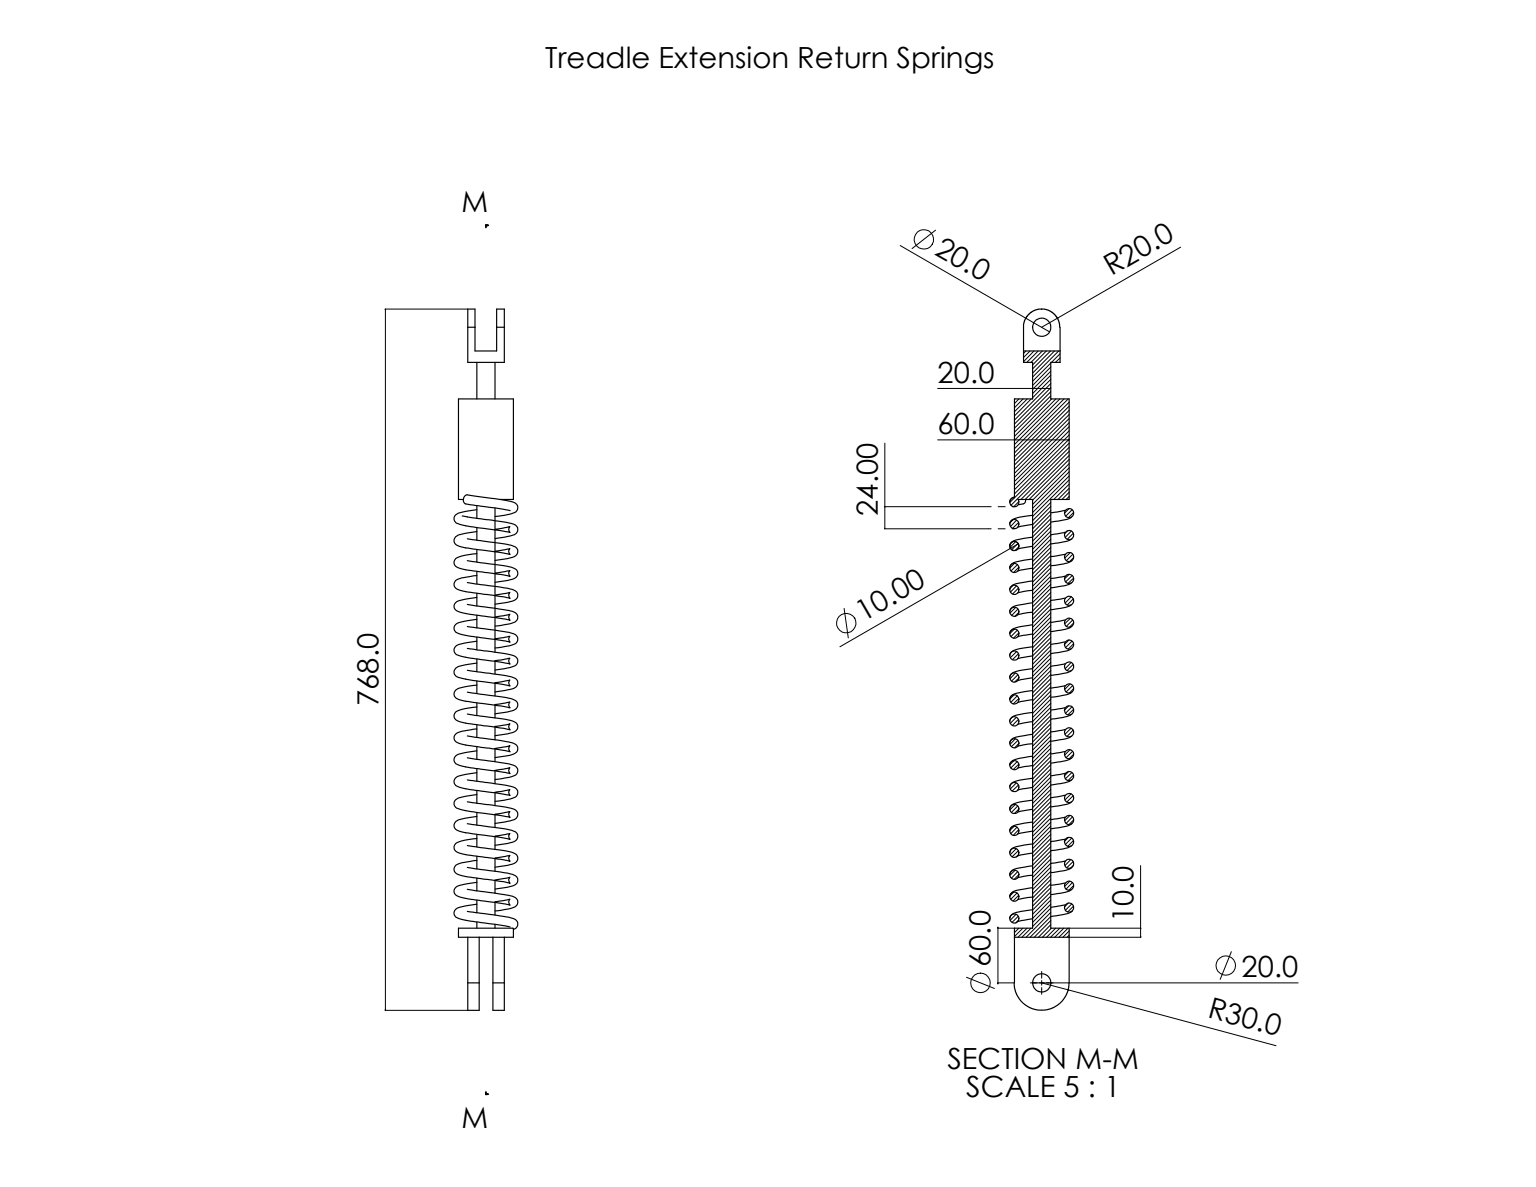
ISO-10303-21;
HEADER;
FILE_DESCRIPTION (('STEP AP214'),
    '1' );
FILE_NAME ('Treadle Extension Return Springs.step',
    '2026-10-21T17:07:05',
    ( '' ),
    ( '' ),
    'SwSTEP 2.0',
    'SolidWorks 2025',
    '' );
FILE_SCHEMA (( 'AUTOMOTIVE_DESIGN' ));
ENDSEC;

DATA;
#1=CARTESIAN_POINT ( 'NONE',  ( 745.1769319972822814, -41.80559628986934229, -346.2694204179732083 ) ) ;
#2=CARTESIAN_POINT ( 'NONE',  ( 764.0069404352550464, -207.0783235625960685, -359.2566176426627180 ) ) ;
#5=( BOUNDED_CURVE ( )  B_SPLINE_CURVE ( 2, ( #42977, #27813, #34735, #31272, #11342, #6564, #43210, #24332, #11582, #18730, #45142, #13500, #10036, #41910, #10254, #1170, #25872, #11803, #43435, #23072, #9239, #22634, #8789, #2069, #32818, #29794, #39983, #36732, #8332, #5090, #40437, #18964, #26092, #37170, #33058, #30023, #43655, #1395, #5529, #15499, #33484, #44108, #12472, #23310, #5303, #15279, #37412, #22395, #5769, #44335, #36499, #29579, #1830, #4863, #29365, #26551, #22857, #19625, #33720, #12025, #40649, #40206, #8568, #36950, #19181, #16161, #33266, #30243, #12690, #26770, #1612, #19399, #15711, #15939, #43874, #12253, #26333, #9002, #40875, #10150, #30713, #2768, #31156, #19857, #37866, #12929, #13166, #27016, #27245, #16861, #37632, #16626, #2991, #23530, #9913, #34150, #5983, #34634, #20075, #27462, #30941, #23985, #24225, #41115, #45034, #20540, #41337, #2520, #17078, #6462, #13390, #45254, #13613, #9467, #44568, #44809, #9687, #23751, #6212, #20305, #34397, #38106, #41560, #41801, #2288, #16387, #38333, #27697, #6679, #33937, #30466, #15422, #12398, #1747, #26925, #19779, #41028, #9388, #44026, #23223, #23455, #33195, #36878, #12841, #8717, #20002, #22552, #9151, #5912, #29712, #34079, #37554, #2216, #29500, #43572, #5445, #30169, #11940, #22783, #8482, #26008, #43789, #19319, #16085, #5228, #40579, #33403, #33863, #12618, #26252, #15629, #5690, #12171, #44260, #19540, #40117, #26477, #26696, #33635, #15854, #29942, #1532, #16310, #37328, #1988, #30392, #44485, #19108, #36657, #40365, #8925, #5017, #22995, #37090, #40793, #41950, #41259, #37788, #45414, #7068, #13775, #27854, #23906, #13537, #9837, #2443, #45176, #34552, #13999, #6822, #28067, #42163, #31078, #10291, #10514, #21149, #17466, #24367, #41720, #10074, #9615, #38471, #38706, #16781, #16545, #24589, #34998, #30630, #44725, #38254, #17221, #13088, #41483, #23677, #27171, #38027, #6137, #20227, #6382, #27611, #34315, #20901, #2684, #20678, #30861, #44955, #13312, #27388, #20463, #2911, #17001, #3131, #24145, #6600, #3375, #34768, #31548, #45650, #31306, #14912, #129, #7303, #25284, #14218, #22057, #14460, #39636, #15137, #18602, #39862, #7748, #17698, #21827, #3611, #28288, #42386, #10757, #25523, #11673, #10994, #31759, #24833, #4055, #29230, #32687, #35920, #38953, #25750, #43305, #11439, #28993, #21380, #32231, #8203, #35454, #4291, #35231, #3826, #25062, #1034, #28537, #17915, #39175, #7525, #810, #31985, #356, #42632, #21599, #35679, #18156, #591, #18382, #14693, #42848, #28769, #11215, #39397, #32462, #43074, #7991, #36147, #4509, #5627, #30330, #11887, #1692, #26638, #29661, #33579, #33143, #44424, #37267, #30115, #12115, #40065, #43737, #15796, #12561, #1930, #8664, #32923, #15579, #43521, #26859, #26196, #40311, #12778, #5175, #33808, #29886, #25959, #18831, #43973, #19052, #19721, #15367, #37036, #8426, #16253, #26424, #4729, #40734, #1268, #36823, #2162, #40968, #40524, #29448, #22271, #36367, #44203, #16033, #22495, #19261, #36606, #4960, #12348, #1479, #22726, #33350, #8875, #22939, #9090, #5388, #19482, #23158, #37501, #27335, #5861, #31026, #30804, #17168, #10234, #2854, #17407, #16481, #41428, #34247, #9779, #27554, #3076, #2380, #44662, #6543, #13939, #20623, #16947, #41658, #16720, #19950, #45124, #44897, #3310, #24083, #24313, #13482, #10013, #38197, #34717, #30561, #31253, #45591, #23620, #28014, #34943, #41890, #23399, #34025, #45354, #13715, #31489, #2620, #13023, #9330, #13257, #27113, #41203, #23846, #34494, #9560, #27793, #37729, #38418, #6081, #20168, #37958, #6317, #20845, #20399, #6769, #42797, #3555, #38648, #35867, #32175, #763, #32414, #42108, #21772, #7006, #14163, #538, #21093, #28940, #21320, #14864, #22007, #25464, #976, #14642, #24535, #28716, #10458, #35179, #17640, #31704, #43017, #18551, #17859, #71, #11382, #28234, #39119, #42329, #298, #10695, #31926, #3994, #24778, #35396, #39583, #38896, #39339, #7250, #3769, #7940, #14398, #11157, #25227, #28478, #32633, #42579, #18092, #18334, #10937, #25009, #36097, #4244, #7692, #4462, #15079, #7468, #21540, #35622, #32859, #18773, #4675, #11839, #29399, #22894, #25910, #9040, #11621, #25699, #5575, #40474, #4903, #40253, #36545, #29166, #26138, #15533, #40685, #33527, #23109, #37211, #12064, #36986, #19667, #2112, #19002, #39810, #40020, #29836, #36314, #8157, #5340, #19215, #1875, #19434, #43250, #8826, #22220, #22440, #1209, #33760, #33094, #1431, #15317, #8610, #12511, #43471, #15748, #8371, #43917, #29614, #43692, #22675, #36772, #15983, #5127, #33302, #12297, #30066, #26372, #44147, #26587, #45296, #34441, #12730, #41840, #38146, #9957, #23352, #13210, #13655, #31199, #41380, #9282, #23573, #30281, #41600, #13431, #38369, #37454, #23794, #6497, #6027, #33978, #20575, #37905, #37678, #24027, #17117, #9729, #24261, #5813, #2564, #41158, #16669, #2806, #16429, #34671, #12973, #10185, #44374, #26809, #6716, #27736, #20119, #40915, #6259, #34194, #20792, #30978, #34888, #20346, #16897, #16201, #2329, #45076, #19901, #30509, #30755, #44612, #9509, #27063, #44848, #27287, #39526, #31651, #27962, #45535, #21263, #38836, #42277, #17805, #32114, #25404, #10880, #31872, #24948, #19, #7189, #3939, #35342, #28417, #10637, #21712, #7881, #38590, #42515, #7635, #24718, #14584, #14111, #3251, #21957, #42058, #17343, #14805, #13888, #28184, #18033, #10406, #24483, #42736, #39063, #35809, #39280, #3718, #3493, #6945, #21028, #7411, #35116, #4185, #243, #18280, #28879, #32354, #31429, #21486, #17581, #35563, #14339, #479, #28658, #11100, #708, #25170, #42959, #11327, #5288, #36043, #33043, #43193, #39969, #11562, #25859, #43639, #22167, #29348, #40421, #36257, #33249, #1154, #4614, #26315, #18711, #4406, #1595, #15693, #12456, #29109, #12008, #12236, #8314, #8106, #8773, #29777, #22614, #22841, #36934, #39758, #15021, #32800, #15259, #25644, #43421, #8550, #11788, #43853, #22379, #15920, #18496, #32575, #26535, #19381, #36483, #1381, #4848, #918, #15484, #18947, #30004, #33466, #44091, #40633, #29564, #36714, #8986, #26072, #40185, #5074, #19165, #27679, #30228, #16845, #13596, #37396, #41784, #2973, #9895, #37153, #5512, #13149, #37848, #45236, #16371, #5968, #30698, #5750, #26999, #23738, #12911, #2504, #30448, #41543, #23054, #41322, #17062, #23968, #19608, #33701, #27230, #6197, #2051, #44551, #16145, #44794, #19839, #41095, #20288, #9450, #16610, #23514, #38090, #44319, #9672, #12674, #26754, #40858, #9220, #34618, #23295, #33921, #34381, #2272, #37615, #20058, #2750, #13373, #30924, #34135, #45020, #27446, #6445, #20524, #31139, #42687, #35062, #14529, #35753, #39233, #14755, #28354, #38317, #42458, #24207, #3194, #24897, #31372, #4132, #14285, #45710, #31822, #25119, #10134, #7134, #17283, #14062, #45480, #28134, #17758, #42010, #3436, #28605, #10354, #7362, #7586, #35293 ),
 .UNSPECIFIED., .F., .T. ) 
 B_SPLINE_CURVE_WITH_KNOTS ( ( 3, 2, 2, 2, 2, 2, 2, 2, 2, 2, 2, 2, 2, 2, 2, 2, 2, 2, 2, 2, 2, 2, 2, 2, 2, 2, 2, 2, 2, 2, 2, 2, 2, 2, 2, 2, 2, 2, 2, 2, 2, 2, 2, 2, 2, 2, 2, 2, 2, 2, 2, 2, 2, 2, 2, 2, 2, 2, 2, 2, 2, 2, 2, 2, 2, 2, 2, 2, 2, 2, 2, 2, 2, 2, 2, 2, 2, 2, 2, 2, 2, 2, 2, 2, 2, 2, 2, 2, 2, 2, 2, 2, 2, 2, 2, 2, 2, 2, 2, 2, 2, 2, 2, 2, 2, 2, 2, 2, 2, 2, 2, 2, 2, 2, 2, 2, 2, 2, 2, 2, 2, 2, 2, 2, 2, 2, 2, 2, 2, 2, 2, 2, 2, 2, 2, 2, 2, 2, 2, 2, 2, 2, 2, 2, 2, 2, 2, 2, 2, 2, 2, 2, 2, 2, 2, 2, 2, 2, 2, 2, 2, 2, 2, 2, 2, 2, 2, 2, 2, 2, 2, 2, 2, 2, 2, 2, 2, 2, 2, 2, 2, 2, 2, 2, 2, 2, 2, 2, 2, 2, 2, 2, 2, 2, 2, 2, 2, 2, 2, 2, 2, 2, 2, 2, 2, 2, 2, 2, 2, 2, 2, 2, 2, 2, 2, 2, 2, 2, 2, 2, 2, 2, 2, 2, 2, 2, 2, 2, 2, 2, 2, 2, 2, 2, 2, 2, 2, 2, 2, 2, 2, 2, 2, 2, 2, 2, 2, 2, 2, 2, 2, 2, 2, 2, 2, 2, 2, 2, 2, 2, 2, 2, 2, 2, 2, 2, 2, 2, 2, 2, 2, 2, 2, 2, 2, 2, 2, 2, 2, 2, 2, 2, 2, 2, 2, 2, 2, 2, 2, 2, 2, 2, 2, 2, 2, 2, 2, 2, 2, 2, 2, 2, 2, 2, 2, 2, 2, 2, 2, 2, 2, 2, 2, 2, 2, 2, 2, 2, 2, 2, 2, 2, 2, 2, 2, 2, 2, 2, 2, 2, 2, 2, 2, 2, 2, 2, 2, 2, 2, 2, 2, 2, 2, 2, 2, 2, 2, 2, 2, 2, 2, 2, 2, 2, 2, 2, 2, 2, 2, 2, 2, 2, 2, 2, 2, 2, 2, 2, 2, 2, 2, 2, 2, 2, 2, 2, 2, 2, 2, 2, 2, 2, 2, 2, 2, 2, 2, 2, 2, 2, 2, 2, 2, 2, 2, 2, 2, 2, 2, 2, 2, 2, 2, 2, 2, 2, 2, 2, 2, 2, 2, 2, 2, 2, 2, 2, 2, 2, 2, 2, 2, 2, 2, 2, 2, 2, 2, 2, 2, 2, 2, 3 ),
 ( 0.000000000000000000, 0.002272727272727272617, 0.004545454545454545234, 0.006818181818181817851, 0.009090909090909090468, 0.01136363636363636395, 0.01363636363636363570, 0.01590909090909090745, 0.01818181818181818094, 0.02045454545454545442, 0.02272727272727272790, 0.02500000000000000139, 0.02727272727272727140, 0.02954545454545454489, 0.03181818181818181490, 0.03409090909090908839, 0.03636363636363636187, 0.03863636363636363535, 0.04090909090909090884, 0.04318181818181818232, 0.04545454545454545581, 0.04772727272727272929, 0.05000000000000000278, 0.05227272727272727626, 0.05454545454545454281, 0.05681818181818181629, 0.05909090909090908977, 0.06136363636363636326, 0.06363636363636362980, 0.06590909090909090329, 0.06818181818181817677, 0.07045454545454545026, 0.07272727272727272374, 0.07499999999999999722, 0.07727272727272727071, 0.07954545454545454419, 0.08181818181818181768, 0.08409090909090909116, 0.08636363636363636465, 0.08863636363636363813, 0.09090909090909091161, 0.09318181818181818510, 0.09545454545454545858, 0.09772727272727273207, 0.1000000000000000056, 0.1022727272727272790, 0.1045454545454545525, 0.1068181818181818121, 0.1090909090909090856, 0.1113636363636363591, 0.1136363636363636326, 0.1159090909090909061, 0.1181818181818181795, 0.1204545454545454530, 0.1227272727272727265, 0.1250000000000000000, 0.1272727272727272596, 0.1295454545454545470, 0.1318181818181818066, 0.1340909090909090939, 0.1363636363636363535, 0.1386363636363636409, 0.1409090909090909005, 0.1431818181818181879, 0.1454545454545454475, 0.1477272727272727348, 0.1499999999999999944, 0.1522727272727272818, 0.1545454545454545414, 0.1568181818181818288, 0.1590909090909090884, 0.1613636363636363757, 0.1636363636363636354, 0.1659090909090909227, 0.1681818181818181823, 0.1704545454545454419, 0.1727272727272727293, 0.1749999999999999889, 0.1772727272727272763, 0.1795454545454545359, 0.1818181818181818232, 0.1840909090909090828, 0.1863636363636363702, 0.1886363636363636298, 0.1909090909090909172, 0.1931818181818181768, 0.1954545454545454641, 0.1977272727272727237, 0.2000000000000000111, 0.2022727272727272707, 0.2045454545454545581, 0.2068181818181818177, 0.2090909090909091050, 0.2113636363636363646, 0.2136363636363636243, 0.2159090909090909116, 0.2181818181818181712, 0.2204545454545454586, 0.2227272727272727182, 0.2250000000000000056, 0.2272727272727272652, 0.2295454545454545525, 0.2318181818181818121, 0.2340909090909090995, 0.2363636363636363591, 0.2386363636363636465, 0.2409090909090909061, 0.2431818181818181934, 0.2454545454545454530, 0.2477272727272727404, 0.2500000000000000000, 0.2522727272727272596, 0.2545454545454545192, 0.2568181818181818343, 0.2590909090909090939, 0.2613636363636363535, 0.2636363636363636131, 0.2659090909090909283, 0.2681818181818181879, 0.2704545454545454475, 0.2727272727272727071, 0.2750000000000000222, 0.2772727272727272818, 0.2795454545454545414, 0.2818181818181818010, 0.2840909090909091161, 0.2863636363636363757, 0.2886363636363636354, 0.2909090909090908950, 0.2931818181818181546, 0.2954545454545454697, 0.2977272727272727293, 0.2999999999999999889, 0.3022727272727272485, 0.3045454545454545636, 0.3068181818181818232, 0.3090909090909090828, 0.3113636363636363424, 0.3136363636363636576, 0.3159090909090909172, 0.3181818181818181768, 0.3204545454545454364, 0.3227272727272727515, 0.3250000000000000111, 0.3272727272727272707, 0.3295454545454545303, 0.3318181818181818454, 0.3340909090909090495, 0.3363636363636363646, 0.3386363636363636243, 0.3409090909090908839, 0.3431818181818181990, 0.3454545454545454586, 0.3477272727272727182, 0.3499999999999999778, 0.3522727272727272929, 0.3545454545454545525, 0.3568181818181818121, 0.3590909090909090717, 0.3613636363636363869, 0.3636363636363636465, 0.3659090909090909061, 0.3681818181818181657, 0.3704545454545454808, 0.3727272727272727404, 0.3750000000000000000, 0.3772727272727272596, 0.3795454545454545192, 0.3818181818181818343, 0.3840909090909090939, 0.3863636363636363535, 0.3886363636363636131, 0.3909090909090909283, 0.3931818181818181879, 0.3954545454545454475, 0.3977272727272727071, 0.4000000000000000222, 0.4022727272727272818, 0.4045454545454545414, 0.4068181818181818010, 0.4090909090909091161, 0.4113636363636363757, 0.4136363636363636354, 0.4159090909090908950, 0.4181818181818182101, 0.4204545454545454697, 0.4227272727272727293, 0.4249999999999999889, 0.4272727272727272485, 0.4295454545454545636, 0.4318181818181818232, 0.4340909090909090828, 0.4363636363636363424, 0.4386363636363636576, 0.4409090909090909172, 0.4431818181818181768, 0.4454545454545454364, 0.4477272727272727515, 0.4500000000000000111, 0.4522727272727272707, 0.4545454545454545303, 0.4568181818181818454, 0.4590909090909091050, 0.4613636363636363646, 0.4636363636363636243, 0.4659090909090908839, 0.4681818181818181990, 0.4704545454545454586, 0.4727272727272727182, 0.4749999999999999778, 0.4772727272727272929, 0.4795454545454545525, 0.4818181818181818121, 0.4840909090909090717, 0.4863636363636363869, 0.4886363636363636465, 0.4909090909090909061, 0.4931818181818181657, 0.4954545454545454808, 0.4977272727272727959, 0.5000000000000000000, 0.5022727272727273151, 0.5045454545454545192, 0.5068181818181818343, 0.5090909090909090384, 0.5113636363636363535, 0.5136363636363636687, 0.5159090909090908728, 0.5181818181818181879, 0.5204545454545455030, 0.5227272727272727071, 0.5250000000000000222, 0.5272727272727272263, 0.5295454545454545414, 0.5318181818181818565, 0.5340909090909090606, 0.5363636363636363757, 0.5386363636363636909, 0.5409090909090908950, 0.5431818181818182101, 0.5454545454545454142, 0.5477272727272727293, 0.5500000000000000444, 0.5522727272727272485, 0.5545454545454545636, 0.5568181818181817677, 0.5590909090909090828, 0.5613636363636363980, 0.5636363636363636020, 0.5659090909090909172, 0.5681818181818182323, 0.5704545454545454364, 0.5727272727272727515, 0.5749999999999999556, 0.5772727272727272707, 0.5795454545454545858, 0.5818181818181817899, 0.5840909090909089940, 0.5863636363636363091, 0.5886363636363636243, 0.5909090909090909394, 0.5931818181818181435, 0.5954545454545454586, 0.5977272727272727737, 0.5999999999999999778, 0.6022727272727272929, 0.6045454545454544970, 0.6068181818181818121, 0.6090909090909091272, 0.6113636363636363313, 0.6136363636363636465, 0.6159090909090909616, 0.6181818181818181657, 0.6204545454545454808, 0.6227272727272726849, 0.6250000000000000000, 0.6272727272727273151, 0.6295454545454545192, 0.6318181818181818343, 0.6340909090909090384, 0.6363636363636363535, 0.6386363636363636687, 0.6409090909090908728, 0.6431818181818181879, 0.6454545454545455030, 0.6477272727272727071, 0.6500000000000000222, 0.6522727272727272263, 0.6545454545454545414, 0.6568181818181818565, 0.6590909090909090606, 0.6613636363636363757, 0.6636363636363636909, 0.6659090909090908950, 0.6681818181818180991, 0.6704545454545454142, 0.6727272727272727293, 0.6750000000000000444, 0.6772727272727272485, 0.6795454545454545636, 0.6818181818181817677, 0.6840909090909090828, 0.6863636363636363980, 0.6886363636363636020, 0.6909090909090909172, 0.6931818181818182323, 0.6954545454545454364, 0.6977272727272727515, 0.6999999999999999556, 0.7022727272727272707, 0.7045454545454545858, 0.7068181818181817899, 0.7090909090909091050, 0.7113636363636363091, 0.7136363636363636243, 0.7159090909090909394, 0.7181818181818181435, 0.7204545454545454586, 0.7227272727272727737, 0.7249999999999999778, 0.7272727272727272929, 0.7295454545454544970, 0.7318181818181818121, 0.7340909090909091272, 0.7363636363636363313, 0.7386363636363636465, 0.7409090909090909616, 0.7431818181818181657, 0.7454545454545454808, 0.7477272727272726849, 0.7500000000000000000, 0.7522727272727273151, 0.7545454545454545192, 0.7568181818181818343, 0.7590909090909090384, 0.7613636363636363535, 0.7636363636363636687, 0.7659090909090908728, 0.7681818181818181879, 0.7704545454545455030, 0.7727272727272727071, 0.7750000000000000222, 0.7772727272727272263, 0.7795454545454545414, 0.7818181818181818565, 0.7840909090909090606, 0.7863636363636363757, 0.7886363636363636909, 0.7909090909090908950, 0.7931818181818182101, 0.7954545454545454142, 0.7977272727272727293, 0.8000000000000000444, 0.8022727272727272485, 0.8045454545454545636, 0.8068181818181817677, 0.8090909090909090828, 0.8113636363636363980, 0.8136363636363636020, 0.8159090909090909172, 0.8181818181818182323, 0.8204545454545454364, 0.8227272727272727515, 0.8249999999999999556, 0.8272727272727272707, 0.8295454545454545858, 0.8318181818181817899, 0.8340909090909091050, 0.8363636363636364202, 0.8386363636363636243, 0.8409090909090909394, 0.8431818181818181435, 0.8454545454545454586, 0.8477272727272727737, 0.8499999999999999778, 0.8522727272727272929, 0.8545454545454544970, 0.8568181818181818121, 0.8590909090909091272, 0.8613636363636363313, 0.8636363636363636465, 0.8659090909090909616, 0.8681818181818181657, 0.8704545454545454808, 0.8727272727272726849, 0.8750000000000000000, 0.8772727272727273151, 0.8795454545454545192, 0.8818181818181818343, 0.8840909090909090384, 0.8863636363636363535, 0.8886363636363636687, 0.8909090909090908728, 0.8931818181818181879, 0.8954545454545455030, 0.8977272727272727071, 0.9000000000000000222, 0.9022727272727272263, 0.9045454545454545414, 0.9068181818181818565, 0.9090909090909090606, 0.9113636363636363757, 0.9136363636363636909, 0.9159090909090908950, 0.9181818181818182101, 0.9204545454545453032, 0.9227272727272727293, 0.9250000000000000444, 0.9272727272727272485, 0.9295454545454545636, 0.9318181818181817677, 0.9340909090909090828, 0.9363636363636363980, 0.9386363636363636020, 0.9409090909090909172, 0.9431818181818182323, 0.9454545454545454364, 0.9477272727272727515, 0.9499999999999999556, 0.9522727272727272707, 0.9545454545454545858, 0.9568181818181817899, 0.9590909090909091050, 0.9613636363636363091, 0.9636363636363636243, 0.9659090909090909394, 0.9681818181818181435, 0.9704545454545454586, 0.9727272727272727737, 0.9749999999999999778, 0.9772727272727272929, 0.9779695260516495514 ),
 .UNSPECIFIED. ) 
 CURVE ( )  GEOMETRIC_REPRESENTATION_ITEM ( )  RATIONAL_B_SPLINE_CURVE ( ( 1.000000000000000000, 0.9898214418809326842, 1.000000000000000000, 0.9898214418809326842, 1.000000000000000000, 0.9898214418809326842, 1.000000000000000000, 0.9898214418809326842, 1.000000000000000000, 0.9898214418809326842, 1.000000000000000000, 0.9898214418809326842, 1.000000000000000000, 0.9898214418809326842, 1.000000000000000000, 0.9898214418809326842, 1.000000000000000000, 0.9898214418809326842, 1.000000000000000000, 0.9898214418809326842, 1.000000000000000000, 0.9898214418809326842, 1.000000000000000000, 0.9898214418809326842, 1.000000000000000000, 0.9898214418809326842, 1.000000000000000000, 0.9898214418809326842, 1.000000000000000000, 0.9898214418809326842, 1.000000000000000000, 0.9898214418809326842, 1.000000000000000000, 0.9898214418809326842, 1.000000000000000000, 0.9898214418809326842, 1.000000000000000000, 0.9898214418809326842, 1.000000000000000000, 0.9898214418809326842, 1.000000000000000000, 0.9898214418809326842, 1.000000000000000000, 0.9898214418809326842, 1.000000000000000000, 0.9898214418809326842, 1.000000000000000000, 0.9898214418809326842, 1.000000000000000000, 0.9898214418809326842, 1.000000000000000000, 0.9898214418809326842, 1.000000000000000000, 0.9898214418809326842, 1.000000000000000000, 0.9898214418809326842, 1.000000000000000000, 0.9898214418809326842, 1.000000000000000000, 0.9898214418809326842, 1.000000000000000000, 0.9898214418809326842, 1.000000000000000000, 0.9898214418809326842, 1.000000000000000000, 0.9898214418809326842, 1.000000000000000000, 0.9898214418809326842, 1.000000000000000000, 0.9898214418809326842, 1.000000000000000000, 0.9898214418809326842, 1.000000000000000000, 0.9898214418809326842, 1.000000000000000000, 0.9898214418809326842, 1.000000000000000000, 0.9898214418809326842, 1.000000000000000000, 0.9898214418809326842, 1.000000000000000000, 0.9898214418809326842, 1.000000000000000000, 0.9898214418809326842, 1.000000000000000000, 0.9898214418809326842, 1.000000000000000000, 0.9898214418809326842, 1.000000000000000000, 0.9898214418809326842, 1.000000000000000000, 0.9898214418809326842, 1.000000000000000000, 0.9898214418809326842, 1.000000000000000000, 0.9898214418809326842, 1.000000000000000000, 0.9898214418809326842, 1.000000000000000000, 0.9898214418809326842, 1.000000000000000000, 0.9898214418809326842, 1.000000000000000000, 0.9898214418809326842, 1.000000000000000000, 0.9898214418809326842, 1.000000000000000000, 0.9898214418809326842, 1.000000000000000000, 0.9898214418809326842, 1.000000000000000000, 0.9898214418809326842, 1.000000000000000000, 0.9898214418809326842, 1.000000000000000000, 0.9898214418809326842, 1.000000000000000000, 0.9898214418809326842, 1.000000000000000000, 0.9898214418809326842, 1.000000000000000000, 0.9898214418809326842, 1.000000000000000000, 0.9898214418809326842, 1.000000000000000000, 0.9898214418809326842, 1.000000000000000000, 0.9898214418809326842, 1.000000000000000000, 0.9898214418809326842, 1.000000000000000000, 0.9898214418809326842, 1.000000000000000000, 0.9898214418809326842, 1.000000000000000000, 0.9898214418809326842, 1.000000000000000000, 0.9898214418809326842, 1.000000000000000000, 0.9898214418809326842, 1.000000000000000000, 0.9898214418809326842, 1.000000000000000000, 0.9898214418809326842, 1.000000000000000000, 0.9898214418809326842, 1.000000000000000000, 0.9898214418809326842, 1.000000000000000000, 0.9898214418809326842, 1.000000000000000000, 0.9898214418809326842, 1.000000000000000000, 0.9898214418809326842, 1.000000000000000000, 0.9898214418809326842, 1.000000000000000000, 0.9898214418809326842, 1.000000000000000000, 0.9898214418809326842, 1.000000000000000000, 0.9898214418809326842, 1.000000000000000000, 0.9898214418809326842, 1.000000000000000000, 0.9898214418809326842, 1.000000000000000000, 0.9898214418809326842, 1.000000000000000000, 0.9898214418809326842, 1.000000000000000000, 0.9898214418809326842, 1.000000000000000000, 0.9898214418809326842, 1.000000000000000000, 0.9898214418809326842, 1.000000000000000000, 0.9898214418809326842, 1.000000000000000000, 0.9898214418809326842, 1.000000000000000000, 0.9898214418809326842, 1.000000000000000000, 0.9898214418809326842, 1.000000000000000000, 0.9898214418809326842, 1.000000000000000000, 0.9898214418809326842, 1.000000000000000000, 0.9898214418809326842, 1.000000000000000000, 0.9898214418809326842, 1.000000000000000000, 0.9898214418809326842, 1.000000000000000000, 0.9898214418809326842, 1.000000000000000000, 0.9898214418809326842, 1.000000000000000000, 0.9898214418809326842, 1.000000000000000000, 0.9898214418809326842, 1.000000000000000000, 0.9898214418809326842, 1.000000000000000000, 0.9898214418809326842, 1.000000000000000000, 0.9898214418809326842, 1.000000000000000000, 0.9898214418809326842, 1.000000000000000000, 0.9898214418809326842, 1.000000000000000000, 0.9898214418809326842, 1.000000000000000000, 0.9898214418809326842, 1.000000000000000000, 0.9898214418809326842, 1.000000000000000000, 0.9898214418809326842, 1.000000000000000000, 0.9898214418809326842, 1.000000000000000000, 0.9898214418809326842, 1.000000000000000000, 0.9898214418809326842, 1.000000000000000000, 0.9898214418809326842, 1.000000000000000000, 0.9898214418809326842, 1.000000000000000000, 0.9898214418809326842, 1.000000000000000000, 0.9898214418809326842, 1.000000000000000000, 0.9898214418809326842, 1.000000000000000000, 0.9898214418809326842, 1.000000000000000000, 0.9898214418809326842, 1.000000000000000000, 0.9898214418809326842, 1.000000000000000000, 0.9898214418809326842, 1.000000000000000000, 0.9898214418809326842, 1.000000000000000000, 0.9898214418809326842, 1.000000000000000000, 0.9898214418809326842, 1.000000000000000000, 0.9898214418809326842, 1.000000000000000000, 0.9898214418809326842, 1.000000000000000000, 0.9898214418809326842, 1.000000000000000000, 0.9898214418809326842, 1.000000000000000000, 0.9898214418809326842, 1.000000000000000000, 0.9898214418809326842, 1.000000000000000000, 0.9898214418809326842, 1.000000000000000000, 0.9898214418809326842, 1.000000000000000000, 0.9898214418809326842, 1.000000000000000000, 0.9898214418809326842, 1.000000000000000000, 0.9898214418809326842, 1.000000000000000000, 0.9898214418809326842, 1.000000000000000000, 0.9898214418809326842, 1.000000000000000000, 0.9898214418809326842, 1.000000000000000000, 0.9898214418809326842, 1.000000000000000000, 0.9898214418809326842, 1.000000000000000000, 0.9898214418809326842, 1.000000000000000000, 0.9898214418809326842, 1.000000000000000000, 0.9898214418809326842, 1.000000000000000000, 0.9898214418809326842, 1.000000000000000000, 0.9898214418809326842, 1.000000000000000000, 0.9898214418809326842, 1.000000000000000000, 0.9898214418809326842, 1.000000000000000000, 0.9898214418809326842, 1.000000000000000000, 0.9898214418809326842, 1.000000000000000000, 0.9898214418809326842, 1.000000000000000000, 0.9898214418809326842, 1.000000000000000000, 0.9898214418809326842, 1.000000000000000000, 0.9898214418809326842, 1.000000000000000000, 0.9898214418809326842, 1.000000000000000000, 0.9898214418809326842, 1.000000000000000000, 0.9898214418809326842, 1.000000000000000000, 0.9898214418809326842, 1.000000000000000000, 0.9898214418809326842, 1.000000000000000000, 0.9898214418809326842, 1.000000000000000000, 0.9898214418809326842, 1.000000000000000000, 0.9898214418809326842, 1.000000000000000000, 0.9898214418809326842, 1.000000000000000000, 0.9898214418809326842, 1.000000000000000000, 0.9898214418809326842, 1.000000000000000000, 0.9898214418809326842, 1.000000000000000000, 0.9898214418809326842, 1.000000000000000000, 0.9898214418809326842, 1.000000000000000000, 0.9898214418809326842, 1.000000000000000000, 0.9898214418809326842, 1.000000000000000000, 0.9898214418809326842, 1.000000000000000000, 0.9898214418809326842, 1.000000000000000000, 0.9898214418809326842, 1.000000000000000000, 0.9898214418809326842, 1.000000000000000000, 0.9898214418809326842, 1.000000000000000000, 0.9898214418809326842, 1.000000000000000000, 0.9898214418809326842, 1.000000000000000000, 0.9898214418809326842, 1.000000000000000000, 0.9898214418809326842, 1.000000000000000000, 0.9898214418809326842, 1.000000000000000000, 0.9898214418809326842, 1.000000000000000000, 0.9898214418809326842, 1.000000000000000000, 0.9898214418809326842, 1.000000000000000000, 0.9898214418809326842, 1.000000000000000000, 0.9898214418809326842, 1.000000000000000000, 0.9898214418809326842, 1.000000000000000000, 0.9898214418809326842, 1.000000000000000000, 0.9898214418809326842, 1.000000000000000000, 0.9898214418809326842, 1.000000000000000000, 0.9898214418809326842, 1.000000000000000000, 0.9898214418809326842, 1.000000000000000000, 0.9898214418809326842, 1.000000000000000000, 0.9898214418809326842, 1.000000000000000000, 0.9898214418809326842, 1.000000000000000000, 0.9898214418809326842, 1.000000000000000000, 0.9898214418809326842, 1.000000000000000000, 0.9898214418809326842, 1.000000000000000000, 0.9898214418809326842, 1.000000000000000000, 0.9898214418809326842, 1.000000000000000000, 0.9898214418809326842, 1.000000000000000000, 0.9898214418809326842, 1.000000000000000000, 0.9898214418809326842, 1.000000000000000000, 0.9898214418809326842, 1.000000000000000000, 0.9898214418809326842, 1.000000000000000000, 0.9898214418809326842, 1.000000000000000000, 0.9898214418809326842, 1.000000000000000000, 0.9898214418809326842, 1.000000000000000000, 0.9898214418809326842, 1.000000000000000000, 0.9898214418809326842, 1.000000000000000000, 0.9898214418809326842, 1.000000000000000000, 0.9898214418809326842, 1.000000000000000000, 0.9898214418809326842, 1.000000000000000000, 0.9898214418809326842, 1.000000000000000000, 0.9898214418809326842, 1.000000000000000000, 0.9898214418809326842, 1.000000000000000000, 0.9898214418809326842, 1.000000000000000000, 0.9898214418809326842, 1.000000000000000000, 0.9898214418809326842, 1.000000000000000000, 0.9898214418809326842, 1.000000000000000000, 0.9898214418809326842, 1.000000000000000000, 0.9898214418809326842, 1.000000000000000000, 0.9898214418809326842, 1.000000000000000000, 0.9898214418809326842, 1.000000000000000000, 0.9898214418809326842, 1.000000000000000000, 0.9898214418809326842, 1.000000000000000000, 0.9898214418809326842, 1.000000000000000000, 0.9898214418809326842, 1.000000000000000000, 0.9898214418809326842, 1.000000000000000000, 0.9898214418809326842, 1.000000000000000000, 0.9898214418809326842, 1.000000000000000000, 0.9898214418809326842, 1.000000000000000000, 0.9898214418809326842, 1.000000000000000000, 0.9898214418809326842, 1.000000000000000000, 0.9898214418809326842, 1.000000000000000000, 0.9898214418809326842, 1.000000000000000000, 0.9898214418809326842, 1.000000000000000000, 0.9898214418809326842, 1.000000000000000000, 0.9898214418809326842, 1.000000000000000000, 0.9898214418809326842, 1.000000000000000000, 0.9898214418809326842, 1.000000000000000000, 0.9898214418809326842, 1.000000000000000000, 0.9898214418809326842, 1.000000000000000000, 0.9898214418809326842, 1.000000000000000000, 0.9898214418809326842, 1.000000000000000000, 0.9898214418809326842, 1.000000000000000000, 0.9898214418809326842, 1.000000000000000000, 0.9898214418809326842, 1.000000000000000000, 0.9898214418809326842, 1.000000000000000000, 0.9898214418809326842, 1.000000000000000000, 0.9898214418809326842, 1.000000000000000000, 0.9898214418809326842, 1.000000000000000000, 0.9898214418809326842, 1.000000000000000000, 0.9898214418809326842, 1.000000000000000000, 0.9898214418809326842, 1.000000000000000000, 0.9898214418809326842, 1.000000000000000000, 0.9898214418809326842, 1.000000000000000000, 0.9898214418809326842, 1.000000000000000000, 0.9898214418809326842, 1.000000000000000000, 0.9898214418809326842, 1.000000000000000000, 0.9898214418809326842, 1.000000000000000000, 0.9898214418809326842, 1.000000000000000000, 0.9898214418809326842, 1.000000000000000000, 0.9898214418809326842, 1.000000000000000000, 0.9898214418809326842, 1.000000000000000000, 0.9898214418809326842, 1.000000000000000000, 0.9898214418809326842, 1.000000000000000000, 0.9898214418809326842, 1.000000000000000000, 0.9898214418809326842, 1.000000000000000000, 0.9898214418809326842, 1.000000000000000000, 0.9898214418809326842, 1.000000000000000000, 0.9898214418809326842, 1.000000000000000000, 0.9898214418809326842, 1.000000000000000000, 0.9898214418809326842, 1.000000000000000000, 0.9898214418809326842, 1.000000000000000000, 0.9898214418809326842, 1.000000000000000000, 0.9898214418809326842, 1.000000000000000000, 0.9898214418809326842, 1.000000000000000000, 0.9898214418809326842, 1.000000000000000000, 0.9898214418809326842, 1.000000000000000000, 0.9898214418809326842, 1.000000000000000000, 0.9898214418809326842, 1.000000000000000000, 0.9898214418809326842, 1.000000000000000000, 0.9898214418809326842, 1.000000000000000000, 0.9898214418809326842, 1.000000000000000000, 0.9898214418809326842, 1.000000000000000000, 0.9898214418809326842, 1.000000000000000000, 0.9898214418809326842, 1.000000000000000000, 0.9898214418809326842, 1.000000000000000000, 0.9898214418809326842, 1.000000000000000000, 0.9898214418809326842, 1.000000000000000000, 0.9898214418809326842, 1.000000000000000000, 0.9898214418809326842, 1.000000000000000000, 0.9898214418809326842, 1.000000000000000000, 0.9898214418809326842, 1.000000000000000000, 0.9898214418809326842, 1.000000000000000000, 0.9898214418809326842, 1.000000000000000000, 0.9898214418809326842, 1.000000000000000000, 0.9898214418809326842, 1.000000000000000000, 0.9898214418809326842, 1.000000000000000000, 0.9898214418809326842, 1.000000000000000000, 0.9898214418809326842, 1.000000000000000000, 0.9898214418809326842, 1.000000000000000000, 0.9898214418809326842, 1.000000000000000000, 0.9898214418809326842, 1.000000000000000000, 0.9898214418809326842, 1.000000000000000000, 0.9898214418809326842, 1.000000000000000000, 0.9898214418809326842, 1.000000000000000000, 0.9898214418809326842, 1.000000000000000000, 0.9898214418809326842, 1.000000000000000000, 0.9898214418809326842, 1.000000000000000000, 0.9898214418809326842, 1.000000000000000000, 0.9898214418809326842, 1.000000000000000000, 0.9898214418809326842, 1.000000000000000000, 0.9898214418809326842, 1.000000000000000000, 0.9898214418809326842, 1.000000000000000000, 0.9898214418809326842, 1.000000000000000000, 0.9898214418809326842, 1.000000000000000000, 0.9898214418809326842, 1.000000000000000000, 0.9898214418809326842, 1.000000000000000000, 0.9898214418809326842, 1.000000000000000000, 0.9898214418809326842, 1.000000000000000000, 0.9898214418809326842, 1.000000000000000000, 0.9898214418809326842, 1.000000000000000000, 0.9898214418809326842, 1.000000000000000000, 0.9898214418809326842, 1.000000000000000000, 0.9898214418809326842, 1.000000000000000000, 0.9898214418809326842, 1.000000000000000000, 0.9898214418809326842, 1.000000000000000000, 0.9898214418809326842, 1.000000000000000000, 0.9898214418809326842, 1.000000000000000000, 0.9898214418809326842, 1.000000000000000000, 0.9898214418809326842, 1.000000000000000000, 0.9898214418809326842, 1.000000000000000000, 0.9898214418809326842, 1.000000000000000000, 0.9898214418809326842, 1.000000000000000000, 0.9898214418809326842, 1.000000000000000000, 0.9898214418809326842, 1.000000000000000000, 0.9898214418809326842, 1.000000000000000000, 0.9898214418809326842, 1.000000000000000000, 0.9898214418809326842, 1.000000000000000000, 0.9898214418809326842, 1.000000000000000000, 0.9898214418809326842, 1.000000000000000000, 0.9898214418809326842, 1.000000000000000000, 0.9898214418809326842, 1.000000000000000000, 0.9898214418809326842, 1.000000000000000000, 0.9898214418809326842, 1.000000000000000000, 0.9898214418809326842, 1.000000000000000000, 0.9898214418809326842, 1.000000000000000000, 0.9898214418809326842, 1.000000000000000000, 0.9898214418809326842, 1.000000000000000000, 0.9898214418809326842, 1.000000000000000000, 0.9898214418809326842, 1.000000000000000000, 0.9898214418809326842, 1.000000000000000000, 0.9898214418809326842, 1.000000000000000000, 0.9898214418809326842, 1.000000000000000000, 0.9898214418809326842, 1.000000000000000000, 0.9898214418809326842, 1.000000000000000000, 0.9898214418809326842, 1.000000000000000000, 0.9898214418809326842, 1.000000000000000000, 0.9898214418809326842, 1.000000000000000000, 0.9898214418809326842, 1.000000000000000000, 0.9898214418809326842, 1.000000000000000000, 0.9898214418809326842, 1.000000000000000000, 0.9898214418809326842, 1.000000000000000000, 0.9898214418809326842, 1.000000000000000000, 0.9898214418809326842, 1.000000000000000000, 0.9898214418809326842, 1.000000000000000000, 0.9898214418809326842, 1.000000000000000000, 0.9898214418809326842, 1.000000000000000000, 0.9898214418809326842, 1.000000000000000000, 0.9898214418809326842, 1.000000000000000000, 0.9898214418809326842, 1.000000000000000000, 0.9898214418809326842, 1.000000000000000000, 0.9898214418809326842, 1.000000000000000000, 0.9898214418809326842, 1.000000000000000000, 0.9898214418809326842, 1.000000000000000000, 0.9898214418809326842, 1.000000000000000000, 0.9898214418809326842, 1.000000000000000000, 0.9898214418809326842, 1.000000000000000000, 0.9898214418809326842, 1.000000000000000000, 0.9898214418809326842, 1.000000000000000000, 0.9898214418809326842, 1.000000000000000000, 0.9898214418809326842, 1.000000000000000000, 0.9898214418809326842, 1.000000000000000000, 0.9898214418809326842, 1.000000000000000000, 0.9898214418809326842, 1.000000000000000000, 0.9898214418809326842, 1.000000000000000000, 0.9898214418809326842, 1.000000000000000000, 0.9898214418809326842, 1.000000000000000000, 0.9898214418809326842, 1.000000000000000000, 0.9898214418809326842, 1.000000000000000000, 0.9898214418809326842, 1.000000000000000000, 0.9898214418809326842, 1.000000000000000000, 0.9898214418809326842, 1.000000000000000000, 0.9898214418809326842, 1.000000000000000000, 0.9898214418809326842, 1.000000000000000000, 0.9898214418809326842, 1.000000000000000000, 0.9898214418809326842, 1.000000000000000000, 0.9898214418809326842, 1.000000000000000000, 0.9898214418809326842, 1.000000000000000000, 0.9898214418809326842, 1.000000000000000000, 0.9898214418809326842, 1.000000000000000000, 0.9898214418809326842, 1.000000000000000000, 0.9898214418809326842, 1.000000000000000000, 0.9898214418809326842, 1.000000000000000000, 0.9898214418809326842, 1.000000000000000000, 0.9898214418809326842, 1.000000000000000000, 0.9898214418809326842, 1.000000000000000000, 0.9898214418809326842, 1.000000000000000000, 0.9898214418809326842, 1.000000000000000000, 0.9898214418809326842, 1.000000000000000000, 0.9898214418809326842, 1.000000000000000000, 0.9898214418809326842, 1.000000000000000000, 0.9898214418809326842, 1.000000000000000000, 0.9898214418809326842, 1.000000000000000000, 0.9898214418809326842, 1.000000000000000000, 0.9898214418809326842, 1.000000000000000000, 0.9898214418809326842, 1.000000000000000000, 0.9898214418809326842, 1.000000000000000000, 0.9898214418809326842, 1.000000000000000000, 0.9898214418809326842, 1.000000000000000000, 0.9898214418809326842, 1.000000000000000000, 0.9898214418809326842, 1.000000000000000000, 0.9898214418809326842, 1.000000000000000000, 0.9898214418809326842, 1.000000000000000000, 0.9898214418809326842, 1.000000000000000000, 0.9898214418809326842, 1.000000000000000000, 0.9898214418809326842, 1.000000000000000000, 0.9898214418809326842, 1.000000000000000000, 0.9898214418809326842, 1.000000000000000000, 0.9968793409778355930, 0.9956722167842187998 ) ) 
 REPRESENTATION_ITEM ( '' )  );
#7=CARTESIAN_POINT ( 'NONE',  ( 770.0799878456142551, -205.9874144716870035, -362.9823548866085616 ) ) ;
#9=CARTESIAN_POINT ( 'NONE',  ( 768.8385539511368734, -47.26014174441477422, -306.4236121716840557 ) ) ;
#14=CARTESIAN_POINT ( 'NONE',  ( 786.2694204179717872, -309.2817908451525568, -305.1769319972829067 ) ) ;
#17=CARTESIAN_POINT ( 'NONE',  ( 758.4439275373578084, -156.5545181178802636, -353.2243759319684386 ) ) ;
#18=CARTESIAN_POINT ( 'NONE',  ( 804.9363028652555840, -160.2709662947836762, -338.2165204200192079 ) ) ;
#19=CARTESIAN_POINT ( 'NONE',  ( 755.3201227861273992, -339.7255117493285184, -345.3687786644892981 ) ) ;
#24=CARTESIAN_POINT ( 'NONE',  ( 787.4999999999992042, -462.9681489794447202, -270.0000000000000568 ) ) ;
#28=CARTESIAN_POINT ( 'NONE',  ( 799.9636004259356241, -382.9181544815159555, -311.2241431872006956 ) ) ;
#32=CARTESIAN_POINT ( 'NONE',  ( 804.4286716492782716, -377.3618753856920875, -345.3141322388244703 ) ) ;
#34=CARTESIAN_POINT ( 'NONE',  ( 755.5913626894240451, -229.6454272087890729, -346.6156483768012890 ) ) ;
#37=CARTESIAN_POINT ( 'NONE',  ( 796.7737145352015204, -404.6346026584193396, -370.7187646348536987 ) ) ;
#43=CARTESIAN_POINT ( 'NONE',  ( 812.7932403749906598, -39.18005720387496638, -327.7687537140311633 ) ) ;
#44=CARTESIAN_POINT ( 'NONE',  ( 803.6646147819161570, -281.9073299311468759, -348.8264449731210561 ) ) ;
#48=CARTESIAN_POINT ( 'NONE',  ( 773.7305795820266212, -33.28179084515333130, -374.8230680027170365 ) ) ;
#49=CARTESIAN_POINT ( 'NONE',  ( 760.5453621957607311, -93.07832356259645223, -323.8424801807151425 ) ) ;
#55=CARTESIAN_POINT ( 'NONE',  ( 793.2243759319678702, -98.53286901714187707, -318.4439275373583200 ) ) ;
#57=CARTESIAN_POINT ( 'NONE',  ( 794.9819416627830151, -84.99823902205663728, -319.9864689768909898 ) ) ;
#58=CARTESIAN_POINT ( 'NONE',  ( 805.1016975059191054, -390.8965053807772279, -343.0745993439771837 ) ) ;
#62=CARTESIAN_POINT ( 'NONE',  ( 791.1614460488616487, -395.2601417444136587, -373.5763878283158874 ) ) ;
#67=CARTESIAN_POINT ( 'NONE',  ( 814.5518280994195948, -255.7255117493287742, -332.4837098697145734 ) ) ;
#71=CARTESIAN_POINT ( 'NONE',  ( 755.5713283507202505, -245.3618753856925139, -334.6858677611754729 ) ) ;
#72=ORIENTED_EDGE ( 'NONE', *, *, #44085, .T. ) ;
#73=CARTESIAN_POINT ( 'NONE',  ( 767.8955696845333705, -360.4527844766010958, -362.1676090361162323 ) ) ;
#74=CARTESIAN_POINT ( 'NONE',  ( 778.2165204200184689, -22.81642084023865280, -364.9363028652563230 ) ) ;
#81=CARTESIAN_POINT ( 'NONE',  ( 768.0187753319979720, -32.63460265842044095, -318.0580252608186242 ) ) ;
#83=CARTESIAN_POINT ( 'NONE',  ( 745.7194118038753459, -277.6454272087889308, -348.7631598425976449 ) ) ;
#86=CARTESIAN_POINT ( 'NONE',  ( 795.1360043628807261, -212.0891481129652902, -360.2193346964456282 ) ) ;
#87=CARTESIAN_POINT ( 'NONE',  ( 787.6308680596127942, -395.2601417444136587, -364.1105419155492768 ) ) ;
#89=CARTESIAN_POINT ( 'NONE',  ( 779.4763451958990572, -104.7363362996985785, -365.0264073115438919 ) ) ;
#93=CARTESIAN_POINT ( 'NONE',  ( 745.1769319972822814, 6.194403710130517382, -346.2694204179732083 ) ) ;
#94=CARTESIAN_POINT ( 'NONE',  ( 792.2312462859673587, -323.9073299311468190, -307.2067596250082602 ) ) ;
#97=CARTESIAN_POINT ( 'NONE',  ( 771.2633955100217236, -71.90732993114760063, -363.4237431249939618 ) ) ;
#99=CARTESIAN_POINT ( 'NONE',  ( 793.4146539503750546, -193.9874144716870319, -307.6481478633938877 ) ) ;
#101=CARTESIAN_POINT ( 'NONE',  ( 792.2312462859673587, -443.9073299311464780, -307.2067596250082602 ) ) ;
#105=ADVANCED_FACE ( 'NONE', ( #37931 ), #16695, .F. ) ;
#106=CARTESIAN_POINT ( 'NONE',  ( 803.6646147819161570, -449.9073299311463643, -348.8264449731210561 ) ) ;
#107=CARTESIAN_POINT ( 'NONE',  ( 779.9999999999992042, -462.9681489794448339, -370.0000000000000568 ) ) ;
#113=CARTESIAN_POINT ( 'NONE',  ( 756.1348686366196716, -305.2601417444139429, -347.5531968255698416 ) ) ;
#117=CARTESIAN_POINT ( 'NONE',  ( 749.8865473780648472, -284.5328690171412518, -322.1177392798429082 ) ) ;
#122=CARTESIAN_POINT ( 'NONE',  ( 803.8651313633788504, -53.26014174441475291, -332.4468031744301015 ) ) ;
#123=CARTESIAN_POINT ( 'NONE',  ( 756.5762568750052424, -147.1800572038746395, -348.7366044899774238 ) ) ;
#124=CARTESIAN_POINT ( 'NONE',  ( 797.8594530101008786, -205.5436935675108430, -322.1405469898980982 ) ) ;
#126=CARTESIAN_POINT ( 'NONE',  ( 745.7998596910086917, -149.3618753856928265, -332.5602148656461168 ) ) ;
#129=CARTESIAN_POINT ( 'NONE',  ( 755.5713283507202505, -125.3618753856928834, -334.6858677611754729 ) ) ;
#131=CARTESIAN_POINT ( 'NONE',  ( 800.9840315886518738, -388.9181544815158986, -354.1144889064786412 ) ) ;
#140=CARTESIAN_POINT ( 'NONE',  ( 772.4468031744293057, -393.8272453906067199, -363.8651313633793620 ) ) ;
#141=CARTESIAN_POINT ( 'NONE',  ( 756.3353852180819104, -365.9073299311465917, -331.1735550268788302 ) ) ;
#142=CARTESIAN_POINT ( 'NONE',  ( 781.2370466360911223, -164.7363362996983938, -304.9990715423533629 ) ) ;
#146=CARTESIAN_POINT ( 'NONE',  ( 805.0264073115434940, -294.3510508353230648, -339.4763451958999099 ) ) ;
#147=CARTESIAN_POINT ( 'NONE',  ( 803.6646147819161570, -449.9073299311463643, -348.8264449731210561 ) ) ;
#148=CARTESIAN_POINT ( 'NONE',  ( 802.2119215644370342, -150.0090635724257027, -367.5423716828165084 ) ) ;
#151=EDGE_CURVE ( 'NONE', #10014, #17032, #19697, .T. ) ;
#154=CARTESIAN_POINT ( 'NONE',  ( 749.2812353651451076, -198.4527844766017495, -323.2262854647983090 ) ) ;
#158=CARTESIAN_POINT ( 'NONE',  ( 746.7653713866222915, -113.2601417444145682, -351.0478386215610271 ) ) ;
#160=CARTESIAN_POINT ( 'NONE',  ( 754.9967657858570647, -337.5436935675102177, -365.0032342141425374 ) ) ;
#166=CARTESIAN_POINT ( 'NONE',  ( 791.1614460488616487, -395.2601417444136587, -373.5763878283158874 ) ) ;
#167=CARTESIAN_POINT ( 'NONE',  ( 745.7998596910086917, -413.3618753856920307, -332.5602148656461168 ) ) ;
#172=CARTESIAN_POINT ( 'NONE',  ( 776.2433038121456548, -180.8965053807779952, -374.8207195650711014 ) ) ;
#177=CARTESIAN_POINT ( 'NONE',  ( 747.2067596250078623, -27.18005720387500901, -352.2312462859687230 ) ) ;
#181=CARTESIAN_POINT ( 'NONE',  ( 810.4231160770870019, -456.5545181178792404, -321.9338519418446936 ) ) ;
#182=ORIENTED_EDGE ( 'NONE', *, *, #32039, .F. ) ;
#186=CARTESIAN_POINT ( 'NONE',  ( 785.3141322388236176, -285.7255117493286889, -364.4286716492789537 ) ) ;
#191=CARTESIAN_POINT ( 'NONE',  ( 799.2566176426618085, -264.0090635724253616, -324.0069404352559559 ) ) ;
#192=CARTESIAN_POINT ( 'NONE',  ( 778.2165204200184689, -238.8164208402379813, -364.9363028652563230 ) ) ;
#194=CARTESIAN_POINT ( 'NONE',  ( 800.0135310231082713, -110.0891481129656597, -325.0180583372163028 ) ) ;
#198=CARTESIAN_POINT ( 'NONE',  ( 791.7608162188021197, 205.0000000000000568, -339.9999999999999432 ) ) ;
#199=CARTESIAN_POINT ( 'NONE',  ( 755.8990559732751535, -35.46360902697151829, -365.9055244015606831 ) ) ;
#200=CARTESIAN_POINT ( 'NONE',  ( 779.9999999999992042, 16.45630643248849267, -339.9999999999999432 ) ) ;
#206=CARTESIAN_POINT ( 'NONE',  ( 780.5236548040995785, 3.263663700301089765, -314.9735926884559944 ) ) ;
#207=CARTESIAN_POINT ( 'NONE',  ( 808.3070685750232087, -114.9982390220565378, -361.1904061080339829 ) ) ;
#211=CARTESIAN_POINT ( 'NONE',  ( 796.9462024416508257, -228.4527844766015789, -308.9653473494370246 ) ) ;
#216=CARTESIAN_POINT ( 'NONE',  ( 773.7943932421234194, -287.8055962898685038, -305.5313806188329409 ) ) ;
#218=CARTESIAN_POINT ( 'NONE',  ( 749.2812353651451076, -318.4527844766014368, -323.2262854647983090 ) ) ;
#219=LINE ( 'NONE', #30953, #25011 ) ;
#222=CARTESIAN_POINT ( 'NONE',  ( 756.5762568750052424, -387.1800572038738437, -348.7366044899774238 ) ) ;
#224=CARTESIAN_POINT ( 'NONE',  ( 755.0636971347428243, -196.2709662947835909, -341.7834795799807353 ) ) ;
#225=CARTESIAN_POINT ( 'NONE',  ( 776.2433038121456548, -84.89650538077830788, -374.8207195650711014 ) ) ;
#229=CARTESIAN_POINT ( 'NONE',  ( 779.4709603349208464, -216.3510508353233490, -314.7162404726379918 ) ) ;
#231=CARTESIAN_POINT ( 'NONE',  ( 798.0661480581538854, -50.53286901714203339, -309.5768839229118043 ) ) ;
#233=CARTESIAN_POINT ( 'NONE',  ( 808.9106007788763009, -452.9681489794446065, -335.7521713694408731 ) ) ;
#237=CARTESIAN_POINT ( 'NONE',  ( 814.8207195650702488, -338.1908817542433212, -336.2433038121456548 ) ) ;
#240=CARTESIAN_POINT ( 'NONE',  ( 754.7162404726377645, -134.7363362996984790, -339.4709603349214717 ) ) ;
#241=CARTESIAN_POINT ( 'NONE',  ( 801.9419747391806368, -162.4527844766018632, -351.9812246680014027 ) ) ;
#243=CARTESIAN_POINT ( 'NONE',  ( 778.2165204200184689, -358.8164208402375834, -364.9363028652563230 ) ) ;
#244=ORIENTED_EDGE ( 'NONE', *, *, #43927, .T. ) ;
#253=CARTESIAN_POINT ( 'NONE',  ( 810.4231160770870019, -384.5545181178795247, -321.9338519418446936 ) ) ;
#254=CARTESIAN_POINT ( 'NONE',  ( 782.4968714119720516, 13.18357915976123174, -305.0891759886411023 ) ) ;
#257=CARTESIAN_POINT ( 'NONE',  ( 771.2633955100217236, -359.9073299311467053, -363.4237431249939618 ) ) ;
#261=CARTESIAN_POINT ( 'NONE',  ( 784.1219089521767955, -237.2817908451526421, -315.0488828828318333 ) ) ;
#264=CARTESIAN_POINT ( 'NONE',  ( 779.9999999999992042, 126.4563064324884465, -329.9999999999999432 ) ) ;
#265=CARTESIAN_POINT ( 'NONE',  ( 808.3070685750232087, -426.9982390220555430, -361.1904061080339829 ) ) ;
#269=CARTESIAN_POINT ( 'NONE',  ( 809.4421496042219815, -454.3218287316016699, -345.7584569706272077 ) ) ;
#271=CARTESIAN_POINT ( 'NONE',  ( 796.9462024416508257, -60.45278447660215448, -308.9653473494370246 ) ) ;
#272=CARTESIAN_POINT ( 'NONE',  ( 758.0580252608178853, -270.4527844766014937, -328.0187753319985404 ) ) ;
#276=CARTESIAN_POINT ( 'NONE',  ( 764.1737431748507561, -58.37269993606236085, -371.6461892240376415 ) ) ;
#277=CARTESIAN_POINT ( 'NONE',  ( 803.8651313633788504, -77.26014174441466764, -332.4468031744301015 ) ) ;
#280=VECTOR ( 'NONE', #1161, 1000.000000000000000 ) ;
#283=CARTESIAN_POINT ( 'NONE',  ( 771.2633955100217236, -95.90732993114751537, -363.4237431249939618 ) ) ;
#284=CARTESIAN_POINT ( 'NONE',  ( 803.8651313633788504, -389.2601417444136018, -332.4468031744301015 ) ) ;
#287=CARTESIAN_POINT ( 'NONE',  ( 793.4146539503750546, -409.9874144716863498, -307.6481478633938877 ) ) ;
#293=CARTESIAN_POINT ( 'NONE',  ( 796.7737145352015204, -260.6346026584197375, -370.7187646348536987 ) ) ;
#298=CARTESIAN_POINT ( 'NONE',  ( 764.8639956371174549, -248.0891481129651766, -319.7806653035542581 ) ) ;
#300=CARTESIAN_POINT ( 'NONE',  ( 788.7366044899766848, -371.9073299311465917, -316.5762568750059813 ) ) ;
#301=CARTESIAN_POINT ( 'NONE',  ( 759.7806653035534055, -30.99823902205680071, -324.8639956371180801 ) ) ;
#304=FACE_OUTER_BOUND ( 'NONE', #10068, .T. ) ;
#306=CARTESIAN_POINT ( 'NONE',  ( 794.9819416627830151, -12.99823902205686821, -319.9864689768909898 ) ) ;
#310=CARTESIAN_POINT ( 'NONE',  ( 799.9636004259356241, -262.9181544815162965, -311.2241431872006956 ) ) ;
#313=CARTESIAN_POINT ( 'NONE',  ( 800.0135310231082713, -254.0891481129652334, -325.0180583372163028 ) ) ;
#314=CARTESIAN_POINT ( 'NONE',  ( 789.9200121543843807, -385.9874144716864066, -317.0176451133914384 ) ) ;
#316=CARTESIAN_POINT ( 'NONE',  ( 763.0428371773158460, -131.4636090269711985, -358.7617431975195359 ) ) ;
#319=CARTESIAN_POINT ( 'NONE',  ( 808.7758568127978833, -4.169232653505813069, -320.0363995740631822 ) ) ;
#320=CARTESIAN_POINT ( 'NONE',  ( 777.4774526936600978, -322.2709662947830793, -304.7301800767028226 ) ) ;
#321=CARTESIAN_POINT ( 'NONE',  ( 759.9999999999992042, 205.0000000000000568, -360.0000000000000000 ) ) ;
#325=CARTESIAN_POINT ( 'NONE',  ( 813.2346286133761168, -197.2601417444143124, -328.9521613784389160 ) ) ;
#327=CARTESIAN_POINT ( 'NONE',  ( 755.2512626584698410, -439.5436935675101040, -315.2512626584710915 ) ) ;
#333=CARTESIAN_POINT ( 'NONE',  ( 790.8050863131179540, -452.8379544210779954, -362.5841948692291226 ) ) ;
#339=VECTOR ( 'NONE', #33787, 1000.000000000000000 ) ;
#340=CARTESIAN_POINT ( 'NONE',  ( 757.2208543904082489, -304.7146871989594388, -350.9844846989624330 ) ) ;
#342=AXIS2_PLACEMENT_3D ( 'NONE', #45315, #17601, #13908 ) ;
#343=CARTESIAN_POINT ( 'NONE',  ( 766.5853460496234675, -301.9874144716867477, -372.3518521366060554 ) ) ;
#349=CARTESIAN_POINT ( 'NONE',  ( 755.5713283507202505, -149.3618753856928265, -334.6858677611754729 ) ) ;
#350=CARTESIAN_POINT ( 'NONE',  ( 759.7806653035534055, -222.9982390220561399, -324.8639956371180801 ) ) ;
#353=CARTESIAN_POINT ( 'NONE',  ( 745.4481719005789273, -147.7255117493291152, -347.5162901302853129 ) ) ;
#356=CARTESIAN_POINT ( 'NONE',  ( 758.0580252608178853, -150.4527844766018916, -328.0187753319985404 ) ) ;
#358=CARTESIAN_POINT ( 'NONE',  ( 790.9844846989617508, -406.3726999360612808, -317.2208543904092721 ) ) ;
#368=CARTESIAN_POINT ( 'NONE',  ( 761.4292242960306112, -377.4636090269704596, -323.2154366446414429 ) ) ;
#370=CARTESIAN_POINT ( 'NONE',  ( 755.8990559732751535, -179.4636090269710849, -365.9055244015606831 ) ) ;
#374=CARTESIAN_POINT ( 'NONE',  ( 761.2382568024794409, -303.6237781080503169, -356.9571628226838129 ) ) ;
#375=CARTESIAN_POINT ( 'NONE',  ( 800.2193346964447755, -450.9982390220554294, -355.1360043628815788 ) ) ;
#376=CARTESIAN_POINT ( 'NONE',  ( 791.0478386215596629, -189.8272453906073736, -306.7653713866226326 ) ) ;
#383=CARTESIAN_POINT ( 'NONE',  ( 767.7687537140311633, -215.9073299311471317, -372.7932403749916830 ) ) ;
#388=CARTESIAN_POINT ( 'NONE',  ( 807.5423716828161105, -105.0783235625964096, -362.2119215644372048 ) ) ;
#390=CARTESIAN_POINT ( 'NONE',  ( 814.5518280994195948, -351.7255117493284047, -332.4837098697145734 ) ) ;
#392=CARTESIAN_POINT ( 'NONE',  ( 758.7867965644027208, 16.45630643248849267, -318.7867965644036872 ) ) ;
#395=CARTESIAN_POINT ( 'NONE',  ( 752.4576283171824116, -405.0783235625954148, -317.7880784355627952 ) ) ;
#397=CARTESIAN_POINT ( 'NONE',  ( 747.2067596250078623, -411.1800572038738437, -352.2312462859687230 ) ) ;
#401=AXIS2_PLACEMENT_3D ( 'NONE', #14674, #35902, #42831 ) ;
#403=CARTESIAN_POINT ( 'NONE',  ( 764.3348316497523456, -190.7146871989597798, -308.6759233522265617 ) ) ;
#410=CARTESIAN_POINT ( 'NONE',  ( 748.9653473494363425, -26.63460265842045871, -356.9462024416521331 ) ) ;
#414=CARTESIAN_POINT ( 'NONE',  ( 797.8822607201568644, -438.5545181178793541, -370.1134526219340160 ) ) ;
#418=CARTESIAN_POINT ( 'NONE',  ( 781.8018195045266339, -286.2709662947833635, -365.1927285166406705 ) ) ;
#422=CARTESIAN_POINT ( 'NONE',  ( 763.0428371773158460, -275.4636090269708575, -358.7617431975195359 ) ) ;
#423=CARTESIAN_POINT ( 'NONE',  ( 804.9363028652555840, -256.2709662947834204, -338.2165204200192079 ) ) ;
#425=CARTESIAN_POINT ( 'NONE',  ( 781.7834795799800531, -130.8164208402383224, -315.0636971347436202 ) ) ;
#432=CARTESIAN_POINT ( 'NONE',  ( 745.1792804349281596, -86.19088175424408860, -343.7566961878542884 ) ) ;
#439=CARTESIAN_POINT ( 'NONE',  ( 804.1105419155481968, -51.82724539060782121, -347.6308680596136469 ) ) ;
#440=CARTESIAN_POINT ( 'NONE',  ( 763.2262854647970016, -104.6346026584202207, -309.2812353651462445 ) ) ;
#447=CARTESIAN_POINT ( 'NONE',  ( 748.3538107759620743, -304.7146871989594388, -355.8262568251490165 ) ) ;
#451=CARTESIAN_POINT ( 'NONE',  ( 801.1904061080336987, -308.0891481129650629, -368.3070685750235498 ) ) ;
#456=CARTESIAN_POINT ( 'NONE',  ( 774.6858677611749044, -393.7255117493283478, -315.5713283507209894 ) ) ;
#459=CARTESIAN_POINT ( 'NONE',  ( 791.1614460488616487, -83.26014174441466764, -373.5763878283158874 ) ) ;
#462=VECTOR ( 'NONE', #12893, 1000.000000000000000 ) ;
#464=CARTESIAN_POINT ( 'NONE',  ( 779.4709603349208464, -192.3510508353233774, -314.7162404726379918 ) ) ;
#468=CARTESIAN_POINT ( 'NONE',  ( 813.9316612368132837, -31.44195992623299674, -348.6739635108323228 ) ) ;
#474=CARTESIAN_POINT ( 'NONE',  ( 754.3581564841646241, -353.4636090269705733, -316.1443688327762516 ) ) ;
#477=CARTESIAN_POINT ( 'NONE',  ( 786.5483106153019435, -175.6454272087892718, -364.1601925771022366 ) ) ;
#478=CARTESIAN_POINT ( 'NONE',  ( 759.9864689768902508, -146.0891481129655176, -354.9819416627836404 ) ) ;
#479=CARTESIAN_POINT ( 'NONE',  ( 755.3201227861273992, -363.7255117493284615, -345.3687786644892981 ) ) ;
#481=CARTESIAN_POINT ( 'NONE',  ( 770.0799878456142551, 10.01258552831232329, -362.9823548866085616 ) ) ;
#484=CIRCLE ( 'NONE', #5652, 30.00000000000002842 ) ;
#489=CARTESIAN_POINT ( 'NONE',  ( 747.6481478633932056, -373.0999726633340856, -353.4146539503763620 ) ) ;
#491=CARTESIAN_POINT ( 'NONE',  ( 796.9462024416508257, 11.54721552339759860, -308.9653473494370246 ) ) ;
#495=CARTESIAN_POINT ( 'NONE',  ( 800.0135310231082713, -350.0891481129648923, -325.0180583372163028 ) ) ;
#498=CARTESIAN_POINT ( 'NONE',  ( 755.8894580844503253, -231.8272453906072315, -332.3691319403863531 ) ) ;
#502=CARTESIAN_POINT ( 'NONE',  ( 759.0252816721024374, -432.9982390220555999, -368.0189434323527280 ) ) ;
#507=CARTESIAN_POINT ( 'NONE',  ( 777.5031285880264704, -70.81642084023850714, -374.9108240113588408 ) ) ;
#508=CARTESIAN_POINT ( 'NONE',  ( 758.0580252608178853, -294.4527844766013800, -328.0187753319985404 ) ) ;
#512=CARTESIAN_POINT ( 'NONE',  ( 797.8822607201568644, -78.55451811788046257, -370.1134526219340160 ) ) ;
#513=CARTESIAN_POINT ( 'NONE',  ( 770.0799878456142551, -85.98741447168738716, -362.9823548866085616 ) ) ;
#517=CARTESIAN_POINT ( 'NONE',  ( 754.8072714833581358, -4.816420840238714085, -338.1981804954720587 ) ) ;
#519=CARTESIAN_POINT ( 'NONE',  ( 768.0187753319979720, -80.63460265842029173, -318.0580252608186242 ) ) ;
#522=CARTESIAN_POINT ( 'NONE',  ( 775.9200461376533440, -407.8055962898681628, -315.3028492785443291 ) ) ;
#525=CARTESIAN_POINT ( 'NONE',  ( 812.6845335610512393, -415.9874144716862361, -353.5525998758768651 ) ) ;
#532=CARTESIAN_POINT ( 'NONE',  ( 812.7932403749906598, -255.1800572038742700, -327.7687537140311633 ) ) ;
#536=CARTESIAN_POINT ( 'NONE',  ( 760.7433823573367135, -60.00906357242598688, -355.9930595647440441 ) ) ;
#538=CARTESIAN_POINT ( 'NONE',  ( 797.6776695296629214, -235.5436935675107293, -357.6776695296636603 ) ) ;
#540=CARTESIAN_POINT ( 'NONE',  ( 800.2193346964447755, -354.9982390220557704, -355.1360043628815788 ) ) ;
#541=CARTESIAN_POINT ( 'NONE',  ( 765.0180583372156207, -48.99823902205675807, -360.0135310231089534 ) ) ;
#546=CARTESIAN_POINT ( 'NONE',  ( 785.3687786644884454, -35.36187538569316047, -315.3201227861279676 ) ) ;
#550=CARTESIAN_POINT ( 'NONE',  ( 786.2694204179717872, -285.2817908451526137, -305.1769319972829067 ) ) ;
#554=CARTESIAN_POINT ( 'NONE',  ( 804.4286716492782716, -257.3618753856924286, -345.3141322388244703 ) ) ;
#556=CARTESIAN_POINT ( 'NONE',  ( 796.9571628226829034, -119.4636090269712554, -321.2382568024804641 ) ) ;
#558=FACE_BOUND ( 'NONE', #9290, .T. ) ;
#559=CARTESIAN_POINT ( 'NONE',  ( 796.7737145352015204, -308.6346026584195670, -370.7187646348536987 ) ) ;
#564=CARTESIAN_POINT ( 'NONE',  ( 808.7758568127978833, -196.1692326535052473, -320.0363995740631822 ) ) ;
#566=CARTESIAN_POINT ( 'NONE',  ( 808.3070685750230950, -450.9982390220554294, -361.1904061080339261 ) ) ;
#572=CARTESIAN_POINT ( 'NONE',  ( 763.2154366446407039, 2.376221891948710585, -321.4292242960311228 ) ) ;
#574=CARTESIAN_POINT ( 'NONE',  ( 799.9999999999993179, -512.9681489794448908, -370.0000000000000000 ) ) ;
#578=CARTESIAN_POINT ( 'NONE',  ( 779.4709603349208464, -288.3510508353231216, -314.7162404726379918 ) ) ;
#580=CARTESIAN_POINT ( 'NONE',  ( 815.0009284576459549, -294.3510508353230648, -338.7629533639073429 ) ) ;
#583=ORIENTED_EDGE ( 'NONE', *, *, #12485, .T. ) ;
#585=CARTESIAN_POINT ( 'NONE',  ( 758.6633372737375112, -68.53286901714197654, -326.9102291470432533 ) ) ;
#586=CARTESIAN_POINT ( 'NONE',  ( 803.4237431249931660, -159.1800572038746111, -331.2633955100225194 ) ) ;
#587=CARTESIAN_POINT ( 'NONE',  ( 781.7834795799800531, -202.8164208402380950, -315.0636971347436202 ) ) ;
#589=CARTESIAN_POINT ( 'NONE',  ( 815.2698199232961542, -136.8164208402382371, -342.5225473063383106 ) ) ;
#591=CARTESIAN_POINT ( 'NONE',  ( 771.1735550268780344, -153.1800572038746111, -316.3353852180828198 ) ) ;
#594=CARTESIAN_POINT ( 'NONE',  ( 804.6971507214547046, -387.2817908451522726, -344.0799538623459739 ) ) ;
#602=CARTESIAN_POINT ( 'NONE',  ( 805.2837595273609850, -386.7363362996977116, -340.5290396650784714 ) ) ;
#604=CARTESIAN_POINT ( 'NONE',  ( 749.5768839229115201, -180.5545181178801499, -358.0661480581553064 ) ) ;
#608=CARTESIAN_POINT ( 'NONE',  ( 802.7791456095903868, -340.7146871989592114, -329.0155153010375102 ) ) ;
#609=CARTESIAN_POINT ( 'NONE',  ( 754.8072714833581358, -436.8164208402372992, -338.1981804954720587 ) ) ;
#610=CARTESIAN_POINT ( 'NONE',  ( 802.2119215644370342, -174.0090635724256742, -367.5423716828165084 ) ) ;
#615=CARTESIAN_POINT ( 'NONE',  ( 813.1304606946831655, -209.9073299311471317, -352.3570229623691716 ) ) ;
#617=CARTESIAN_POINT ( 'NONE',  ( 804.9363028652555840, -16.27096629478413092, -338.2165204200192079 ) ) ;
#619=CARTESIAN_POINT ( 'NONE',  ( 744.8212110874229666, -90.89650538077827946, -336.2046728542121627 ) ) ;
#621=CARTESIAN_POINT ( 'NONE',  ( 792.2312462859673587, -323.9073299311468190, -307.2067596250082602 ) ) ;
#627=CARTESIAN_POINT ( 'NONE',  ( 815.1787889125755555, -414.8965053807771710, -343.7953271457877804 ) ) ;
#629=CARTESIAN_POINT ( 'NONE',  ( 800.9747183278959710, -420.9982390220555999, -311.9810565676471583 ) ) ;
#632=ORIENTED_EDGE ( 'NONE', *, *, #43023, .F. ) ;
#634=CARTESIAN_POINT ( 'NONE',  ( 746.0683387631852383, -187.4419599262325278, -331.3260364891676204 ) ) ;
#639=CARTESIAN_POINT ( 'NONE',  ( 815.2698199232961542, -40.81642084023859951, -342.5225473063383106 ) ) ;
#643=CARTESIAN_POINT ( 'NONE',  ( 745.7194118038753459, -445.6454272087883055, -348.7631598425976449 ) ) ;
#648=CARTESIAN_POINT ( 'NONE',  ( 791.9812246680005501, -284.6346026584196807, -361.9419747391813189 ) ) ;
#652=CARTESIAN_POINT ( 'NONE',  ( 796.9571628226829034, -287.4636090269708575, -321.2382568024804641 ) ) ;
#653=CARTESIAN_POINT ( 'NONE',  ( 788.7366044899766848, -299.9073299311468759, -316.5762568750059813 ) ) ;
#655=CARTESIAN_POINT ( 'NONE',  ( 803.6646147819161570, -113.9073299311474301, -348.8264449731210561 ) ) ;
#657=EDGE_LOOP ( 'NONE', ( #6082, #28881, #4838, #12896, #5628, #10326, #36542, #16472, #9881, #21547, #42805 ) ) ;
#662=CARTESIAN_POINT ( 'NONE',  ( 754.3581564841646241, -89.46360902697134065, -316.1443688327762516 ) ) ;
#669=CARTESIAN_POINT ( 'NONE',  ( 769.0155153010367712, -58.37269993606236085, -362.7791456095907279 ) ) ;
#670=CARTESIAN_POINT ( 'NONE',  ( 782.5225473063383106, -94.27096629478387513, -375.2698199232970637 ) ) ;
#672=CARTESIAN_POINT ( 'NONE',  ( 797.6776695296629214, -451.5436935675099903, -357.6776695296636603 ) ) ;
#674=CARTESIAN_POINT ( 'NONE',  ( 808.3070685750230950, -234.9982390220561683, -361.1904061080339261 ) ) ;
#679=CARTESIAN_POINT ( 'NONE',  ( 811.6461892240364477, -316.7146871989593819, -324.1737431748509835 ) ) ;
#681=CARTESIAN_POINT ( 'NONE',  ( 763.2262854647970016, -320.6346026584195670, -309.2812353651462445 ) ) ;
#685=CARTESIAN_POINT ( 'NONE',  ( 759.9864689768902508, -434.0891481129646081, -354.9819416627836404 ) ) ;
#687=CARTESIAN_POINT ( 'NONE',  ( 754.8072714833581358, -196.8164208402380950, -338.1981804954720587 ) ) ;
#688=CARTESIAN_POINT ( 'NONE',  ( 813.9316612368132837, -79.44195992623286884, -348.6739635108323228 ) ) ;
#692=CIRCLE ( 'NONE', #18407, 30.00000000000008171 ) ;
#695=CARTESIAN_POINT ( 'NONE',  ( 758.6633372737375112, -236.5328690171414792, -326.9102291470432533 ) ) ;
#697=CARTESIAN_POINT ( 'NONE',  ( 813.2346286133761168, -29.26014174441482751, -328.9521613784389160 ) ) ;
#699=CARTESIAN_POINT ( 'NONE',  ( 806.8957046614239061, -452.9681489794451181, -342.6393539086462852 ) ) ;
#703=CARTESIAN_POINT ( 'NONE',  ( 755.8990559732751535, -347.4636090269705733, -365.9055244015606831 ) ) ;
#706=CARTESIAN_POINT ( 'NONE',  ( 790.0220218866281812, -175.0999726633346825, -363.2186876482849129 ) ) ;
#707=CARTESIAN_POINT ( 'NONE',  ( 781.7834795799800531, -178.8164208402381519, -315.0636971347436202 ) ) ;
#708=CARTESIAN_POINT ( 'NONE',  ( 755.5713283507202505, -365.3618753856920875, -334.6858677611754729 ) ) ;
#719=CARTESIAN_POINT ( 'NONE',  ( 812.3518521366052028, -409.0999726633340288, -326.5853460496235243 ) ) ;
#720=CARTESIAN_POINT ( 'NONE',  ( 751.9810565676468741, -2.089148112965993231, -360.9747183278973921 ) ) ;
#723=CARTESIAN_POINT ( 'NONE',  ( 803.4237431249931660, -351.1800572038740142, -331.2633955100225194 ) ) ;
#727=CARTESIAN_POINT ( 'NONE',  ( 783.0745993439762742, -272.1908817542434917, -365.1016975059196739 ) ) ;
#732=CARTESIAN_POINT ( 'NONE',  ( 814.2001403089898304, -449.3618753856918602, -347.4397851343538264 ) ) ;
#737=CARTESIAN_POINT ( 'NONE',  ( 763.0537975583475827, -96.45278447660203369, -371.0346526505627480 ) ) ;
#738=CARTESIAN_POINT ( 'NONE',  ( 797.8594530101008786, -301.5436935675105588, -322.1405469898980982 ) ) ;
#742=CARTESIAN_POINT ( 'NONE',  ( 788.6739635108323228, -79.64542720878957027, -373.9316612368139090 ) ) ;
#743=CARTESIAN_POINT ( 'NONE',  ( 786.6156483768007774, -97.44195992623281199, -315.5913626894246136 ) ) ;
#747=CARTESIAN_POINT ( 'NONE',  ( 797.6776695296629214, 4.456306432488530866, -357.6776695296636603 ) ) ;
#748=CARTESIAN_POINT ( 'NONE',  ( 756.1348686366196716, -113.2601417444145682, -347.5531968255698416 ) ) ;
#750=CARTESIAN_POINT ( 'NONE',  ( 762.3223304703356007, -103.5436935675111272, -322.3223304703362828 ) ) ;
#751=CARTESIAN_POINT ( 'NONE',  ( 805.1016975059191054, -414.8965053807771710, -343.0745993439771837 ) ) ;
#754=DIRECTION ( 'NONE',  ( -1.000000000000000000, -0.000000000000000000, -0.000000000000000000 ) ) ;
#760=ORIENTED_EDGE ( 'NONE', *, *, #25320, .T. ) ;
#761=CARTESIAN_POINT ( 'NONE',  ( 793.0897708529556667, -78.55451811788046257, -361.3366627262616362 ) ) ;
#763=CARTESIAN_POINT ( 'NONE',  ( 804.9363028652555840, -232.2709662947834488, -338.2165204200192079 ) ) ;
#765=CARTESIAN_POINT ( 'NONE',  ( 797.8594530101008786, -397.5436935675100472, -322.1405469898980982 ) ) ;
#766=CARTESIAN_POINT ( 'NONE',  ( 774.6858677611749044, -33.72551174932952733, -315.5713283507209894 ) ) ;
#771=EDGE_CURVE ( 'NONE', #13016, #19801, #19550, .T. ) ;
#772=CARTESIAN_POINT ( 'NONE',  ( 755.0636971347428243, -4.270966294784170003, -341.7834795799807353 ) ) ;
#775=CARTESIAN_POINT ( 'NONE',  ( 809.0717654672305343, -292.9181544815162397, -360.1688906516309885 ) ) ;
#778=CARTESIAN_POINT ( 'NONE',  ( 754.8072714833581358, -268.8164208402378108, -338.1981804954720587 ) ) ;
#780=CARTESIAN_POINT ( 'NONE',  ( 793.0897708529556667, -126.5545181178803205, -361.3366627262616362 ) ) ;
#783=CARTESIAN_POINT ( 'NONE',  ( 745.7998596910086917, -341.3618753856922012, -332.5602148656461168 ) ) ;
#787=CARTESIAN_POINT ( 'NONE',  ( 795.6651683502461765, -202.7146871989597514, -371.3240766477733814 ) ) ;
#789=CARTESIAN_POINT ( 'NONE',  ( 815.1787889125755555, -438.8965053807771710, -343.7953271457877804 ) ) ;
#794=CARTESIAN_POINT ( 'NONE',  ( 780.5290396650775619, 11.64894916467595642, -365.2837595273619513 ) ) ;
#800=CARTESIAN_POINT ( 'NONE',  ( 786.6156483768007774, -289.4419599262321299, -315.5913626894246136 ) ) ;
#801=CARTESIAN_POINT ( 'NONE',  ( 751.2241431872005251, -280.1692326535049347, -359.9636004259367610 ) ) ;
#806=CARTESIAN_POINT ( 'NONE',  ( 805.0264073115434940, -78.35105083532376113, -339.4763451958999099 ) ) ;
#808=CARTESIAN_POINT ( 'NONE',  ( 804.7487373415286811, -163.5436935675109567, -364.7487373415288516 ) ) ;
#809=EDGE_LOOP ( 'NONE', ( #44423, #29622, #244, #36475, #38067, #15995 ) ) ;
#810=CARTESIAN_POINT ( 'NONE',  ( 755.5713283507202505, -149.3618753856928265, -334.6858677611754729 ) ) ;
#811=VERTEX_POINT ( 'NONE', #11356 ) ;
#812=CARTESIAN_POINT ( 'NONE',  ( 769.0155153010367712, -442.3726999360611103, -362.7791456095907279 ) ) ;
#813=( BOUNDED_CURVE ( )  B_SPLINE_CURVE ( 2, ( #30233, #2278, #8779, #33709, #16615, #44325, #30702 ),
 .UNSPECIFIED., .F., .T. ) 
 B_SPLINE_CURVE_WITH_KNOTS ( ( 3, 2, 2, 3 ),
 ( 0.006081874955971018626, 0.006818181818181817851, 0.009090909090909090468, 0.01033270150184909669 ),
 .UNSPECIFIED. ) 
 CURVE ( )  GEOMETRIC_REPRESENTATION_ITEM ( )  RATIONAL_B_SPLINE_CURVE ( ( 0.4977709609702910543, 0.4983514209501199721, 0.5000002209606653203, 0.4949109396520706694, 0.5000002209606653203, 0.4972194953619585855, 0.4974774836351868457 ) ) 
 REPRESENTATION_ITEM ( '' )  );
#818=DIRECTION ( 'NONE',  ( 0.000000000000000000, -1.000000000000000000, 0.000000000000000000 ) ) ;
#820=VERTEX_POINT ( 'NONE', #11128 ) ;
#821=CARTESIAN_POINT ( 'NONE',  ( 769.9779781133707957, -379.0999726633341993, -316.7813123517150871 ) ) ;
#823=CARTESIAN_POINT ( 'NONE',  ( 786.2694204179717872, -213.2817908451527842, -305.1769319972829067 ) ) ;
#828=CARTESIAN_POINT ( 'NONE',  ( 789.9200121543843807, -313.9874144716866908, -317.0176451133914384 ) ) ;
#830=CARTESIAN_POINT ( 'NONE',  ( 768.9521613784389729, -177.8272453906074304, -373.2346286133773106 ) ) ;
#834=CARTESIAN_POINT ( 'NONE',  ( 772.4837098697145166, -215.3618753856925707, -374.5518280994205611 ) ) ;
#836=CARTESIAN_POINT ( 'NONE',  ( 758.0580252608178853, -6.452784476602343666, -328.0187753319985404 ) ) ;
#838=CARTESIAN_POINT ( 'NONE',  ( 778.7502325331095108, -96.35105083532370429, -304.6391490659818828 ) ) ;
#840=CARTESIAN_POINT ( 'NONE',  ( 751.6929314249748586, -342.9982390220557136, -318.8095938919659034 ) ) ;
#845=CARTESIAN_POINT ( 'NONE',  ( 791.1614460488616487, -419.2601417444136587, -373.5763878283158874 ) ) ;
#846=CARTESIAN_POINT ( 'NONE',  ( 749.2812353651451076, -414.4527844766010389, -323.2262854647983090 ) ) ;
#850=CARTESIAN_POINT ( 'NONE',  ( 754.8983024940795303, -186.8965053807779668, -336.9254006560228163 ) ) ;
#852=CARTESIAN_POINT ( 'NONE',  ( 758.0141637701419768, -207.0783235625960685, -367.2620300519063790 ) ) ;
#859=CARTESIAN_POINT ( 'NONE',  ( 744.7301800767019131, -52.81642084023856398, -337.4774526936615757 ) ) ;
#860=CARTESIAN_POINT ( 'NONE',  ( 757.7880784355613741, -450.0090635724248500, -312.4576283171834916 ) ) ;
#862=CARTESIAN_POINT ( 'NONE',  ( 804.8461984189677878, -314.1908817542433781, -336.9566956441385628 ) ) ;
#869=CARTESIAN_POINT ( 'NONE',  ( 763.8424801807145741, -306.0090635724252479, -320.5453621957614700 ) ) ;
#870=CARTESIAN_POINT ( 'NONE',  ( 781.7834795799800531, -274.8164208402378108, -315.0636971347436202 ) ) ;
#872=CARTESIAN_POINT ( 'NONE',  ( 803.4237431249931660, -135.1800572038746679, -331.2633955100225194 ) ) ;
#878=CARTESIAN_POINT ( 'NONE',  ( 795.8262568251477660, -70.37269993606230400, -308.3538107759623585 ) ) ;
#885=CARTESIAN_POINT ( 'NONE',  ( 814.2001403089898304, -89.36187538569299704, -347.4397851343538264 ) ) ;
#889=CARTESIAN_POINT ( 'NONE',  ( 754.9967657858570647, -241.5436935675106156, -365.0032342141425374 ) ) ;
#892=CARTESIAN_POINT ( 'NONE',  ( 810.1134526219336749, -320.5328690171411949, -357.8822607201570349 ) ) ;
#894=CARTESIAN_POINT ( 'NONE',  ( 758.8095938919642549, -320.0891481129648355, -311.6929314249763365 ) ) ;
#898=CARTESIAN_POINT ( 'NONE',  ( 785.3141322388236176, -405.7255117493283478, -364.4286716492789537 ) ) ;
#899=CARTESIAN_POINT ( 'NONE',  ( 778.1981804954714335, -226.2709662947834204, -314.8072714833589885 ) ) ;
#900=CARTESIAN_POINT ( 'NONE',  ( 778.7502325331095108, -72.35105083532378956, -304.6391490659818828 ) ) ;
#905=CARTESIAN_POINT ( 'NONE',  ( 763.2154366446407039, -237.6237781080505442, -321.4292242960311228 ) ) ;
#907=CARTESIAN_POINT ( 'NONE',  ( 810.1134526219336749, -56.53286901714201917, -357.8822607201570349 ) ) ;
#911=VERTEX_POINT ( 'NONE', #25198 ) ;
#912=CARTESIAN_POINT ( 'NONE',  ( 750.9282345327678740, -328.9181544815160692, -319.8311093483690115 ) ) ;
#916=CARTESIAN_POINT ( 'NONE',  ( 804.4086373105744769, -193.6454272087891582, -333.3843516231986541 ) ) ;
#917=CARTESIAN_POINT ( 'NONE',  ( 762.1405469898971887, -169.5436935675108430, -357.8594530101015607 ) ) ;
#918=CARTESIAN_POINT ( 'NONE',  ( 778.1981804954715471, -394.2709662947829088, -314.8072714833591021 ) ) ;
#929=CARTESIAN_POINT ( 'NONE',  ( 749.5768839229115201, -396.5545181178794678, -358.0661480581553064 ) ) ;
#931=CARTESIAN_POINT ( 'NONE',  ( 787.5162901302840055, -11.36187538569323863, -305.4481719005793252 ) ) ;
#934=CARTESIAN_POINT ( 'NONE',  ( 800.0135310231082713, -374.0891481129647786, -325.0180583372163028 ) ) ;
#938=CARTESIAN_POINT ( 'NONE',  ( 793.0897708529556667, -246.5545181178799510, -361.3366627262616362 ) ) ;
#943=CARTESIAN_POINT ( 'NONE',  ( 772.4999999999993179, -512.9681489794448908, -339.9999999999999432 ) ) ;
#947=CARTESIAN_POINT ( 'NONE',  ( 800.2193346964447755, -306.9982390220558273, -355.1360043628815788 ) ) ;
#951=CARTESIAN_POINT ( 'NONE',  ( 768.9521613784389729, -57.82724539060780700, -373.2346286133773106 ) ) ;
#952=CARTESIAN_POINT ( 'NONE',  ( 780.5290396650775619, -108.3510508353236759, -365.2837595273619513 ) ) ;
#956=CARTESIAN_POINT ( 'NONE',  ( 768.0187753319979720, -8.634602658420517329, -318.0580252608186242 ) ) ;
#957=CARTESIAN_POINT ( 'NONE',  ( 798.7617431975189675, -147.6237781080508285, -323.0428371773161871 ) ) ;
#959=CARTESIAN_POINT ( 'NONE',  ( 804.9363028652555840, -112.2709662947838325, -338.2165204200192079 ) ) ;
#961=CARTESIAN_POINT ( 'NONE',  ( 765.8855110935204493, -406.1692326535045368, -319.0159684113471599 ) ) ;
#974=CARTESIAN_POINT ( 'NONE',  ( 759.0159684113467620, -88.91815448151682233, -325.8855110935213020 ) ) ;
#976=CARTESIAN_POINT ( 'NONE',  ( 774.6312213355098493, -239.3618753856924855, -364.6798772138717482 ) ) ;
#978=CARTESIAN_POINT ( 'NONE',  ( 756.3353852180819104, -389.9073299311465348, -331.1735550268788302 ) ) ;
#979=CARTESIAN_POINT ( 'NONE',  ( 759.9864689768902508, -50.08914811296584446, -354.9819416627836404 ) ) ;
#984=CARTESIAN_POINT ( 'NONE',  ( 754.8072714833581358, -28.81642084023863148, -338.1981804954720587 ) ) ;
#986=ORIENTED_EDGE ( 'NONE', *, *, #23842, .F. ) ;
#987=CARTESIAN_POINT ( 'NONE',  ( 764.1737431748507561, -298.3726999360616787, -371.6461892240376415 ) ) ;
#991=CARTESIAN_POINT ( 'NONE',  ( 774.6312213355099630, -263.3618753856924855, -364.6798772138717482 ) ) ;
#994=CARTESIAN_POINT ( 'NONE',  ( 802.5472867521000353, -148.3726999360620198, -350.8726784830461156 ) ) ;
#997=CARTESIAN_POINT ( 'NONE',  ( 759.8311093483677041, -22.16923265350575889, -310.9282345327691814 ) ) ;
#998=CARTESIAN_POINT ( 'NONE',  ( 754.9967657858570647, -361.5436935675103882, -365.0032342141425943 ) ) ;
#1003=CARTESIAN_POINT ( 'NONE',  ( 810.1134526219336749, -248.5328690171414223, -357.8822607201570349 ) ) ;
#1005=CARTESIAN_POINT ( 'NONE',  ( 804.7487373415286811, 4.456306432488530866, -364.7487373415288516 ) ) ;
#1011=CARTESIAN_POINT ( 'NONE',  ( 803.8651313633788504, 18.73985825558501972, -332.4468031744301015 ) ) ;
#1020=CARTESIAN_POINT ( 'NONE',  ( 783.0433043558608688, -288.8965053807775121, -315.1538015810313027 ) ) ;
#1023=CARTESIAN_POINT ( 'NONE',  ( 807.5423716828161105, -321.0783235625956991, -362.2119215644372048 ) ) ;
#1030=DIRECTION ( 'NONE',  ( 0.000000000000000000, 0.000000000000000000, 1.000000000000000000 ) ) ;
#1031=CARTESIAN_POINT ( 'NONE',  ( 749.2812353651451076, -198.4527844766017495, -323.2262854647983090 ) ) ;
#1034=CARTESIAN_POINT ( 'NONE',  ( 757.8323909638828582, -146.6346026584200786, -352.1044303154654358 ) ) ;
#1037=CARTESIAN_POINT ( 'NONE',  ( 757.4527132478984868, -424.3726999360612808, -329.1273215169538844 ) ) ;
#1043=CARTESIAN_POINT ( 'NONE',  ( 755.5913626894240451, -397.6454272087885329, -346.6156483768012890 ) ) ;
#1045=CARTESIAN_POINT ( 'NONE',  ( 815.3608509340175488, -218.7363362996982232, -341.2497674668889545 ) ) ;
#1050=CARTESIAN_POINT ( 'NONE',  ( 763.2154366446407039, -333.6237781080502600, -321.4292242960311228 ) ) ;
#1052=CARTESIAN_POINT ( 'NONE',  ( 771.3260364891663130, -187.6454272087892434, -306.0683387631859773 ) ) ;
#1056=VECTOR ( 'NONE', #20439, 1000.000000000000000 ) ;
#1057=CARTESIAN_POINT ( 'NONE',  ( 744.7301800767020268, -244.8164208402379245, -337.4774526936615189 ) ) ;
#1059=CARTESIAN_POINT ( 'NONE',  ( 778.2165204200184689, -22.81642084023865280, -364.9363028652563230 ) ) ;
#1061=CARTESIAN_POINT ( 'NONE',  ( 778.7502325331095108, -120.3510508353236048, -304.6391490659818828 ) ) ;
#1063=CARTESIAN_POINT ( 'NONE',  ( 777.5031285880264704, -358.8164208402375834, -374.9108240113588408 ) ) ;
#1070=CARTESIAN_POINT ( 'NONE',  ( 747.3154664389472828, -403.9874144716863498, -326.4474001241230781 ) ) ;
#1071=CARTESIAN_POINT ( 'NONE',  ( 810.7187646348534145, -450.4527844766009821, -356.7737145352016341 ) ) ;
#1075=CARTESIAN_POINT ( 'NONE',  ( 766.7756240680305382, -182.5328690171416497, -361.5560724626415663 ) ) ;
#1077=CARTESIAN_POINT ( 'NONE',  ( 759.8311093483677041, -238.1692326535050768, -310.9282345327691814 ) ) ;
#1082=CARTESIAN_POINT ( 'NONE',  ( 785.3687786644884454, -155.3618753856927128, -315.3201227861279676 ) ) ;
#1085=CARTESIAN_POINT ( 'NONE',  ( 772.5602148656447525, -57.72551174932945628, -305.7998596910095443 ) ) ;
#1087=CARTESIAN_POINT ( 'NONE',  ( 807.2620300519052989, -432.0090635724247932, -318.0141637701419768 ) ) ;
#1089=CARTESIAN_POINT ( 'NONE',  ( 805.2837595273609850, -314.7363362996979959, -340.5290396650784714 ) ) ;
#1093=CARTESIAN_POINT ( 'NONE',  ( 802.1676090361156639, -278.6346026584196807, -327.8955696845344505 ) ) ;
#1097=CARTESIAN_POINT ( 'NONE',  ( 769.0155153010367712, -274.3726999360617356, -362.7791456095907279 ) ) ;
#1098=CARTESIAN_POINT ( 'NONE',  ( 759.9864689768902508, -290.0891481129650629, -354.9819416627836404 ) ) ;
#1100=CARTESIAN_POINT ( 'NONE',  ( 797.8594530101008786, -157.5436935675108998, -322.1405469898980982 ) ) ;
#1106=CARTESIAN_POINT ( 'NONE',  ( 815.3608509340175488, -98.73633629969859271, -341.2497674668889545 ) ) ;
#1112=CARTESIAN_POINT ( 'NONE',  ( 763.2262854647970016, -128.6346026584201354, -309.2812353651462445 ) ) ;
#1117=CARTESIAN_POINT ( 'NONE',  ( 800.9747183278959710, -252.9982390220560831, -311.9810565676471583 ) ) ;
#1122=CARTESIAN_POINT ( 'NONE',  ( 815.0009284576459549, -318.3510508353230080, -338.7629533639073429 ) ) ;
#1124=CARTESIAN_POINT ( 'NONE',  ( 777.5031285880264704, -358.8164208402375834, -374.9108240113588408 ) ) ;
#1128=CARTESIAN_POINT ( 'NONE',  ( 758.0580252608178853, -414.4527844766010389, -328.0187753319985404 ) ) ;
#1130=CARTESIAN_POINT ( 'NONE',  ( 803.6646147819161570, -209.9073299311470748, -348.8264449731210561 ) ) ;
#1133=CARTESIAN_POINT ( 'NONE',  ( 808.7758568127978833, -100.1692326535055315, -320.0363995740631822 ) ) ;
#1139=CARTESIAN_POINT ( 'NONE',  ( 803.8651313633788504, -221.2601417444142271, -332.4468031744301015 ) ) ;
#1142=CARTESIAN_POINT ( 'NONE',  ( 749.8865473780648472, -68.53286901714197654, -322.1177392798429082 ) ) ;
#1144=CARTESIAN_POINT ( 'NONE',  ( 805.7454966640377734, -452.9681489794450044, -346.1170114844039745 ) ) ;
#1147=CARTESIAN_POINT ( 'NONE',  ( 804.1009440267234822, -359.4636090269705164, -314.0944755984392600 ) ) ;
#1152=CARTESIAN_POINT ( 'NONE',  ( 763.8424801807145741, -186.0090635724255890, -320.5453621957614700 ) ) ;
#1153=CARTESIAN_POINT ( 'NONE',  ( 759.7806653035534055, -174.9982390220563673, -324.8639956371180801 ) ) ;
#1154=CARTESIAN_POINT ( 'NONE',  ( 802.1676090361155502, -374.6346026584193396, -327.8955696845344505 ) ) ;
#1156=CARTESIAN_POINT ( 'NONE',  ( 765.8855110935204493, 25.83076734649409545, -319.0159684113471599 ) ) ;
#1161=DIRECTION ( 'NONE',  ( -0.000000000000000000, -1.110223024625155554E-15, -1.000000000000000000 ) ) ;
#1165=CARTESIAN_POINT ( 'NONE',  ( 749.5768839229115201, -420.5545181178793541, -358.0661480581553064 ) ) ;
#1166=CARTESIAN_POINT ( 'NONE',  ( 767.6429770376291799, -9.180057203875058747, -306.8695393053162093 ) ) ;
#1169=CARTESIAN_POINT ( 'NONE',  ( 771.1735550268778070, -393.1800572038737300, -316.3353852180827630 ) ) ;
#1170=CARTESIAN_POINT ( 'NONE',  ( 804.6798772138710092, 8.274488250670337663, -334.6312213355106451 ) ) ;
#1173=CARTESIAN_POINT ( 'NONE',  ( 787.5531968255692163, -261.8272453906071746, -316.1348686366205811 ) ) ;
#1183=CARTESIAN_POINT ( 'NONE',  ( 802.1676090361156639, -302.6346026584196238, -327.8955696845344505 ) ) ;
#1187=CARTESIAN_POINT ( 'NONE',  ( 814.4686193811664907, -51.28179084515328867, -346.2056067578752732 ) ) ;
#1188=CARTESIAN_POINT ( 'NONE',  ( 796.7845633553578182, -105.6237781080509421, -358.5707757039688204 ) ) ;
#1192=CARTESIAN_POINT ( 'NONE',  ( 801.9419747391806368, -18.45278447660230725, -351.9812246680014027 ) ) ;
#1193=CARTESIAN_POINT ( 'NONE',  ( 772.3691319403857278, -119.2601417444145397, -315.8894580844506663 ) ) ;
#1194=CARTESIAN_POINT ( 'NONE',  ( 788.7366044899766848, -131.9073299311473875, -316.5762568750059813 ) ) ;
#1195=CARTESIAN_POINT ( 'NONE',  ( 786.6156483768007774, -433.4419599262316183, -315.5913626894246136 ) ) ;
#1207=CARTESIAN_POINT ( 'NONE',  ( 784.1219089521767955, -93.28179084515315367, -315.0488828828318333 ) ) ;
#1209=CARTESIAN_POINT ( 'NONE',  ( 781.8018195045267476, -286.2709662947833067, -365.1927285166407273 ) ) ;
#1211=CARTESIAN_POINT ( 'NONE',  ( 765.0180583372156207, -384.9982390220556567, -360.0135310231089534 ) ) ;
#1212=CARTESIAN_POINT ( 'NONE',  ( 803.6646147819161570, -65.90732993114758642, -348.8264449731210561 ) ) ;
#1214=FACE_BOUND ( 'NONE', #39130, .T. ) ;
#1217=CARTESIAN_POINT ( 'NONE',  ( 813.5763878283155464, -27.82724539060790292, -351.1614460488615350 ) ) ;
#1220=CARTESIAN_POINT ( 'NONE',  ( 788.6739635108323228, -319.6454272087888739, -373.9316612368139090 ) ) ;
#1223=CARTESIAN_POINT ( 'NONE',  ( 788.8264449731200330, -261.1800572038741848, -363.6646147819171233 ) ) ;
#1225=CARTESIAN_POINT ( 'NONE',  ( 787.5531968255692163, -141.8272453906075157, -316.1348686366205811 ) ) ;
#1229=CARTESIAN_POINT ( 'NONE',  ( 815.0009284576459549, -6.351050835323991173, -338.7629533639073429 ) ) ;
#1230=CARTESIAN_POINT ( 'NONE',  ( 758.8095938919644823, -344.0891481129648355, -311.6929314249762797 ) ) ;
#1234=CARTESIAN_POINT ( 'NONE',  ( 754.0944755984390895, -231.6237781080504874, -364.1009440267246760 ) ) ;
#1237=CARTESIAN_POINT ( 'NONE',  ( 812.7932403749906598, 8.819942796124882634, -327.7687537140311633 ) ) ;
#1245=CARTESIAN_POINT ( 'NONE',  ( 763.2154366446407039, -21.62377810805121570, -321.4292242960311228 ) ) ;
#1253=CARTESIAN_POINT ( 'NONE',  ( 764.0069404352550464, -327.0783235625956991, -359.2566176426627180 ) ) ;
#1255=CARTESIAN_POINT ( 'NONE',  ( 803.8556311672234642, -321.6237781080502600, -365.6418435158340117 ) ) ;
#1262=CARTESIAN_POINT ( 'NONE',  ( 789.9200121543843807, -73.98741447168741558, -317.0176451133914384 ) ) ;
#1265=CARTESIAN_POINT ( 'NONE',  ( 787.4397851343537695, -189.7255117493290300, -374.2001403089903988 ) ) ;
#1268=CARTESIAN_POINT ( 'NONE',  ( 797.8594530101009923, -181.5436935675108430, -322.1405469898982119 ) ) ;
#1271=CARTESIAN_POINT ( 'NONE',  ( 805.2837595273609850, -434.7363362996975980, -340.5290396650784714 ) ) ;
#1276=DIRECTION ( 'NONE',  ( 1.000000000000000000, 0.000000000000000000, 0.000000000000000000 ) ) ;
#1278=CARTESIAN_POINT ( 'NONE',  ( 755.1538015810308480, -446.1908817542429802, -343.0433043558613804 ) ) ;
#1280=CARTESIAN_POINT ( 'NONE',  ( 813.5763878283155464, -219.8272453906073167, -351.1614460488615350 ) ) ;
#1285=CARTESIAN_POINT ( 'NONE',  ( 770.0799878456142551, -325.9874144716865771, -362.9823548866085616 ) ) ;
#1286=PLANE ( 'NONE',  #12170 ) ;
#1287=CARTESIAN_POINT ( 'NONE',  ( 764.1737431748507561, -202.3726999360618777, -371.6461892240376415 ) ) ;
#1292=CARTESIAN_POINT ( 'NONE',  ( 813.1304606946831655, -257.9073299311469327, -352.3570229623691716 ) ) ;
#1295=CARTESIAN_POINT ( 'NONE',  ( 767.8955696845333705, -24.45278447660229304, -362.1676090361162323 ) ) ;
#1297=CARTESIAN_POINT ( 'NONE',  ( 805.9055244015594326, -123.6237781080508569, -315.8990559732753240 ) ) ;
#1299=CARTESIAN_POINT ( 'NONE',  ( 772.4837098697144029, -383.3618753856921444, -374.5518280994205611 ) ) ;
#1300=EDGE_CURVE ( 'NONE', #38426, #11372, #5435, .T. ) ;
#1306=CARTESIAN_POINT ( 'NONE',  ( 801.9419747391806368, -378.4527844766011526, -351.9812246680014027 ) ) ;
#1307=CARTESIAN_POINT ( 'NONE',  ( 764.1737431748507561, -10.37269993606250473, -371.6461892240376415 ) ) ;
#1311=CARTESIAN_POINT ( 'NONE',  ( 803.2186876482843445, -175.9874144716871172, -350.0220218866286928 ) ) ;
#1313=CARTESIAN_POINT ( 'NONE',  ( 764.3348316497523456, -214.7146871989597230, -308.6759233522265617 ) ) ;
#1317=CARTESIAN_POINT ( 'NONE',  ( 778.2165204200184689, -142.8164208402382656, -364.9363028652563230 ) ) ;
#1319=CARTESIAN_POINT ( 'NONE',  ( 772.4837098697144029, -95.36187538569294020, -374.5518280994205611 ) ) ;
#1321=CARTESIAN_POINT ( 'NONE',  ( 773.4516893846965786, -19.64542720878974791, -315.8398074228977066 ) ) ;
#1323=CARTESIAN_POINT ( 'NONE',  ( 802.9823548866075953, -313.0999726633342561, -330.0799878456151077 ) ) ;
#1326=CARTESIAN_POINT ( 'NONE',  ( 774.6312213355099630, -311.3618753856922581, -364.6798772138717482 ) ) ;
#1330=CARTESIAN_POINT ( 'NONE',  ( 790.9844846989617508, -286.3726999360617356, -317.2208543904092721 ) ) ;
#1331=CARTESIAN_POINT ( 'NONE',  ( 794.9819416627830151, -300.9982390220559409, -319.9864689768909898 ) ) ;
#1333=CARTESIAN_POINT ( 'NONE',  ( 791.9812246680005501, -140.6346026584201070, -361.9419747391813189 ) ) ;
#1334=CARTESIAN_POINT ( 'NONE',  ( 779.9999999999992042, -462.9681489794448339, -339.9999999999999432 ) ) ;
#1336=CARTESIAN_POINT ( 'NONE',  ( 779.9999999999992042, -452.9681489794448339, -350.0000000000000000 ) ) ;
#1339=CARTESIAN_POINT ( 'NONE',  ( 781.2370466360911223, -68.73633629969867798, -304.9990715423533629 ) ) ;
#1346=CARTESIAN_POINT ( 'NONE',  ( 749.2812353651451076, -150.4527844766018916, -323.2262854647983090 ) ) ;
#1350=CARTESIAN_POINT ( 'NONE',  ( 798.7617431975189675, -435.6237781080499190, -323.0428371773161871 ) ) ;
#1352=CARTESIAN_POINT ( 'NONE',  ( 787.5162901302840055, -275.3618753856923149, -305.4481719005792684 ) ) ;
#1355=CARTESIAN_POINT ( 'NONE',  ( 805.9055244015594326, -339.6237781080502600, -315.8990559732753240 ) ) ;
#1357=CARTESIAN_POINT ( 'NONE',  ( 812.7932403749906598, -351.1800572038740142, -327.7687537140311633 ) ) ;
#1362=CARTESIAN_POINT ( 'NONE',  ( 759.7806653035534055, -414.9982390220555430, -324.8639956371180801 ) ) ;
#1363=CARTESIAN_POINT ( 'NONE',  ( 813.2346286133761168, -125.2601417444145255, -328.9521613784389160 ) ) ;
#1368=CARTESIAN_POINT ( 'NONE',  ( 793.2243759319678702, -242.5328690171414507, -318.4439275373583200 ) ) ;
#1370=CARTESIAN_POINT ( 'NONE',  ( 792.2269492836462632, -443.1233509495419298, -372.8191558162650949 ) ) ;
#1371=CARTESIAN_POINT ( 'NONE',  ( 748.3538107759620743, -64.71468719896019195, -355.8262568251490165 ) ) ;
#1375=CARTESIAN_POINT ( 'NONE',  ( 814.8207195650702488, -386.1908817542432075, -336.2433038121456548 ) ) ;
#1379=CARTESIAN_POINT ( 'NONE',  ( 800.9840315886518738, -172.9181544815165239, -354.1144889064786412 ) ) ;
#1380=CARTESIAN_POINT ( 'NONE',  ( 768.0187753319979720, -200.6346026584199365, -318.0580252608186242 ) ) ;
#1381=CARTESIAN_POINT ( 'NONE',  ( 771.1735550268780344, -393.1800572038737869, -316.3353852180828198 ) ) ;
#1391=CARTESIAN_POINT ( 'NONE',  ( 750.9282345327678740, -424.9181544815158986, -319.8311093483690115 ) ) ;
#1392=CARTESIAN_POINT ( 'NONE',  ( 745.4481719005789273, -27.72551174932954510, -347.5162901302853697 ) ) ;
#1394=CARTESIAN_POINT ( 'NONE',  ( 803.6646147819161570, -401.9073299311463643, -348.8264449731210561 ) ) ;
#1395=CARTESIAN_POINT ( 'NONE',  ( 755.3201227861273992, -3.725511749329622813, -345.3687786644892981 ) ) ;
#1398=CARTESIAN_POINT ( 'NONE',  ( 758.4439275373578084, -252.5545181178799226, -353.2243759319684386 ) ) ;
#1399=CARTESIAN_POINT ( 'NONE',  ( 777.4774526936600978, -154.2709662947836478, -304.7301800767027657 ) ) ;
#1402=CARTESIAN_POINT ( 'NONE',  ( 762.3223304703356007, 16.45630643248849267, -322.3223304703362828 ) ) ;
#1408=CARTESIAN_POINT ( 'NONE',  ( 754.8072714833581358, -316.8164208402377540, -338.1981804954720587 ) ) ;
#1410=CARTESIAN_POINT ( 'NONE',  ( 809.0717654672305343, -100.9181544815167513, -360.1688906516309885 ) ) ;
#1411=CARTESIAN_POINT ( 'NONE',  ( 789.9200121543843807, -121.9874144716872593, -317.0176451133914384 ) ) ;
#1414=CARTESIAN_POINT ( 'NONE',  ( 802.1676090361156639, -14.63460265842049424, -327.8955696845344505 ) ) ;
#1415=CARTESIAN_POINT ( 'NONE',  ( 784.0799538623451781, -131.8055962898690439, -364.6971507214555572 ) ) ;
#1416=CARTESIAN_POINT ( 'NONE',  ( 794.9819416627830151, -132.9982390220564810, -319.9864689768909898 ) ) ;
#1419=CARTESIAN_POINT ( 'NONE',  ( 768.8385539511368734, 24.73985825558500551, -306.4236121716840557 ) ) ;
#1430=CARTESIAN_POINT ( 'NONE',  ( 766.9102291470427417, -90.55451811788041994, -318.6633372737382501 ) ) ;
#1431=CARTESIAN_POINT ( 'NONE',  ( 771.2633955100217236, -287.9073299311468759, -363.4237431249939618 ) ) ;
#1434=CARTESIAN_POINT ( 'NONE',  ( 803.6646147819161570, -377.9073299311466485, -348.8264449731210561 ) ) ;
#1435=CARTESIAN_POINT ( 'NONE',  ( 764.8639956371174549, -32.08914811296588709, -319.7806653035542013 ) ) ;
#1439=CARTESIAN_POINT ( 'NONE',  ( 744.6391490659812007, -14.73633629969885384, -338.7502325331110455 ) ) ;
#1442=CARTESIAN_POINT ( 'NONE',  ( 745.7194118038753459, -301.6454272087889308, -348.7631598425976449 ) ) ;
#1445=CARTESIAN_POINT ( 'NONE',  ( 774.6312213355099630, -287.3618753856923718, -364.6798772138717482 ) ) ;
#1446=CARTESIAN_POINT ( 'NONE',  ( 755.8894580844503253, -135.8272453906076009, -332.3691319403863531 ) ) ;
#1449=CARTESIAN_POINT ( 'NONE',  ( 800.1688906516307043, -10.16923265350579442, -369.0717654672308186 ) ) ;
#1450=CARTESIAN_POINT ( 'NONE',  ( 796.9462024416508257, -348.4527844766012095, -308.9653473494370246 ) ) ;
#1454=CARTESIAN_POINT ( 'NONE',  ( 766.5853460496234675, -253.9874144716868329, -372.3518521366060554 ) ) ;
#1456=CARTESIAN_POINT ( 'NONE',  ( 813.9316612368132837, -439.4419599262316751, -348.6739635108323228 ) ) ;
#1461=CARTESIAN_POINT ( 'NONE',  ( 801.3366627262608972, -32.53286901714208312, -353.0897708529566899 ) ) ;
#1465=ORIENTED_EDGE ( 'NONE', *, *, #22138, .T. ) ;
#1466=CARTESIAN_POINT ( 'NONE',  ( 803.2186876482843445, -319.9874144716866340, -350.0220218866286928 ) ) ;
#1469=CARTESIAN_POINT ( 'NONE',  ( 754.0944755984390895, -327.6237781080502600, -364.1009440267246760 ) ) ;
#1476=CARTESIAN_POINT ( 'NONE',  ( 754.9967657858570647, -169.5436935675108430, -365.0032342141425374 ) ) ;
#1479=CARTESIAN_POINT ( 'NONE',  ( 785.3141322388236176, -189.7255117493290300, -364.4286716492789537 ) ) ;
#1481=CARTESIAN_POINT ( 'NONE',  ( 784.1219089521767955, -429.2817908451521021, -315.0488828828318333 ) ) ;
#1485=DIRECTION ( 'NONE',  ( 0.000000000000000000, -1.000000000000000000, 0.000000000000000000 ) ) ;
#1489=CARTESIAN_POINT ( 'NONE',  ( 775.8780910478218402, -441.2817908451521021, -364.9511171171680530 ) ) ;
#1491=CARTESIAN_POINT ( 'NONE',  ( 755.8990559732751535, -203.4636090269709996, -365.9055244015606831 ) ) ;
#1493=DIRECTION ( 'NONE',  ( 0.000000000000000000, 0.000000000000000000, -1.000000000000000000 ) ) ;
#1494=CARTESIAN_POINT ( 'NONE',  ( 759.7806653035534055, -174.9982390220563673, -324.8639956371180801 ) ) ;
#1495=CARTESIAN_POINT ( 'NONE',  ( 765.8855110935204493, -310.1692326535048778, -319.0159684113471599 ) ) ;
#1497=CARTESIAN_POINT ( 'NONE',  ( 812.3518521366052028, -217.0999726633345972, -326.5853460496235243 ) ) ;
#1500=CARTESIAN_POINT ( 'NONE',  ( 759.0159684113467620, -40.91815448151695023, -325.8855110935213020 ) ) ;
#1502=CARTESIAN_POINT ( 'NONE',  ( 808.3070685750232087, -234.9982390220561683, -361.1904061080339829 ) ) ;
#1505=CARTESIAN_POINT ( 'NONE',  ( 755.3201227861273992, -27.72551174932954510, -345.3687786644892981 ) ) ;
#1508=ADVANCED_FACE ( 'NONE', ( #20430, #38223 ), #24111, .T. ) ;
#1509=CARTESIAN_POINT ( 'NONE',  ( 808.7758568127978833, -148.1692326535053610, -320.0363995740631822 ) ) ;
#1511=CARTESIAN_POINT ( 'NONE',  ( 747.2067596250078623, -363.1800572038739006, -352.2312462859687230 ) ) ;
#1516=CARTESIAN_POINT ( 'NONE',  ( 803.6646147819161570, -377.9073299311466485, -348.8264449731210561 ) ) ;
#1518=CARTESIAN_POINT ( 'NONE',  ( 776.2046728542105711, 3.809118245755632959, -304.8212110874238761 ) ) ;
#1522=CARTESIAN_POINT ( 'NONE',  ( 786.6156483768007774, -217.4419599262324141, -315.5913626894246136 ) ) ;
#1524=CARTESIAN_POINT ( 'NONE',  ( 756.1443688327750579, -213.6237781080506011, -314.3581564841659315 ) ) ;
#1528=EDGE_CURVE ( 'NONE', #39743, #11556, #13743, .T. ) ;
#1531=CARTESIAN_POINT ( 'NONE',  ( 810.7187646348534145, -66.45278447660216159, -356.7737145352016341 ) ) ;
#1532=CARTESIAN_POINT ( 'NONE',  ( 778.1981804954715471, -82.27096629478390355, -314.8072714833591021 ) ) ;
#1534=CARTESIAN_POINT ( 'NONE',  ( 805.2837595273609850, -2.736336299698892027, -340.5290396650784714 ) ) ;
#1536=CARTESIAN_POINT ( 'NONE',  ( 772.4468031744293057, -321.8272453906070609, -363.8651313633793620 ) ) ;
#1545=CARTESIAN_POINT ( 'NONE',  ( 755.5913626894240451, -325.6454272087888739, -346.6156483768012890 ) ) ;
#1546=CARTESIAN_POINT ( 'NONE',  ( 762.1405469898971887, -313.5436935675102745, -357.8594530101015607 ) ) ;
#1547=CARTESIAN_POINT ( 'NONE',  ( 768.0187753319979720, -152.6346026584200786, -318.0580252608186242 ) ) ;
#1551=CARTESIAN_POINT ( 'NONE',  ( 793.5525998758768083, -103.0999726633349525, -372.6845335610516941 ) ) ;
#1557=CARTESIAN_POINT ( 'NONE',  ( 745.0891759886404770, -124.2709662947837899, -342.4968714119734159 ) ) ;
#1562=CARTESIAN_POINT ( 'NONE',  ( 814.9108240113580450, -256.2709662947834204, -337.5031285880265273 ) ) ;
#1563=CARTESIAN_POINT ( 'NONE',  ( 812.7932403749906598, -447.1800572038736732, -327.7687537140311633 ) ) ;
#1565=VECTOR ( 'NONE', #44163, 1000.000000000000000 ) ;
#1566=CARTESIAN_POINT ( 'NONE',  ( 761.9338519418445230, -326.5328690171411381, -370.4231160770881957 ) ) ;
#1567=CARTESIAN_POINT ( 'NONE',  ( 745.7998596910086917, -77.36187538569302546, -332.5602148656461168 ) ) ;
#1569=CARTESIAN_POINT ( 'NONE',  ( 804.7487373415286811, -355.5436935675103882, -364.7487373415288516 ) ) ;
#1574=CARTESIAN_POINT ( 'NONE',  ( 805.9055244015594326, -123.6237781080508569, -315.8990559732753240 ) ) ;
#1579=CARTESIAN_POINT ( 'NONE',  ( 790.8726784830453198, -250.7146871989595809, -362.5472867521010585 ) ) ;
#1582=CARTESIAN_POINT ( 'NONE',  ( 752.4576283171824116, -429.0783235625953580, -317.7880784355627952 ) ) ;
#1583=CARTESIAN_POINT ( 'NONE',  ( 801.9858362298568863, -75.07832356259649487, -312.7379699480935642 ) ) ;
#1585=VERTEX_POINT ( 'NONE', #4019 ) ;
#1587=CARTESIAN_POINT ( 'NONE',  ( 802.2119215644370342, -366.0090635724250774, -367.5423716828165084 ) ) ;
#1588=CARTESIAN_POINT ( 'NONE',  ( 774.6858677611749044, -225.7255117493289163, -315.5713283507209894 ) ) ;
#1592=CARTESIAN_POINT ( 'NONE',  ( 800.9840315886518738, -220.9181544815164102, -354.1144889064786412 ) ) ;
#1593=CARTESIAN_POINT ( 'NONE',  ( 791.9812246680005501, -188.6346026584199365, -361.9419747391813189 ) ) ;
#1595=CARTESIAN_POINT ( 'NONE',  ( 804.4286716492782716, -377.3618753856920875, -345.3141322388244703 ) ) ;
#1598=CARTESIAN_POINT ( 'NONE',  ( 788.8264449731200330, -117.1800572038746964, -363.6646147819171233 ) ) ;
#1604=LINE ( 'NONE', #25652, #280 ) ;
#1608=CARTESIAN_POINT ( 'NONE',  ( 802.2119215644370342, -462.0090635724247932, -367.5423716828165084 ) ) ;
#1609=CARTESIAN_POINT ( 'NONE',  ( 751.9810565676468741, -26.08914811296592262, -360.9747183278973921 ) ) ;
#1611=CARTESIAN_POINT ( 'NONE',  ( 758.0580252608178853, -414.4527844766010389, -328.0187753319985404 ) ) ;
#1612=CARTESIAN_POINT ( 'NONE',  ( 785.3141322388236176, -21.72551174932956641, -364.4286716492789537 ) ) ;
#1615=CARTESIAN_POINT ( 'NONE',  ( 804.1105419155481968, -267.8272453906071746, -347.6308680596136469 ) ) ;
#1616=CARTESIAN_POINT ( 'NONE',  ( 792.2312462859673587, -155.9073299311473306, -307.2067596250082602 ) ) ;
#1619=CARTESIAN_POINT ( 'NONE',  ( 768.1267186599862953, 16.45630643248851044, -317.8138973628999224 ) ) ;
#1621=DIRECTION ( 'NONE',  ( 0.9164815115825496461, 0.1263042864341401839, 0.3796167358741286413 ) ) ;
#1623=CARTESIAN_POINT ( 'NONE',  ( 764.8639956371174549, -320.0891481129648355, -319.7806653035542013 ) ) ;
#1625=CARTESIAN_POINT ( 'NONE',  ( 748.6759233522253680, -112.3726999360621761, -324.3348316497537098 ) ) ;
#1626=CARTESIAN_POINT ( 'NONE',  ( 799.4546378042377910, -129.0783235625963243, -356.1575198192848006 ) ) ;
#1629=CARTESIAN_POINT ( 'NONE',  ( 803.4237431249931660, -39.18005720387496638, -331.2633955100225194 ) ) ;
#1630=CARTESIAN_POINT ( 'NONE',  ( 793.2243759319678702, -146.5328690171417350, -318.4439275373583200 ) ) ;
#1631=CARTESIAN_POINT ( 'NONE',  ( 774.6858677611749044, -129.7255117493292289, -315.5713283507209894 ) ) ;
#1633=CARTESIAN_POINT ( 'NONE',  ( 790.8726784830453198, -442.7146871989589840, -362.5472867521010585 ) ) ;
#1639=CARTESIAN_POINT ( 'NONE',  ( 746.4236121716829757, -279.8272453906071746, -328.8385539511384650 ) ) ;
#1645=ORIENTED_EDGE ( 'NONE', *, *, #20048, .T. ) ;
#1646=CARTESIAN_POINT ( 'NONE',  ( 758.4439275373578084, -132.5545181178802920, -353.2243759319684386 ) ) ;
#1648=VERTEX_POINT ( 'NONE', #28962 ) ;
#1649=CARTESIAN_POINT ( 'NONE',  ( 803.6646147819161570, -401.9073299311463643, -348.8264449731210561 ) ) ;
#1650=CARTESIAN_POINT ( 'NONE',  ( 800.2193346964447755, -90.99823902205663728, -355.1360043628815788 ) ) ;
#1654=CARTESIAN_POINT ( 'NONE',  ( 814.2805881961230625, -1.645427208789804308, -331.2368401574024119 ) ) ;
#1657=CARTESIAN_POINT ( 'NONE',  ( 745.7194118038753459, -325.6454272087888739, -348.7631598425976449 ) ) ;
#1659=CARTESIAN_POINT ( 'NONE',  ( 779.9999999999992042, -462.9681489794448339, -339.9999999999999432 ) ) ;
#1660=CARTESIAN_POINT ( 'NONE',  ( 803.4237431249931660, -279.1800572038741848, -331.2633955100225194 ) ) ;
#1662=CARTESIAN_POINT ( 'NONE',  ( 769.0155153010367712, -154.3726999360620198, -362.7791456095907279 ) ) ;
#1665=CARTESIAN_POINT ( 'NONE',  ( 763.2262854647970016, -344.6346026584195101, -309.2812353651462445 ) ) ;
#1669=CARTESIAN_POINT ( 'NONE',  ( 783.7566961878529810, -432.8965053807771142, -305.1792804349288417 ) ) ;
#1675=CARTESIAN_POINT ( 'NONE',  ( 800.7704444035546203, -28.16923265350574468, -326.0291762391768771 ) ) ;
#1681=CARTESIAN_POINT ( 'NONE',  ( 756.7813123517142913, -331.9874144716865203, -329.9779781133712504 ) ) ;
#1684=CARTESIAN_POINT ( 'NONE',  ( 793.4146539503750546, -313.9874144716866908, -307.6481478633938877 ) ) ;
#1689=CARTESIAN_POINT ( 'NONE',  ( 777.5031285880264704, -166.8164208402382087, -374.9108240113588408 ) ) ;
#1692=CARTESIAN_POINT ( 'NONE',  ( 804.4286716492782716, -161.3618753856927697, -345.3141322388244703 ) ) ;
#1694=CARTESIAN_POINT ( 'NONE',  ( 760.7433823573367135, -420.0090635724249069, -355.9930595647440441 ) ) ;
#1701=CARTESIAN_POINT ( 'NONE',  ( 790.0220218866281812, -439.0999726633339719, -363.2186876482849129 ) ) ;
#1704=CARTESIAN_POINT ( 'NONE',  ( 802.2119215644370342, -198.0090635724255606, -367.5423716828165084 ) ) ;
#1708=CARTESIAN_POINT ( 'NONE',  ( 792.1044303154645831, -180.4527844766017211, -317.8323909638837677 ) ) ;
#1709=CARTESIAN_POINT ( 'NONE',  ( 754.9735926884551418, -378.3510508353227806, -340.5236548041000333 ) ) ;
#1711=CARTESIAN_POINT ( 'NONE',  ( 745.1792804349281596, -230.1908817542436338, -343.7566961878542884 ) ) ;
#1712=CARTESIAN_POINT ( 'NONE',  ( 799.9999999999993179, -462.9681489794448339, -362.3606797749978909 ) ) ;
#1714=CARTESIAN_POINT ( 'NONE',  ( 772.4468031744293057, -57.82724539060780700, -363.8651313633793620 ) ) ;
#1716=CARTESIAN_POINT ( 'NONE',  ( 796.9462024416508257, -252.4527844766015789, -308.9653473494370246 ) ) ;
#1720=CARTESIAN_POINT ( 'NONE',  ( 785.3687786644884454, -35.36187538569316047, -315.3201227861279676 ) ) ;
#1722=CARTESIAN_POINT ( 'NONE',  ( 754.0944755984390895, -135.6237781080508853, -364.1009440267246760 ) ) ;
#1724=CARTESIAN_POINT ( 'NONE',  ( 777.4774526936600978, -370.2709662947831362, -304.7301800767027657 ) ) ;
#1728=CARTESIAN_POINT ( 'NONE',  ( 805.1927285166397041, -376.8164208402375834, -341.8018195045277707 ) ) ;
#1731=CARTESIAN_POINT ( 'NONE',  ( 772.5602148656447525, -441.7255117493282910, -305.7998596910095443 ) ) ;
#1732=CARTESIAN_POINT ( 'NONE',  ( 772.4999999999993179, -512.9681489794448908, -339.9999999999999432 ) ) ;
#1736=CARTESIAN_POINT ( 'NONE',  ( 758.6633372737375112, -212.5328690171415076, -326.9102291470432533 ) ) ;
#1740=CARTESIAN_POINT ( 'NONE',  ( 754.0944755984390895, -231.6237781080504874, -364.1009440267246760 ) ) ;
#1741=CARTESIAN_POINT ( 'NONE',  ( 779.9999999999992042, 126.4563064324884465, -329.9999999999999432 ) ) ;
#1744=CARTESIAN_POINT ( 'NONE',  ( 757.8323909638827445, -146.6346026584200217, -352.1044303154654358 ) ) ;
#1746=CARTESIAN_POINT ( 'NONE',  ( 745.0891759886404770, -76.27096629478394618, -342.4968714119734159 ) ) ;
#1747=CARTESIAN_POINT ( 'NONE',  ( 764.8639956371174549, -56.08914811296581604, -319.7806653035542581 ) ) ;
#1749=CARTESIAN_POINT ( 'NONE',  ( 801.5560724626406000, -0.5545181178807169209, -326.7756240680316182 ) ) ;
#1750=CARTESIAN_POINT ( 'NONE',  ( 769.9779781133707957, -307.0999726633343130, -316.7813123517150871 ) ) ;
#1758=CARTESIAN_POINT ( 'NONE',  ( 801.5560724626406000, -336.5545181178796952, -326.7756240680316182 ) ) ;
#1759=CARTESIAN_POINT ( 'NONE',  ( 767.8955696845333705, -336.4527844766012095, -362.1676090361162323 ) ) ;
#1760=CARTESIAN_POINT ( 'NONE',  ( 759.9864689768902508, -146.0891481129655176, -354.9819416627836404 ) ) ;
#1764=CARTESIAN_POINT ( 'NONE',  ( 768.9521613784389729, -129.8272453906075725, -373.2346286133773106 ) ) ;
#1772=CARTESIAN_POINT ( 'NONE',  ( 759.0252816721024374, -144.9982390220564525, -368.0189434323527280 ) ) ;
#1775=CARTESIAN_POINT ( 'NONE',  ( 796.7737145352015204, -260.6346026584197375, -370.7187646348536987 ) ) ;
#1777=CARTESIAN_POINT ( 'NONE',  ( 793.3938497862117174, -453.0432664090020580, -372.3358127763067955 ) ) ;
#1780=CARTESIAN_POINT ( 'NONE',  ( 776.2433038121456548, -348.8965053807774552, -374.8207195650711014 ) ) ;
#1781=CARTESIAN_POINT ( 'NONE',  ( 787.5162901302840055, -83.36187538569296862, -305.4481719005792684 ) ) ;
#1784=CARTESIAN_POINT ( 'NONE',  ( 811.0346526505616112, -350.6346026584192828, -323.0537975583477532 ) ) ;
#1787=ORIENTED_EDGE ( 'NONE', *, *, #3181, .F. ) ;
#1791=CARTESIAN_POINT ( 'NONE',  ( 791.1614460488616487, -131.2601417444144829, -373.5763878283158874 ) ) ;
#1796=CARTESIAN_POINT ( 'NONE',  ( 779.4709603349208464, -0.3510508353240099355, -314.7162404726379918 ) ) ;
#1799=CARTESIAN_POINT ( 'NONE',  ( 781.2497674668890113, -420.3510508353225532, -375.3608509340180603 ) ) ;
#1805=CARTESIAN_POINT ( 'NONE',  ( 802.2119215644370342, -390.0090635724249069, -367.5423716828165084 ) ) ;
#1808=CARTESIAN_POINT ( 'NONE',  ( 804.4286716492782716, -233.3618753856925423, -345.3141322388244703 ) ) ;
#1811=CARTESIAN_POINT ( 'NONE',  ( 760.7433823573367135, -228.0090635724254753, -355.9930595647440441 ) ) ;
#1812=CARTESIAN_POINT ( 'NONE',  ( 767.8955696845333705, -216.4527844766016926, -362.1676090361162323 ) ) ;
#1815=CARTESIAN_POINT ( 'NONE',  ( 767.8955696845333705, -96.45278447660203369, -362.1676090361162323 ) ) ;
#1826=CARTESIAN_POINT ( 'NONE',  ( 807.2620300519052989, -456.0090635724247932, -318.0141637701419768 ) ) ;
#1827=CARTESIAN_POINT ( 'NONE',  ( 792.3570229623691148, -45.18005720387493795, -373.1304606946836770 ) ) ;
#1829=CARTESIAN_POINT ( 'NONE',  ( 778.1981804954714335, -394.2709662947827951, -314.8072714833589885 ) ) ;
#1830=CARTESIAN_POINT ( 'NONE',  ( 788.7366044899766848, -11.90732993114778182, -316.5762568750059813 ) ) ;
#1831=ADVANCED_FACE ( 'NONE', ( #32886 ), #35889, .F. ) ;
#1834=CARTESIAN_POINT ( 'NONE',  ( 755.5913626894240451, -277.6454272087889308, -346.6156483768012890 ) ) ;
#1835=CARTESIAN_POINT ( 'NONE',  ( 767.6429770376289525, -177.1800572038744690, -306.8695393053162093 ) ) ;
#1836=EDGE_CURVE ( 'NONE', #1585, #820, #32766, .T. ) ;
#1840=DIRECTION ( 'NONE',  ( 0.000000000000000000, -1.000000000000000000, 0.000000000000000000 ) ) ;
#1847=CARTESIAN_POINT ( 'NONE',  ( 804.6798772138708955, -351.7255117493284047, -334.6312213355107019 ) ) ;
#1850=CARTESIAN_POINT ( 'NONE',  ( 749.5768839229115201, -84.55451811788046257, -358.0661480581553064 ) ) ;
#1851=CARTESIAN_POINT ( 'NONE',  ( 760.5453621957607311, -117.0783235625963528, -323.8424801807151425 ) ) ;
#1855=CARTESIAN_POINT ( 'NONE',  ( 774.6858677611749044, -33.72551174932952733, -315.5713283507209894 ) ) ;
#1856=CARTESIAN_POINT ( 'NONE',  ( 802.7791456095903868, -124.7146871989599930, -329.0155153010375102 ) ) ;
#1857=CARTESIAN_POINT ( 'NONE',  ( 781.7834795799800531, -130.8164208402383224, -315.0636971347436202 ) ) ;
#1860=CARTESIAN_POINT ( 'NONE',  ( 760.5453621957607311, -429.0783235625953580, -323.8424801807151425 ) ) ;
#1866=CARTESIAN_POINT ( 'NONE',  ( 783.7953271457878373, -272.1908817542434917, -375.1787889125761239 ) ) ;
#1873=CARTESIAN_POINT ( 'NONE',  ( 761.4292242960306112, -113.4636090269712554, -323.2154366446414429 ) ) ;
#1874=CARTESIAN_POINT ( 'NONE',  ( 764.8639956371174549, -104.0891481129656881, -319.7806653035542013 ) ) ;
#1875=CARTESIAN_POINT ( 'NONE',  ( 800.2193346964446619, -282.9982390220559409, -355.1360043628816925 ) ) ;
#1877=CARTESIAN_POINT ( 'NONE',  ( 804.6798772138708955, -423.7255117493281205, -334.6312213355107019 ) ) ;
#1878=CARTESIAN_POINT ( 'NONE',  ( 788.8264449731200330, -69.18005720387488111, -363.6646147819171233 ) ) ;
#1880=DIRECTION ( 'NONE',  ( 0.000000000000000000, -1.000000000000000000, 0.000000000000000000 ) ) ;
#1881=AXIS2_PLACEMENT_3D ( 'NONE', #11229, #39189, #39876 ) ;
#1885=CARTESIAN_POINT ( 'NONE',  ( 809.0717654672305343, -340.9181544815160123, -360.1688906516309885 ) ) ;
#1889=CARTESIAN_POINT ( 'NONE',  ( 778.1981804954714335, -298.2709662947830793, -314.8072714833589885 ) ) ;
#1892=CARTESIAN_POINT ( 'NONE',  ( 776.9254006560222479, -140.1908817542438896, -314.8983024940802125 ) ) ;
#1896=CARTESIAN_POINT ( 'NONE',  ( 808.0189434323515343, -398.0891481129647218, -319.0252816721025511 ) ) ;
#1900=CARTESIAN_POINT ( 'NONE',  ( 814.5518280994195948, -15.72551174932958951, -332.4837098697145734 ) ) ;
#1906=CARTESIAN_POINT ( 'NONE',  ( 804.9511171171677688, -5.805596289869448867, -335.8780910478229202 ) ) ;
#1913=CARTESIAN_POINT ( 'NONE',  ( 805.1927285166397041, -40.81642084023859951, -341.8018195045277707 ) ) ;
#1915=CARTESIAN_POINT ( 'NONE',  ( 802.7791456095903868, -316.7146871989593819, -329.0155153010375102 ) ) ;
#1919=CARTESIAN_POINT ( 'NONE',  ( 771.2368401574024119, -325.4419599262320162, -374.2805881961240857 ) ) ;
#1927=CARTESIAN_POINT ( 'NONE',  ( 763.0537975583475827, -192.4527844766016926, -371.0346526505627480 ) ) ;
#1930=CARTESIAN_POINT ( 'NONE',  ( 767.8955696845334842, -168.4527844766018347, -362.1676090361161755 ) ) ;
#1932=CARTESIAN_POINT ( 'NONE',  ( 785.3687786644884454, 12.63812461430668321, -315.3201227861279676 ) ) ;
#1939=CARTESIAN_POINT ( 'NONE',  ( 787.5531968255692163, -429.8272453906067199, -316.1348686366205811 ) ) ;
#1942=CARTESIAN_POINT ( 'NONE',  ( 764.1737431748507561, -226.3726999360617924, -371.6461892240376415 ) ) ;
#1944=CIRCLE ( 'NONE', #7884, 10.00000000000000888 ) ;
#1946=CARTESIAN_POINT ( 'NONE',  ( 756.5762568750052424, -195.1800572038744974, -348.7366044899774238 ) ) ;
#1947=CARTESIAN_POINT ( 'NONE',  ( 802.7791456095903868, -364.7146871989592114, -329.0155153010375102 ) ) ;
#1949=CARTESIAN_POINT ( 'NONE',  ( 754.3581564841646241, -233.4636090269708575, -316.1443688327762516 ) ) ;
#1952=CARTESIAN_POINT ( 'NONE',  ( 786.5483106153019435, -55.64542720878963422, -364.1601925771022366 ) ) ;
#1956=CARTESIAN_POINT ( 'NONE',  ( 792.2312462859673587, -251.9073299311470748, -307.2067596250082602 ) ) ;
#1958=DIRECTION ( 'NONE',  ( 0.000000000000000000, -1.000000000000000000, 0.000000000000000000 ) ) ;
#1960=CARTESIAN_POINT ( 'NONE',  ( 778.1981804954714335, -58.27096629478398171, -314.8072714833589885 ) ) ;
#1963=CARTESIAN_POINT ( 'NONE',  ( 744.9990715423526808, -138.3510508353236048, -341.2370466360926002 ) ) ;
#1965=CARTESIAN_POINT ( 'NONE',  ( 754.9967657858570647, -385.5436935675102745, -365.0032342141425374 ) ) ;
#1970=CARTESIAN_POINT ( 'NONE',  ( 781.8018195045266339, -406.2709662947829088, -365.1927285166406705 ) ) ;
#1972=CARTESIAN_POINT ( 'NONE',  ( 793.3938497862117174, -453.0432664090020012, -372.3358127763067955 ) ) ;
#1976=CARTESIAN_POINT ( 'NONE',  ( 765.8855110935204493, -214.1692326535052189, -319.0159684113471599 ) ) ;
#1977=CARTESIAN_POINT ( 'NONE',  ( 759.7806653035534055, -126.9982390220565094, -324.8639956371180801 ) ) ;
#1979=CARTESIAN_POINT ( 'NONE',  ( 746.7653713866222915, -209.2601417444142839, -351.0478386215610271 ) ) ;
#1982=AXIS2_PLACEMENT_3D ( 'NONE', #35770, #7151, #28373 ) ;
#1984=CARTESIAN_POINT ( 'NONE',  ( 803.4237431249931660, -159.1800572038746111, -331.2633955100225194 ) ) ;
#1987=CARTESIAN_POINT ( 'NONE',  ( 808.0189434323515343, -86.08914811296573077, -319.0252816721025511 ) ) ;
#1988=CARTESIAN_POINT ( 'NONE',  ( 788.7366044899766848, -83.90732993114754379, -316.5762568750059813 ) ) ;
#1990=CARTESIAN_POINT ( 'NONE',  ( 793.9708237608222134, -22.91815448151701062, -319.2295555964448681 ) ) ;
#1993=CARTESIAN_POINT ( 'NONE',  ( 786.5483106153019435, -343.6454272087887603, -364.1601925771022366 ) ) ;
#2000=CARTESIAN_POINT ( 'NONE',  ( 796.9571628226829034, -335.4636090269705733, -321.2382568024804641 ) ) ;
#2001=CARTESIAN_POINT ( 'NONE',  ( 764.8639956371174549, -320.0891481129648355, -319.7806653035542013 ) ) ;
#2002=CARTESIAN_POINT ( 'NONE',  ( 774.6312213355099630, -143.3618753856927697, -364.6798772138717482 ) ) ;
#2005=LINE ( 'NONE', #36893, #4197 ) ;
#2006=CARTESIAN_POINT ( 'NONE',  ( 784.0799538623451781, -275.8055962898685038, -364.6971507214555572 ) ) ;
#2007=CARTESIAN_POINT ( 'NONE',  ( 752.7379699480933368, -108.0090635724258448, -361.9858362298580232 ) ) ;
#2014=CARTESIAN_POINT ( 'NONE',  ( 810.7187646348534145, -138.4527844766019200, -356.7737145352016341 ) ) ;
#2017=CARTESIAN_POINT ( 'NONE',  ( 815.2698199232961542, -256.8164208402379245, -342.5225473063383106 ) ) ;
#2022=CARTESIAN_POINT ( 'NONE',  ( 749.8865473780648472, -332.5328690171411381, -322.1177392798429082 ) ) ;
#2024=CARTESIAN_POINT ( 'NONE',  ( 744.7301800767019131, -100.8164208402383792, -337.4774526936615757 ) ) ;
#2026=CARTESIAN_POINT ( 'NONE',  ( 763.2262854647970016, -368.6346026584193964, -309.2812353651462445 ) ) ;
#2031=CARTESIAN_POINT ( 'NONE',  ( 766.5853460496234675, -109.9874144716873019, -372.3518521366060554 ) ) ;
#2036=VERTEX_POINT ( 'NONE', #19918 ) ;
#2037=CARTESIAN_POINT ( 'NONE',  ( 761.2382568024794409, -15.62377810805123524, -356.9571628226838129 ) ) ;
#2039=CARTESIAN_POINT ( 'NONE',  ( 744.9990715423526808, -426.3510508353226669, -341.2370466360926002 ) ) ;
#2043=CARTESIAN_POINT ( 'NONE',  ( 757.7880784355613741, -378.0090635724250774, -312.4576283171834916 ) ) ;
#2044=CARTESIAN_POINT ( 'NONE',  ( 805.1927285166397041, -232.8164208402379245, -341.8018195045277707 ) ) ;
#2049=CARTESIAN_POINT ( 'NONE',  ( 786.5483106153019435, -223.6454272087891013, -364.1601925771022366 ) ) ;
#2050=CARTESIAN_POINT ( 'NONE',  ( 781.7834795799800531, -226.8164208402380098, -315.0636971347436202 ) ) ;
#2051=CARTESIAN_POINT ( 'NONE',  ( 781.7834795799800531, -418.8164208402374129, -315.0636971347436202 ) ) ;
#2054=CARTESIAN_POINT ( 'NONE',  ( 788.8264449731200330, -93.18005720387481006, -363.6646147819171233 ) ) ;
#2065=CARTESIAN_POINT ( 'NONE',  ( 809.0717654672305343, -460.9181544815156713, -360.1688906516309885 ) ) ;
#2066=CARTESIAN_POINT ( 'NONE',  ( 763.0537975583476964, -24.45278447660228949, -371.0346526505628617 ) ) ;
#2068=CARTESIAN_POINT ( 'NONE',  ( 804.6798772138708955, -399.7255117493283478, -334.6312213355107019 ) ) ;
#2069=CARTESIAN_POINT ( 'NONE',  ( 795.1360043628808398, 3.910851887033986785, -360.2193346964456282 ) ) ;
#2072=CARTESIAN_POINT ( 'NONE',  ( 802.5472867521000353, -292.3726999360616219, -350.8726784830461156 ) ) ;
#2073=CARTESIAN_POINT ( 'NONE',  ( 746.8695393053150156, -149.9073299311473875, -327.6429770376306010 ) ) ;
#2076=CARTESIAN_POINT ( 'NONE',  ( 772.1467562141141343, 16.45630643248850689, -315.9110025235851253 ) ) ;
#2083=CARTESIAN_POINT ( 'NONE',  ( 756.3353852180819104, -365.9073299311465917, -331.1735550268788302 ) ) ;
#2086=CARTESIAN_POINT ( 'NONE',  ( 755.8990559732751535, -107.4636090269713122, -365.9055244015606831 ) ) ;
#2087=CARTESIAN_POINT ( 'NONE',  ( 763.2154366446407039, -165.6237781080507716, -321.4292242960311228 ) ) ;
#2092=CARTESIAN_POINT ( 'NONE',  ( 795.1360043628807261, -44.08914811296584446, -360.2193346964456282 ) ) ;
#2093=CARTESIAN_POINT ( 'NONE',  ( 801.3366627262608972, -176.5328690171416213, -353.0897708529566899 ) ) ;
#2094=CARTESIAN_POINT ( 'NONE',  ( 788.8264449731200330, -141.1800572038746395, -363.6646147819171233 ) ) ;
#2096=CARTESIAN_POINT ( 'NONE',  ( 804.1601925771018387, -439.4419599262316751, -346.5483106153029098 ) ) ;
#2101=CARTESIAN_POINT ( 'NONE',  ( 781.2370466360911223, -260.7363362996981095, -304.9990715423533629 ) ) ;
#2110=CARTESIAN_POINT ( 'NONE',  ( 804.8461984189677878, -122.1908817542439749, -336.9566956441385628 ) ) ;
#2111=CARTESIAN_POINT ( 'NONE',  ( 757.8323909638827445, -98.63460265842024910, -352.1044303154654358 ) ) ;
#2112=CARTESIAN_POINT ( 'NONE',  ( 800.0135310231082713, -278.0891481129651197, -325.0180583372163028 ) ) ;
#2114=CARTESIAN_POINT ( 'NONE',  ( 800.0135310231082713, -422.0891481129647218, -325.0180583372163028 ) ) ;
#2115=CARTESIAN_POINT ( 'NONE',  ( 759.7806653035534055, -78.99823902205662307, -324.8639956371180801 ) ) ;
#2123=CARTESIAN_POINT ( 'NONE',  ( 752.7379699480933368, -348.0090635724251342, -361.9858362298580232 ) ) ;
#2126=CARTESIAN_POINT ( 'NONE',  ( 785.3687786644884454, -299.3618753856922581, -315.3201227861279676 ) ) ;
#2128=CARTESIAN_POINT ( 'NONE',  ( 780.5236548040995785, -188.7363362996983085, -314.9735926884559944 ) ) ;
#2131=CARTESIAN_POINT ( 'NONE',  ( 751.6929314249750860, -366.9982390220557136, -318.8095938919659034 ) ) ;
#2136=CARTESIAN_POINT ( 'NONE',  ( 772.5602148656447525, -33.72551174932952733, -305.7998596910095443 ) ) ;
#2137=CARTESIAN_POINT ( 'NONE',  ( 768.0187753319979720, -248.6346026584197659, -318.0580252608186242 ) ) ;
#2138=DIRECTION ( 'NONE',  ( -1.000000000000000000, 0.000000000000000000, -0.000000000000000000 ) ) ;
#2141=CARTESIAN_POINT ( 'NONE',  ( 754.8983024940795303, -42.89650538077842157, -336.9254006560228163 ) ) ;
#2148=CARTESIAN_POINT ( 'NONE',  ( 793.2243759319678702, -338.5328690171411381, -318.4439275373583200 ) ) ;
#2151=CARTESIAN_POINT ( 'NONE',  ( 791.1614460488616487, -347.2601417444138860, -373.5763878283158874 ) ) ;
#2153=ORIENTED_EDGE ( 'NONE', *, *, #42791, .T. ) ;
#2158=CARTESIAN_POINT ( 'NONE',  ( 792.3570229623688874, -213.1800572038743553, -373.1304606946836202 ) ) ;
#2162=CARTESIAN_POINT ( 'NONE',  ( 802.1676090361155502, -182.6346026584199649, -327.8955696845344505 ) ) ;
#2164=CARTESIAN_POINT ( 'NONE',  ( 755.0636971347428243, -340.2709662947831362, -341.7834795799807353 ) ) ;
#2165=CARTESIAN_POINT ( 'NONE',  ( 774.6858677611749044, 14.27448825067031812, -315.5713283507209894 ) ) ;
#2170=CARTESIAN_POINT ( 'NONE',  ( 791.7608162188021197, 178.9475563372491251, -360.0000000000000000 ) ) ;
#2172=CARTESIAN_POINT ( 'NONE',  ( 804.4086373105744769, -433.6454272087884760, -333.3843516231986541 ) ) ;
#2176=CARTESIAN_POINT ( 'NONE',  ( 793.5525998758768083, -223.0999726633346256, -372.6845335610516941 ) ) ;
#2179=CARTESIAN_POINT ( 'NONE',  ( 768.0187753319979720, -200.6346026584199365, -318.0580252608186242 ) ) ;
#2180=CARTESIAN_POINT ( 'NONE',  ( 801.3366627262608972, -368.5328690171409676, -353.0897708529566899 ) ) ;
#2182=CARTESIAN_POINT ( 'NONE',  ( 746.4236121716829757, -207.8272453906073451, -328.8385539511384650 ) ) ;
#2185=CARTESIAN_POINT ( 'NONE',  ( 787.5531968255692163, -93.82724539060770041, -316.1348686366205811 ) ) ;
#2188=CARTESIAN_POINT ( 'NONE',  ( 764.0069404352550464, -423.0783235625953580, -359.2566176426627180 ) ) ;
#2189=CARTESIAN_POINT ( 'NONE',  ( 745.4481719005789273, -267.7255117493287457, -347.5162901302853697 ) ) ;
#2192=CARTESIAN_POINT ( 'NONE',  ( 804.6798772138708955, -39.72551174932951312, -334.6312213355107019 ) ) ;
#2194=CARTESIAN_POINT ( 'NONE',  ( 748.3538107759620743, -160.7146871989598651, -355.8262568251490165 ) ) ;
#2196=CARTESIAN_POINT ( 'NONE',  ( 767.6429770376289525, -393.1800572038737300, -306.8695393053162093 ) ) ;
#2200=CARTESIAN_POINT ( 'NONE',  ( 768.0187753319979720, -392.6346026584193396, -318.0580252608186242 ) ) ;
#2206=CARTESIAN_POINT ( 'NONE',  ( 801.3366627262608972, -224.5328690171415076, -353.0897708529566899 ) ) ;
#2207=CARTESIAN_POINT ( 'NONE',  ( 778.1981804954714335, -130.2709662947837899, -314.8072714833589885 ) ) ;
#2209=CARTESIAN_POINT ( 'NONE',  ( 798.0661480581538854, -242.5328690171414507, -309.5768839229118043 ) ) ;
#2213=CARTESIAN_POINT ( 'NONE',  ( 778.1981804954714335, -178.2709662947835625, -314.8072714833589885 ) ) ;
#2215=CARTESIAN_POINT ( 'NONE',  ( 792.3570229623688874, -93.18005720387481006, -373.1304606946836202 ) ) ;
#2216=CARTESIAN_POINT ( 'NONE',  ( 801.9419747391806368, -66.45278447660216159, -351.9812246680014027 ) ) ;
#2218=CARTESIAN_POINT ( 'NONE',  ( 798.5707757039680246, -5.463609026971610660, -356.7845633553585003 ) ) ;
#2220=CARTESIAN_POINT ( 'NONE',  ( 802.5472867521000353, -340.3726999360615082, -350.8726784830461156 ) ) ;
#2226=CARTESIAN_POINT ( 'NONE',  ( 793.9708237608222134, -310.9181544815160123, -319.2295555964448681 ) ) ;
#2227=CARTESIAN_POINT ( 'NONE',  ( 791.9812246680005501, -308.6346026584195670, -361.9419747391813189 ) ) ;
#2228=CARTESIAN_POINT ( 'NONE',  ( 811.3240766477731540, -148.3726999360620198, -355.6651683502462902 ) ) ;
#2232=CARTESIAN_POINT ( 'NONE',  ( 756.7813123517142913, -259.9874144716869182, -329.9779781133712504 ) ) ;
#2233=CARTESIAN_POINT ( 'NONE',  ( 745.1792804349281596, -110.1908817542440033, -343.7566961878542884 ) ) ;
#2240=CARTESIAN_POINT ( 'NONE',  ( 787.5162901302840055, -179.3618753856927128, -305.4481719005793252 ) ) ;
#2243=CARTESIAN_POINT ( 'NONE',  ( 744.7301800767019131, -316.8164208402377540, -337.4774526936615757 ) ) ;
#2249=CARTESIAN_POINT ( 'NONE',  ( 759.8311093483677041, -358.1692326535047641, -310.9282345327691814 ) ) ;
#2250=CARTESIAN_POINT ( 'NONE',  ( 814.5518280994195948, -87.72551174932937101, -332.4837098697145734 ) ) ;
#2252=CARTESIAN_POINT ( 'NONE',  ( 751.6929314249748586, -390.9982390220557136, -318.8095938919659034 ) ) ;
#2256=CARTESIAN_POINT ( 'NONE',  ( 768.8385539511368734, -119.2601417444145397, -306.4236121716840557 ) ) ;
#2262=CARTESIAN_POINT ( 'NONE',  ( 746.0683387631852383, -427.4419599262317888, -331.3260364891676204 ) ) ;
#2265=ORIENTED_EDGE ( 'NONE', *, *, #28091, .F. ) ;
#2266=CARTESIAN_POINT ( 'NONE',  ( 781.2370466360911223, -380.7363362996977116, -304.9990715423533629 ) ) ;
#2267=CARTESIAN_POINT ( 'NONE',  ( 755.0636971347428243, -244.2709662947834204, -341.7834795799807353 ) ) ;
#2270=CARTESIAN_POINT ( 'NONE',  ( 798.5707757039680246, -221.4636090269709428, -356.7845633553585003 ) ) ;
#2271=CARTESIAN_POINT ( 'NONE',  ( 759.7806653035534055, -222.9982390220561399, -324.8639956371180801 ) ) ;
#2272=CARTESIAN_POINT ( 'NONE',  ( 781.8018195045267476, -430.2709662947827383, -365.1927285166407273 ) ) ;
#2275=CARTESIAN_POINT ( 'NONE',  ( 765.0180583372156207, -96.99823902205660886, -360.0135310231089534 ) ) ;
#2276=ORIENTED_EDGE ( 'NONE', *, *, #36789, .T. ) ;
#2278=CARTESIAN_POINT ( 'NONE',  ( 781.3877698825695006, 18.31902617013176027, -309.9999999999999432 ) ) ;
#2284=CARTESIAN_POINT ( 'NONE',  ( 757.7880784355613741, -450.0090635724248500, -312.4576283171834916 ) ) ;
#2285=CARTESIAN_POINT ( 'NONE',  ( 814.2001403089898304, -41.36187538569314626, -347.4397851343538264 ) ) ;
#2287=CARTESIAN_POINT ( 'NONE',  ( 764.8639956371174549, -440.0891481129644944, -319.7806653035542013 ) ) ;
#2288=CARTESIAN_POINT ( 'NONE',  ( 756.5762568750052424, -51.18005720387493085, -348.7366044899774238 ) ) ;
#2292=CARTESIAN_POINT ( 'NONE',  ( 804.6971507214547046, -291.2817908451525000, -344.0799538623459739 ) ) ;
#2293=CARTESIAN_POINT ( 'NONE',  ( 772.5602148656447525, -177.7255117493290868, -305.7998596910095443 ) ) ;
#2296=DIRECTION ( 'NONE',  ( 0.000000000000000000, 0.000000000000000000, -1.000000000000000000 ) ) ;
#2297=CARTESIAN_POINT ( 'NONE',  ( 779.9999999999992042, -462.9681489794448339, -309.9999999999998863 ) ) ;
#2298=CARTESIAN_POINT ( 'NONE',  ( 808.7758568127978833, -244.1692326535050768, -320.0363995740631822 ) ) ;
#2303=CARTESIAN_POINT ( 'NONE',  ( 768.0187753319979720, -368.6346026584193964, -318.0580252608186242 ) ) ;
#2305=CARTESIAN_POINT ( 'NONE',  ( 757.7880784355613741, -90.00906357242590161, -312.4576283171834916 ) ) ;
#2306=CARTESIAN_POINT ( 'NONE',  ( 764.0069404352550464, -159.0783235625962391, -359.2566176426627180 ) ) ;
#2310=CARTESIAN_POINT ( 'NONE',  ( 755.3201227861273992, -51.72551174932946338, -345.3687786644892981 ) ) ;
#2311=CARTESIAN_POINT ( 'NONE',  ( 783.0433043558608688, -168.8965053807780237, -315.1538015810313027 ) ) ;
#2314=CARTESIAN_POINT ( 'NONE',  ( 786.2056067578752163, -11.80559628986942577, -374.4686193811670023 ) ) ;
#2320=CARTESIAN_POINT ( 'NONE',  ( 745.1792804349281596, -278.1908817542434917, -343.7566961878542884 ) ) ;
#2327=CARTESIAN_POINT ( 'NONE',  ( 757.4527132478984868, -112.3726999360621761, -329.1273215169538844 ) ) ;
#2328=CARTESIAN_POINT ( 'NONE',  ( 774.6858677611749044, -129.7255117493292289, -315.5713283507209894 ) ) ;
#2329=CARTESIAN_POINT ( 'NONE',  ( 803.4237431249931660, -327.1800572038741279, -331.2633955100225194 ) ) ;
#2331=CARTESIAN_POINT ( 'NONE',  ( 759.7806653035534055, -438.9982390220553157, -324.8639956371180801 ) ) ;
#2338=CARTESIAN_POINT ( 'NONE',  ( 764.1737431748507561, -346.3726999360614514, -371.6461892240376415 ) ) ;
#2340=CARTESIAN_POINT ( 'NONE',  ( 762.3223304703356007, -319.5436935675104451, -322.3223304703362828 ) ) ;
#2342=CARTESIAN_POINT ( 'NONE',  ( 802.9823548866075953, -193.0999726633346256, -330.0799878456151077 ) ) ;
#2346=CARTESIAN_POINT ( 'NONE',  ( 808.3070685750232087, -378.9982390220557136, -361.1904061080339829 ) ) ;
#2352=CARTESIAN_POINT ( 'NONE',  ( 796.9462024416508257, -36.45278447660223975, -308.9653473494370246 ) ) ;
#2353=CARTESIAN_POINT ( 'NONE',  ( 757.8323909638827445, -242.6346026584197659, -352.1044303154654358 ) ) ;
#2358=CARTESIAN_POINT ( 'NONE',  ( 773.3843516231979720, -61.44195992623291147, -364.4086373105754433 ) ) ;
#2368=CARTESIAN_POINT ( 'NONE',  ( 763.2154366446407039, -381.6237781080500326, -321.4292242960311228 ) ) ;
#2372=CARTESIAN_POINT ( 'NONE',  ( 800.1688906516307043, -370.1692326535045936, -369.0717654672308186 ) ) ;
#2377=CARTESIAN_POINT ( 'NONE',  ( 801.1904061080336987, -212.0891481129652902, -368.3070685750235498 ) ) ;
#2379=EDGE_LOOP ( 'NONE', ( #8972, #28124, #19949, #21029, #42065, #14516 ) ) ;
#2380=CARTESIAN_POINT ( 'NONE',  ( 781.7834795799800531, -202.8164208402380950, -315.0636971347436202 ) ) ;
#2382=ADVANCED_FACE ( 'NONE', ( #23813 ), #13228, .F. ) ;
#2383=CARTESIAN_POINT ( 'NONE',  ( 755.5713283507202505, -341.3618753856922012, -334.6858677611754729 ) ) ;
#2384=CARTESIAN_POINT ( 'NONE',  ( 762.3223304703356007, 16.45630643248849267, -322.3223304703362828 ) ) ;
#2392=CARTESIAN_POINT ( 'NONE',  ( 757.4527132478984868, -448.3726999360611103, -329.1273215169538844 ) ) ;
#2397=CARTESIAN_POINT ( 'NONE',  ( 810.4231160770870019, -240.5545181178798941, -321.9338519418446936 ) ) ;
#2400=CARTESIAN_POINT ( 'NONE',  ( 764.8639956371174549, -200.0891481129653187, -319.7806653035542013 ) ) ;
#2401=CARTESIAN_POINT ( 'NONE',  ( 759.2295555964440155, -376.1692326535046504, -353.9708237608231229 ) ) ;
#2402=CARTESIAN_POINT ( 'NONE',  ( 776.2046728542105711, -212.1908817542436623, -304.8212110874238761 ) ) ;
#2405=CARTESIAN_POINT ( 'NONE',  ( 761.4292242960306112, -65.46360902697142592, -323.2154366446414429 ) ) ;
#2409=CARTESIAN_POINT ( 'NONE',  ( 758.6633372737375112, -428.5328690171409107, -326.9102291470432533 ) ) ;
#2410=CARTESIAN_POINT ( 'NONE',  ( 801.1904061080338124, -260.0891481129650629, -368.3070685750236066 ) ) ;
#2414=CARTESIAN_POINT ( 'NONE',  ( 764.8639956371174549, -32.08914811296588709, -319.7806653035542013 ) ) ;
#2417=CARTESIAN_POINT ( 'NONE',  ( 791.1614460488616487, -179.2601417444143692, -373.5763878283158874 ) ) ;
#2419=CARTESIAN_POINT ( 'NONE',  ( 749.2812353651451076, -414.4527844766010389, -323.2262854647983090 ) ) ;
#2424=CARTESIAN_POINT ( 'NONE',  ( 756.5762568750052424, -411.1800572038738437, -348.7366044899774238 ) ) ;
#2425=FACE_OUTER_BOUND ( 'NONE', #15070, .T. ) ;
#2431=CARTESIAN_POINT ( 'NONE',  ( 775.9200461376533440, -239.8055962898687028, -315.3028492785443291 ) ) ;
#2433=CARTESIAN_POINT ( 'NONE',  ( 791.1614460488616487, -251.2601417444141134, -373.5763878283158874 ) ) ;
#2434=CARTESIAN_POINT ( 'NONE',  ( 799.9999999999993179, 205.0000000000000568, -319.9999999999999432 ) ) ;
#2439=CARTESIAN_POINT ( 'NONE',  ( 785.3141322388236176, -189.7255117493290300, -364.4286716492789537 ) ) ;
#2441=CARTESIAN_POINT ( 'NONE',  ( 763.2262854647970016, -128.6346026584201354, -309.2812353651462445 ) ) ;
#2443=CARTESIAN_POINT ( 'NONE',  ( 774.6312213355098493, -95.36187538569296862, -364.6798772138717482 ) ) ;
#2445=CARTESIAN_POINT ( 'NONE',  ( 772.4468031744293057, -33.82724539060788516, -363.8651313633793620 ) ) ;
#2447=CARTESIAN_POINT ( 'NONE',  ( 758.4439275373578084, -372.5545181178796383, -353.2243759319684386 ) ) ;
#2454=CARTESIAN_POINT ( 'NONE',  ( 775.8780910478218402, -369.2817908451523294, -364.9511171171680530 ) ) ;
#2455=CARTESIAN_POINT ( 'NONE',  ( 791.9812246680005501, -332.6346026584195101, -361.9419747391813189 ) ) ;
#2456=CARTESIAN_POINT ( 'NONE',  ( 797.8822607201568644, -150.5545181178802352, -370.1134526219340160 ) ) ;
#2461=CARTESIAN_POINT ( 'NONE',  ( 763.2154366446407039, -261.6237781080504305, -321.4292242960311228 ) ) ;
#2462=CARTESIAN_POINT ( 'NONE',  ( 791.0478386215596629, -117.8272453906076151, -306.7653713866226326 ) ) ;
#2468=CARTESIAN_POINT ( 'NONE',  ( 745.0891759886404770, -172.2709662947836478, -342.4968714119734159 ) ) ;
#2471=CARTESIAN_POINT ( 'NONE',  ( 745.0891759886404770, -316.2709662947832499, -342.4968714119734159 ) ) ;
#2478=CARTESIAN_POINT ( 'NONE',  ( 745.1769319972822814, -377.8055962898682765, -346.2694204179732083 ) ) ;
#2479=CARTESIAN_POINT ( 'NONE',  ( 814.5518280994195948, -111.7255117493293000, -332.4837098697145734 ) ) ;
#2481=CARTESIAN_POINT ( 'NONE',  ( 751.9810565676468741, -386.0891481129647786, -360.9747183278973921 ) ) ;
#2485=CARTESIAN_POINT ( 'NONE',  ( 778.7502325331095108, -144.3510508353235764, -304.6391490659818828 ) ) ;
#2491=CARTESIAN_POINT ( 'NONE',  ( 800.7704444035546203, -4.169232653505813069, -326.0291762391768771 ) ) ;
#2493=CARTESIAN_POINT ( 'NONE',  ( 814.2001403089898304, 6.638124614306706306, -347.4397851343538264 ) ) ;
#2497=CARTESIAN_POINT ( 'NONE',  ( 797.8594530101008786, -181.5436935675108145, -322.1405469898980982 ) ) ;
#2498=CARTESIAN_POINT ( 'NONE',  ( 745.1792804349281596, -422.1908817542430370, -343.7566961878542884 ) ) ;
#2501=CARTESIAN_POINT ( 'NONE',  ( 766.9102291470427417, -234.5545181178799794, -318.6633372737382501 ) ) ;
#2502=CARTESIAN_POINT ( 'NONE',  ( 755.3201227861273992, -219.7255117493289447, -345.3687786644892981 ) ) ;
#2504=CARTESIAN_POINT ( 'NONE',  ( 754.8072714833583632, -412.8164208402373561, -338.1981804954721156 ) ) ;
#2510=CARTESIAN_POINT ( 'NONE',  ( 802.2119215644370342, -6.009063572426154742, -367.5423716828165084 ) ) ;
#2516=CARTESIAN_POINT ( 'NONE',  ( 810.4231160770870019, -432.5545181178793541, -321.9338519418446936 ) ) ;
#2517=CARTESIAN_POINT ( 'NONE',  ( 767.7687537140311633, -71.90732993114760063, -372.7932403749916830 ) ) ;
#2519=CARTESIAN_POINT ( 'NONE',  ( 803.4237431249931660, -423.1800572038737300, -331.2633955100225194 ) ) ;
#2520=CARTESIAN_POINT ( 'NONE',  ( 803.6646147819162707, -41.90732993114767879, -348.8264449731211130 ) ) ;
#2524=CARTESIAN_POINT ( 'NONE',  ( 758.4439275373578084, -276.5545181178798657, -353.2243759319684386 ) ) ;
#2525=CARTESIAN_POINT ( 'NONE',  ( 810.7187646348534145, -210.4527844766016926, -356.7737145352016341 ) ) ;
#2531=CARTESIAN_POINT ( 'NONE',  ( 744.9990715423526808, -234.3510508353232638, -341.2370466360926002 ) ) ;
#2533=CARTESIAN_POINT ( 'NONE',  ( 814.5518280994195948, -279.7255117493288026, -332.4837098697145734 ) ) ;
#2537=CARTESIAN_POINT ( 'NONE',  ( 788.7366044899766848, -347.9073299311467053, -316.5762568750059813 ) ) ;
#2541=CARTESIAN_POINT ( 'NONE',  ( 788.7631598425961101, -49.44195992623295410, -305.7194118038759143 ) ) ;
#2542=CARTESIAN_POINT ( 'NONE',  ( 755.8398074228967971, -139.4419599262326699, -333.4516893846970333 ) ) ;
#2546=CARTESIAN_POINT ( 'NONE',  ( 795.1360043628807261, -68.08914811296575920, -360.2193346964456282 ) ) ;
#2547=CARTESIAN_POINT ( 'NONE',  ( 756.7813123517142913, -163.9874144716871456, -329.9779781133712504 ) ) ;
#2549=CARTESIAN_POINT ( 'NONE',  ( 791.1614460488616487, -11.26014174441488258, -373.5763878283158874 ) ) ;
#2554=CARTESIAN_POINT ( 'NONE',  ( 773.7305795820266212, -273.2817908451526137, -374.8230680027170365 ) ) ;
#2555=CIRCLE ( 'NONE', #20984, 30.00000000000008171 ) ;
#2562=CARTESIAN_POINT ( 'NONE',  ( 769.0155153010367712, -130.3726999360621619, -362.7791456095907279 ) ) ;
#2563=CARTESIAN_POINT ( 'NONE',  ( 774.6312213355099630, -119.3618753856928691, -364.6798772138717482 ) ) ;
#2564=CARTESIAN_POINT ( 'NONE',  ( 756.5762568750052424, -315.1800572038740711, -348.7366044899774238 ) ) ;
#2566=CARTESIAN_POINT ( 'NONE',  ( 785.3687786644884454, -443.3618753856917465, -315.3201227861279676 ) ) ;
#2574=CARTESIAN_POINT ( 'NONE',  ( 754.3581564841646241, -353.4636090269705733, -316.1443688327762516 ) ) ;
#2579=CARTESIAN_POINT ( 'NONE',  ( 756.3353852180819104, -317.9073299311468190, -331.1735550268788302 ) ) ;
#2581=CARTESIAN_POINT ( 'NONE',  ( 775.8780910478218402, -177.2817908451528695, -364.9511171171680530 ) ) ;
#2585=CARTESIAN_POINT ( 'NONE',  ( 805.0032342141413437, -373.5436935675102177, -314.9967657858572352 ) ) ;
#2592=CARTESIAN_POINT ( 'NONE',  ( 748.9653473494363425, -2.634602658420536869, -356.9462024416521331 ) ) ;
#2593=CARTESIAN_POINT ( 'NONE',  ( 794.9819416627830151, -252.9982390220560831, -319.9864689768909898 ) ) ;
#2598=CARTESIAN_POINT ( 'NONE',  ( 786.6156483768007774, -49.44195992623295410, -315.5913626894246136 ) ) ;
#2605=CARTESIAN_POINT ( 'NONE',  ( 762.3223304703356007, -55.54369356751127640, -322.3223304703362828 ) ) ;
#2606=CARTESIAN_POINT ( 'NONE',  ( 794.1144889064781864, -370.1692326535045936, -360.9840315886528401 ) ) ;
#2610=CARTESIAN_POINT ( 'NONE',  ( 758.0141637701419768, -375.0783235625955285, -367.2620300519063790 ) ) ;
#2617=CARTESIAN_POINT ( 'NONE',  ( 787.5162901302840055, -203.3618753856925991, -305.4481719005792684 ) ) ;
#2620=CARTESIAN_POINT ( 'NONE',  ( 756.5762568750052424, -219.1800572038744122, -348.7366044899774238 ) ) ;
#2622=CARTESIAN_POINT ( 'NONE',  ( 765.0180583372156207, -312.9982390220559409, -360.0135310231089534 ) ) ;
#2623=CARTESIAN_POINT ( 'NONE',  ( 804.4086373105744769, -457.6454272087884760, -333.3843516231986541 ) ) ;
#2633=CARTESIAN_POINT ( 'NONE',  ( 755.8894580844503253, -447.8272453906067199, -332.3691319403863531 ) ) ;
#2637=CARTESIAN_POINT ( 'NONE',  ( 745.7194118038753459, -229.6454272087890729, -348.7631598425976449 ) ) ;
#2640=CARTESIAN_POINT ( 'NONE',  ( 797.8594530101008786, -205.5436935675108430, -322.1405469898980982 ) ) ;
#2641=CARTESIAN_POINT ( 'NONE',  ( 757.2208543904082489, -376.7146871989592682, -350.9844846989624330 ) ) ;
#2642=CARTESIAN_POINT ( 'NONE',  ( 752.7379699480933368, -252.0090635724254184, -361.9858362298580232 ) ) ;
#2645=CARTESIAN_POINT ( 'NONE',  ( 796.9571628226829034, -71.46360902697141171, -321.2382568024804641 ) ) ;
#2649=CARTESIAN_POINT ( 'NONE',  ( 777.4774526936600978, -274.2709662947832499, -304.7301800767028226 ) ) ;
#2652=CARTESIAN_POINT ( 'NONE',  ( 804.9363028652555840, -40.27096629478405987, -338.2165204200192079 ) ) ;
#2655=CARTESIAN_POINT ( 'NONE',  ( 803.8556311672234642, -177.6237781080507148, -365.6418435158340117 ) ) ;
#2658=CARTESIAN_POINT ( 'NONE',  ( 811.0346526505616112, -422.6346026584192259, -323.0537975583477532 ) ) ;
#2663=CARTESIAN_POINT ( 'NONE',  ( 797.6776695296629214, -427.5436935675101040, -357.6776695296636603 ) ) ;
#2671=CARTESIAN_POINT ( 'NONE',  ( 799.4546378042377910, -249.0783235625959549, -356.1575198192848006 ) ) ;
#2672=CARTESIAN_POINT ( 'NONE',  ( 755.0636971347428243, -124.2709662947837899, -341.7834795799807353 ) ) ;
#2674=CARTESIAN_POINT ( 'NONE',  ( 815.1787889125755555, -246.8965053807777679, -343.7953271457877804 ) ) ;
#2680=CARTESIAN_POINT ( 'NONE',  ( 793.2243759319678702, -26.53286901714210799, -318.4439275373583200 ) ) ;
#2681=CARTESIAN_POINT ( 'NONE',  ( 756.5762568750052424, -171.1800572038745543, -348.7366044899774238 ) ) ;
#2683=CARTESIAN_POINT ( 'NONE',  ( 814.5518280994195948, -111.7255117493293000, -332.4837098697145734 ) ) ;
#2684=CARTESIAN_POINT ( 'NONE',  ( 797.6776695296629214, -115.5436935675110988, -357.6776695296636603 ) ) ;
#2686=CARTESIAN_POINT ( 'NONE',  ( 766.9102291470427417, -42.55451811788057626, -318.6633372737382501 ) ) ;
#2687=CARTESIAN_POINT ( 'NONE',  ( 775.8780910478218402, -345.2817908451523863, -364.9511171171680530 ) ) ;
#2696=CARTESIAN_POINT ( 'NONE',  ( 755.5913626894240451, -373.6454272087887034, -346.6156483768012890 ) ) ;
#2697=CARTESIAN_POINT ( 'NONE',  ( 755.3201227861273992, -339.7255117493285184, -345.3687786644892981 ) ) ;
#2698=CARTESIAN_POINT ( 'NONE',  ( 804.1009440267234822, -119.4636090269712554, -314.0944755984392600 ) ) ;
#2702=CARTESIAN_POINT ( 'NONE',  ( 770.0799878456142551, -253.9874144716868329, -362.9823548866085616 ) ) ;
#2703=CARTESIAN_POINT ( 'NONE',  ( 804.1009440267234822, -143.4636090269711701, -314.0944755984392600 ) ) ;
#2706=EDGE_CURVE ( 'NONE', #8202, #16020, #43813, .T. ) ;
#2712=CARTESIAN_POINT ( 'NONE',  ( 800.9747183278959710, -156.9982390220564241, -311.9810565676471583 ) ) ;
#2715=CARTESIAN_POINT ( 'NONE',  ( 811.0346526505616112, -302.6346026584196238, -323.0537975583477532 ) ) ;
#2717=CARTESIAN_POINT ( 'NONE',  ( 787.4999999999992042, -462.9681489794448339, -369.0473750965555837 ) ) ;
#2720=ORIENTED_EDGE ( 'NONE', *, *, #37012, .T. ) ;
#2722=CARTESIAN_POINT ( 'NONE',  ( 813.9316612368132837, -367.4419599262319025, -348.6739635108323228 ) ) ;
#2723=CARTESIAN_POINT ( 'NONE',  ( 808.0189434323515343, -110.0891481129656597, -319.0252816721025511 ) ) ;
#2725=CARTESIAN_POINT ( 'NONE',  ( 814.9108240113580450, -376.2709662947829656, -337.5031285880265273 ) ) ;
#2726=CARTESIAN_POINT ( 'NONE',  ( 787.4999999999992042, -512.9681489794448908, -309.9999999999998863 ) ) ;
#2732=CARTESIAN_POINT ( 'NONE',  ( 776.2433038121456548, -156.8965053807780805, -374.8207195650711014 ) ) ;
#2737=CARTESIAN_POINT ( 'NONE',  ( 794.1144889064781864, -10.16923265350579442, -360.9840315886528401 ) ) ;
#2739=CARTESIAN_POINT ( 'NONE',  ( 782.4968714119720516, -10.81642084023869543, -305.0891759886411023 ) ) ;
#2743=CARTESIAN_POINT ( 'NONE',  ( 815.3608509340175488, -410.7363362996976548, -341.2497674668889545 ) ) ;
#2745=CARTESIAN_POINT ( 'NONE',  ( 794.9819416627830151, -252.9982390220560831, -319.9864689768909898 ) ) ;
#2748=CARTESIAN_POINT ( 'NONE',  ( 790.0220218866281812, -271.0999726633344267, -363.2186876482849129 ) ) ;
#2749=CARTESIAN_POINT ( 'NONE',  ( 778.1981804954714335, -202.2709662947834772, -314.8072714833589885 ) ) ;
#2750=CARTESIAN_POINT ( 'NONE',  ( 771.2633955100217236, -431.9073299311464211, -363.4237431249939618 ) ) ;
#2756=CARTESIAN_POINT ( 'NONE',  ( 755.8990559732751535, -11.46360902697159290, -365.9055244015606831 ) ) ;
#2763=CARTESIAN_POINT ( 'NONE',  ( 790.9844846989617508, 1.627300063937458408, -317.2208543904092721 ) ) ;
#2764=CARTESIAN_POINT ( 'NONE',  ( 772.5602148656447525, -81.72551174932937101, -305.7998596910095443 ) ) ;
#2767=CARTESIAN_POINT ( 'NONE',  ( 771.2633955100217236, -431.9073299311464211, -363.4237431249939618 ) ) ;
#2768=CARTESIAN_POINT ( 'NONE',  ( 755.3201227861273992, -27.72551174932954510, -345.3687786644892981 ) ) ;
#2771=CARTESIAN_POINT ( 'NONE',  ( 801.1904061080336987, -188.0891481129653187, -368.3070685750235498 ) ) ;
#2776=CARTESIAN_POINT ( 'NONE',  ( 764.3348316497523456, -262.7146871989594956, -308.6759233522265617 ) ) ;
#2778=CARTESIAN_POINT ( 'NONE',  ( 749.2812353651451076, -270.4527844766014937, -323.2262854647983090 ) ) ;
#2782=CARTESIAN_POINT ( 'NONE',  ( 774.6858677611749044, -345.7255117493285184, -315.5713283507209894 ) ) ;
#2784=CARTESIAN_POINT ( 'NONE',  ( 786.2056067578752163, -59.80559628986927834, -374.4686193811670023 ) ) ;
#2785=CARTESIAN_POINT ( 'NONE',  ( 763.2154366446407039, -141.6237781080508569, -321.4292242960311228 ) ) ;
#2790=CARTESIAN_POINT ( 'NONE',  ( 755.5713283507202505, -77.36187538569302546, -334.6858677611754729 ) ) ;
#2791=CARTESIAN_POINT ( 'NONE',  ( 776.9566956441375396, -156.8965053807780805, -364.8461984189686405 ) ) ;
#2793=CARTESIAN_POINT ( 'NONE',  ( 800.1688906516307043, 13.83076734649413098, -369.0717654672308186 ) ) ;
#2799=CARTESIAN_POINT ( 'NONE',  ( 783.7953271457878373, -320.1908817542434349, -375.1787889125761239 ) ) ;
#2804=CARTESIAN_POINT ( 'NONE',  ( 784.1219089521767955, -141.2817908451530400, -315.0488828828318333 ) ) ;
#2805=CARTESIAN_POINT ( 'NONE',  ( 759.9864689768902508, -122.0891481129656171, -354.9819416627836404 ) ) ;
#2806=CARTESIAN_POINT ( 'NONE',  ( 754.8072714833583632, -316.8164208402377540, -338.1981804954721156 ) ) ;
#2807=ORIENTED_EDGE ( 'NONE', *, *, #14574, .T. ) ;
#2808=CARTESIAN_POINT ( 'NONE',  ( 774.6858677611749044, -417.7255117493283478, -315.5713283507209894 ) ) ;
#2815=CARTESIAN_POINT ( 'NONE',  ( 747.6481478633932056, -349.0999726633342561, -353.4146539503763620 ) ) ;
#2818=CARTESIAN_POINT ( 'NONE',  ( 755.5713283507202505, -317.3618753856922581, -334.6858677611754729 ) ) ;
#2820=CARTESIAN_POINT ( 'NONE',  ( 758.4439275373578084, -180.5545181178801499, -353.2243759319684386 ) ) ;
#2823=CARTESIAN_POINT ( 'NONE',  ( 744.7301800767020268, -364.8164208402375266, -337.4774526936615189 ) ) ;
#2828=CARTESIAN_POINT ( 'NONE',  ( 751.9810565676468741, -2.089148112965993231, -360.9747183278973921 ) ) ;
#2829=CARTESIAN_POINT ( 'NONE',  ( 755.0636971347428243, -244.2709662947834204, -341.7834795799807353 ) ) ;
#2833=CARTESIAN_POINT ( 'NONE',  ( 799.9636004259356241, -22.91815448151701062, -311.2241431872006956 ) ) ;
#2834=CARTESIAN_POINT ( 'NONE',  ( 770.0799878456142551, -37.98741447168752927, -362.9823548866085616 ) ) ;
#2840=EDGE_LOOP ( 'NONE', ( #30324, #23890, #9441, #26256, #17162 ) ) ;
#2841=CARTESIAN_POINT ( 'NONE',  ( 768.0187753319979720, -56.63460265842036279, -318.0580252608186242 ) ) ;
#2842=CARTESIAN_POINT ( 'NONE',  ( 780.5290396650775619, -372.3510508353228374, -365.2837595273619513 ) ) ;
#2845=CARTESIAN_POINT ( 'NONE',  ( 815.1787889125755555, -366.8965053807773984, -343.7953271457877804 ) ) ;
#2849=ORIENTED_EDGE ( 'NONE', *, *, #4352, .F. ) ;
#2851=CARTESIAN_POINT ( 'NONE',  ( 812.7932403749906598, -231.1800572038743553, -327.7687537140311633 ) ) ;
#2854=CARTESIAN_POINT ( 'NONE',  ( 758.0580252608178853, -198.4527844766017495, -328.0187753319985404 ) ) ;
#2857=CARTESIAN_POINT ( 'NONE',  ( 757.8323909638827445, -314.6346026584194533, -352.1044303154654358 ) ) ;
#2858=CARTESIAN_POINT ( 'NONE',  ( 755.8894580844503253, -447.8272453906067199, -332.3691319403863531 ) ) ;
#2861=CARTESIAN_POINT ( 'NONE',  ( 791.7608162188021197, 205.0000000000000568, -339.9999999999999432 ) ) ;
#2864=CARTESIAN_POINT ( 'NONE',  ( 754.7162404726377645, -446.7363362996975980, -339.4709603349214717 ) ) ;
#2865=LINE ( 'NONE', #23856, #12937 ) ;
#2868=CARTESIAN_POINT ( 'NONE',  ( 746.4236121716829757, -255.8272453906072315, -328.8385539511384650 ) ) ;
#2871=CARTESIAN_POINT ( 'NONE',  ( 791.9812246680005501, -212.6346026584198796, -361.9419747391813189 ) ) ;
#2872=CARTESIAN_POINT ( 'NONE',  ( 803.8651313633788504, -413.2601417444136018, -332.4468031744301015 ) ) ;
#2873=CARTESIAN_POINT ( 'NONE',  ( 813.5763878283155464, -243.8272453906072030, -351.1614460488615350 ) ) ;
#2876=CARTESIAN_POINT ( 'NONE',  ( 804.1105419155481968, -75.82724539060775726, -347.6308680596136469 ) ) ;
#2879=CARTESIAN_POINT ( 'NONE',  ( 786.6156483768007774, -433.4419599262316183, -315.5913626894246136 ) ) ;
#2880=CARTESIAN_POINT ( 'NONE',  ( 748.9653473494365699, -266.6346026584197375, -356.9462024416520762 ) ) ;
#2883=CARTESIAN_POINT ( 'NONE',  ( 804.9363028652555840, -88.27096629478390355, -338.2165204200192079 ) ) ;
#2885=CARTESIAN_POINT ( 'NONE',  ( 815.1787889125755555, -150.8965053807781089, -343.7953271457877804 ) ) ;
#2887=CARTESIAN_POINT ( 'NONE',  ( 777.5031285880264704, -406.8164208402375266, -374.9108240113588408 ) ) ;
#2891=CARTESIAN_POINT ( 'NONE',  ( 774.6858677611749044, -417.7255117493283478, -315.5713283507209894 ) ) ;
#2899=CARTESIAN_POINT ( 'NONE',  ( 761.2382568024794409, -255.6237781080504874, -356.9571628226838129 ) ) ;
#2901=CARTESIAN_POINT ( 'NONE',  ( 808.7758568127978833, -244.1692326535050768, -320.0363995740631822 ) ) ;
#2906=CARTESIAN_POINT ( 'NONE',  ( 794.1144889064781864, -58.16923265350564520, -360.9840315886528401 ) ) ;
#2907=CARTESIAN_POINT ( 'NONE',  ( 767.8955696845333705, -168.4527844766018347, -362.1676090361162323 ) ) ;
#2910=CARTESIAN_POINT ( 'NONE',  ( 801.1904061080336987, -116.0891481129656029, -368.3070685750235498 ) ) ;
#2911=CARTESIAN_POINT ( 'NONE',  ( 774.6312213355098493, -119.3618753856928834, -364.6798772138717482 ) ) ;
#2913=CARTESIAN_POINT ( 'NONE',  ( 757.4527132478984868, -40.37269993606240348, -329.1273215169538844 ) ) ;
#2914=CARTESIAN_POINT ( 'NONE',  ( 766.0291762391763086, -346.9181544815160123, -360.7704444035551319 ) ) ;
#2919=FACE_OUTER_BOUND ( 'NONE', #27553, .T. ) ;
#2922=CARTESIAN_POINT ( 'NONE',  ( 757.4527132478984868, -376.3726999360614514, -329.1273215169538844 ) ) ;
#2923=CARTESIAN_POINT ( 'NONE',  ( 771.1735550268778070, -345.1800572038739006, -316.3353852180827630 ) ) ;
#2924=CARTESIAN_POINT ( 'NONE',  ( 754.3581564841646241, -137.4636090269711985, -316.1443688327762516 ) ) ;
#2925=CIRCLE ( 'NONE', #21356, 20.00000000000001776 ) ;
#2929=CARTESIAN_POINT ( 'NONE',  ( 804.1601925771018387, -271.4419599262321867, -346.5483106153029098 ) ) ;
#2931=CARTESIAN_POINT ( 'NONE',  ( 778.7629533639073998, -152.7363362996983938, -375.0009284576466371 ) ) ;
#2936=CARTESIAN_POINT ( 'NONE',  ( 814.5518280994195948, -183.7255117493290300, -332.4837098697145166 ) ) ;
#2939=CARTESIAN_POINT ( 'NONE',  ( 814.5518280994195948, -303.7255117493287457, -332.4837098697145734 ) ) ;
#2945=CARTESIAN_POINT ( 'NONE',  ( 761.9338519418445230, -374.5328690171410813, -370.4231160770881957 ) ) ;
#2946=CARTESIAN_POINT ( 'NONE',  ( 763.2262854647970016, -128.6346026584201354, -309.2812353651462445 ) ) ;
#2949=CARTESIAN_POINT ( 'NONE',  ( 814.2001403089898304, -401.3618753856920307, -347.4397851343538264 ) ) ;
#2954=CARTESIAN_POINT ( 'NONE',  ( 752.4576283171824116, -141.0783235625962959, -317.7880784355627952 ) ) ;
#2961=CARTESIAN_POINT ( 'NONE',  ( 755.2512626584698410, -7.543693567511430942, -315.2512626584710915 ) ) ;
#2965=CARTESIAN_POINT ( 'NONE',  ( 804.9363028652555840, -184.2709662947835909, -338.2165204200192079 ) ) ;
#2966=CARTESIAN_POINT ( 'NONE',  ( 813.5763878283155464, -411.8272453906067199, -351.1614460488615350 ) ) ;
#2968=CARTESIAN_POINT ( 'NONE',  ( 804.9363028652555840, -256.2709662947834204, -338.2165204200192079 ) ) ;
#2971=CARTESIAN_POINT ( 'NONE',  ( 799.2566176426618085, -240.0090635724253900, -324.0069404352559559 ) ) ;
#2972=CARTESIAN_POINT ( 'NONE',  ( 757.8323909638827445, -242.6346026584197659, -352.1044303154654358 ) ) ;
#2973=CARTESIAN_POINT ( 'NONE',  ( 788.8264449731201466, -405.1800572038737869, -363.6646147819170665 ) ) ;
#2974=CARTESIAN_POINT ( 'NONE',  ( 781.7834795799800531, -82.81642084023846451, -315.0636971347436202 ) ) ;
#2975=EDGE_CURVE ( 'NONE', #24210, #43683, #44116, .T. ) ;
#2979=CARTESIAN_POINT ( 'NONE',  ( 772.4999999999993179, -512.9681489794448908, -339.9999999999999432 ) ) ;
#2981=CARTESIAN_POINT ( 'NONE',  ( 749.5768839229115201, -60.55451811788051941, -358.0661480581553064 ) ) ;
#2987=CARTESIAN_POINT ( 'NONE',  ( 755.3028492785439312, -15.28179084515340058, -335.9200461376539693 ) ) ;
#2988=CARTESIAN_POINT ( 'NONE',  ( 805.0032342141413437, -85.54369356751118403, -314.9967657858572352 ) ) ;
#2990=CARTESIAN_POINT ( 'NONE',  ( 804.6798772138708955, -447.7255117493280636, -334.6312213355107019 ) ) ;
#2991=CARTESIAN_POINT ( 'NONE',  ( 774.6858677611749044, -33.72551174932952733, -315.5713283507209894 ) ) ;
#2993=CARTESIAN_POINT ( 'NONE',  ( 763.0537975583475827, -192.4527844766016926, -371.0346526505627480 ) ) ;
#2998=CARTESIAN_POINT ( 'NONE',  ( 813.9316612368132837, -271.4419599262321867, -348.6739635108323228 ) ) ;
#3001=CARTESIAN_POINT ( 'NONE',  ( 745.0891759886404770, -292.2709662947831930, -342.4968714119734159 ) ) ;
#3002=DIRECTION ( 'NONE',  ( -1.000000000000000000, -0.000000000000000000, -0.000000000000000000 ) ) ;
#3005=CARTESIAN_POINT ( 'NONE',  ( 811.6461892240364477, -28.71468719896028077, -324.1737431748509835 ) ) ;
#3006=CARTESIAN_POINT ( 'NONE',  ( 755.5713283507202505, -389.3618753856919739, -334.6858677611754729 ) ) ;
#3009=CARTESIAN_POINT ( 'NONE',  ( 815.1787889125755555, -54.89650538077837183, -343.7953271457877804 ) ) ;
#3010=CARTESIAN_POINT ( 'NONE',  ( 804.1601925771018387, -151.4419599262326415, -346.5483106153029098 ) ) ;
#3015=CARTESIAN_POINT ( 'NONE',  ( 758.0580252608178853, -54.45278447660219001, -328.0187753319985404 ) ) ;
#3016=CARTESIAN_POINT ( 'NONE',  ( 776.9566956441375396, -180.8965053807779952, -364.8461984189686405 ) ) ;
#3019=CARTESIAN_POINT ( 'NONE',  ( 807.5423716828161105, 14.92167643740321381, -362.2119215644372048 ) ) ;
#3024=CARTESIAN_POINT ( 'NONE',  ( 773.7305795820266212, -297.2817908451526137, -374.8230680027170365 ) ) ;
#3028=CARTESIAN_POINT ( 'NONE',  ( 755.8894580844503253, -135.8272453906076009, -332.3691319403863531 ) ) ;
#3029=CARTESIAN_POINT ( 'NONE',  ( 788.8264449731200330, -165.1800572038745258, -363.6646147819171233 ) ) ;
#3036=CARTESIAN_POINT ( 'NONE',  ( 802.2119215644370342, -390.0090635724249069, -367.5423716828165084 ) ) ;
#3040=CARTESIAN_POINT ( 'NONE',  ( 758.0580252608178853, -342.4527844766013231, -328.0187753319985404 ) ) ;
#3041=DIRECTION ( 'NONE',  ( 0.000000000000000000, -1.000000000000000000, 0.000000000000000000 ) ) ;
#3042=CARTESIAN_POINT ( 'NONE',  ( 800.9840315886518738, -220.9181544815164102, -354.1144889064786412 ) ) ;
#3045=CARTESIAN_POINT ( 'NONE',  ( 808.3070685750232087, -402.9982390220555999, -361.1904061080339829 ) ) ;
#3050=CARTESIAN_POINT ( 'NONE',  ( 749.2812353651451076, -54.45278447660219001, -323.2262854647983090 ) ) ;
#3051=CARTESIAN_POINT ( 'NONE',  ( 797.6776695296629214, -259.5436935675106156, -357.6776695296636603 ) ) ;
#3056=CARTESIAN_POINT ( 'NONE',  ( 746.4236121716829757, -39.82724539060786384, -328.8385539511384650 ) ) ;
#3057=CARTESIAN_POINT ( 'NONE',  ( 770.0799878456142551, -61.98741447168745822, -362.9823548866085616 ) ) ;
#3061=CARTESIAN_POINT ( 'NONE',  ( 799.9999999999993179, -512.9681489794448908, -309.9999999999998863 ) ) ;
#3063=CARTESIAN_POINT ( 'NONE',  ( 792.1044303154645831, -60.45278447660215448, -317.8323909638837677 ) ) ;
#3064=CARTESIAN_POINT ( 'NONE',  ( 758.6633372737375112, -380.5328690171409676, -326.9102291470432533 ) ) ;
#3067=CARTESIAN_POINT ( 'NONE',  ( 813.9316612368132837, -367.4419599262319025, -348.6739635108323228 ) ) ;
#3072=CARTESIAN_POINT ( 'NONE',  ( 814.2001403089898304, -209.3618753856926276, -347.4397851343538264 ) ) ;
#3076=CARTESIAN_POINT ( 'NONE',  ( 778.1981804954715471, -202.2709662947835341, -314.8072714833591021 ) ) ;
#3078=CARTESIAN_POINT ( 'NONE',  ( 803.4237431249931660, -375.1800572038739574, -331.2633955100225194 ) ) ;
#3079=CARTESIAN_POINT ( 'NONE',  ( 778.1981804954714335, -10.27096629478414691, -314.8072714833589885 ) ) ;
#3083=EDGE_LOOP ( 'NONE', ( #15792, #4178, #15921, #13120 ) ) ;
#3084=CARTESIAN_POINT ( 'NONE',  ( 791.9812246680005501, 3.365397341579444479, -361.9419747391813189 ) ) ;
#3088=CARTESIAN_POINT ( 'NONE',  ( 745.5313806188320314, -279.2817908451526137, -333.7943932421247268 ) ) ;
#3092=CARTESIAN_POINT ( 'NONE',  ( 800.2193346964447755, -210.9982390220561967, -355.1360043628815788 ) ) ;
#3093=CARTESIAN_POINT ( 'NONE',  ( 783.0433043558608688, -408.8965053807772847, -315.1538015810313027 ) ) ;
#3096=CARTESIAN_POINT ( 'NONE',  ( 799.2566176426618085, -96.00906357242585898, -324.0069404352559559 ) ) ;
#3098=CARTESIAN_POINT ( 'NONE',  ( 781.2497674668890113, 11.64894916467595642, -375.3608509340180603 ) ) ;
#3099=CARTESIAN_POINT ( 'NONE',  ( 746.8695393053151292, -293.9073299311468759, -327.6429770376306578 ) ) ;
#3102=CARTESIAN_POINT ( 'NONE',  ( 788.8264449731200330, -93.18005720387481006, -363.6646147819171233 ) ) ;
#3104=CARTESIAN_POINT ( 'NONE',  ( 754.0944755984390895, -183.6237781080507148, -364.1009440267246760 ) ) ;
#3106=CARTESIAN_POINT ( 'NONE',  ( 800.9747183278959710, -420.9982390220555999, -311.9810565676471583 ) ) ;
#3109=ADVANCED_FACE ( 'NONE', ( #13398 ), #38115, .F. ) ;
#3111=CARTESIAN_POINT ( 'NONE',  ( 758.0580252608178853, -414.4527844766010389, -328.0187753319985404 ) ) ;
#3112=CARTESIAN_POINT ( 'NONE',  ( 791.7608162188021197, 240.0000000000000853, -360.0000000000000000 ) ) ;
#3117=CARTESIAN_POINT ( 'NONE',  ( 764.0069404352550464, -255.0783235625958980, -359.2566176426627180 ) ) ;
#3120=CARTESIAN_POINT ( 'NONE',  ( 813.9316612368132837, -247.4419599262323004, -348.6739635108323228 ) ) ;
#3125=CARTESIAN_POINT ( 'NONE',  ( 783.0433043558608688, -48.89650538077840025, -315.1538015810313027 ) ) ;
#3126=CARTESIAN_POINT ( 'NONE',  ( 771.1735550268778070, -153.1800572038746395, -316.3353852180827630 ) ) ;
#3127=CARTESIAN_POINT ( 'NONE',  ( 765.0180583372156207, -216.9982390220562252, -360.0135310231089534 ) ) ;
#3129=CARTESIAN_POINT ( 'NONE',  ( 772.5602148656447525, -105.7255117493293000, -305.7998596910095443 ) ) ;
#3131=CARTESIAN_POINT ( 'NONE',  ( 767.8955696845334842, -120.4527844766019768, -362.1676090361161755 ) ) ;
#3133=CARTESIAN_POINT ( 'NONE',  ( 755.8894580844503253, -39.82724539060786384, -332.3691319403863531 ) ) ;
#3134=CARTESIAN_POINT ( 'NONE',  ( 755.3028492785439312, -399.2817908451522726, -335.9200461376539693 ) ) ;
#3141=CARTESIAN_POINT ( 'NONE',  ( 802.9823548866075953, -361.0999726633341425, -330.0799878456151077 ) ) ;
#3142=CARTESIAN_POINT ( 'NONE',  ( 754.8072714833581358, -340.8164208402376971, -338.1981804954720587 ) ) ;
#3144=CARTESIAN_POINT ( 'NONE',  ( 813.5763878283155464, -123.8272453906076009, -351.1614460488615350 ) ) ;
#3148=CARTESIAN_POINT ( 'NONE',  ( 761.2382568024794409, -279.6237781080503737, -356.9571628226838129 ) ) ;
#3149=CARTESIAN_POINT ( 'NONE',  ( 804.9363028652555840, -448.2709662947827951, -338.2165204200192079 ) ) ;
#3150=CARTESIAN_POINT ( 'NONE',  ( 773.7305795820266212, -153.2817908451529831, -374.8230680027170365 ) ) ;
#3151=PLANE ( 'NONE',  #34830 ) ;
#3155=CARTESIAN_POINT ( 'NONE',  ( 792.3570229623691148, -165.1800572038745543, -373.1304606946836770 ) ) ;
#3159=CARTESIAN_POINT ( 'NONE',  ( 754.9967657858570647, -289.5436935675103882, -365.0032342141425374 ) ) ;
#3166=CARTESIAN_POINT ( 'NONE',  ( 754.0944755984390895, -375.6237781080501463, -364.1009440267246760 ) ) ;
#3167=CARTESIAN_POINT ( 'NONE',  ( 814.5518280994195948, -135.7255117493291152, -332.4837098697145734 ) ) ;
#3168=CARTESIAN_POINT ( 'NONE',  ( 744.7301800767019131, -388.8164208402374129, -337.4774526936615757 ) ) ;
#3173=CARTESIAN_POINT ( 'NONE',  ( 746.0683387631852383, -139.4419599262326699, -331.3260364891676204 ) ) ;
#3180=CARTESIAN_POINT ( 'NONE',  ( 796.7737145352015204, -20.63460265842048003, -370.7187646348536987 ) ) ;
#3181=EDGE_CURVE ( 'NONE', #29825, #17451, #35755, .T. ) ;
#3184=CARTESIAN_POINT ( 'NONE',  ( 791.9812246680005501, -188.6346026584199365, -361.9419747391813189 ) ) ;
#3185=CARTESIAN_POINT ( 'NONE',  ( 750.9282345327678740, -424.9181544815158986, -319.8311093483690115 ) ) ;
#3189=CARTESIAN_POINT ( 'NONE',  ( 767.8955696845333705, -264.4527844766016074, -362.1676090361162323 ) ) ;
#3192=CARTESIAN_POINT ( 'NONE',  ( 802.9823548866075953, -241.0999726633345119, -330.0799878456151077 ) ) ;
#3193=CARTESIAN_POINT ( 'NONE',  ( 755.5713283507202505, -269.3618753856924286, -334.6858677611754729 ) ) ;
#3194=CARTESIAN_POINT ( 'NONE',  ( 778.1981804954715471, -442.2709662947827383, -314.8072714833591021 ) ) ;
#3195=CARTESIAN_POINT ( 'NONE',  ( 788.7366044899766848, -83.90732993114754379, -316.5762568750059813 ) ) ;
#3199=CARTESIAN_POINT ( 'NONE',  ( 744.6391490659812007, -38.73633629969877035, -338.7502325331110455 ) ) ;
#3206=CARTESIAN_POINT ( 'NONE',  ( 784.1219089521767955, 2.718209154846545683, -315.0488828828318333 ) ) ;
#3207=CARTESIAN_POINT ( 'NONE',  ( 763.0537975583476964, -72.45278447660213317, -371.0346526505628617 ) ) ;
#3210=CARTESIAN_POINT ( 'NONE',  ( 764.8639956371174549, -416.0891481129645513, -319.7806653035542013 ) ) ;
#3212=CARTESIAN_POINT ( 'NONE',  ( 814.2001403089898304, -209.3618753856926276, -347.4397851343538264 ) ) ;
#3218=CARTESIAN_POINT ( 'NONE',  ( 813.2346286133761168, -269.2601417444139997, -328.9521613784389160 ) ) ;
#3221=CARTESIAN_POINT ( 'NONE',  ( 767.7687537140311633, -287.9073299311468759, -372.7932403749916830 ) ) ;
#3222=LINE ( 'NONE', #31169, #16909 ) ;
#3225=CARTESIAN_POINT ( 'NONE',  ( 800.2193346964447755, -402.9982390220555430, -355.1360043628815788 ) ) ;
#3227=CARTESIAN_POINT ( 'NONE',  ( 781.8018195045266339, -190.2709662947835909, -365.1927285166406705 ) ) ;
#3228=CARTESIAN_POINT ( 'NONE',  ( 812.6845335610512393, -55.98741447168748664, -353.5525998758768651 ) ) ;
#3229=CARTESIAN_POINT ( 'NONE',  ( 775.9200461376533440, -191.8055962898689017, -315.3028492785443291 ) ) ;
#3235=CARTESIAN_POINT ( 'NONE',  ( 804.9363028652555840, -88.27096629478390355, -338.2165204200192079 ) ) ;
#3236=CARTESIAN_POINT ( 'NONE',  ( 790.8726784830453198, -202.7146871989597514, -362.5472867521010585 ) ) ;
#3238=CARTESIAN_POINT ( 'NONE',  ( 815.0009284576459549, -6.351050835323991173, -338.7629533639073429 ) ) ;
#3242=VECTOR ( 'NONE', #3579, 1000.000000000000000 ) ;
#3245=CARTESIAN_POINT ( 'NONE',  ( 747.6481478633932056, -301.0999726633342561, -353.4146539503763620 ) ) ;
#3249=CARTESIAN_POINT ( 'NONE',  ( 790.9844846989617508, -142.3726999360620766, -317.2208543904092721 ) ) ;
#3250=CARTESIAN_POINT ( 'NONE',  ( 755.0636971347428243, -148.2709662947837330, -341.7834795799807353 ) ) ;
#3251=CARTESIAN_POINT ( 'NONE',  ( 785.3687786644885591, -347.3618753856922012, -315.3201227861280813 ) ) ;
#3262=CARTESIAN_POINT ( 'NONE',  ( 815.3608509340175488, -362.7363362996977116, -341.2497674668889545 ) ) ;
#3266=CARTESIAN_POINT ( 'NONE',  ( 802.1676090361156639, -326.6346026584193396, -327.8955696845344505 ) ) ;
#3267=CARTESIAN_POINT ( 'NONE',  ( 804.6971507214547046, -219.2817908451527558, -344.0799538623459739 ) ) ;
#3274=CARTESIAN_POINT ( 'NONE',  ( 810.7187646348534145, -402.4527844766010389, -356.7737145352016341 ) ) ;
#3280=CARTESIAN_POINT ( 'NONE',  ( 777.5031285880264704, -46.81642084023858530, -374.9108240113588408 ) ) ;
#3281=CARTESIAN_POINT ( 'NONE',  ( 756.5762568750052424, -291.1800572038741848, -348.7366044899774238 ) ) ;
#3285=CARTESIAN_POINT ( 'NONE',  ( 805.6418435158337843, -29.46360902697153250, -363.8556311672236916 ) ) ;
#3286=CARTESIAN_POINT ( 'NONE',  ( 760.5453621957607311, -69.07832356259653750, -323.8424801807151425 ) ) ;
#3294=CARTESIAN_POINT ( 'NONE',  ( 802.1676090361156639, -62.63460265842031305, -327.8955696845344505 ) ) ;
#3296=CARTESIAN_POINT ( 'NONE',  ( 759.2295555964440155, -352.1692326535046504, -353.9708237608231229 ) ) ;
#3300=CARTESIAN_POINT ( 'NONE',  ( 756.1443688327750579, -405.6237781080500326, -314.3581564841659315 ) ) ;
#3306=CARTESIAN_POINT ( 'NONE',  ( 792.2312462859673587, -251.9073299311470748, -307.2067596250082602 ) ) ;
#3308=ORIENTED_EDGE ( 'NONE', *, *, #36589, .T. ) ;
#3310=CARTESIAN_POINT ( 'NONE',  ( 805.1927285166399315, -208.8164208402380666, -341.8018195045277707 ) ) ;
#3313=CARTESIAN_POINT ( 'NONE',  ( 778.1981804954714335, -370.2709662947831362, -314.8072714833589885 ) ) ;
#3314=CARTESIAN_POINT ( 'NONE',  ( 795.1360043628807261, -20.08914811296592973, -360.2193346964456282 ) ) ;
#3322=CARTESIAN_POINT ( 'NONE',  ( 793.0897708529556667, -462.5545181178792973, -361.3366627262616362 ) ) ;
#3324=DIRECTION ( 'NONE',  ( -0.000000000000000000, -1.110223024625155554E-15, -1.000000000000000000 ) ) ;
#3326=CARTESIAN_POINT ( 'NONE',  ( 754.3581564841646241, -257.4636090269708575, -316.1443688327762516 ) ) ;
#3331=CARTESIAN_POINT ( 'NONE',  ( 800.2193346964447755, -234.9982390220561683, -355.1360043628815788 ) ) ;
#3332=CARTESIAN_POINT ( 'NONE',  ( 758.6633372737375112, -404.5328690171409107, -326.9102291470432533 ) ) ;
#3335=CARTESIAN_POINT ( 'NONE',  ( 804.4086373105744769, -121.6454272087894282, -333.3843516231986541 ) ) ;
#3340=CARTESIAN_POINT ( 'NONE',  ( 786.2056067578752163, 12.19440371013049784, -374.4686193811670023 ) ) ;
#3341=CARTESIAN_POINT ( 'NONE',  ( 813.1304606946831655, -305.9073299311468190, -352.3570229623691716 ) ) ;
#3344=CARTESIAN_POINT ( 'NONE',  ( 785.3687786644884454, -83.36187538569296862, -315.3201227861279676 ) ) ;
#3346=CARTESIAN_POINT ( 'NONE',  ( 788.7631598425961101, -217.4419599262324141, -305.7194118038759143 ) ) ;
#3348=CARTESIAN_POINT ( 'NONE',  ( 782.5225473063381969, -430.2709662947827383, -375.2698199232970637 ) ) ;
#3349=CARTESIAN_POINT ( 'NONE',  ( 779.9999999999992042, -462.9681489794448339, -339.9999999999999432 ) ) ;
#3354=CARTESIAN_POINT ( 'NONE',  ( 762.1405469898971887, -433.5436935675099903, -357.8594530101015607 ) ) ;
#3355=CIRCLE ( 'NONE', #43885, 30.00000000000008171 ) ;
#3361=CARTESIAN_POINT ( 'NONE',  ( 802.7791456095903868, -268.7146871989595525, -329.0155153010375102 ) ) ;
#3363=CARTESIAN_POINT ( 'NONE',  ( 811.6461892240364477, -292.7146871989594956, -324.1737431748509835 ) ) ;
#3369=CARTESIAN_POINT ( 'NONE',  ( 763.2154366446407039, -45.62377810805114109, -321.4292242960311228 ) ) ;
#3370=CARTESIAN_POINT ( 'NONE',  ( 771.1735550268778070, -177.1800572038744690, -316.3353852180827630 ) ) ;
#3371=CARTESIAN_POINT ( 'NONE',  ( 774.6858677611749044, -201.7255117493290015, -315.5713283507209894 ) ) ;
#3374=CARTESIAN_POINT ( 'NONE',  ( 800.9747183278959710, -108.9982390220565804, -311.9810565676471583 ) ) ;
#3375=CARTESIAN_POINT ( 'NONE',  ( 759.9864689768902508, -122.0891481129656171, -354.9819416627836404 ) ) ;
#3377=CARTESIAN_POINT ( 'NONE',  ( 754.7162404726377645, -398.7363362996976548, -339.4709603349214717 ) ) ;
#3385=CARTESIAN_POINT ( 'NONE',  ( 773.4516893846965786, -355.6454272087887603, -315.8398074228977066 ) ) ;
#3386=CARTESIAN_POINT ( 'NONE',  ( 800.2193346964447755, -354.9982390220557704, -355.1360043628815788 ) ) ;
#3387=CARTESIAN_POINT ( 'NONE',  ( 773.7305795820266212, -153.2817908451529831, -374.8230680027170365 ) ) ;
#3389=CIRCLE ( 'NONE', #44586, 30.00000000000008171 ) ;
#3394=CARTESIAN_POINT ( 'NONE',  ( 804.6798772138708955, -447.7255117493280636, -334.6312213355107019 ) ) ;
#3395=CARTESIAN_POINT ( 'NONE',  ( 810.4231160770870019, -144.5545181178802636, -321.9338519418446936 ) ) ;
#3400=CARTESIAN_POINT ( 'NONE',  ( 808.0189434323515343, -206.0891481129653471, -319.0252816721025511 ) ) ;
#3403=CARTESIAN_POINT ( 'NONE',  ( 804.7487373415286811, -331.5436935675104451, -364.7487373415288516 ) ) ;
#3410=CARTESIAN_POINT ( 'NONE',  ( 813.2346286133761168, -389.2601417444136018, -328.9521613784389160 ) ) ;
#3411=CARTESIAN_POINT ( 'NONE',  ( 751.6929314249748586, -126.9982390220565094, -318.8095938919659034 ) ) ;
#3412=CARTESIAN_POINT ( 'NONE',  ( 745.0891759886404770, -436.2709662947827951, -342.4968714119734159 ) ) ;
#3416=CARTESIAN_POINT ( 'NONE',  ( 752.4576283171824116, -165.0783235625962391, -317.7880784355627952 ) ) ;
#3420=CIRCLE ( 'NONE', #15201, 20.00000000000001776 ) ;
#3421=CARTESIAN_POINT ( 'NONE',  ( 767.8955696845333705, -144.4527844766018632, -362.1676090361162323 ) ) ;
#3423=CARTESIAN_POINT ( 'NONE',  ( 749.2812353651451076, -6.452784476602343666, -323.2262854647983090 ) ) ;
#3425=ORIENTED_EDGE ( 'NONE', *, *, #40263, .F. ) ;
#3426=CARTESIAN_POINT ( 'NONE',  ( 802.2119215644370342, -414.0090635724249637, -367.5423716828165084 ) ) ;
#3429=CARTESIAN_POINT ( 'NONE',  ( 757.8323909638827445, -266.6346026584197375, -352.1044303154654358 ) ) ;
#3434=CARTESIAN_POINT ( 'NONE',  ( 787.5531968255692163, -261.8272453906071746, -316.1348686366205811 ) ) ;
#3435=CARTESIAN_POINT ( 'NONE',  ( 803.4237431249931660, -255.1800572038742700, -331.2633955100225194 ) ) ;
#3436=CARTESIAN_POINT ( 'NONE',  ( 800.2193346964446619, -450.9982390220554294, -355.1360043628816925 ) ) ;
#3437=CARTESIAN_POINT ( 'NONE',  ( 771.2633955100217236, -119.9073299311474443, -363.4237431249939618 ) ) ;
#3442=CARTESIAN_POINT ( 'NONE',  ( 786.2694204179717872, -45.28179084515329578, -305.1769319972829067 ) ) ;
#3448=CARTESIAN_POINT ( 'NONE',  ( 758.4439275373578084, -12.55451811788067751, -353.2243759319684386 ) ) ;
#3449=CARTESIAN_POINT ( 'NONE',  ( 811.0346526505617248, -110.6346026584201923, -323.0537975583478101 ) ) ;
#3454=CARTESIAN_POINT ( 'NONE',  ( 792.3570229623688874, -189.1800572038744122, -373.1304606946836202 ) ) ;
#3459=DIRECTION ( 'NONE',  ( -0.000000000000000000, 0.000000000000000000, 1.000000000000000000 ) ) ;
#3460=CARTESIAN_POINT ( 'NONE',  ( 754.0944755984390895, -255.6237781080504874, -364.1009440267246760 ) ) ;
#3463=CARTESIAN_POINT ( 'NONE',  ( 813.1304606946830518, -329.9073299311467053, -352.3570229623690580 ) ) ;
#3464=FACE_OUTER_BOUND ( 'NONE', #14443, .T. ) ;
#3467=CARTESIAN_POINT ( 'NONE',  ( 814.8230680027162407, -29.80559628986937781, -333.7305795820267917 ) ) ;
#3468=CARTESIAN_POINT ( 'NONE',  ( 804.9363028652555840, -376.2709662947829656, -338.2165204200192079 ) ) ;
#3471=CARTESIAN_POINT ( 'NONE',  ( 746.7653713866222915, -65.26014174441471027, -351.0478386215610271 ) ) ;
#3472=CARTESIAN_POINT ( 'NONE',  ( 794.1144889064781864, -178.1692326535052473, -360.9840315886528401 ) ) ;
#3476=CARTESIAN_POINT ( 'NONE',  ( 771.1735550268778070, -81.18005720387481006, -316.3353852180827630 ) ) ;
#3477=CARTESIAN_POINT ( 'NONE',  ( 799.4546378042377910, -201.0783235625961254, -356.1575198192848006 ) ) ;
#3480=CARTESIAN_POINT ( 'NONE',  ( 788.7631598425961101, -25.44195992623301450, -305.7194118038759143 ) ) ;
#3485=CARTESIAN_POINT ( 'NONE',  ( 799.9636004259356241, -310.9181544815160123, -311.2241431872006956 ) ) ;
#3486=AXIS2_PLACEMENT_3D ( 'NONE', #31839, #14303, #14077 ) ;
#3491=CARTESIAN_POINT ( 'NONE',  ( 769.0155153010367712, -154.3726999360620198, -362.7791456095907279 ) ) ;
#3492=CARTESIAN_POINT ( 'NONE',  ( 781.7834795799800531, -154.8164208402382371, -315.0636971347436202 ) ) ;
#3493=CARTESIAN_POINT ( 'NONE',  ( 797.6776695296629214, -355.5436935675103882, -357.6776695296636603 ) ) ;
#3504=CARTESIAN_POINT ( 'NONE',  ( 814.8207195650702488, -362.1908817542432644, -336.2433038121456548 ) ) ;
#3509=CARTESIAN_POINT ( 'NONE',  ( 804.9363028652555840, -376.2709662947829656, -338.2165204200192079 ) ) ;
#3512=CARTESIAN_POINT ( 'NONE',  ( 805.2837595273609850, -218.7363362996982232, -340.5290396650784714 ) ) ;
#3516=CARTESIAN_POINT ( 'NONE',  ( 810.7187646348534145, -426.4527844766010389, -356.7737145352016341 ) ) ;
#3521=CARTESIAN_POINT ( 'NONE',  ( 800.9747183278959710, -36.99823902205679360, -311.9810565676471583 ) ) ;
#3522=CARTESIAN_POINT ( 'NONE',  ( 774.6858677611749044, -297.7255117493286889, -315.5713283507209894 ) ) ;
#3526=CARTESIAN_POINT ( 'NONE',  ( 811.3240766477731540, -28.37269993606244967, -355.6651683502462902 ) ) ;
#3527=CARTESIAN_POINT ( 'NONE',  ( 793.2243759319678702, -74.53286901714196233, -318.4439275373583200 ) ) ;
#3535=CARTESIAN_POINT ( 'NONE',  ( 781.7834795799800531, 13.18357915976123174, -315.0636971347436202 ) ) ;
#3536=VERTEX_POINT ( 'NONE', #11072 ) ;
#3537=CARTESIAN_POINT ( 'NONE',  ( 801.9419747391806368, -66.45278447660216159, -351.9812246680014027 ) ) ;
#3539=CARTESIAN_POINT ( 'NONE',  ( 769.1273215169530886, -382.7146871989591546, -317.4527132478988847 ) ) ;
#3543=CARTESIAN_POINT ( 'NONE',  ( 752.4576283171824116, -405.0783235625954148, -317.7880784355627952 ) ) ;
#3546=ORIENTED_EDGE ( 'NONE', *, *, #36022, .T. ) ;
#3551=CARTESIAN_POINT ( 'NONE',  ( 745.0891759886404770, -244.2709662947834204, -342.4968714119734159 ) ) ;
#3555=CARTESIAN_POINT ( 'NONE',  ( 800.0135310231082713, -230.0891481129652618, -325.0180583372163028 ) ) ;
#3557=CARTESIAN_POINT ( 'NONE',  ( 797.6776695296629214, -355.5436935675103882, -357.6776695296636603 ) ) ;
#3558=CARTESIAN_POINT ( 'NONE',  ( 804.6798772138708955, -15.72551174932958951, -334.6312213355107019 ) ) ;
#3563=CARTESIAN_POINT ( 'NONE',  ( 797.6776695296629214, -19.54369356751139364, -357.6776695296636603 ) ) ;
#3564=DIRECTION ( 'NONE',  ( -0.7071067811865697772, 0.000000000000000000, 0.7071067811865252573 ) ) ;
#3565=DIRECTION ( 'NONE',  ( -0.000000000000000000, 1.110223024625155554E-15, 1.000000000000000000 ) ) ;
#3566=VERTEX_POINT ( 'NONE', #36012 ) ;
#3567=CARTESIAN_POINT ( 'NONE',  ( 745.1792804349281596, -278.1908817542434917, -343.7566961878542884 ) ) ;
#3571=CARTESIAN_POINT ( 'NONE',  ( 774.6312213355099630, -239.3618753856924570, -364.6798772138717482 ) ) ;
#3572=CARTESIAN_POINT ( 'NONE',  ( 756.7813123517142913, -379.9874144716865203, -329.9779781133712504 ) ) ;
#3575=CARTESIAN_POINT ( 'NONE',  ( 766.9102291470427417, -114.5545181178803631, -318.6633372737382501 ) ) ;
#3577=CARTESIAN_POINT ( 'NONE',  ( 761.9338519418445230, 9.467130982857780097, -370.4231160770881957 ) ) ;
#3578=CARTESIAN_POINT ( 'NONE',  ( 758.8095938919644823, -320.0891481129648923, -311.6929314249762797 ) ) ;
#3579=DIRECTION ( 'NONE',  ( -0.000000000000000000, 1.000000000000000000, -0.000000000000000000 ) ) ;
#3580=FACE_OUTER_BOUND ( 'NONE', #40404, .T. ) ;
#3581=CARTESIAN_POINT ( 'NONE',  ( 785.3141322388236176, -93.72551174932934259, -364.4286716492789537 ) ) ;
#3583=CARTESIAN_POINT ( 'NONE',  ( 748.3538107759620743, -208.7146871989596946, -355.8262568251490165 ) ) ;
#3585=CARTESIAN_POINT ( 'NONE',  ( 751.6929314249748586, -438.9982390220553157, -318.8095938919659034 ) ) ;
#3589=CARTESIAN_POINT ( 'NONE',  ( 796.7845633553578182, 14.37622189194867417, -358.5707757039688204 ) ) ;
#3596=CARTESIAN_POINT ( 'NONE',  ( 797.8594530101008786, -229.5436935675106440, -322.1405469898980982 ) ) ;
#3598=CARTESIAN_POINT ( 'NONE',  ( 754.8983024940795303, -282.8965053807776258, -336.9254006560228163 ) ) ;
#3600=CARTESIAN_POINT ( 'NONE',  ( 814.8230680027162407, -293.8055962898685607, -333.7305795820267917 ) ) ;
#3606=CARTESIAN_POINT ( 'NONE',  ( 766.7756240680305382, -38.53286901714206891, -361.5560724626415663 ) ) ;
#3607=CARTESIAN_POINT ( 'NONE',  ( 756.3353852180819104, -197.9073299311472169, -331.1735550268788302 ) ) ;
#3609=CARTESIAN_POINT ( 'NONE',  ( 808.3070685750230950, -138.9982390220563957, -361.1904061080339261 ) ) ;
#3611=CARTESIAN_POINT ( 'NONE',  ( 792.1044303154646968, -132.4527844766019200, -317.8323909638837677 ) ) ;
#3613=CARTESIAN_POINT ( 'NONE',  ( 804.1105419155481968, -387.8272453906067767, -347.6308680596136469 ) ) ;
#3620=CARTESIAN_POINT ( 'NONE',  ( 804.1105419155481968, -387.8272453906067767, -347.6308680596136469 ) ) ;
#3621=CARTESIAN_POINT ( 'NONE',  ( 781.8018195045266339, -358.2709662947829088, -365.1927285166406705 ) ) ;
#3622=CARTESIAN_POINT ( 'NONE',  ( 793.5525998758768083, -175.0999726633346825, -372.6845335610516941 ) ) ;
#3626=CARTESIAN_POINT ( 'NONE',  ( 798.7617431975189675, -291.6237781080503169, -323.0428371773161871 ) ) ;
#3627=CARTESIAN_POINT ( 'NONE',  ( 781.7834795799800531, -442.8164208402372992, -315.0636971347436202 ) ) ;
#3628=CARTESIAN_POINT ( 'NONE',  ( 776.2046728542105711, -164.1908817542438612, -304.8212110874238761 ) ) ;
#3633=CARTESIAN_POINT ( 'NONE',  ( 787.4397851343537695, -213.7255117493289731, -374.2001403089903988 ) ) ;
#3638=CARTESIAN_POINT ( 'NONE',  ( 761.9338519418445230, -110.5328690171418629, -370.4231160770881957 ) ) ;
#3640=CARTESIAN_POINT ( 'NONE',  ( 763.0537975583475827, -336.4527844766012095, -371.0346526505627480 ) ) ;
#3641=DIRECTION ( 'NONE',  ( 1.000000000000000000, 0.000000000000000000, -0.000000000000000000 ) ) ;
#3645=CARTESIAN_POINT ( 'NONE',  ( 746.7653713866222915, -425.2601417444136018, -351.0478386215610271 ) ) ;
#3646=CARTESIAN_POINT ( 'NONE',  ( 782.5225473063381969, -142.2709662947837330, -375.2698199232970637 ) ) ;
#3647=CARTESIAN_POINT ( 'NONE',  ( 796.7737145352015204, -404.6346026584193396, -370.7187646348536987 ) ) ;
#3651=CARTESIAN_POINT ( 'NONE',  ( 768.8385539511368734, -191.2601417444143976, -306.4236121716840557 ) ) ;
#3657=CARTESIAN_POINT ( 'NONE',  ( 758.8095938919642549, -56.08914811296580893, -311.6929314249763365 ) ) ;
#3660=CARTESIAN_POINT ( 'NONE',  ( 744.6391490659812007, -446.7363362996975980, -338.7502325331110455 ) ) ;
#3665=CARTESIAN_POINT ( 'NONE',  ( 755.3201227861273992, -267.7255117493286320, -345.3687786644892981 ) ) ;
#3669=CARTESIAN_POINT ( 'NONE',  ( 793.9708237608222134, -262.9181544815162965, -319.2295555964448681 ) ) ;
#3670=CARTESIAN_POINT ( 'NONE',  ( 762.3223304703356007, -247.5436935675106724, -322.3223304703362828 ) ) ;
#3672=CARTESIAN_POINT ( 'NONE',  ( 781.7834795799800531, -106.8164208402383935, -315.0636971347436202 ) ) ;
#3677=CARTESIAN_POINT ( 'NONE',  ( 745.1792804349281596, -62.19088175424416676, -343.7566961878542884 ) ) ;
#3683=CARTESIAN_POINT ( 'NONE',  ( 755.5913626894240451, -13.64542720878976390, -346.6156483768012890 ) ) ;
#3684=CARTESIAN_POINT ( 'NONE',  ( 813.1304606946831655, -89.90732993114752958, -352.3570229623691716 ) ) ;
#3688=CARTESIAN_POINT ( 'NONE',  ( 763.0537975583475827, -240.4527844766015221, -371.0346526505627480 ) ) ;
#3692=CARTESIAN_POINT ( 'NONE',  ( 766.5853460496234675, -277.9874144716867477, -372.3518521366060554 ) ) ;
#3694=CARTESIAN_POINT ( 'NONE',  ( 808.0189434323515343, -302.0891481129650629, -319.0252816721025511 ) ) ;
#3698=CARTESIAN_POINT ( 'NONE',  ( 801.9419747391806368, -378.4527844766011526, -351.9812246680014027 ) ) ;
#3700=CARTESIAN_POINT ( 'NONE',  ( 788.7366044899766848, -203.9073299311471885, -316.5762568750059813 ) ) ;
#3701=CARTESIAN_POINT ( 'NONE',  ( 814.8230680027162407, -101.8055962898691718, -333.7305795820267917 ) ) ;
#3706=CARTESIAN_POINT ( 'NONE',  ( 765.8855110935204493, -214.1692326535052189, -319.0159684113471599 ) ) ;
#3708=CARTESIAN_POINT ( 'NONE',  ( 744.8212110874229666, -42.89650538077842157, -336.2046728542121627 ) ) ;
#3713=CARTESIAN_POINT ( 'NONE',  ( 793.5525998758768083, -319.0999726633342561, -372.6845335610516941 ) ) ;
#3716=CARTESIAN_POINT ( 'NONE',  ( 755.8894580844503253, -159.8272453906075157, -332.3691319403863531 ) ) ;
#3717=CARTESIAN_POINT ( 'NONE',  ( 802.1676090361156639, -134.6346026584201070, -327.8955696845344505 ) ) ;
#3718=CARTESIAN_POINT ( 'NONE',  ( 800.2193346964446619, -354.9982390220557136, -355.1360043628816925 ) ) ;
#3727=CARTESIAN_POINT ( 'NONE',  ( 766.4474001241216001, -379.0999726633341993, -307.3154664389482491 ) ) ;
#3728=CARTESIAN_POINT ( 'NONE',  ( 814.9108240113580450, -16.27096629478413092, -337.5031285880265273 ) ) ;
#3731=CARTESIAN_POINT ( 'NONE',  ( 791.9812246680005501, -356.6346026584193964, -361.9419747391813189 ) ) ;
#3734=CARTESIAN_POINT ( 'NONE',  ( 780.5236548040995785, -236.7363362996981380, -314.9735926884559944 ) ) ;
#3738=CARTESIAN_POINT ( 'NONE',  ( 755.2512626584698410, -415.5436935675102177, -315.2512626584710915 ) ) ;
#3743=CARTESIAN_POINT ( 'NONE',  ( 763.0537975583475827, -48.45278447660219712, -371.0346526505627480 ) ) ;
#3745=CARTESIAN_POINT ( 'NONE',  ( 797.8594530101008786, -277.5436935675105019, -322.1405469898980982 ) ) ;
#3749=CARTESIAN_POINT ( 'NONE',  ( 745.1792804349281596, -38.19088175424422360, -343.7566961878542884 ) ) ;
#3750=CARTESIAN_POINT ( 'NONE',  ( 765.8855110935204493, -70.16923265350563099, -319.0159684113471599 ) ) ;
#3753=CARTESIAN_POINT ( 'NONE',  ( 771.1735550268778070, 14.81994279612486309, -316.3353852180827630 ) ) ;
#3755=CARTESIAN_POINT ( 'NONE',  ( 788.7366044899766848, -107.9073299311474727, -316.5762568750059813 ) ) ;
#3756=CARTESIAN_POINT ( 'NONE',  ( 795.9930595647434757, -387.0783235625955285, -320.7433823573372820 ) ) ;
#3759=CARTESIAN_POINT ( 'NONE',  ( 783.7566961878529810, -408.8965053807772847, -305.1792804349288417 ) ) ;
#3760=LINE ( 'NONE', #7240, #27889 ) ;
#3761=ORIENTED_EDGE ( 'NONE', *, *, #25566, .T. ) ;
#3765=CARTESIAN_POINT ( 'NONE',  ( 808.3070685750230950, -258.9982390220561115, -361.1904061080339261 ) ) ;
#3769=CARTESIAN_POINT ( 'NONE',  ( 797.8594530101009923, -253.5436935675105588, -322.1405469898982119 ) ) ;
#3771=CARTESIAN_POINT ( 'NONE',  ( 762.1405469898971887, -361.5436935675103882, -357.8594530101015607 ) ) ;
#3772=CARTESIAN_POINT ( 'NONE',  ( 758.0580252608178853, -6.452784476602343666, -328.0187753319985404 ) ) ;
#3777=CARTESIAN_POINT ( 'NONE',  ( 757.8323909638827445, -2.634602658420536869, -352.1044303154654358 ) ) ;
#3778=FACE_OUTER_BOUND ( 'NONE', #39106, .T. ) ;
#3781=CARTESIAN_POINT ( 'NONE',  ( 750.9282345327678740, -280.9181544815162965, -319.8311093483690115 ) ) ;
#3784=CARTESIAN_POINT ( 'NONE',  ( 781.7834795799800531, -274.8164208402378108, -315.0636971347436202 ) ) ;
#3785=CARTESIAN_POINT ( 'NONE',  ( 784.0799538623451781, -395.8055962898682765, -364.6971507214555572 ) ) ;
#3788=CARTESIAN_POINT ( 'NONE',  ( 790.0220218866281812, -127.0999726633348672, -363.2186876482849129 ) ) ;
#3792=CARTESIAN_POINT ( 'NONE',  ( 810.1134526219336749, 15.46713098285775878, -357.8822607201570349 ) ) ;
#3793=CARTESIAN_POINT ( 'NONE',  ( 767.6429770376291799, -321.1800572038740711, -306.8695393053162093 ) ) ;
#3796=CARTESIAN_POINT ( 'NONE',  ( 746.7653713866222915, -185.2601417444143692, -351.0478386215610271 ) ) ;
#3798=CARTESIAN_POINT ( 'NONE',  ( 799.9636004259356241, 1.081845518482914104, -311.2241431872006956 ) ) ;
#3804=CARTESIAN_POINT ( 'NONE',  ( 754.8983024940795303, 5.103494619221427442, -336.9254006560228163 ) ) ;
#3806=LINE ( 'NONE', #574, #29221 ) ;
#3810=CARTESIAN_POINT ( 'NONE',  ( 755.8398074228967971, -307.4419599262320730, -333.4516893846970333 ) ) ;
#3812=CARTESIAN_POINT ( 'NONE',  ( 803.8556311672234642, -297.6237781080502600, -365.6418435158340117 ) ) ;
#3815=EDGE_CURVE ( 'NONE', #31813, #29825, #6235, .T. ) ;
#3816=VERTEX_POINT ( 'NONE', #6003 ) ;
#3819=CARTESIAN_POINT ( 'NONE',  ( 784.0799538623451781, -59.80559628986927834, -364.6971507214555572 ) ) ;
#3820=CARTESIAN_POINT ( 'NONE',  ( 781.7834795799800531, -154.8164208402382371, -315.0636971347436202 ) ) ;
#3821=CARTESIAN_POINT ( 'NONE',  ( 755.5713283507202505, -221.3618753856925707, -334.6858677611754729 ) ) ;
#3823=CARTESIAN_POINT ( 'NONE',  ( 810.7187646348534145, -138.4527844766019200, -356.7737145352016341 ) ) ;
#3824=VERTEX_POINT ( 'NONE', #23331 ) ;
#3825=VECTOR ( 'NONE', #37918, 1000.000000000000000 ) ;
#3826=CARTESIAN_POINT ( 'NONE',  ( 762.1405469898973024, -145.5436935675109851, -357.8594530101016176 ) ) ;
#3828=CARTESIAN_POINT ( 'NONE',  ( 773.4516893846965786, -403.6454272087884760, -315.8398074228977066 ) ) ;
#3836=CARTESIAN_POINT ( 'NONE',  ( 754.7162404726377645, -398.7363362996976548, -339.4709603349214717 ) ) ;
#3838=CARTESIAN_POINT ( 'NONE',  ( 814.4686193811664907, -171.2817908451529263, -346.2056067578752732 ) ) ;
#3843=CARTESIAN_POINT ( 'NONE',  ( 804.9511171171677688, -293.8055962898685607, -335.8780910478229202 ) ) ;
#3845=CARTESIAN_POINT ( 'NONE',  ( 745.7194118038753459, -205.6454272087891297, -348.7631598425976449 ) ) ;
#3851=CARTESIAN_POINT ( 'NONE',  ( 811.0346526505617248, -206.6346026584198796, -323.0537975583478101 ) ) ;
#3853=CARTESIAN_POINT ( 'NONE',  ( 778.1981804954714335, 13.72903370521577138, -314.8072714833589885 ) ) ;
#3855=CARTESIAN_POINT ( 'NONE',  ( 746.0683387631852383, -91.44195992623282621, -331.3260364891676204 ) ) ;
#3857=CARTESIAN_POINT ( 'NONE',  ( 772.5602148656447525, -345.7255117493285184, -305.7998596910095443 ) ) ;
#3864=CARTESIAN_POINT ( 'NONE',  ( 808.7758568127978833, -412.1692326535045936, -320.0363995740631822 ) ) ;
#3865=CARTESIAN_POINT ( 'NONE',  ( 792.2312462859673587, -419.9073299311465348, -307.2067596250082602 ) ) ;
#3869=CARTESIAN_POINT ( 'NONE',  ( 815.1787889125755555, -174.8965053807779952, -343.7953271457877804 ) ) ;
#3875=CARTESIAN_POINT ( 'NONE',  ( 745.0891759886404770, -52.27096629478401724, -342.4968714119734159 ) ) ;
#3879=CARTESIAN_POINT ( 'NONE',  ( 788.6739635108323228, -439.6454272087884760, -373.9316612368139090 ) ) ;
#3883=CARTESIAN_POINT ( 'NONE',  ( 756.3353852180819104, -293.9073299311468759, -331.1735550268788302 ) ) ;
#3887=CARTESIAN_POINT ( 'NONE',  ( 766.0291762391763086, -298.9181544815161828, -360.7704444035551319 ) ) ;
#3888=CARTESIAN_POINT ( 'NONE',  ( 767.8955696845333705, -264.4527844766016074, -362.1676090361162323 ) ) ;
#3890=CARTESIAN_POINT ( 'NONE',  ( 762.3223304703356007, -127.5436935675110561, -322.3223304703362828 ) ) ;
#3896=CARTESIAN_POINT ( 'NONE',  ( 814.2805881961230625, -73.64542720878957027, -331.2368401574024119 ) ) ;
#3902=CARTESIAN_POINT ( 'NONE',  ( 763.8424801807145741, -42.00906357242603661, -320.5453621957614700 ) ) ;
#3903=CARTESIAN_POINT ( 'NONE',  ( 814.5518280994195948, -111.7255117493292857, -332.4837098697145166 ) ) ;
#3907=CARTESIAN_POINT ( 'NONE',  ( 745.0891759886404770, -220.2709662947834772, -342.4968714119734159 ) ) ;
#3912=CARTESIAN_POINT ( 'NONE',  ( 814.8230680027162407, -317.8055962898684470, -333.7305795820267917 ) ) ;
#3915=CARTESIAN_POINT ( 'NONE',  ( 796.7737145352015204, -308.6346026584195670, -370.7187646348536987 ) ) ;
#3918=CARTESIAN_POINT ( 'NONE',  ( 767.8955696845333705, -384.4527844766011526, -362.1676090361162323 ) ) ;
#3920=CARTESIAN_POINT ( 'NONE',  ( 800.0135310231082713, -206.0891481129653471, -325.0180583372163028 ) ) ;
#3921=CARTESIAN_POINT ( 'NONE',  ( 783.7566961878529810, -96.89650538077825104, -305.1792804349288417 ) ) ;
#3924=ORIENTED_EDGE ( 'NONE', *, *, #9203, .T. ) ;
#3925=CARTESIAN_POINT ( 'NONE',  ( 803.8651313633788504, -197.2601417444143124, -332.4468031744301015 ) ) ;
#3927=CARTESIAN_POINT ( 'NONE',  ( 814.8230680027162407, -29.80559628986937781, -333.7305795820267917 ) ) ;
#3929=CARTESIAN_POINT ( 'NONE',  ( 791.7608162188021197, 205.0000000000000568, -319.9999999999999432 ) ) ;
#3933=CARTESIAN_POINT ( 'NONE',  ( 771.3260364891663130, -331.6454272087888171, -306.0683387631859773 ) ) ;
#3936=CARTESIAN_POINT ( 'NONE',  ( 798.5707757039680246, -173.4636090269710849, -356.7845633553585003 ) ) ;
#3937=CARTESIAN_POINT ( 'NONE',  ( 794.9819416627830151, -156.9982390220564241, -319.9864689768909898 ) ) ;
#3939=CARTESIAN_POINT ( 'NONE',  ( 754.8072714833583632, -340.8164208402376403, -338.1981804954721156 ) ) ;
#3949=CARTESIAN_POINT ( 'NONE',  ( 795.8262568251477660, -382.3726999360613945, -308.3538107759623585 ) ) ;
#3951=CARTESIAN_POINT ( 'NONE',  ( 808.0189434323515343, 9.910851887033969021, -319.0252816721025511 ) ) ;
#3955=CARTESIAN_POINT ( 'NONE',  ( 756.5762568750052424, -363.1800572038739006, -348.7366044899774238 ) ) ;
#3958=CARTESIAN_POINT ( 'NONE',  ( 766.9102291470427417, -234.5545181178799794, -318.6633372737382501 ) ) ;
#3962=CARTESIAN_POINT ( 'NONE',  ( 814.9108240113580450, -400.2709662947828519, -337.5031285880265273 ) ) ;
#3967=CARTESIAN_POINT ( 'NONE',  ( 808.3070685750230950, -66.99823902205672255, -361.1904061080339261 ) ) ;
#3968=CARTESIAN_POINT ( 'NONE',  ( 771.1735550268778070, -273.1800572038742985, -316.3353852180827630 ) ) ;
#3973=CARTESIAN_POINT ( 'NONE',  ( 766.4474001241216001, -67.09997266333506616, -307.3154664389482491 ) ) ;
#3974=CARTESIAN_POINT ( 'NONE',  ( 780.5290396650775619, -84.35105083532374692, -365.2837595273619513 ) ) ;
#3977=CARTESIAN_POINT ( 'NONE',  ( 756.5762568750052424, -3.180057203875080063, -348.7366044899774238 ) ) ;
#3979=CARTESIAN_POINT ( 'NONE',  ( 774.6858677611749044, -81.72551174932937101, -315.5713283507209894 ) ) ;
#3980=CARTESIAN_POINT ( 'NONE',  ( 789.9200121543843807, -385.9874144716864066, -317.0176451133914384 ) ) ;
#3983=CARTESIAN_POINT ( 'NONE',  ( 808.7758568127978833, -388.1692326535045936, -320.0363995740631822 ) ) ;
#3987=AXIS2_PLACEMENT_3D ( 'NONE', #32877, #40697, #44160 ) ;
#3988=ORIENTED_EDGE ( 'NONE', *, *, #22865, .F. ) ;
#3989=CARTESIAN_POINT ( 'NONE',  ( 805.0032342141412300, -253.5436935675104735, -314.9967657858571783 ) ) ;
#3993=CARTESIAN_POINT ( 'NONE',  ( 802.9823548866075953, -49.09997266333511590, -330.0799878456151077 ) ) ;
#3994=CARTESIAN_POINT ( 'NONE',  ( 774.6858677611749044, -249.7255117493288594, -315.5713283507209894 ) ) ;
#3996=CARTESIAN_POINT ( 'NONE',  ( 794.9819416627830151, -348.9982390220558273, -319.9864689768909898 ) ) ;
#3997=CARTESIAN_POINT ( 'NONE',  ( 765.0180583372156207, -0.9982390220569063999, -360.0135310231089534 ) ) ;
#4003=CARTESIAN_POINT ( 'NONE',  ( 759.9864689768902508, -26.08914811296592262, -354.9819416627836404 ) ) ;
#4004=FACE_OUTER_BOUND ( 'NONE', #29408, .T. ) ;
#4008=CARTESIAN_POINT ( 'NONE',  ( 783.7953271457878373, -272.1908817542434917, -375.1787889125761239 ) ) ;
#4012=CARTESIAN_POINT ( 'NONE',  ( 774.6858677611749044, -249.7255117493288594, -315.5713283507209894 ) ) ;
#4014=CARTESIAN_POINT ( 'NONE',  ( 755.5913626894240451, -109.6454272087894566, -346.6156483768012890 ) ) ;
#4017=CARTESIAN_POINT ( 'NONE',  ( 794.1144889064781864, -442.1692326535044231, -360.9840315886528401 ) ) ;
#4018=CARTESIAN_POINT ( 'NONE',  ( 805.0032342141413437, -301.5436935675105588, -314.9967657858572352 ) ) ;
#4019=CARTESIAN_POINT ( 'NONE',  ( 787.4999999999992042, -512.9681489794448908, -350.0000000000000000 ) ) ;
#4022=CARTESIAN_POINT ( 'NONE',  ( 746.0683387631852383, -187.4419599262325278, -331.3260364891676204 ) ) ;
#4024=CARTESIAN_POINT ( 'NONE',  ( 805.0032342141412300, -445.5436935675098766, -314.9967657858571783 ) ) ;
#4032=CARTESIAN_POINT ( 'NONE',  ( 800.7704444035546203, 19.83076734649410966, -326.0291762391768771 ) ) ;
#4039=CARTESIAN_POINT ( 'NONE',  ( 805.1016975059191054, -294.8965053807775689, -343.0745993439771837 ) ) ;
#4042=CARTESIAN_POINT ( 'NONE',  ( 748.3538107759620743, -304.7146871989594388, -355.8262568251490165 ) ) ;
#4043=DIRECTION ( 'NONE',  ( 0.000000000000000000, 0.000000000000000000, -1.000000000000000000 ) ) ;
#4048=CARTESIAN_POINT ( 'NONE',  ( 776.9566956441375396, -84.89650538077830788, -364.8461984189686405 ) ) ;
#4049=CARTESIAN_POINT ( 'NONE',  ( 765.0180583372156207, -168.9982390220563673, -360.0135310231089534 ) ) ;
#4050=CARTESIAN_POINT ( 'NONE',  ( 800.2193346964447755, -210.9982390220561967, -355.1360043628815788 ) ) ;
#4053=CARTESIAN_POINT ( 'NONE',  ( 772.4837098697144029, -143.3618753856927697, -374.5518280994205611 ) ) ;
#4055=CARTESIAN_POINT ( 'NONE',  ( 804.4286716492782716, -137.3618753856928265, -345.3141322388244703 ) ) ;
#4057=CARTESIAN_POINT ( 'NONE',  ( 784.1219089521767955, -381.2817908451523294, -315.0488828828318333 ) ) ;
#4061=CYLINDRICAL_SURFACE ( 'NONE', #24012, 10.00000000000000888 ) ;
#4068=CARTESIAN_POINT ( 'NONE',  ( 796.9571628226829034, -383.4636090269704596, -321.2382568024804641 ) ) ;
#4070=CARTESIAN_POINT ( 'NONE',  ( 750.9282345327678740, -184.9181544815165239, -319.8311093483690115 ) ) ;
#4074=CARTESIAN_POINT ( 'NONE',  ( 800.7704444035546203, -340.1692326535047641, -326.0291762391768771 ) ) ;
#4075=CARTESIAN_POINT ( 'NONE',  ( 755.0636971347428243, -436.2709662947827951, -341.7834795799807353 ) ) ;
#4076=CARTESIAN_POINT ( 'NONE',  ( 752.7379699480933368, -180.0090635724255890, -361.9858362298580232 ) ) ;
#4083=CARTESIAN_POINT ( 'NONE',  ( 763.2262854647970016, -224.6346026584198228, -309.2812353651462445 ) ) ;
#4090=CARTESIAN_POINT ( 'NONE',  ( 751.2241431872005251, -88.16923265350555994, -359.9636004259367610 ) ) ;
#4092=CARTESIAN_POINT ( 'NONE',  ( 801.1904061080336987, -332.0891481129649492, -368.3070685750235498 ) ) ;
#4098=CARTESIAN_POINT ( 'NONE',  ( 766.5853460496234675, -397.9874144716864066, -372.3518521366060554 ) ) ;
#4100=CARTESIAN_POINT ( 'NONE',  ( 777.5031285880264704, -430.8164208402374129, -374.9108240113588408 ) ) ;
#4104=VECTOR ( 'NONE', #21357, 1000.000000000000000 ) ;
#4106=CARTESIAN_POINT ( 'NONE',  ( 795.6651683502461765, -178.7146871989598083, -371.3240766477733814 ) ) ;
#4110=ORIENTED_EDGE ( 'NONE', *, *, #45593, .F. ) ;
#4115=CARTESIAN_POINT ( 'NONE',  ( 792.2312462859673587, -35.90732993114770011, -307.2067596250082602 ) ) ;
#4118=CARTESIAN_POINT ( 'NONE',  ( 804.1009440267234822, -431.4636090269702322, -314.0944755984392600 ) ) ;
#4121=SHAPE_DEFINITION_REPRESENTATION ( #14099, #28408 ) ;
#4124=CARTESIAN_POINT ( 'NONE',  ( 788.8264449731200330, -285.1800572038740711, -363.6646147819171233 ) ) ;
#4130=CARTESIAN_POINT ( 'NONE',  ( 775.8780910478218402, -297.2817908451526137, -364.9511171171680530 ) ) ;
#4131=CARTESIAN_POINT ( 'NONE',  ( 804.6798772138708955, -279.7255117493288026, -334.6312213355107019 ) ) ;
#4132=CARTESIAN_POINT ( 'NONE',  ( 788.7366044899766848, -443.9073299311464780, -316.5762568750059813 ) ) ;
#4133=CARTESIAN_POINT ( 'NONE',  ( 800.0135310231082713, -134.0891481129655745, -325.0180583372163028 ) ) ;
#4139=CARTESIAN_POINT ( 'NONE',  ( 810.4231160770870019, -96.55451811788039151, -321.9338519418446936 ) ) ;
#4140=CARTESIAN_POINT ( 'NONE',  ( 759.9999999999992042, -512.9681489794448908, -339.9999999999999432 ) ) ;
#4145=CARTESIAN_POINT ( 'NONE',  ( 800.9840315886518738, -52.91815448151692891, -354.1144889064786412 ) ) ;
#4146=CARTESIAN_POINT ( 'NONE',  ( 767.7687537140311633, -119.9073299311474443, -372.7932403749916830 ) ) ;
#4151=CARTESIAN_POINT ( 'NONE',  ( 815.2698199232961542, -232.8164208402379245, -342.5225473063383106 ) ) ;
#4155=CARTESIAN_POINT ( 'NONE',  ( 807.5423716828161105, -321.0783235625956991, -362.2119215644372048 ) ) ;
#4158=CARTESIAN_POINT ( 'NONE',  ( 792.2312462859673587, -323.9073299311468190, -307.2067596250082602 ) ) ;
#4159=CARTESIAN_POINT ( 'NONE',  ( 779.9999999999992042, -462.9681489794448339, -339.9999999999999432 ) ) ;
#4163=CARTESIAN_POINT ( 'NONE',  ( 762.1405469898971887, -433.5436935675099903, -357.8594530101015607 ) ) ;
#4165=CARTESIAN_POINT ( 'NONE',  ( 812.6845335610512393, -79.98741447168740137, -353.5525998758768651 ) ) ;
#4171=CARTESIAN_POINT ( 'NONE',  ( 802.7791456095903868, -196.7146871989598083, -329.0155153010375102 ) ) ;
#4174=CARTESIAN_POINT ( 'NONE',  ( 798.0661480581538854, -26.53286901714210799, -309.5768839229118043 ) ) ;
#4178=ORIENTED_EDGE ( 'NONE', *, *, #40459, .T. ) ;
#4180=CARTESIAN_POINT ( 'NONE',  ( 791.0478386215596629, -333.8272453906070041, -306.7653713866226326 ) ) ;
#4183=CARTESIAN_POINT ( 'NONE',  ( 775.8780910478218402, -201.2817908451528126, -364.9511171171680530 ) ) ;
#4184=CARTESIAN_POINT ( 'NONE',  ( 771.2633955100217236, -191.9073299311471885, -363.4237431249939618 ) ) ;
#4185=CARTESIAN_POINT ( 'NONE',  ( 781.8018195045267476, -358.2709662947830225, -365.1927285166407273 ) ) ;
#4196=CARTESIAN_POINT ( 'NONE',  ( 776.2046728542105711, -428.1908817542430938, -304.8212110874238761 ) ) ;
#4197=VECTOR ( 'NONE', #23243, 1000.000000000000000 ) ;
#4198=CARTESIAN_POINT ( 'NONE',  ( 758.8095938919644823, -8.089148112965974136, -311.6929314249762797 ) ) ;
#4201=CARTESIAN_POINT ( 'NONE',  ( 805.1927285166397041, -352.8164208402374129, -341.8018195045277707 ) ) ;
#4205=CARTESIAN_POINT ( 'NONE',  ( 793.0897708529556667, -270.5545181178798657, -361.3366627262616362 ) ) ;
#4209=CARTESIAN_POINT ( 'NONE',  ( 808.0189434323515343, -446.0891481129646081, -319.0252816721025511 ) ) ;
#4214=CARTESIAN_POINT ( 'NONE',  ( 767.6429770376289525, -105.1800572038747248, -306.8695393053162093 ) ) ;
#4215=CARTESIAN_POINT ( 'NONE',  ( 755.0636971347428243, -268.2709662947833067, -341.7834795799807353 ) ) ;
#4219=CARTESIAN_POINT ( 'NONE',  ( 754.3581564841646241, -65.46360902697142592, -316.1443688327762516 ) ) ;
#4220=CARTESIAN_POINT ( 'NONE',  ( 775.9200461376533440, -95.80559628986917176, -315.3028492785443291 ) ) ;
#4224=CARTESIAN_POINT ( 'NONE',  ( 795.1360043628807261, 3.910851887033985896, -360.2193346964456282 ) ) ;
#4225=CARTESIAN_POINT ( 'NONE',  ( 764.0069404352550464, -111.0783235625964096, -359.2566176426627180 ) ) ;
#4227=CARTESIAN_POINT ( 'NONE',  ( 804.4286716492782716, -89.36187538569299704, -345.3141322388244703 ) ) ;
#4229=CARTESIAN_POINT ( 'NONE',  ( 804.1601925771018387, -415.4419599262318457, -346.5483106153029098 ) ) ;
#4232=CARTESIAN_POINT ( 'NONE',  ( 781.2497674668890113, -396.3510508353228374, -375.3608509340180603 ) ) ;
#4236=VECTOR ( 'NONE', #31435, 1000.000000000000000 ) ;
#4242=CARTESIAN_POINT ( 'NONE',  ( 796.9571628226829034, -71.46360902697141171, -321.2382568024804641 ) ) ;
#4244=CARTESIAN_POINT ( 'NONE',  ( 791.9812246680005501, -260.6346026584197375, -361.9419747391813189 ) ) ;
#4246=CARTESIAN_POINT ( 'NONE',  ( 755.3201227861273992, -411.7255117493282910, -345.3687786644892981 ) ) ;
#4247=CARTESIAN_POINT ( 'NONE',  ( 803.6646147819161570, -41.90732993114767169, -348.8264449731210561 ) ) ;
#4251=CARTESIAN_POINT ( 'NONE',  ( 778.2165204200184689, -22.81642084023865280, -364.9363028652563230 ) ) ;
#4255=CARTESIAN_POINT ( 'NONE',  ( 771.3260364891663130, -307.6454272087888171, -306.0683387631859773 ) ) ;
#4258=CARTESIAN_POINT ( 'NONE',  ( 778.2165204200184689, -262.8164208402379245, -364.9363028652563230 ) ) ;
#4260=CARTESIAN_POINT ( 'NONE',  ( 755.1538015810308480, -110.1908817542440033, -343.0433043558613804 ) ) ;
#4261=DIRECTION ( 'NONE',  ( 0.000000000000000000, 0.000000000000000000, -1.000000000000000000 ) ) ;
#4262=CARTESIAN_POINT ( 'NONE',  ( 804.7487373415286811, -331.5436935675104451, -364.7487373415288516 ) ) ;
#4267=CARTESIAN_POINT ( 'NONE',  ( 788.7631598425961101, -193.4419599262325278, -305.7194118038759143 ) ) ;
#4269=CARTESIAN_POINT ( 'NONE',  ( 781.2370466360911223, 3.263663700301089765, -304.9990715423533629 ) ) ;
#4274=CARTESIAN_POINT ( 'NONE',  ( 795.1360043628807261, -452.0891481129646650, -360.2193346964456282 ) ) ;
#4279=EDGE_LOOP ( 'NONE', ( #11514, #37775, #36088, #40359, #36090, #1787 ) ) ;
#4280=CARTESIAN_POINT ( 'NONE',  ( 761.2382568024794409, -279.6237781080503737, -356.9571628226838129 ) ) ;
#4282=CARTESIAN_POINT ( 'NONE',  ( 747.3154664389472828, -307.9874144716866340, -326.4474001241230781 ) ) ;
#4283=DIRECTION ( 'NONE',  ( 1.000000000000000000, 0.000000000000000000, -0.000000000000000000 ) ) ;
#4287=CARTESIAN_POINT ( 'NONE',  ( 780.5290396650775619, -84.35105083532374692, -365.2837595273619513 ) ) ;
#4288=FACE_OUTER_BOUND ( 'NONE', #809, .T. ) ;
#4289=CARTESIAN_POINT ( 'NONE',  ( 745.0891759886404770, -148.2709662947837330, -342.4968714119734159 ) ) ;
#4291=CARTESIAN_POINT ( 'NONE',  ( 767.8955696845334842, -144.4527844766018632, -362.1676090361161755 ) ) ;
#4294=CARTESIAN_POINT ( 'NONE',  ( 802.5472867521000353, -436.3726999360612240, -350.8726784830461156 ) ) ;
#4301=CARTESIAN_POINT ( 'NONE',  ( 783.0745993439762742, -392.1908817542432075, -365.1016975059196739 ) ) ;
#4303=CARTESIAN_POINT ( 'NONE',  ( 810.4231160770870019, -168.5545181178802352, -321.9338519418446936 ) ) ;
#4305=CARTESIAN_POINT ( 'NONE',  ( 799.9999999999993179, 166.4563064324884465, -319.9999999999999432 ) ) ;
#4306=CARTESIAN_POINT ( 'NONE',  ( 799.4546378042377910, -321.0783235625956991, -356.1575198192848006 ) ) ;
#4308=CARTESIAN_POINT ( 'NONE',  ( 762.1177392798416577, -186.5545181178801215, -309.8865473780659272 ) ) ;
#4313=CARTESIAN_POINT ( 'NONE',  ( 801.1904061080338124, -212.0891481129653187, -368.3070685750236066 ) ) ;
#4315=CARTESIAN_POINT ( 'NONE',  ( 803.4237431249931660, -15.18005720387504631, -331.2633955100225194 ) ) ;
#4317=CARTESIAN_POINT ( 'NONE',  ( 814.8230680027162407, -101.8055962898691718, -333.7305795820267917 ) ) ;
#4319=CARTESIAN_POINT ( 'NONE',  ( 796.9462024416508257, -324.4527844766013231, -308.9653473494370246 ) ) ;
#4325=CARTESIAN_POINT ( 'NONE',  ( 803.8556311672234642, -417.6237781080499190, -365.6418435158340117 ) ) ;
#4327=CARTESIAN_POINT ( 'NONE',  ( 815.2698199232961542, -424.8164208402372992, -342.5225473063383106 ) ) ;
#4332=CARTESIAN_POINT ( 'NONE',  ( 801.3366627262608972, -176.5328690171416213, -353.0897708529566899 ) ) ;
#4334=CARTESIAN_POINT ( 'NONE',  ( 754.0944755984390895, -183.6237781080507148, -364.1009440267246760 ) ) ;
#4340=CARTESIAN_POINT ( 'NONE',  ( 814.2001403089898304, -41.36187538569314626, -347.4397851343538264 ) ) ;
#4342=CARTESIAN_POINT ( 'NONE',  ( 755.8990559732751535, -443.4636090269702322, -365.9055244015606831 ) ) ;
#4348=CARTESIAN_POINT ( 'NONE',  ( 792.1044303154645831, -300.4527844766012663, -317.8323909638837677 ) ) ;
#4352=EDGE_CURVE ( 'NONE', #30163, #19609, #2865, .T. ) ;
#4353=CARTESIAN_POINT ( 'NONE',  ( 761.4292242960306112, -305.4636090269706870, -323.2154366446414429 ) ) ;
#4354=CARTESIAN_POINT ( 'NONE',  ( 771.2633955100217236, -287.9073299311468759, -363.4237431249939618 ) ) ;
#4356=CARTESIAN_POINT ( 'NONE',  ( 774.6858677611749044, -129.7255117493292289, -315.5713283507209894 ) ) ;
#4359=CIRCLE ( 'NONE', #27193, 4.999999999999982236 ) ;
#4362=CARTESIAN_POINT ( 'NONE',  ( 799.9636004259356241, -70.91815448151683654, -311.2241431872006956 ) ) ;
#4363=CARTESIAN_POINT ( 'NONE',  ( 799.9999999999993179, -512.9681489794448908, -339.9999999999999432 ) ) ;
#4368=CARTESIAN_POINT ( 'NONE',  ( 759.0252816721024374, -120.9982390220565378, -368.0189434323527280 ) ) ;
#4370=CARTESIAN_POINT ( 'NONE',  ( 789.5670355615794733, -453.0432664090020012, -363.0970091259334822 ) ) ;
#4371=EDGE_CURVE ( 'NONE', #30631, #35503, #14730, .T. ) ;
#4373=CARTESIAN_POINT ( 'NONE',  ( 792.3570229623688874, -237.1800572038742985, -373.1304606946836202 ) ) ;
#4377=CARTESIAN_POINT ( 'NONE',  ( 771.2368401574024119, -301.4419599262320730, -374.2805881961240857 ) ) ;
#4379=CARTESIAN_POINT ( 'NONE',  ( 815.2698199232961542, -328.8164208402375834, -342.5225473063383106 ) ) ;
#4384=CARTESIAN_POINT ( 'NONE',  ( 785.3687786644884454, -419.3618753856918033, -315.3201227861279676 ) ) ;
#4387=CARTESIAN_POINT ( 'NONE',  ( 795.6651683502461765, -82.71468719896012090, -371.3240766477733814 ) ) ;
#4388=LINE ( 'NONE', #28217, #21097 ) ;
#4393=CARTESIAN_POINT ( 'NONE',  ( 761.2382568024794409, -231.6237781080504874, -356.9571628226838129 ) ) ;
#4395=CARTESIAN_POINT ( 'NONE',  ( 815.1787889125755555, -78.89650538077832209, -343.7953271457877804 ) ) ;
#4400=CARTESIAN_POINT ( 'NONE',  ( 786.2694204179717872, -333.2817908451523863, -305.1769319972829067 ) ) ;
#4404=CARTESIAN_POINT ( 'NONE',  ( 790.9844846989617508, -190.3726999360619629, -317.2208543904092721 ) ) ;
#4405=CARTESIAN_POINT ( 'NONE',  ( 781.8018195045266339, -166.2709662947835909, -365.1927285166406705 ) ) ;
#4406=CARTESIAN_POINT ( 'NONE',  ( 805.1927285166399315, -376.8164208402375834, -341.8018195045277707 ) ) ;
#4416=CARTESIAN_POINT ( 'NONE',  ( 788.6739635108323228, -415.6454272087885897, -373.9316612368139090 ) ) ;
#4418=CARTESIAN_POINT ( 'NONE',  ( 772.5602148656447525, -9.725511749329603717, -305.7998596910095443 ) ) ;
#4422=CARTESIAN_POINT ( 'NONE',  ( 797.8594530101008786, -373.5436935675101040, -322.1405469898980982 ) ) ;
#4424=EDGE_CURVE ( 'NONE', #12399, #24210, #3389, .T. ) ;
#4426=CARTESIAN_POINT ( 'NONE',  ( 772.4999999999993179, -462.9681489794447771, -310.9526249034443026 ) ) ;
#4427=CARTESIAN_POINT ( 'NONE',  ( 804.6971507214547046, -243.2817908451526705, -344.0799538623459739 ) ) ;
#4437=CARTESIAN_POINT ( 'NONE',  ( 795.1360043628807261, -308.0891481129650629, -360.2193346964456282 ) ) ;
#4442=CARTESIAN_POINT ( 'NONE',  ( 797.8822607201568644, -54.55451811788054783, -370.1134526219340160 ) ) ;
#4443=CARTESIAN_POINT ( 'NONE',  ( 775.9200461376533440, -119.8055962898690865, -315.3028492785443291 ) ) ;
#4446=CARTESIAN_POINT ( 'NONE',  ( 764.8639956371174549, -8.089148112965974136, -319.7806653035542013 ) ) ;
#4447=CARTESIAN_POINT ( 'NONE',  ( 783.0433043558608688, -144.8965053807781089, -315.1538015810313027 ) ) ;
#4449=CARTESIAN_POINT ( 'NONE',  ( 800.0135310231082713, -110.0891481129656597, -325.0180583372163028 ) ) ;
#4450=CARTESIAN_POINT ( 'NONE',  ( 755.0488828828309806, -401.8055962898681059, -344.1219089521771934 ) ) ;
#4456=ORIENTED_EDGE ( 'NONE', *, *, #28091, .T. ) ;
#4460=CARTESIAN_POINT ( 'NONE',  ( 787.5531968255692163, -69.82724539060775726, -316.1348686366205811 ) ) ;
#4462=CARTESIAN_POINT ( 'NONE',  ( 785.3141322388236176, -261.7255117493288026, -364.4286716492789537 ) ) ;
#4464=CARTESIAN_POINT ( 'NONE',  ( 802.1676090361156639, -398.6346026584193396, -327.8955696845344505 ) ) ;
#4465=CARTESIAN_POINT ( 'NONE',  ( 785.3141322388236176, -45.72551174932949181, -364.4286716492789537 ) ) ;
#4469=CARTESIAN_POINT ( 'NONE',  ( 755.5713283507202505, -5.361875385693257279, -334.6858677611754729 ) ) ;
#4472=CARTESIAN_POINT ( 'NONE',  ( 793.5525998758768083, -295.0999726633343698, -372.6845335610516941 ) ) ;
#4475=CARTESIAN_POINT ( 'NONE',  ( 755.3201227861273992, -243.7255117493287742, -345.3687786644892981 ) ) ;
#4477=CARTESIAN_POINT ( 'NONE',  ( 804.8461984189677878, -146.1908817542438896, -336.9566956441385628 ) ) ;
#4480=CARTESIAN_POINT ( 'NONE',  ( 756.1443688327750579, -21.62377810805121570, -314.3581564841659315 ) ) ;
#4481=CARTESIAN_POINT ( 'NONE',  ( 801.1904061080338124, -356.0891481129648355, -368.3070685750236066 ) ) ;
#4482=DIRECTION ( 'NONE',  ( 0.9164815115825537539, 0.1263042864341373805, 0.3796167358741193709 ) ) ;
#4485=CARTESIAN_POINT ( 'NONE',  ( 811.6461892240364477, -244.7146871989596093, -324.1737431748509835 ) ) ;
#4487=CARTESIAN_POINT ( 'NONE',  ( 752.4576283171824116, -429.0783235625953580, -317.7880784355627952 ) ) ;
#4492=CARTESIAN_POINT ( 'NONE',  ( 793.2243759319678702, 21.46713098285774279, -318.4439275373583200 ) ) ;
#4498=CARTESIAN_POINT ( 'NONE',  ( 756.7813123517142913, -307.9874144716866340, -329.9779781133712504 ) ) ;
#4500=CARTESIAN_POINT ( 'NONE',  ( 800.1688906516307043, -346.1692326535047641, -369.0717654672308186 ) ) ;
#4505=CARTESIAN_POINT ( 'NONE',  ( 764.0069404352550464, -87.07832356259646645, -359.2566176426627180 ) ) ;
#4506=DIRECTION ( 'NONE',  ( -0.000000000000000000, 1.000000000000000000, -0.000000000000000000 ) ) ;
#4507=CARTESIAN_POINT ( 'NONE',  ( 782.5225473063381969, -142.2709662947837330, -375.2698199232970637 ) ) ;
#4509=CARTESIAN_POINT ( 'NONE',  ( 803.4237431249931660, -159.1800572038746111, -331.2633955100225194 ) ) ;
#4511=CARTESIAN_POINT ( 'NONE',  ( 804.8461984189677878, -434.1908817542430370, -336.9566956441385628 ) ) ;
#4516=CARTESIAN_POINT ( 'NONE',  ( 779.9999999999992042, -462.9681489794448339, -339.9999999999999432 ) ) ;
#4519=CARTESIAN_POINT ( 'NONE',  ( 804.4086373105744769, -409.6454272087884760, -333.3843516231986541 ) ) ;
#4520=CARTESIAN_POINT ( 'NONE',  ( 799.9999999999993179, 205.0000000000000568, -329.9999999999999432 ) ) ;
#4521=CARTESIAN_POINT ( 'NONE',  ( 778.7629533639073998, -200.7363362996982801, -375.0009284576466371 ) ) ;
#4525=CARTESIAN_POINT ( 'NONE',  ( 804.1601925771018387, -319.4419599262320730, -346.5483106153029098 ) ) ;
#4527=CARTESIAN_POINT ( 'NONE',  ( 781.2370466360911223, -188.7363362996983085, -304.9990715423533629 ) ) ;
#4531=CARTESIAN_POINT ( 'NONE',  ( 814.9108240113580450, -232.2709662947834488, -337.5031285880265273 ) ) ;
#4533=CARTESIAN_POINT ( 'NONE',  ( 803.6646147819161570, -17.90732993114776406, -348.8264449731210561 ) ) ;
#4535=CARTESIAN_POINT ( 'NONE',  ( 800.1688906516307043, -106.1692326535054889, -369.0717654672308186 ) ) ;
#4537=CARTESIAN_POINT ( 'NONE',  ( 814.2001403089898304, -377.3618753856920875, -347.4397851343538264 ) ) ;
#4542=CARTESIAN_POINT ( 'NONE',  ( 771.2368401574024119, -397.4419599262317320, -374.2805881961240857 ) ) ;
#4543=CARTESIAN_POINT ( 'NONE',  ( 815.2698199232961542, -448.8164208402371855, -342.5225473063383106 ) ) ;
#4547=CARTESIAN_POINT ( 'NONE',  ( 804.9511171171677688, -197.8055962898688733, -335.8780910478229202 ) ) ;
#4550=CARTESIAN_POINT ( 'NONE',  ( 758.0141637701419768, -183.0783235625961538, -367.2620300519063790 ) ) ;
#4554=CARTESIAN_POINT ( 'NONE',  ( 768.0187753319979720, -80.63460265842029173, -318.0580252608186242 ) ) ;
#4557=CARTESIAN_POINT ( 'NONE',  ( 755.3201227861273992, -147.7255117493291152, -345.3687786644892981 ) ) ;
#4559=CARTESIAN_POINT ( 'NONE',  ( 755.2512626584698410, -55.54369356751127640, -315.2512626584710915 ) ) ;
#4561=CARTESIAN_POINT ( 'NONE',  ( 771.3260364891663130, -451.6454272087884192, -306.0683387631859773 ) ) ;
#4562=ORIENTED_EDGE ( 'NONE', *, *, #23842, .T. ) ;
#4563=CARTESIAN_POINT ( 'NONE',  ( 793.0897708529556667, -318.5545181178796952, -361.3366627262616362 ) ) ;
#4566=CARTESIAN_POINT ( 'NONE',  ( 785.3687786644884454, -299.3618753856922581, -315.3201227861279676 ) ) ;
#4569=CARTESIAN_POINT ( 'NONE',  ( 755.3028492785439312, -279.2817908451526137, -335.9200461376539693 ) ) ;
#4570=CARTESIAN_POINT ( 'NONE',  ( 804.4286716492782716, -281.3618753856923718, -345.3141322388244703 ) ) ;
#4572=CARTESIAN_POINT ( 'NONE',  ( 771.2633955100217236, -167.9073299311473022, -363.4237431249939618 ) ) ;
#4576=LINE ( 'NONE', #32529, #15283 ) ;
#4578=CARTESIAN_POINT ( 'NONE',  ( 766.4474001241216001, -91.09997266333496668, -307.3154664389482491 ) ) ;
#4585=CARTESIAN_POINT ( 'NONE',  ( 745.7998596910086917, -125.3618753856928834, -332.5602148656461168 ) ) ;
#4589=CARTESIAN_POINT ( 'NONE',  ( 814.2001403089898304, -281.3618753856923718, -347.4397851343538264 ) ) ;
#4591=CARTESIAN_POINT ( 'NONE',  ( 749.8865473780648472, -308.5328690171412518, -322.1177392798429082 ) ) ;
#4593=CARTESIAN_POINT ( 'NONE',  ( 787.4397851343537695, -357.7255117493285184, -374.2001403089903988 ) ) ;
#4594=CARTESIAN_POINT ( 'NONE',  ( 759.9999999999992042, -512.9681489794448908, -329.9999999999999432 ) ) ;
#4597=CARTESIAN_POINT ( 'NONE',  ( 794.9819416627830151, -420.9982390220555999, -319.9864689768909898 ) ) ;
#4598=CARTESIAN_POINT ( 'NONE',  ( 792.1044303154645831, -228.4527844766015789, -317.8323909638837677 ) ) ;
#4599=CARTESIAN_POINT ( 'NONE',  ( 766.5853460496234675, -85.98741447168738716, -372.3518521366060554 ) ) ;
#4603=CARTESIAN_POINT ( 'NONE',  ( 786.6156483768007774, -241.4419599262322720, -315.5913626894246136 ) ) ;
#4605=CARTESIAN_POINT ( 'NONE',  ( 815.0009284576459549, -78.35105083532376113, -338.7629533639073429 ) ) ;
#4606=CARTESIAN_POINT ( 'NONE',  ( 809.2691622578233819, -452.9681489794448908, -335.3267997378328005 ) ) ;
#4608=CARTESIAN_POINT ( 'NONE',  ( 783.7953271457878373, -344.1908817542433212, -375.1787889125761239 ) ) ;
#4610=ADVANCED_FACE ( 'NONE', ( #4004 ), #6555, .T. ) ;
#4612=CARTESIAN_POINT ( 'NONE',  ( 760.7433823573367135, -180.0090635724255890, -355.9930595647440441 ) ) ;
#4613=CARTESIAN_POINT ( 'NONE',  ( 758.0580252608178853, -174.4527844766018063, -328.0187753319985404 ) ) ;
#4614=CARTESIAN_POINT ( 'NONE',  ( 803.4237431249931660, -375.1800572038739574, -331.2633955100225194 ) ) ;
#4616=CARTESIAN_POINT ( 'NONE',  ( 783.0433043558608688, 23.10349461922137237, -315.1538015810313027 ) ) ;
#4619=FACE_OUTER_BOUND ( 'NONE', #21389, .T. ) ;
#4628=CARTESIAN_POINT ( 'NONE',  ( 766.4474001241216001, -403.0999726633339719, -307.3154664389482491 ) ) ;
#4630=CARTESIAN_POINT ( 'NONE',  ( 746.8695393053151292, -5.907329931147799584, -327.6429770376306578 ) ) ;
#4633=CARTESIAN_POINT ( 'NONE',  ( 778.2165204200184689, -406.8164208402375266, -364.9363028652563230 ) ) ;
#4637=CARTESIAN_POINT ( 'NONE',  ( 769.0155153010367712, -250.3726999360618208, -362.7791456095907279 ) ) ;
#4648=CARTESIAN_POINT ( 'NONE',  ( 803.4237431249931660, -303.1800572038740711, -331.2633955100225194 ) ) ;
#4651=CARTESIAN_POINT ( 'NONE',  ( 793.5525998758768083, -79.09997266333503774, -372.6845335610516941 ) ) ;
#4652=CARTESIAN_POINT ( 'NONE',  ( 803.8651313633788504, -125.2601417444145255, -332.4468031744301015 ) ) ;
#4655=CARTESIAN_POINT ( 'NONE',  ( 802.1676090361156639, -38.63460265842041252, -327.8955696845344505 ) ) ;
#4656=CARTESIAN_POINT ( 'NONE',  ( 760.5453621957607311, -141.0783235625962959, -323.8424801807151425 ) ) ;
#4657=CARTESIAN_POINT ( 'NONE',  ( 804.4286716492782716, -113.3618753856929260, -345.3141322388244703 ) ) ;
#4658=CARTESIAN_POINT ( 'NONE',  ( 780.5290396650775619, -420.3510508353225532, -365.2837595273619513 ) ) ;
#4673=CARTESIAN_POINT ( 'NONE',  ( 757.4527132478984868, -88.37269993606226137, -329.1273215169538844 ) ) ;
#4675=CARTESIAN_POINT ( 'NONE',  ( 762.1405469898973024, -265.5436935675106156, -357.8594530101016176 ) ) ;
#4677=CARTESIAN_POINT ( 'NONE',  ( 788.8264449731200330, -405.1800572038737300, -363.6646147819171233 ) ) ;
#4678=CARTESIAN_POINT ( 'NONE',  ( 804.9363028652555840, -40.27096629478405987, -338.2165204200192079 ) ) ;
#4679=VECTOR ( 'NONE', #30619, 1000.000000000000000 ) ;
#4683=EDGE_CURVE ( 'NONE', #30422, #8509, #29098, .T. ) ;
#4684=CARTESIAN_POINT ( 'NONE',  ( 814.2805881961230625, -25.64542720878973014, -331.2368401574024119 ) ) ;
#4687=CARTESIAN_POINT ( 'NONE',  ( 814.4686193811664907, -315.2817908451525000, -346.2056067578752732 ) ) ;
#4690=CARTESIAN_POINT ( 'NONE',  ( 803.6646147819161570, -257.9073299311469896, -348.8264449731210561 ) ) ;
#4692=CARTESIAN_POINT ( 'NONE',  ( 796.9571628226829034, -143.4636090269711701, -321.2382568024804641 ) ) ;
#4694=CARTESIAN_POINT ( 'NONE',  ( 787.4397851343537695, -357.7255117493285184, -374.2001403089903988 ) ) ;
#4699=CARTESIAN_POINT ( 'NONE',  ( 764.3348316497523456, -238.7146871989596661, -308.6759233522265617 ) ) ;
#4701=CARTESIAN_POINT ( 'NONE',  ( 758.8095938919642549, 15.91085188703394238, -311.6929314249763365 ) ) ;
#4702=DIRECTION ( 'NONE',  ( 0.000000000000000000, -1.000000000000000000, 0.000000000000000000 ) ) ;
#4706=CARTESIAN_POINT ( 'NONE',  ( 765.8855110935204493, -22.16923265350575889, -319.0159684113471599 ) ) ;
#4712=ORIENTED_EDGE ( 'NONE', *, *, #26956, .T. ) ;
#4713=CARTESIAN_POINT ( 'NONE',  ( 794.9819416627830151, -36.99823902205679360, -319.9864689768909898 ) ) ;
#4714=CARTESIAN_POINT ( 'NONE',  ( 763.2154366446407039, -333.6237781080502600, -321.4292242960311228 ) ) ;
#4716=CARTESIAN_POINT ( 'NONE',  ( 744.8212110874229666, -330.8965053807774552, -336.2046728542121627 ) ) ;
#4717=LINE ( 'NONE', #32913, #7931 ) ;
#4723=CARTESIAN_POINT ( 'NONE',  ( 760.5453621957607311, -69.07832356259653750, -323.8424801807151425 ) ) ;
#4726=CARTESIAN_POINT ( 'NONE',  ( 747.2067596250078623, -171.1800572038745543, -352.2312462859687230 ) ) ;
#4729=CARTESIAN_POINT ( 'NONE',  ( 792.1044303154646968, -180.4527844766017495, -317.8323909638837677 ) ) ;
#4732=CARTESIAN_POINT ( 'NONE',  ( 793.9708237608222134, -430.9181544815157849, -319.2295555964448681 ) ) ;
#4739=CARTESIAN_POINT ( 'NONE',  ( 758.4439275373578084, -444.5545181178792973, -353.2243759319684386 ) ) ;
#4741=CARTESIAN_POINT ( 'NONE',  ( 768.9521613784389729, -201.8272453906073451, -373.2346286133773106 ) ) ;
#4745=CARTESIAN_POINT ( 'NONE',  ( 793.2243759319678702, -314.5328690171411949, -318.4439275373583200 ) ) ;
#4747=CARTESIAN_POINT ( 'NONE',  ( 744.6391490659812007, -182.7363362996983369, -338.7502325331110455 ) ) ;
#4752=CARTESIAN_POINT ( 'NONE',  ( 815.2698199232962679, -256.8164208402379245, -342.5225473063383674 ) ) ;
#4755=CARTESIAN_POINT ( 'NONE',  ( 785.3141322388236176, -21.72551174932956641, -364.4286716492789537 ) ) ;
#4757=CARTESIAN_POINT ( 'NONE',  ( 749.8865473780648472, -116.5328690171418202, -322.1177392798429082 ) ) ;
#4759=CARTESIAN_POINT ( 'NONE',  ( 758.8095938919642549, -368.0891481129647786, -311.6929314249763365 ) ) ;
#4765=CARTESIAN_POINT ( 'NONE',  ( 762.3223304703356007, -391.5436935675101608, -322.3223304703362828 ) ) ;
#4766=CARTESIAN_POINT ( 'NONE',  ( 815.3608509340175488, -2.736336299698892027, -341.2497674668889545 ) ) ;
#4769=ORIENTED_EDGE ( 'NONE', *, *, #9705, .F. ) ;
#4770=CARTESIAN_POINT ( 'NONE',  ( 770.0799878456142551, -205.9874144716870035, -362.9823548866085616 ) ) ;
#4772=CARTESIAN_POINT ( 'NONE',  ( 815.1787889125755555, -222.8965053807778531, -343.7953271457877804 ) ) ;
#4775=CARTESIAN_POINT ( 'NONE',  ( 797.8594530101008786, -85.54369356751118403, -322.1405469898980982 ) ) ;
#4781=CARTESIAN_POINT ( 'NONE',  ( 801.1904061080336987, -92.08914811296568814, -368.3070685750235498 ) ) ;
#4782=ADVANCED_FACE ( 'NONE', ( #3778 ), #11166, .T. ) ;
#4784=CARTESIAN_POINT ( 'NONE',  ( 759.0159684113467620, -16.91815448151702839, -325.8855110935213020 ) ) ;
#4786=CARTESIAN_POINT ( 'NONE',  ( 804.4086373105744769, -313.6454272087888171, -333.3843516231986541 ) ) ;
#4789=CARTESIAN_POINT ( 'NONE',  ( 781.8018195045266339, -334.2709662947829656, -365.1927285166406705 ) ) ;
#4793=CARTESIAN_POINT ( 'NONE',  ( 804.8461984189677878, -290.1908817542434349, -336.9566956441385628 ) ) ;
#4794=CARTESIAN_POINT ( 'NONE',  ( 781.7834795799800531, -298.8164208402377540, -315.0636971347436202 ) ) ;
#4796=CARTESIAN_POINT ( 'NONE',  ( 767.8955696845333705, -144.4527844766018632, -362.1676090361162323 ) ) ;
#4802=CARTESIAN_POINT ( 'NONE',  ( 804.1009440267234822, -95.46360902697132644, -314.0944755984392600 ) ) ;
#4807=ORIENTED_EDGE ( 'NONE', *, *, #43927, .F. ) ;
#4808=CIRCLE ( 'NONE', #34301, 30.00000000000008171 ) ;
#4809=CARTESIAN_POINT ( 'NONE',  ( 767.6429770376291799, -129.1800572038746679, -306.8695393053162093 ) ) ;
#4814=CARTESIAN_POINT ( 'NONE',  ( 745.0891759886404770, -268.2709662947833067, -342.4968714119734159 ) ) ;
#4820=CARTESIAN_POINT ( 'NONE',  ( 783.7566961878529810, -312.8965053807775689, -305.1792804349288417 ) ) ;
#4822=CARTESIAN_POINT ( 'NONE',  ( 810.7187646348534145, -354.4527844766012095, -356.7737145352016341 ) ) ;
#4826=CARTESIAN_POINT ( 'NONE',  ( 803.4237431249931660, -423.1800572038737300, -331.2633955100225194 ) ) ;
#4828=CARTESIAN_POINT ( 'NONE',  ( 793.4146539503750546, -121.9874144716872593, -307.6481478633938877 ) ) ;
#4832=CARTESIAN_POINT ( 'NONE',  ( 755.8398074228967971, -235.4419599262323857, -333.4516893846970333 ) ) ;
#4835=CARTESIAN_POINT ( 'NONE',  ( 786.2056067578752163, -59.80559628986927834, -374.4686193811670023 ) ) ;
#4836=CARTESIAN_POINT ( 'NONE',  ( 808.2983282543862060, -452.9681489794448908, -337.2950253338145785 ) ) ;
#4838=ORIENTED_EDGE ( 'NONE', *, *, #29496, .T. ) ;
#4840=CARTESIAN_POINT ( 'NONE',  ( 744.6391490659812007, -326.7363362996979390, -338.7502325331110455 ) ) ;
#4846=CARTESIAN_POINT ( 'NONE',  ( 796.1575198192839480, -198.0090635724255606, -359.4546378042384163 ) ) ;
#4847=CARTESIAN_POINT ( 'NONE',  ( 764.8639956371174549, -200.0891481129653187, -319.7806653035542013 ) ) ;
#4848=CARTESIAN_POINT ( 'NONE',  ( 774.6858677611749044, -393.7255117493283478, -315.5713283507209894 ) ) ;
#4850=CARTESIAN_POINT ( 'NONE',  ( 795.9930595647434757, 20.92167643740319605, -320.7433823573372820 ) ) ;
#4858=CARTESIAN_POINT ( 'NONE',  ( 781.2370466360911223, -428.7363362996975980, -304.9990715423533629 ) ) ;
#4859=CARTESIAN_POINT ( 'NONE',  ( 767.7687537140311633, -23.90732993114773919, -372.7932403749916830 ) ) ;
#4862=CARTESIAN_POINT ( 'NONE',  ( 800.0135310231082713, -398.0891481129647218, -325.0180583372163028 ) ) ;
#4863=CARTESIAN_POINT ( 'NONE',  ( 792.1044303154646968, -12.45278447660232324, -317.8323909638837677 ) ) ;
#4866=CARTESIAN_POINT ( 'NONE',  ( 796.9571628226829034, -239.4636090269709143, -321.2382568024804641 ) ) ;
#4867=CARTESIAN_POINT ( 'NONE',  ( 767.7687537140311633, -167.9073299311473022, -372.7932403749916830 ) ) ;
#4870=CARTESIAN_POINT ( 'NONE',  ( 794.9298647675502707, 16.45630643248849978, -314.4833286358118016 ) ) ;
#4876=CARTESIAN_POINT ( 'NONE',  ( 805.1927285166397041, -304.8164208402376403, -341.8018195045277707 ) ) ;
#4879=CARTESIAN_POINT ( 'NONE',  ( 813.5763878283155464, -99.82724539060768620, -351.1614460488615350 ) ) ;
#4880=CARTESIAN_POINT ( 'NONE',  ( 764.0069404352550464, -111.0783235625964096, -359.2566176426627180 ) ) ;
#4883=CARTESIAN_POINT ( 'NONE',  ( 759.7806653035534055, -30.99823902205680071, -324.8639956371180801 ) ) ;
#4884=CARTESIAN_POINT ( 'NONE',  ( 800.7704444035546203, -124.1692326535054463, -326.0291762391768771 ) ) ;
#4885=CARTESIAN_POINT ( 'NONE',  ( 774.6312213355099630, -143.3618753856927697, -364.6798772138717482 ) ) ;
#4888=CARTESIAN_POINT ( 'NONE',  ( 801.9858362298568863, 20.92167643740319605, -312.7379699480935642 ) ) ;
#4902=CARTESIAN_POINT ( 'NONE',  ( 796.9571628226829034, -95.46360902697132644, -321.2382568024804641 ) ) ;
#4903=CARTESIAN_POINT ( 'NONE',  ( 759.7806653035535192, -270.9982390220561115, -324.8639956371181370 ) ) ;
#4904=ORIENTED_EDGE ( 'NONE', *, *, #19574, .F. ) ;
#4905=CARTESIAN_POINT ( 'NONE',  ( 804.9363028652555840, -400.2709662947828519, -338.2165204200192079 ) ) ;
#4906=CARTESIAN_POINT ( 'NONE',  ( 768.0187753319979720, -32.63460265842044095, -318.0580252608186242 ) ) ;
#4907=ADVANCED_FACE ( 'NONE', ( #28024 ), #22684, .T. ) ;
#4912=CARTESIAN_POINT ( 'NONE',  ( 815.3608509340175488, -26.73633629969882008, -341.2497674668889545 ) ) ;
#4915=CARTESIAN_POINT ( 'NONE',  ( 755.8990559732751535, -323.4636090269706301, -365.9055244015606831 ) ) ;
#4918=CARTESIAN_POINT ( 'NONE',  ( 800.0135310231082713, -302.0891481129650629, -325.0180583372163028 ) ) ;
#4920=CARTESIAN_POINT ( 'NONE',  ( 793.9708237608222134, -142.9181544815166376, -319.2295555964448681 ) ) ;
#4923=CARTESIAN_POINT ( 'NONE',  ( 813.2346286133761168, -5.260141744414903897, -328.9521613784389160 ) ) ;
#4924=CARTESIAN_POINT ( 'NONE',  ( 744.7301800767020268, -340.8164208402376403, -337.4774526936615189 ) ) ;
#4929=CARTESIAN_POINT ( 'NONE',  ( 795.6651683502461765, -250.7146871989595809, -371.3240766477733814 ) ) ;
#4931=CARTESIAN_POINT ( 'NONE',  ( 800.1688906516307043, -442.1692326535044231, -369.0717654672308186 ) ) ;
#4938=CARTESIAN_POINT ( 'NONE',  ( 803.2186876482843445, -31.98741447168754348, -350.0220218866286928 ) ) ;
#4944=CARTESIAN_POINT ( 'NONE',  ( 800.2193346964447755, -42.99823902205675807, -355.1360043628815788 ) ) ;
#4948=CARTESIAN_POINT ( 'NONE',  ( 786.6156483768007774, -313.4419599262320730, -315.5913626894246136 ) ) ;
#4950=CARTESIAN_POINT ( 'NONE',  ( 805.9055244015594326, -339.6237781080502600, -315.8990559732753240 ) ) ;
#4954=CARTESIAN_POINT ( 'NONE',  ( 759.2295555964440155, -88.16923265350555994, -353.9708237608231229 ) ) ;
#4957=CARTESIAN_POINT ( 'NONE',  ( 754.9967657858570647, -193.5436935675108714, -365.0032342141425374 ) ) ;
#4960=CARTESIAN_POINT ( 'NONE',  ( 791.9812246680005501, -188.6346026584199365, -361.9419747391813189 ) ) ;
#4963=CARTESIAN_POINT ( 'NONE',  ( 796.1575198192839480, -414.0090635724249637, -359.4546378042384163 ) ) ;
#4970=CARTESIAN_POINT ( 'NONE',  ( 804.1105419155481968, -435.8272453906066062, -347.6308680596136469 ) ) ;
#4972=CARTESIAN_POINT ( 'NONE',  ( 776.2046728542105711, -212.1908817542436623, -304.8212110874238761 ) ) ;
#4976=CARTESIAN_POINT ( 'NONE',  ( 771.1735550268778070, -201.1800572038744690, -316.3353852180827630 ) ) ;
#4977=CARTESIAN_POINT ( 'NONE',  ( 765.8855110935204493, -334.1692326535047073, -319.0159684113471599 ) ) ;
#4979=CARTESIAN_POINT ( 'NONE',  ( 786.2694204179717872, -213.2817908451527842, -305.1769319972829067 ) ) ;
#4982=CARTESIAN_POINT ( 'NONE',  ( 805.2837595273609850, -50.73633629969874193, -340.5290396650784714 ) ) ;
#4984=CARTESIAN_POINT ( 'NONE',  ( 749.2812353651451076, -246.4527844766016074, -323.2262854647983090 ) ) ;
#4987=CARTESIAN_POINT ( 'NONE',  ( 800.0135310231082713, -14.08914811296595460, -325.0180583372163028 ) ) ;
#4990=CARTESIAN_POINT ( 'NONE',  ( 773.7943932421234194, -119.8055962898690865, -305.5313806188329409 ) ) ;
#4992=CARTESIAN_POINT ( 'NONE',  ( 805.0032342141412300, -373.5436935675101040, -314.9967657858571783 ) ) ;
#4993=DIRECTION ( 'NONE',  ( 0.000000000000000000, 1.000000000000000000, 0.000000000000000000 ) ) ;
#4994=DIRECTION ( 'NONE',  ( 1.000000000000000000, 0.000000000000000000, 0.000000000000000000 ) ) ;
#4998=CARTESIAN_POINT ( 'NONE',  ( 781.7834795799800531, -394.8164208402374697, -315.0636971347436202 ) ) ;
#4999=( BOUNDED_CURVE ( )  B_SPLINE_CURVE ( 3, ( #44055, #30196, #26957, #16336 ),
 .UNSPECIFIED., .F., .T. ) 
 B_SPLINE_CURVE_WITH_KNOTS ( ( 4, 4 ),
 ( 4.712388980384714543, 4.733441231200429478 ),
 .UNSPECIFIED. ) 
 CURVE ( )  GEOMETRIC_REPRESENTATION_ITEM ( )  RATIONAL_B_SPLINE_CURVE ( ( 1.000000000000000000, 0.9999630672356449868, 0.9999630672356449868, 1.000000000000000000 ) ) 
 REPRESENTATION_ITEM ( '' )  );
#5000=CARTESIAN_POINT ( 'NONE',  ( 760.0363995740630116, -10.91815448151704793, -368.7758568127991907 ) ) ;
#5001=CARTESIAN_POINT ( 'NONE',  ( 793.3938497862117174, -453.0432664090020580, -372.3358127763067955 ) ) ;
#5006=CARTESIAN_POINT ( 'NONE',  ( 770.0799878456142551, -229.9874144716869466, -362.9823548866085616 ) ) ;
#5008=CARTESIAN_POINT ( 'NONE',  ( 795.6651683502461765, -226.7146871989596661, -371.3240766477733814 ) ) ;
#5014=CARTESIAN_POINT ( 'NONE',  ( 804.9363028652555840, -136.2709662947837330, -338.2165204200192079 ) ) ;
#5016=CARTESIAN_POINT ( 'NONE',  ( 746.8695393053150156, -77.90732993114757221, -327.6429770376306010 ) ) ;
#5017=CARTESIAN_POINT ( 'NONE',  ( 804.6798772138710092, -87.72551174932935680, -334.6312213355106451 ) ) ;
#5019=CARTESIAN_POINT ( 'NONE',  ( 779.4763451958990572, -8.736336299698871599, -365.0264073115438919 ) ) ;
#5020=VERTEX_POINT ( 'NONE', #29176 ) ;
#5021=CARTESIAN_POINT ( 'NONE',  ( 783.0745993439762742, -320.1908817542434349, -365.1016975059196739 ) ) ;
#5029=CARTESIAN_POINT ( 'NONE',  ( 772.4468031744293057, -321.8272453906070609, -363.8651313633793620 ) ) ;
#5030=CARTESIAN_POINT ( 'NONE',  ( 774.6858677611749044, -273.7255117493288026, -315.5713283507209894 ) ) ;
#5031=CARTESIAN_POINT ( 'NONE',  ( 800.0135310231082713, -158.0891481129655176, -325.0180583372163028 ) ) ;
#5035=CARTESIAN_POINT ( 'NONE',  ( 745.7194118038753459, -109.6454272087894566, -348.7631598425976449 ) ) ;
#5040=CARTESIAN_POINT ( 'NONE',  ( 812.7932403749906598, -135.1800572038746679, -327.7687537140311633 ) ) ;
#5044=CARTESIAN_POINT ( 'NONE',  ( 800.9747183278959710, -276.9982390220559978, -311.9810565676471583 ) ) ;
#5045=CARTESIAN_POINT ( 'NONE',  ( 805.0032342141413437, -445.5436935675099335, -314.9967657858572352 ) ) ;
#5048=CARTESIAN_POINT ( 'NONE',  ( 758.0141637701419768, -327.0783235625956991, -367.2620300519063790 ) ) ;
#5049=CARTESIAN_POINT ( 'NONE',  ( 767.7687537140311633, -71.90732993114760063, -372.7932403749916830 ) ) ;
#5051=CARTESIAN_POINT ( 'NONE',  ( 772.5602148656447525, -345.7255117493285184, -305.7998596910095443 ) ) ;
#5055=CARTESIAN_POINT ( 'NONE',  ( 786.2056067578752163, -107.8055962898691433, -374.4686193811670023 ) ) ;
#5060=CARTESIAN_POINT ( 'NONE',  ( 784.0799538623451781, -227.8055962898687596, -364.6971507214555572 ) ) ;
#5062=CARTESIAN_POINT ( 'NONE',  ( 807.5423716828161105, -417.0783235625954148, -362.2119215644372048 ) ) ;
#5063=CARTESIAN_POINT ( 'NONE',  ( 793.4146539503750546, -73.98741447168741558, -307.6481478633938877 ) ) ;
#5065=EDGE_LOOP ( 'NONE', ( #3924, #20115 ) ) ;
#5067=CARTESIAN_POINT ( 'NONE',  ( 747.6481478633932056, -373.0999726633340856, -353.4146539503763620 ) ) ;
#5068=AXIS2_PLACEMENT_3D ( 'NONE', #45558, #1621, #33275 ) ;
#5069=CARTESIAN_POINT ( 'NONE',  ( 797.8594530101008786, -229.5436935675106440, -322.1405469898980982 ) ) ;
#5072=CARTESIAN_POINT ( 'NONE',  ( 784.1219089521767955, -213.2817908451527842, -315.0488828828318333 ) ) ;
#5073=CARTESIAN_POINT ( 'NONE',  ( 785.3687786644884454, -179.3618753856927128, -315.3201227861279676 ) ) ;
#5074=CARTESIAN_POINT ( 'NONE',  ( 805.1927285166399315, -400.8164208402374697, -341.8018195045277707 ) ) ;
#5082=DIRECTION ( 'NONE',  ( -1.000000000000000000, -0.000000000000000000, -0.000000000000000000 ) ) ;
#5086=CARTESIAN_POINT ( 'NONE',  ( 748.6759233522253680, -400.3726999360612808, -324.3348316497537098 ) ) ;
#5087=CARTESIAN_POINT ( 'NONE',  ( 796.9462024416508257, -36.45278447660224685, -308.9653473494370246 ) ) ;
#5089=CARTESIAN_POINT ( 'NONE',  ( 755.0636971347428243, -412.2709662947829088, -341.7834795799807353 ) ) ;
#5090=CARTESIAN_POINT ( 'NONE',  ( 774.6312213355098493, 0.6381246143067237364, -364.6798772138717482 ) ) ;
#5093=CARTESIAN_POINT ( 'NONE',  ( 804.4086373105744769, -265.6454272087889876, -333.3843516231986541 ) ) ;
#5094=CARTESIAN_POINT ( 'NONE',  ( 805.0032342141412300, -157.5436935675108998, -314.9967657858571783 ) ) ;
#5103=CARTESIAN_POINT ( 'NONE',  ( 756.5762568750052424, -315.1800572038740711, -348.7366044899774238 ) ) ;
#5105=CARTESIAN_POINT ( 'NONE',  ( 814.2805881961230625, -97.64542720878949922, -331.2368401574024119 ) ) ;
#5106=CARTESIAN_POINT ( 'NONE',  ( 803.2186876482843445, -127.9874144716872308, -350.0220218866286928 ) ) ;
#5109=CARTESIAN_POINT ( 'NONE',  ( 759.9864689768902508, -26.08914811296592262, -354.9819416627836404 ) ) ;
#5110=CARTESIAN_POINT ( 'NONE',  ( 755.8398074228967971, -139.4419599262326699, -333.4516893846970333 ) ) ;
#5112=CARTESIAN_POINT ( 'NONE',  ( 754.8983024940795303, -426.8965053807771142, -336.9254006560228163 ) ) ;
#5119=CARTESIAN_POINT ( 'NONE',  ( 815.3608509340175488, -266.7363362996981095, -341.2497674668889545 ) ) ;
#5126=CARTESIAN_POINT ( 'NONE',  ( 754.7162404726377645, -86.73633629969862113, -339.4709603349214717 ) ) ;
#5127=CARTESIAN_POINT ( 'NONE',  ( 759.7806653035535192, -294.9982390220559978, -324.8639956371181370 ) ) ;
#5130=CARTESIAN_POINT ( 'NONE',  ( 785.3141322388236176, -405.7255117493283478, -364.4286716492789537 ) ) ;
#5131=CARTESIAN_POINT ( 'NONE',  ( 795.1360043628807261, -44.08914811296584446, -360.2193346964456282 ) ) ;
#5135=CARTESIAN_POINT ( 'NONE',  ( 760.0363995740630116, -10.91815448151704793, -368.7758568127991907 ) ) ;
#5138=CARTESIAN_POINT ( 'NONE',  ( 805.6418435158337843, -317.4636090269706301, -363.8556311672236916 ) ) ;
#5142=CARTESIAN_POINT ( 'NONE',  ( 792.1044303154645831, -300.4527844766012663, -317.8323909638837677 ) ) ;
#5144=CARTESIAN_POINT ( 'NONE',  ( 755.8894580844503253, -159.8272453906075157, -332.3691319403863531 ) ) ;
#5148=CARTESIAN_POINT ( 'NONE',  ( 745.1769319972822814, -17.80559628986940979, -346.2694204179732083 ) ) ;
#5149=CARTESIAN_POINT ( 'NONE',  ( 814.9108240113580450, -352.2709662947830225, -337.5031285880265273 ) ) ;
#5154=CARTESIAN_POINT ( 'NONE',  ( 814.2001403089898304, 6.638124614306706306, -347.4397851343538264 ) ) ;
#5159=CARTESIAN_POINT ( 'NONE',  ( 759.2295555964440155, -16.16923265350578021, -353.9708237608231229 ) ) ;
#5164=CARTESIAN_POINT ( 'NONE',  ( 801.3366627262608972, -344.5328690171410813, -353.0897708529566899 ) ) ;
#5167=CARTESIAN_POINT ( 'NONE',  ( 749.8865473780648472, -332.5328690171411381, -322.1177392798429082 ) ) ;
#5172=CARTESIAN_POINT ( 'NONE',  ( 767.7687537140311633, -167.9073299311473022, -372.7932403749916830 ) ) ;
#5175=CARTESIAN_POINT ( 'NONE',  ( 755.5713283507202505, -173.3618753856927128, -334.6858677611754729 ) ) ;
#5177=CARTESIAN_POINT ( 'NONE',  ( 787.5531968255692163, -429.8272453906067199, -316.1348686366205811 ) ) ;
#5180=LINE ( 'NONE', #11892, #8545 ) ;
#5184=CARTESIAN_POINT ( 'NONE',  ( 769.0155153010367712, -442.3726999360611103, -362.7791456095907279 ) ) ;
#5186=CARTESIAN_POINT ( 'NONE',  ( 781.2370466360911223, -212.7363362996982232, -304.9990715423533629 ) ) ;
#5188=CARTESIAN_POINT ( 'NONE',  ( 779.9999999999992042, -462.9681489794448339, -339.9999999999999432 ) ) ;
#5189=CARTESIAN_POINT ( 'NONE',  ( 771.1735550268778070, -177.1800572038744690, -316.3353852180827630 ) ) ;
#5190=CARTESIAN_POINT ( 'NONE',  ( 754.9735926884551418, -354.3510508353228943, -340.5236548041000333 ) ) ;
#5192=CARTESIAN_POINT ( 'NONE',  ( 795.8262568251477660, -214.3726999360618493, -308.3538107759623585 ) ) ;
#5193=CARTESIAN_POINT ( 'NONE',  ( 799.9999999999993179, -462.9681489794448339, -309.9999999999998863 ) ) ;
#5196=CARTESIAN_POINT ( 'NONE',  ( 766.0291762391763086, -58.91815448151690759, -360.7704444035551319 ) ) ;
#5199=CARTESIAN_POINT ( 'NONE',  ( 787.5162901302840055, -251.3618753856923718, -305.4481719005793252 ) ) ;
#5202=CARTESIAN_POINT ( 'NONE',  ( 804.9363028652555840, -64.27096629478397460, -338.2165204200192079 ) ) ;
#5204=CARTESIAN_POINT ( 'NONE',  ( 798.0661480581538854, -122.5328690171417918, -309.5768839229118043 ) ) ;
#5206=CARTESIAN_POINT ( 'NONE',  ( 749.2812353651451076, -390.4527844766011526, -323.2262854647983090 ) ) ;
#5211=CARTESIAN_POINT ( 'NONE',  ( 756.5762568750052424, -387.1800572038738437, -348.7366044899774238 ) ) ;
#5212=DIRECTION ( 'NONE',  ( 0.000000000000000000, 0.000000000000000000, 1.000000000000000000 ) ) ;
#5213=CARTESIAN_POINT ( 'NONE',  ( 752.7379699480933368, -12.00906357242613609, -361.9858362298580232 ) ) ;
#5218=CARTESIAN_POINT ( 'NONE',  ( 769.1273215169530886, -214.7146871989597230, -317.4527132478988847 ) ) ;
#5220=CARTESIAN_POINT ( 'NONE',  ( 808.7758568127978833, -220.1692326535051052, -320.0363995740631822 ) ) ;
#5221=FACE_OUTER_BOUND ( 'NONE', #31032, .T. ) ;
#5225=CARTESIAN_POINT ( 'NONE',  ( 804.9511171171677688, -29.80559628986937781, -335.8780910478229202 ) ) ;
#5227=CARTESIAN_POINT ( 'NONE',  ( 808.0189434323515343, -62.08914811296580183, -319.0252816721025511 ) ) ;
#5228=CARTESIAN_POINT ( 'NONE',  ( 765.0180583372156207, -72.99823902205667991, -360.0135310231089534 ) ) ;
#5230=CARTESIAN_POINT ( 'NONE',  ( 780.5236548040995785, 3.263663700301089765, -314.9735926884559944 ) ) ;
#5232=CARTESIAN_POINT ( 'NONE',  ( 773.4516893846965786, -331.6454272087888171, -315.8398074228977066 ) ) ;
#5241=CARTESIAN_POINT ( 'NONE',  ( 763.0428371773158460, -323.4636090269706301, -358.7617431975195359 ) ) ;
#5242=CARTESIAN_POINT ( 'NONE',  ( 803.6646147819161570, -329.9073299311467053, -348.8264449731210561 ) ) ;
#5243=CARTESIAN_POINT ( 'NONE',  ( 804.6798772138708955, -135.7255117493291152, -334.6312213355107019 ) ) ;
#5246=DIRECTION ( 'NONE',  ( -0.000000000000000000, -0.000000000000000000, 1.000000000000000000 ) ) ;
#5247=CARTESIAN_POINT ( 'NONE',  ( 795.8262568251477660, -118.3726999360621619, -308.3538107759623585 ) ) ;
#5253=CARTESIAN_POINT ( 'NONE',  ( 782.4968714119720516, -130.8164208402383224, -305.0891759886411023 ) ) ;
#5256=CARTESIAN_POINT ( 'NONE',  ( 747.2067596250078623, -267.1800572038742985, -352.2312462859687230 ) ) ;
#5257=CARTESIAN_POINT ( 'NONE',  ( 745.0891759886404770, -436.2709662947827951, -342.4968714119734159 ) ) ;
#5260=CARTESIAN_POINT ( 'NONE',  ( 748.3538107759620743, -328.7146871989592682, -355.8262568251490165 ) ) ;
#5261=CARTESIAN_POINT ( 'NONE',  ( 813.1304606946830518, -89.90732993114750116, -352.3570229623690580 ) ) ;
#5263=CARTESIAN_POINT ( 'NONE',  ( 814.9108240113580450, -352.2709662947830225, -337.5031285880265273 ) ) ;
#5268=CARTESIAN_POINT ( 'NONE',  ( 755.3201227861273992, -219.7255117493289447, -345.3687786644892981 ) ) ;
#5269=CARTESIAN_POINT ( 'NONE',  ( 807.5423716828161105, -129.0783235625963243, -362.2119215644372048 ) ) ;
#5275=CARTESIAN_POINT ( 'NONE',  ( 805.0264073115434940, -222.3510508353233206, -339.4763451958999099 ) ) ;
#5277=CARTESIAN_POINT ( 'NONE',  ( 782.4968714119720516, 13.18357915976123174, -305.0891759886411023 ) ) ;
#5278=CARTESIAN_POINT ( 'NONE',  ( 807.5423716828161105, -57.07832356259658013, -362.2119215644372048 ) ) ;
#5282=CARTESIAN_POINT ( 'NONE',  ( 814.8207195650702488, -362.1908817542432644, -336.2433038121456548 ) ) ;
#5283=CARTESIAN_POINT ( 'NONE',  ( 781.7834795799800531, -226.8164208402380098, -315.0636971347436202 ) ) ;
#5286=CARTESIAN_POINT ( 'NONE',  ( 784.1219089521767955, -237.2817908451526421, -315.0488828828318333 ) ) ;
#5287=CARTESIAN_POINT ( 'NONE',  ( 785.3141322388236176, -213.7255117493289731, -364.4286716492789537 ) ) ;
#5288=CARTESIAN_POINT ( 'NONE',  ( 762.3223304703356007, -367.5436935675102745, -322.3223304703362828 ) ) ;
#5291=CARTESIAN_POINT ( 'NONE',  ( 781.8018195045266339, -118.2709662947837899, -365.1927285166406705 ) ) ;
#5299=CARTESIAN_POINT ( 'NONE',  ( 814.4686193811664907, -435.2817908451521021, -346.2056067578752732 ) ) ;
#5300=CARTESIAN_POINT ( 'NONE',  ( 805.0032342141413437, -37.54369356751133324, -314.9967657858572352 ) ) ;
#5302=CARTESIAN_POINT ( 'NONE',  ( 754.8072714833581358, -388.8164208402374129, -338.1981804954720587 ) ) ;
#5303=CARTESIAN_POINT ( 'NONE',  ( 762.3223304703356007, -7.543693567511430942, -322.3223304703362828 ) ) ;
#5306=CARTESIAN_POINT ( 'NONE',  ( 804.4086373105744769, -289.6454272087889308, -333.3843516231986541 ) ) ;
#5307=CARTESIAN_POINT ( 'NONE',  ( 811.0346526505616112, -182.6346026584199649, -323.0537975583477532 ) ) ;
#5314=CARTESIAN_POINT ( 'NONE',  ( 797.6776695296629214, -331.5436935675104451, -357.6776695296636603 ) ) ;
#5317=CARTESIAN_POINT ( 'NONE',  ( 804.1009440267234822, -95.46360902697132644, -314.0944755984392600 ) ) ;
#5318=CARTESIAN_POINT ( 'NONE',  ( 766.7756240680305382, -110.5328690171418629, -361.5560724626415663 ) ) ;
#5322=CARTESIAN_POINT ( 'NONE',  ( 800.2193346964447755, -18.99823902205683979, -355.1360043628815788 ) ) ;
#5323=CARTESIAN_POINT ( 'NONE',  ( 758.6633372737375112, -116.5328690171418202, -326.9102291470432533 ) ) ;
#5325=CARTESIAN_POINT ( 'NONE',  ( 761.2382568024794409, -423.6237781080499190, -356.9571628226838129 ) ) ;
#5331=CARTESIAN_POINT ( 'NONE',  ( 752.7379699480933368, -276.0090635724253048, -361.9858362298580232 ) ) ;
#5338=CARTESIAN_POINT ( 'NONE',  ( 763.8424801807145741, -114.0090635724258163, -320.5453621957614700 ) ) ;
#5340=CARTESIAN_POINT ( 'NONE',  ( 803.6646147819162707, -281.9073299311469327, -348.8264449731211130 ) ) ;
#5342=CARTESIAN_POINT ( 'NONE',  ( 792.1044303154645831, -420.4527844766009252, -317.8323909638837677 ) ) ;
#5343=CARTESIAN_POINT ( 'NONE',  ( 800.0135310231082713, -86.08914811296573077, -325.0180583372163028 ) ) ;
#5349=CARTESIAN_POINT ( 'NONE',  ( 791.0478386215596629, -357.8272453906068904, -306.7653713866226326 ) ) ;
#5352=PLANE ( 'NONE',  #22396 ) ;
#5353=CARTESIAN_POINT ( 'NONE',  ( 781.7834795799800531, -298.8164208402377540, -315.0636971347436202 ) ) ;
#5355=CARTESIAN_POINT ( 'NONE',  ( 769.9779781133707957, -163.0999726633347677, -316.7813123517150871 ) ) ;
#5358=CARTESIAN_POINT ( 'NONE',  ( 815.2698199232962679, -376.8164208402375834, -342.5225473063383674 ) ) ;
#5363=CARTESIAN_POINT ( 'NONE',  ( 748.9653473494363425, -26.63460265842045871, -356.9462024416521331 ) ) ;
#5369=CARTESIAN_POINT ( 'NONE',  ( 802.7791456095903868, -4.714687198960358039, -329.0155153010375102 ) ) ;
#5370=CARTESIAN_POINT ( 'NONE',  ( 755.0636971347428243, -388.2709662947829656, -341.7834795799807353 ) ) ;
#5376=CARTESIAN_POINT ( 'NONE',  ( 773.3843516231979720, -325.4419599262320162, -364.4086373105754433 ) ) ;
#5379=CARTESIAN_POINT ( 'NONE',  ( 746.7653713866222915, -329.2601417444138860, -351.0478386215610271 ) ) ;
#5385=CARTESIAN_POINT ( 'NONE',  ( 782.5225473063381969, -166.2709662947835909, -375.2698199232970637 ) ) ;
#5388=CARTESIAN_POINT ( 'NONE',  ( 765.0180583372156207, -192.9982390220562820, -360.0135310231089534 ) ) ;
#5390=CARTESIAN_POINT ( 'NONE',  ( 801.9419747391806368, 5.547215523397618142, -351.9812246680014027 ) ) ;
#5396=CARTESIAN_POINT ( 'NONE',  ( 755.1538015810308480, -422.1908817542430370, -343.0433043558613804 ) ) ;
#5399=CARTESIAN_POINT ( 'NONE',  ( 745.7194118038753459, -205.6454272087891297, -348.7631598425976449 ) ) ;
#5402=CARTESIAN_POINT ( 'NONE',  ( 800.2193346964447755, -186.9982390220563104, -355.1360043628815788 ) ) ;
#5403=CARTESIAN_POINT ( 'NONE',  ( 772.3691319403857278, -359.2601417444137724, -315.8894580844506663 ) ) ;
#5404=DIRECTION ( 'NONE',  ( 0.000000000000000000, 0.000000000000000000, 1.000000000000000000 ) ) ;
#5405=CARTESIAN_POINT ( 'NONE',  ( 813.5763878283155464, -219.8272453906073167, -351.1614460488615350 ) ) ;
#5408=CARTESIAN_POINT ( 'NONE',  ( 801.5560724626406000, -48.55451811788057626, -326.7756240680316182 ) ) ;
#5412=CARTESIAN_POINT ( 'NONE',  ( 777.4774526936600978, -250.2709662947833351, -304.7301800767028226 ) ) ;
#5416=CARTESIAN_POINT ( 'NONE',  ( 755.3201227861273992, -51.72551174932946338, -345.3687786644892981 ) ) ;
#5419=CARTESIAN_POINT ( 'NONE',  ( 810.1134526219336749, -128.5328690171417634, -357.8822607201570349 ) ) ;
#5421=CARTESIAN_POINT ( 'NONE',  ( 808.3070685750230950, -378.9982390220555999, -361.1904061080339261 ) ) ;
#5425=CARTESIAN_POINT ( 'NONE',  ( 795.1360043628807261, -404.0891481129646081, -360.2193346964456282 ) ) ;
#5427=CARTESIAN_POINT ( 'NONE',  ( 783.7953271457878373, -8.190881754244330182, -375.1787889125761239 ) ) ;
#5432=CARTESIAN_POINT ( 'NONE',  ( 802.7791456095903868, -220.7146871989596661, -329.0155153010375102 ) ) ;
#5435=CIRCLE ( 'NONE', #19453, 30.00000000000008171 ) ;
#5436=CARTESIAN_POINT ( 'NONE',  ( 813.2346286133761168, -221.2601417444142271, -328.9521613784389160 ) ) ;
#5441=CARTESIAN_POINT ( 'NONE',  ( 771.1735550268778070, -177.1800572038744690, -316.3353852180827630 ) ) ;
#5444=CARTESIAN_POINT ( 'NONE',  ( 810.7187646348534145, -90.45278447660209054, -356.7737145352016341 ) ) ;
#5445=CARTESIAN_POINT ( 'NONE',  ( 795.1360043628808398, -68.08914811296577341, -360.2193346964456282 ) ) ;
#5447=CARTESIAN_POINT ( 'NONE',  ( 787.5531968255692163, 2.172754609392001601, -316.1348686366205811 ) ) ;
#5449=CARTESIAN_POINT ( 'NONE',  ( 793.0897708529556667, -366.5545181178795815, -361.3366627262616362 ) ) ;
#5457=CARTESIAN_POINT ( 'NONE',  ( 766.9102291470427417, -330.5545181178796952, -318.6633372737382501 ) ) ;
#5458=CARTESIAN_POINT ( 'NONE',  ( 759.9864689768902508, -338.0891481129649492, -354.9819416627836404 ) ) ;
#5459=CARTESIAN_POINT ( 'NONE',  ( 795.1360043628807261, -164.0891481129655176, -360.2193346964456282 ) ) ;
#5464=CARTESIAN_POINT ( 'NONE',  ( 787.6308680596127942, -275.2601417444140566, -364.1105419155492768 ) ) ;
#5466=CARTESIAN_POINT ( 'NONE',  ( 744.6391490659812007, -134.7363362996984790, -338.7502325331110455 ) ) ;
#5473=CARTESIAN_POINT ( 'NONE',  ( 772.5602148656447525, -153.7255117493291721, -305.7998596910095443 ) ) ;
#5476=CARTESIAN_POINT ( 'NONE',  ( 815.2698199232961542, -280.8164208402378677, -342.5225473063383106 ) ) ;
#5477=CARTESIAN_POINT ( 'NONE',  ( 747.2067596250078623, -435.1800572038737869, -352.2312462859687230 ) ) ;
#5479=CARTESIAN_POINT ( 'NONE',  ( 745.1769319972822814, -353.8055962898683333, -346.2694204179732083 ) ) ;
#5480=CARTESIAN_POINT ( 'NONE',  ( 792.3570229623688874, -93.18005720387481006, -373.1304606946836202 ) ) ;
#5482=ADVANCED_FACE ( 'NONE', ( #38629 ), #36826, .T. ) ;
#5484=CARTESIAN_POINT ( 'NONE',  ( 755.2512626584698410, -367.5436935675102745, -315.2512626584710915 ) ) ;
#5491=CARTESIAN_POINT ( 'NONE',  ( 758.0141637701419768, -111.0783235625964096, -367.2620300519063790 ) ) ;
#5497=CARTESIAN_POINT ( 'NONE',  ( 793.2243759319678702, -2.532869017142183932, -318.4439275373583200 ) ) ;
#5500=CARTESIAN_POINT ( 'NONE',  ( 754.0944755984390895, -423.6237781080499190, -364.1009440267246760 ) ) ;
#5505=CARTESIAN_POINT ( 'NONE',  ( 809.0717654672305343, -364.9181544815158986, -360.1688906516309885 ) ) ;
#5510=CARTESIAN_POINT ( 'NONE',  ( 761.4292242960306112, -209.4636090269709996, -323.2154366446414429 ) ) ;
#5511=CARTESIAN_POINT ( 'NONE',  ( 802.1676090361156639, -206.6346026584198512, -327.8955696845344505 ) ) ;
#5512=CARTESIAN_POINT ( 'NONE',  ( 778.2165204200184689, -406.8164208402375266, -364.9363028652563230 ) ) ;
#5515=CARTESIAN_POINT ( 'NONE',  ( 797.6776695296629214, -115.5436935675110988, -357.6776695296636603 ) ) ;
#5525=CARTESIAN_POINT ( 'NONE',  ( 811.3240766477731540, -436.3726999360612240, -355.6651683502462902 ) ) ;
#5526=CARTESIAN_POINT ( 'NONE',  ( 800.9747183278959710, -36.99823902205679360, -311.9810565676471583 ) ) ;
#5528=CARTESIAN_POINT ( 'NONE',  ( 781.7834795799800531, -394.8164208402374697, -315.0636971347436202 ) ) ;
#5529=CARTESIAN_POINT ( 'NONE',  ( 755.0636971347428243, -4.270966294784170003, -341.7834795799807353 ) ) ;
#5532=CARTESIAN_POINT ( 'NONE',  ( 757.0176451133909268, -277.0999726633344267, -349.9200121543848354 ) ) ;
#5533=CARTESIAN_POINT ( 'NONE',  ( 763.0537975583475827, -168.4527844766018347, -371.0346526505627480 ) ) ;
#5540=CIRCLE ( 'NONE', #30608, 10.00000000000000888 ) ;
#5542=ADVANCED_FACE ( 'NONE', ( #10602 ), #36008, .T. ) ;
#5546=CARTESIAN_POINT ( 'NONE',  ( 756.3353852180819104, -341.9073299311465917, -331.1735550268788302 ) ) ;
#5547=ADVANCED_FACE ( 'NONE', ( #7377 ), #14774, .F. ) ;
#5550=CARTESIAN_POINT ( 'NONE',  ( 764.1737431748507561, -106.3726999360621903, -371.6461892240376415 ) ) ;
#5551=CARTESIAN_POINT ( 'NONE',  ( 786.6156483768007774, -145.4419599262326699, -315.5913626894246136 ) ) ;
#5556=CARTESIAN_POINT ( 'NONE',  ( 800.2193346964447755, -42.99823902205675807, -355.1360043628815788 ) ) ;
#5557=CARTESIAN_POINT ( 'NONE',  ( 761.2382568024794409, -183.6237781080507148, -356.9571628226838129 ) ) ;
#5558=CARTESIAN_POINT ( 'NONE',  ( 791.9812246680005501, -140.6346026584201070, -361.9419747391813189 ) ) ;
#5561=CARTESIAN_POINT ( 'NONE',  ( 773.7943932421234194, 24.19440371013046231, -305.5313806188329409 ) ) ;
#5566=CARTESIAN_POINT ( 'NONE',  ( 749.5768839229115201, -276.5545181178798657, -358.0661480581553064 ) ) ;
#5573=CARTESIAN_POINT ( 'NONE',  ( 773.4516893846965786, -115.6454272087894424, -315.8398074228977066 ) ) ;
#5574=CARTESIAN_POINT ( 'NONE',  ( 755.0636971347428243, -100.2709662947838609, -341.7834795799807353 ) ) ;
#5575=CARTESIAN_POINT ( 'NONE',  ( 756.3353852180820240, -269.9073299311469327, -331.1735550268787733 ) ) ;
#5578=CARTESIAN_POINT ( 'NONE',  ( 788.7366044899766848, -419.9073299311465348, -316.5762568750059813 ) ) ;
#5579=CARTESIAN_POINT ( 'NONE',  ( 797.6776695296629214, -67.54369356751125508, -357.6776695296636603 ) ) ;
#5586=CARTESIAN_POINT ( 'NONE',  ( 750.9282345327678740, -328.9181544815160692, -319.8311093483690115 ) ) ;
#5590=CARTESIAN_POINT ( 'NONE',  ( 762.3223304703356007, -295.5436935675105588, -322.3223304703362828 ) ) ;
#5592=CARTESIAN_POINT ( 'NONE',  ( 763.0428371773158460, -203.4636090269709996, -358.7617431975195359 ) ) ;
#5596=CARTESIAN_POINT ( 'NONE',  ( 745.0891759886404770, -388.2709662947829656, -342.4968714119734159 ) ) ;
#5601=CARTESIAN_POINT ( 'NONE',  ( 758.8095938919642549, -32.08914811296588709, -311.6929314249763365 ) ) ;
#5602=CARTESIAN_POINT ( 'NONE',  ( 765.0180583372156207, -240.9982390220561683, -360.0135310231089534 ) ) ;
#5606=CARTESIAN_POINT ( 'NONE',  ( 758.6633372737375112, -20.53286901714212931, -326.9102291470432533 ) ) ;
#5614=CARTESIAN_POINT ( 'NONE',  ( 759.2295555964440155, -328.1692326535048210, -353.9708237608231229 ) ) ;
#5617=CARTESIAN_POINT ( 'NONE',  ( 749.8865473780648472, -380.5328690171409676, -322.1177392798429082 ) ) ;
#5624=CARTESIAN_POINT ( 'NONE',  ( 745.7998596910086917, -197.3618753856926560, -332.5602148656461168 ) ) ;
#5627=CARTESIAN_POINT ( 'NONE',  ( 804.6798772138710092, -159.7255117493291436, -334.6312213355106451 ) ) ;
#5628=ORIENTED_EDGE ( 'NONE', *, *, #37315, .T. ) ;
#5629=CARTESIAN_POINT ( 'NONE',  ( 801.9419747391806368, -330.4527844766013231, -351.9812246680014027 ) ) ;
#5630=CARTESIAN_POINT ( 'NONE',  ( 790.7339360641449275, -462.9631818684622999, -362.6136660859752965 ) ) ;
#5637=CARTESIAN_POINT ( 'NONE',  ( 783.0745993439762742, -440.1908817542430370, -365.1016975059196739 ) ) ;
#5641=CARTESIAN_POINT ( 'NONE',  ( 754.3581564841646241, -233.4636090269708575, -316.1443688327762516 ) ) ;
#5645=CARTESIAN_POINT ( 'NONE',  ( 795.1360043628807261, -188.0891481129653187, -360.2193346964456282 ) ) ;
#5646=CARTESIAN_POINT ( 'NONE',  ( 786.6156483768007774, -361.4419599262319593, -315.5913626894246136 ) ) ;
#5648=CARTESIAN_POINT ( 'NONE',  ( 804.1009440267234822, -239.4636090269709143, -314.0944755984392600 ) ) ;
#5650=DIRECTION ( 'NONE',  ( -0.000000000000000000, 1.000000000000000000, -0.000000000000000000 ) ) ;
#5651=CARTESIAN_POINT ( 'NONE',  ( 801.5560724626406000, -72.55451811788049099, -326.7756240680316182 ) ) ;
#5652=AXIS2_PLACEMENT_3D ( 'NONE', #36616, #30125, #29897 ) ;
#5656=CARTESIAN_POINT ( 'NONE',  ( 787.4397851343537695, -285.7255117493286889, -374.2001403089903988 ) ) ;
#5659=CARTESIAN_POINT ( 'NONE',  ( 792.1044303154645831, -60.45278447660215448, -317.8323909638837677 ) ) ;
#5662=CARTESIAN_POINT ( 'NONE',  ( 756.1443688327750579, -141.6237781080508569, -314.3581564841659315 ) ) ;
#5664=CARTESIAN_POINT ( 'NONE',  ( 787.5162901302840055, -419.3618753856918033, -305.4481719005792684 ) ) ;
#5669=CARTESIAN_POINT ( 'NONE',  ( 771.2633955100217236, -407.9073299311465348, -363.4237431249939618 ) ) ;
#5671=CARTESIAN_POINT ( 'NONE',  ( 791.0478386215596629, -45.82724539060783542, -306.7653713866226326 ) ) ;
#5675=CARTESIAN_POINT ( 'NONE',  ( 754.8983024940795303, -234.8965053807777963, -336.9254006560228163 ) ) ;
#5676=CARTESIAN_POINT ( 'NONE',  ( 768.0187753319979720, -128.6346026584201354, -318.0580252608186242 ) ) ;
#5678=CARTESIAN_POINT ( 'NONE',  ( 786.2056067578752163, -275.8055962898685038, -374.4686193811670023 ) ) ;
#5684=CARTESIAN_POINT ( 'NONE',  ( 760.5453621957607311, -21.07832356259667250, -323.8424801807151425 ) ) ;
#5685=CARTESIAN_POINT ( 'NONE',  ( 795.1360043628807261, -188.0891481129653187, -360.2193346964456282 ) ) ;
#5688=CARTESIAN_POINT ( 'NONE',  ( 804.7487373415286811, -67.54369356751125508, -364.7487373415288516 ) ) ;
#5690=CARTESIAN_POINT ( 'NONE',  ( 754.8072714833583632, -76.81642084023847872, -338.1981804954721156 ) ) ;
#5692=CARTESIAN_POINT ( 'NONE',  ( 801.5560724626406000, -24.55451811788064020, -326.7756240680316182 ) ) ;
#5695=CARTESIAN_POINT ( 'NONE',  ( 805.2837595273609850, -362.7363362996977116, -340.5290396650784714 ) ) ;
#5703=CARTESIAN_POINT ( 'NONE',  ( 784.1219089521767955, -333.2817908451523863, -315.0488828828318333 ) ) ;
#5704=CARTESIAN_POINT ( 'NONE',  ( 771.1735550268778070, -321.1800572038740142, -316.3353852180827630 ) ) ;
#5705=CARTESIAN_POINT ( 'NONE',  ( 809.0717654672305343, -124.9181544815167086, -360.1688906516309885 ) ) ;
#5707=CARTESIAN_POINT ( 'NONE',  ( 779.9999999999992042, 16.45630643248849267, -329.9999999999999432 ) ) ;
#5709=CARTESIAN_POINT ( 'NONE',  ( 805.6418435158337843, -125.4636090269712412, -363.8556311672236916 ) ) ;
#5716=CARTESIAN_POINT ( 'NONE',  ( 746.8695393053151292, -173.9073299311472454, -327.6429770376306578 ) ) ;
#5719=CARTESIAN_POINT ( 'NONE',  ( 800.9747183278959710, -300.9982390220559409, -311.9810565676471583 ) ) ;
#5720=ADVANCED_FACE ( 'NONE', ( #11291 ), #38795, .F. ) ;
#5721=CARTESIAN_POINT ( 'NONE',  ( 782.4968714119720516, -442.8164208402372992, -305.0891759886411023 ) ) ;
#5725=CARTESIAN_POINT ( 'NONE',  ( 803.8556311672234642, -345.6237781080501463, -365.6418435158340117 ) ) ;
#5727=CARTESIAN_POINT ( 'NONE',  ( 746.8695393053150156, -77.90732993114757221, -327.6429770376306010 ) ) ;
#5729=CARTESIAN_POINT ( 'NONE',  ( 814.2001403089898304, -377.3618753856920875, -347.4397851343538264 ) ) ;
#5733=CARTESIAN_POINT ( 'NONE',  ( 766.5853460496234675, -133.9874144716872024, -372.3518521366060554 ) ) ;
#5738=CARTESIAN_POINT ( 'NONE',  ( 776.9566956441375396, -12.89650538077851216, -364.8461984189686405 ) ) ;
#5740=CARTESIAN_POINT ( 'NONE',  ( 761.9338519418445230, -422.5328690171408539, -370.4231160770881957 ) ) ;
#5744=CARTESIAN_POINT ( 'NONE',  ( 760.0363995740630116, -370.9181544815159555, -368.7758568127991907 ) ) ;
#5748=CARTESIAN_POINT ( 'NONE',  ( 757.0176451133909268, -205.0999726633346256, -349.9200121543848354 ) ) ;
#5749=CARTESIAN_POINT ( 'NONE',  ( 757.8323909638827445, -218.6346026584197944, -352.1044303154654358 ) ) ;
#5750=CARTESIAN_POINT ( 'NONE',  ( 757.8323909638828582, -410.6346026584191691, -352.1044303154654358 ) ) ;
#5753=CARTESIAN_POINT ( 'NONE',  ( 803.6646147819161570, -113.9073299311474301, -348.8264449731210561 ) ) ;
#5758=CARTESIAN_POINT ( 'NONE',  ( 789.5584187865343893, -452.9681489794450613, -363.1011989789364520 ) ) ;
#5765=CARTESIAN_POINT ( 'NONE',  ( 766.4474001241216001, -451.0999726633339151, -307.3154664389482491 ) ) ;
#5766=CARTESIAN_POINT ( 'NONE',  ( 763.0537975583476964, -48.45278447660221133, -371.0346526505628617 ) ) ;
#5768=CARTESIAN_POINT ( 'NONE',  ( 791.9812246680005501, -428.6346026584192259, -361.9419747391813189 ) ) ;
#5769=CARTESIAN_POINT ( 'NONE',  ( 774.6858677611749044, -9.725511749329603717, -315.5713283507209894 ) ) ;
#5771=DIRECTION ( 'NONE',  ( 0.000000000000000000, -1.000000000000000000, 0.000000000000000000 ) ) ;
#5772=CARTESIAN_POINT ( 'NONE',  ( 793.0897708529556667, -294.5545181178797520, -361.3366627262616362 ) ) ;
#5774=CARTESIAN_POINT ( 'NONE',  ( 758.8095938919642549, -176.0891481129653755, -311.6929314249763365 ) ) ;
#5778=CARTESIAN_POINT ( 'NONE',  ( 766.8731515446878575, 16.45630643248848912, -318.5849060538806725 ) ) ;
#5780=CARTESIAN_POINT ( 'NONE',  ( 746.0683387631852383, -235.4419599262323857, -331.3260364891676204 ) ) ;
#5785=CARTESIAN_POINT ( 'NONE',  ( 764.8639956371174549, -368.0891481129647786, -319.7806653035542013 ) ) ;
#5787=CARTESIAN_POINT ( 'NONE',  ( 754.3581564841646241, -113.4636090269712554, -316.1443688327762516 ) ) ;
#5788=CARTESIAN_POINT ( 'NONE',  ( 760.5453621957607311, -165.0783235625962391, -323.8424801807151425 ) ) ;
#5792=AXIS2_PLACEMENT_3D ( 'NONE', #17729, #4994, #23815 ) ;
#5795=CARTESIAN_POINT ( 'NONE',  ( 805.1927285166397041, -64.81642084023852135, -341.8018195045277707 ) ) ;
#5796=CARTESIAN_POINT ( 'NONE',  ( 772.3691319403857278, -167.2601417444143976, -315.8894580844506663 ) ) ;
#5798=CARTESIAN_POINT ( 'NONE',  ( 744.9990715423526808, 5.648949164675971524, -341.2370466360926002 ) ) ;
#5804=CARTESIAN_POINT ( 'NONE',  ( 813.5763878283155464, -267.8272453906071746, -351.1614460488615350 ) ) ;
#5811=CARTESIAN_POINT ( 'NONE',  ( 779.4763451958990572, -128.7363362996984790, -365.0264073115438919 ) ) ;
#5812=CARTESIAN_POINT ( 'NONE',  ( 762.3223304703356007, -103.5436935675111272, -322.3223304703362828 ) ) ;
#5813=CARTESIAN_POINT ( 'NONE',  ( 757.8323909638828582, -314.6346026584195101, -352.1044303154654358 ) ) ;
#5816=CARTESIAN_POINT ( 'NONE',  ( 755.5713283507202505, -437.3618753856919170, -334.6858677611754729 ) ) ;
#5819=CARTESIAN_POINT ( 'NONE',  ( 779.9999999999992042, -462.9681489794448339, -339.9999999999999432 ) ) ;
#5824=CARTESIAN_POINT ( 'NONE',  ( 791.0478386215596629, -333.8272453906070041, -306.7653713866226326 ) ) ;
#5827=CARTESIAN_POINT ( 'NONE',  ( 785.3141322388236176, -285.7255117493286889, -364.4286716492789537 ) ) ;
#5828=CARTESIAN_POINT ( 'NONE',  ( 802.5472867521000353, -196.3726999360619061, -350.8726784830461156 ) ) ;
#5832=CARTESIAN_POINT ( 'NONE',  ( 782.5225473063383106, -382.2709662947829088, -375.2698199232970637 ) ) ;
#5838=CARTESIAN_POINT ( 'NONE',  ( 787.5162901302840055, -35.36187538569316047, -305.4481719005792684 ) ) ;
#5839=CARTESIAN_POINT ( 'NONE',  ( 755.5713283507202505, -245.3618753856925139, -334.6858677611754729 ) ) ;
#5843=CARTESIAN_POINT ( 'NONE',  ( 790.8726784830453198, -58.71468719896019905, -362.5472867521010585 ) ) ;
#5849=CARTESIAN_POINT ( 'NONE',  ( 755.8398074228967971, -379.4419599262318457, -333.4516893846970333 ) ) ;
#5852=CARTESIAN_POINT ( 'NONE',  ( 761.9338519418445230, -350.5328690171411381, -370.4231160770881957 ) ) ;
#5858=CARTESIAN_POINT ( 'NONE',  ( 808.0189434323515343, -206.0891481129653471, -319.0252816721025511 ) ) ;
#5861=CARTESIAN_POINT ( 'NONE',  ( 755.3201227861273992, -195.7255117493290015, -345.3687786644892981 ) ) ;
#5863=CARTESIAN_POINT ( 'NONE',  ( 771.2633955100217236, -335.9073299311468190, -363.4237431249939618 ) ) ;
#5864=CARTESIAN_POINT ( 'NONE',  ( 755.5913626894240451, -445.6454272087883055, -346.6156483768012890 ) ) ;
#5871=CARTESIAN_POINT ( 'NONE',  ( 798.5707757039680246, -461.4636090269701754, -356.7845633553585003 ) ) ;
#5875=CARTESIAN_POINT ( 'NONE',  ( 760.0363995740630116, -226.9181544815163534, -368.7758568127991907 ) ) ;
#5878=CARTESIAN_POINT ( 'NONE',  ( 797.6776695296629214, -187.5436935675108430, -357.6776695296636603 ) ) ;
#5879=CARTESIAN_POINT ( 'NONE',  ( 765.8855110935204493, -358.1692326535047641, -319.0159684113471599 ) ) ;
#5880=CARTESIAN_POINT ( 'NONE',  ( 815.3608509340175488, -218.7363362996982232, -341.2497674668889545 ) ) ;
#5883=CARTESIAN_POINT ( 'NONE',  ( 780.5236548040995785, -68.73633629969867798, -314.9735926884559944 ) ) ;
#5885=FACE_OUTER_BOUND ( 'NONE', #4279, .T. ) ;
#5886=CARTESIAN_POINT ( 'NONE',  ( 787.6308680596127942, -419.2601417444136587, -364.1105419155492768 ) ) ;
#5887=CARTESIAN_POINT ( 'NONE',  ( 782.4968714119720516, -274.8164208402378108, -305.0891759886411023 ) ) ;
#5890=CARTESIAN_POINT ( 'NONE',  ( 757.8323909638827445, -50.63460265842036989, -352.1044303154654358 ) ) ;
#5892=CARTESIAN_POINT ( 'NONE',  ( 798.0661480581538854, -170.5328690171416781, -309.5768839229118043 ) ) ;
#5894=CARTESIAN_POINT ( 'NONE',  ( 792.3570229623688874, -405.1800572038737300, -373.1304606946836202 ) ) ;
#5895=LINE ( 'NONE', #10051, #26845 ) ;
#5898=CARTESIAN_POINT ( 'NONE',  ( 781.7834795799800531, -442.8164208402372992, -315.0636971347436202 ) ) ;
#5903=CARTESIAN_POINT ( 'NONE',  ( 763.2154366446407039, -237.6237781080505442, -321.4292242960311228 ) ) ;
#5905=CARTESIAN_POINT ( 'NONE',  ( 744.9990715423526808, -258.3510508353231785, -341.2370466360926002 ) ) ;
#5909=CARTESIAN_POINT ( 'NONE',  ( 788.8264449731200330, -189.1800572038744122, -363.6646147819171233 ) ) ;
#5911=CARTESIAN_POINT ( 'NONE',  ( 751.9810565676468741, -98.08914811296568814, -360.9747183278973921 ) ) ;
#5912=CARTESIAN_POINT ( 'NONE',  ( 804.9363028652555840, -64.27096629478397460, -338.2165204200192079 ) ) ;
#5914=CARTESIAN_POINT ( 'NONE',  ( 754.7162404726377645, -62.73633629969871350, -339.4709603349214717 ) ) ;
#5916=CARTESIAN_POINT ( 'NONE',  ( 783.0745993439762742, -368.1908817542433212, -365.1016975059196739 ) ) ;
#5922=CARTESIAN_POINT ( 'NONE',  ( 760.7433823573367135, -324.0090635724251911, -355.9930595647440441 ) ) ;
#5923=CARTESIAN_POINT ( 'NONE',  ( 774.6312213355099630, -311.3618753856922581, -364.6798772138717482 ) ) ;
#5924=CARTESIAN_POINT ( 'NONE',  ( 807.2620300519052989, -144.0090635724257027, -318.0141637701419768 ) ) ;
#5928=CARTESIAN_POINT ( 'NONE',  ( 783.7953271457878373, -104.1908817542440175, -375.1787889125761239 ) ) ;
#5935=CARTESIAN_POINT ( 'NONE',  ( 815.2698199232962679, -160.8164208402382371, -342.5225473063383674 ) ) ;
#5938=CARTESIAN_POINT ( 'NONE',  ( 796.9462024416508257, -300.4527844766012663, -308.9653473494370246 ) ) ;
#5943=CARTESIAN_POINT ( 'NONE',  ( 766.5853460496234675, -349.9874144716865771, -372.3518521366060554 ) ) ;
#5944=CARTESIAN_POINT ( 'NONE',  ( 796.9462024416508257, -108.4527844766019911, -308.9653473494370246 ) ) ;
#5946=CARTESIAN_POINT ( 'NONE',  ( 815.2698199232961542, -376.8164208402375834, -342.5225473063383106 ) ) ;
#5949=EDGE_LOOP ( 'NONE', ( #26381, #20221, #15527, #13701, #4110, #18562, #28056, #18264 ) ) ;
#5951=CARTESIAN_POINT ( 'NONE',  ( 749.8865473780648472, -164.5328690171416781, -322.1177392798429082 ) ) ;
#5956=CARTESIAN_POINT ( 'NONE',  ( 770.0799878456142551, -13.98741447168760033, -362.9823548866085616 ) ) ;
#5958=CARTESIAN_POINT ( 'NONE',  ( 803.8556311672234642, -441.6237781080499190, -365.6418435158340117 ) ) ;
#5962=CARTESIAN_POINT ( 'NONE',  ( 807.2620300519052989, -384.0090635724249637, -318.0141637701419768 ) ) ;
#5963=ADVANCED_FACE ( 'NONE', ( #27139, #5885 ), #25824, .F. ) ;
#5966=CARTESIAN_POINT ( 'NONE',  ( 763.0428371773158460, -227.4636090269709143, -358.7617431975195359 ) ) ;
#5967=CARTESIAN_POINT ( 'NONE',  ( 785.3687786644884454, -203.3618753856925991, -315.3201227861279676 ) ) ;
#5968=CARTESIAN_POINT ( 'NONE',  ( 762.1405469898973024, -409.5436935675101608, -357.8594530101016176 ) ) ;
#5970=CARTESIAN_POINT ( 'NONE',  ( 797.8594530101008786, -109.5436935675110988, -322.1405469898980982 ) ) ;
#5979=CARTESIAN_POINT ( 'NONE',  ( 776.2046728542105711, -452.1908817542428665, -304.8212110874238761 ) ) ;
#5980=CARTESIAN_POINT ( 'NONE',  ( 746.8695393053151292, -77.90732993114757221, -327.6429770376306578 ) ) ;
#5982=CARTESIAN_POINT ( 'NONE',  ( 778.1981804954714335, -442.2709662947826814, -314.8072714833589885 ) ) ;
#5983=CARTESIAN_POINT ( 'NONE',  ( 788.7366044899766848, -35.90732993114770011, -316.5762568750059813 ) ) ;
#5985=CARTESIAN_POINT ( 'NONE',  ( 768.0187753319979720, 15.36539734157940629, -318.0580252608186242 ) ) ;
#5986=CARTESIAN_POINT ( 'NONE',  ( 784.1219089521767955, -285.2817908451526137, -315.0488828828318333 ) ) ;
#5987=CARTESIAN_POINT ( 'NONE',  ( 811.0346526505616112, -206.6346026584198512, -323.0537975583477532 ) ) ;
#5992=CARTESIAN_POINT ( 'NONE',  ( 813.2346286133761168, -245.2601417444141987, -328.9521613784389160 ) ) ;
#5994=CARTESIAN_POINT ( 'NONE',  ( 787.5162901302840055, -299.3618753856922581, -305.4481719005792684 ) ) ;
#5998=CARTESIAN_POINT ( 'NONE',  ( 771.2633955100217236, -359.9073299311467053, -363.4237431249939618 ) ) ;
#6000=CARTESIAN_POINT ( 'NONE',  ( 754.0944755984390895, -39.62377810805116951, -364.1009440267246760 ) ) ;
#6001=CARTESIAN_POINT ( 'NONE',  ( 800.7704444035546203, -172.1692326535052757, -326.0291762391768771 ) ) ;
#6003=CARTESIAN_POINT ( 'NONE',  ( 791.7608162188021197, 205.0000000000000568, -350.0000000000000000 ) ) ;
#6006=CARTESIAN_POINT ( 'NONE',  ( 803.4237431249931660, -63.18005720387488822, -331.2633955100225194 ) ) ;
#6007=CARTESIAN_POINT ( 'NONE',  ( 758.6633372737375112, -164.5328690171416781, -326.9102291470432533 ) ) ;
#6010=CARTESIAN_POINT ( 'NONE',  ( 771.2368401574024119, -13.44195992623305713, -374.2805881961240857 ) ) ;
#6015=ORIENTED_EDGE ( 'NONE', *, *, #39078, .F. ) ;
#6017=CARTESIAN_POINT ( 'NONE',  ( 786.2694204179717872, -285.2817908451526137, -305.1769319972829067 ) ) ;
#6018=ORIENTED_EDGE ( 'NONE', *, *, #23778, .F. ) ;
#6025=CARTESIAN_POINT ( 'NONE',  ( 755.5913626894240451, -109.6454272087894566, -346.6156483768012890 ) ) ;
#6026=CARTESIAN_POINT ( 'NONE',  ( 778.1981804954714335, -106.2709662947838467, -314.8072714833589885 ) ) ;
#6027=CARTESIAN_POINT ( 'NONE',  ( 785.3141322388236176, -309.7255117493287457, -364.4286716492789537 ) ) ;
#6029=CARTESIAN_POINT ( 'NONE',  ( 778.1981804954714335, -418.2709662947827383, -314.8072714833589885 ) ) ;
#6036=CARTESIAN_POINT ( 'NONE',  ( 745.5313806188320314, -327.2817908451525000, -333.7943932421247268 ) ) ;
#6039=CARTESIAN_POINT ( 'NONE',  ( 778.1981804954714335, -322.2709662947830225, -314.8072714833589885 ) ) ;
#6041=CARTESIAN_POINT ( 'NONE',  ( 802.5472867521000353, -172.3726999360619914, -350.8726784830461156 ) ) ;
#6046=CARTESIAN_POINT ( 'NONE',  ( 767.6429770376291799, -393.1800572038737869, -306.8695393053162093 ) ) ;
#6051=CARTESIAN_POINT ( 'NONE',  ( 804.7487373415286811, -19.54369356751139364, -364.7487373415288516 ) ) ;
#6052=CARTESIAN_POINT ( 'NONE',  ( 767.8955696845333705, -264.4527844766016074, -362.1676090361162323 ) ) ;
#6056=CARTESIAN_POINT ( 'NONE',  ( 756.1348686366196716, -65.26014174441471027, -347.5531968255698416 ) ) ;
#6064=CARTESIAN_POINT ( 'NONE',  ( 781.8018195045266339, -46.27096629478404566, -365.1927285166406705 ) ) ;
#6066=CARTESIAN_POINT ( 'NONE',  ( 756.1348686366196716, -377.2601417444137724, -347.5531968255698416 ) ) ;
#6070=CARTESIAN_POINT ( 'NONE',  ( 756.1443688327750579, -357.6237781080501463, -314.3581564841659315 ) ) ;
#6075=DIRECTION ( 'NONE',  ( 1.000000000000000000, 0.000000000000000000, 0.000000000000000000 ) ) ;
#6077=CARTESIAN_POINT ( 'NONE',  ( 813.1304606946830518, -209.9073299311470748, -352.3570229623690580 ) ) ;
#6081=CARTESIAN_POINT ( 'NONE',  ( 774.6858677611749044, -225.7255117493289163, -315.5713283507209894 ) ) ;
#6082=ORIENTED_EDGE ( 'NONE', *, *, #8079, .F. ) ;
#6083=CARTESIAN_POINT ( 'NONE',  ( 792.1044303154645831, -324.4527844766013231, -317.8323909638837677 ) ) ;
#6084=CARTESIAN_POINT ( 'NONE',  ( 763.8424801807145741, -450.0090635724248500, -320.5453621957614700 ) ) ;
#6091=CARTESIAN_POINT ( 'NONE',  ( 802.1676090361156639, 9.365397341579420498, -327.8955696845344505 ) ) ;
#6094=CARTESIAN_POINT ( 'NONE',  ( 793.5525998758768083, -247.0999726633344835, -372.6845335610516941 ) ) ;
#6097=CARTESIAN_POINT ( 'NONE',  ( 778.1981804954714335, -226.2709662947834204, -314.8072714833589885 ) ) ;
#6098=CARTESIAN_POINT ( 'NONE',  ( 799.4546378042377910, -345.0783235625956991, -356.1575198192848006 ) ) ;
#6099=CARTESIAN_POINT ( 'NONE',  ( 755.8990559732751535, -251.4636090269709143, -365.9055244015606831 ) ) ;
#6102=CARTESIAN_POINT ( 'NONE',  ( 773.4516893846965786, -67.64542720878958448, -315.8398074228977066 ) ) ;
#6105=VECTOR ( 'NONE', #5650, 1000.000000000000000 ) ;
#6107=CARTESIAN_POINT ( 'NONE',  ( 767.7687537140311633, -263.9073299311469327, -372.7932403749916830 ) ) ;
#6110=CARTESIAN_POINT ( 'NONE',  ( 774.6858677611749044, -57.72551174932945628, -315.5713283507209894 ) ) ;
#6112=CARTESIAN_POINT ( 'NONE',  ( 778.7502325331095108, -168.3510508353234911, -304.6391490659818828 ) ) ;
#6114=CARTESIAN_POINT ( 'NONE',  ( 808.3070685750230950, -402.9982390220555430, -361.1904061080339261 ) ) ;
#6118=CARTESIAN_POINT ( 'NONE',  ( 756.5762568750052424, -435.1800572038737869, -348.7366044899774238 ) ) ;
#6125=CARTESIAN_POINT ( 'NONE',  ( 795.9930595647434757, -267.0783235625958696, -320.7433823573372820 ) ) ;
#6127=CARTESIAN_POINT ( 'NONE',  ( 748.3538107759620743, -256.7146871989595525, -355.8262568251490165 ) ) ;
#6133=CARTESIAN_POINT ( 'NONE',  ( 755.5713283507202505, -173.3618753856927128, -334.6858677611754729 ) ) ;
#6135=CARTESIAN_POINT ( 'NONE',  ( 772.5602148656447525, -129.7255117493292289, -305.7998596910095443 ) ) ;
#6137=CARTESIAN_POINT ( 'NONE',  ( 804.9363028652555840, -112.2709662947838325, -338.2165204200192079 ) ) ;
#6139=CARTESIAN_POINT ( 'NONE',  ( 790.0220218866281812, -55.09997266333508747, -363.2186876482849129 ) ) ;
#6141=CARTESIAN_POINT ( 'NONE',  ( 780.5236548040995785, -356.7363362996978253, -314.9735926884559944 ) ) ;
#6148=CARTESIAN_POINT ( 'NONE',  ( 790.9844846989617508, -358.3726999360613945, -317.2208543904092721 ) ) ;
#6149=CARTESIAN_POINT ( 'NONE',  ( 801.9419747391806368, -306.4527844766013800, -351.9812246680014027 ) ) ;
#6150=CARTESIAN_POINT ( 'NONE',  ( 793.5525998758768083, -151.0999726633347677, -372.6845335610516941 ) ) ;
#6155=CARTESIAN_POINT ( 'NONE',  ( 769.1273215169530886, -262.7146871989594956, -317.4527132478988847 ) ) ;
#6156=CARTESIAN_POINT ( 'NONE',  ( 815.3608509340175488, -146.7363362996984506, -341.2497674668889545 ) ) ;
#6162=CARTESIAN_POINT ( 'NONE',  ( 812.7932403749906598, -183.1800572038744974, -327.7687537140311633 ) ) ;
#6165=CARTESIAN_POINT ( 'NONE',  ( 755.2512626584698410, -295.5436935675105588, -315.2512626584710915 ) ) ;
#6172=CARTESIAN_POINT ( 'NONE',  ( 778.7502325331095108, -360.3510508353228374, -304.6391490659818828 ) ) ;
#6174=CARTESIAN_POINT ( 'NONE',  ( 792.2312462859673587, -107.9073299311474727, -307.2067596250082602 ) ) ;
#6176=CARTESIAN_POINT ( 'NONE',  ( 755.2512626584698410, -391.5436935675101608, -315.2512626584710915 ) ) ;
#6180=CARTESIAN_POINT ( 'NONE',  ( 745.1769319972822814, -137.8055962898690154, -346.2694204179732083 ) ) ;
#6181=CARTESIAN_POINT ( 'NONE',  ( 799.9999999999993179, -462.9681489794448339, -370.0000000000000568 ) ) ;
#6185=CARTESIAN_POINT ( 'NONE',  ( 803.8651313633788504, -5.260141744414903897, -332.4468031744301015 ) ) ;
#6187=CARTESIAN_POINT ( 'NONE',  ( 812.7932403749906598, 8.819942796124882634, -327.7687537140311633 ) ) ;
#6190=CARTESIAN_POINT ( 'NONE',  ( 786.2694204179717872, -405.2817908451522158, -305.1769319972829067 ) ) ;
#6191=CARTESIAN_POINT ( 'NONE',  ( 797.8594530101008786, -277.5436935675105019, -322.1405469898980982 ) ) ;
#6194=CARTESIAN_POINT ( 'NONE',  ( 798.5707757039680246, -269.4636090269708006, -356.7845633553585003 ) ) ;
#6195=CARTESIAN_POINT ( 'NONE',  ( 771.1735550268778070, -225.1800572038743269, -316.3353852180827630 ) ) ;
#6196=VECTOR ( 'NONE', #32919, 1000.000000000000000 ) ;
#6197=CARTESIAN_POINT ( 'NONE',  ( 778.1981804954715471, -418.2709662947828519, -314.8072714833591021 ) ) ;
#6201=CARTESIAN_POINT ( 'NONE',  ( 790.0183182880230106, -452.9681489794449476, -362.9048749981275250 ) ) ;
#6202=CARTESIAN_POINT ( 'NONE',  ( 747.6481478633932056, -13.09997266333522248, -353.4146539503763620 ) ) ;
#6204=CARTESIAN_POINT ( 'NONE',  ( 799.9999999999993179, 166.4563064324884465, -319.9999999999999432 ) ) ;
#6208=CARTESIAN_POINT ( 'NONE',  ( 746.4236121716829757, -447.8272453906067199, -328.8385539511384650 ) ) ;
#6209=CARTESIAN_POINT ( 'NONE',  ( 767.6429770376291799, -81.18005720387482427, -306.8695393053162093 ) ) ;
#6211=CARTESIAN_POINT ( 'NONE',  ( 755.5713283507202505, -437.3618753856919170, -334.6858677611754729 ) ) ;
#6212=CARTESIAN_POINT ( 'NONE',  ( 771.2633955100217236, -47.90732993114767169, -363.4237431249939618 ) ) ;
#6215=CARTESIAN_POINT ( 'NONE',  ( 800.2193346964447755, 5.001760977943074948, -355.1360043628815788 ) ) ;
#6216=CARTESIAN_POINT ( 'NONE',  ( 758.8095938919642549, -200.0891481129653187, -311.6929314249763365 ) ) ;
#6222=CARTESIAN_POINT ( 'NONE',  ( 788.7631598425961101, -289.4419599262321299, -305.7194118038759143 ) ) ;
#6224=CARTESIAN_POINT ( 'NONE',  ( 777.4774526936600978, -274.2709662947833067, -304.7301800767027657 ) ) ;
#6228=CARTESIAN_POINT ( 'NONE',  ( 759.7806653035534055, -342.9982390220557136, -324.8639956371180801 ) ) ;
#6232=CARTESIAN_POINT ( 'NONE',  ( 783.7566961878529810, -48.89650538077840025, -305.1792804349288417 ) ) ;
#6233=CARTESIAN_POINT ( 'NONE',  ( 795.9930595647434757, -147.0783235625962959, -320.7433823573372820 ) ) ;
#6235=LINE ( 'NONE', #9934, #7777 ) ;
#6236=AXIS2_PLACEMENT_3D ( 'NONE', #8173, #15334, #4261 ) ;
#6239=CARTESIAN_POINT ( 'NONE',  ( 756.5762568750052424, -75.18005720387485269, -348.7366044899774238 ) ) ;
#6240=CARTESIAN_POINT ( 'NONE',  ( 804.9511171171677688, -149.8055962898689870, -335.8780910478229202 ) ) ;
#6243=CARTESIAN_POINT ( 'NONE',  ( 815.0009284576459549, 17.64894916467593688, -338.7629533639073429 ) ) ;
#6249=CARTESIAN_POINT ( 'NONE',  ( 755.8990559732751535, -323.4636090269706301, -365.9055244015606831 ) ) ;
#6257=CARTESIAN_POINT ( 'NONE',  ( 760.7433823573367135, -132.0090635724257595, -355.9930595647440441 ) ) ;
#6258=CARTESIAN_POINT ( 'NONE',  ( 804.9363028652555840, -112.2709662947838325, -338.2165204200192079 ) ) ;
#6259=CARTESIAN_POINT ( 'NONE',  ( 781.7834795799800531, -322.8164208402377540, -315.0636971347436202 ) ) ;
#6261=CARTESIAN_POINT ( 'NONE',  ( 802.1676090361156639, -446.6346026584189985, -327.8955696845344505 ) ) ;
#6269=CARTESIAN_POINT ( 'NONE',  ( 813.5763878283155464, -339.8272453906069472, -351.1614460488615350 ) ) ;
#6273=CARTESIAN_POINT ( 'NONE',  ( 754.8072714833581358, -316.8164208402377540, -338.1981804954720587 ) ) ;
#6275=CARTESIAN_POINT ( 'NONE',  ( 755.1538015810308480, -182.1908817542437760, -343.0433043558613804 ) ) ;
#6279=CARTESIAN_POINT ( 'NONE',  ( 792.2312462859673587, -371.9073299311465917, -307.2067596250082602 ) ) ;
#6280=VECTOR ( 'NONE', #38725, 1000.000000000000000 ) ;
#6285=CARTESIAN_POINT ( 'NONE',  ( 787.5162901302840055, -11.36187538569323863, -305.4481719005792684 ) ) ;
#6287=CARTESIAN_POINT ( 'NONE',  ( 801.9419747391806368, -234.4527844766016358, -351.9812246680014027 ) ) ;
#6292=CARTESIAN_POINT ( 'NONE',  ( 760.5453621957607311, -45.07832356259660145, -323.8424801807151425 ) ) ;
#6295=LINE ( 'NONE', #17149, #36528 ) ;
#6300=CARTESIAN_POINT ( 'NONE',  ( 791.9812246680005501, -68.63460265842033436, -361.9419747391813189 ) ) ;
#6301=CARTESIAN_POINT ( 'NONE',  ( 783.0433043558608688, -360.8965053807773984, -315.1538015810313027 ) ) ;
#6305=CARTESIAN_POINT ( 'NONE',  ( 803.8556311672234642, -369.6237781080500895, -365.6418435158340117 ) ) ;
#6314=CARTESIAN_POINT ( 'NONE',  ( 814.5518280994195948, -231.7255117493288310, -332.4837098697145734 ) ) ;
#6317=CARTESIAN_POINT ( 'NONE',  ( 785.3687786644885591, -227.3618753856925423, -315.3201227861280813 ) ) ;
#6319=CARTESIAN_POINT ( 'NONE',  ( 803.6646147819161570, 6.092670068852159559, -348.8264449731210561 ) ) ;
#6327=ORIENTED_EDGE ( 'NONE', *, *, #20624, .F. ) ;
#6328=CARTESIAN_POINT ( 'NONE',  ( 802.9823548866075953, -457.0999726633339151, -330.0799878456151077 ) ) ;
#6331=CARTESIAN_POINT ( 'NONE',  ( 804.1009440267234822, -239.4636090269709143, -314.0944755984392600 ) ) ;
#6334=CARTESIAN_POINT ( 'NONE',  ( 757.8323909638827445, -218.6346026584197944, -352.1044303154654358 ) ) ;
#6336=CARTESIAN_POINT ( 'NONE',  ( 800.7704444035546203, -388.1692326535045936, -326.0291762391768771 ) ) ;
#6337=CARTESIAN_POINT ( 'NONE',  ( 745.5313806188320314, -255.2817908451526705, -333.7943932421247268 ) ) ;
#6339=CARTESIAN_POINT ( 'NONE',  ( 799.9999999999993179, -462.9681489794448339, -309.9999999999998863 ) ) ;
#6340=CARTESIAN_POINT ( 'NONE',  ( 784.1219089521767955, -69.28179084515321051, -315.0488828828318333 ) ) ;
#6344=CARTESIAN_POINT ( 'NONE',  ( 765.8855110935204493, -430.1692326535043094, -319.0159684113471599 ) ) ;
#6345=CARTESIAN_POINT ( 'NONE',  ( 772.4837098697145166, -263.3618753856924286, -374.5518280994205611 ) ) ;
#6348=CARTESIAN_POINT ( 'NONE',  ( 774.6858677611749044, -81.72551174932937101, -315.5713283507209894 ) ) ;
#6351=CARTESIAN_POINT ( 'NONE',  ( 813.9316612368132837, -151.4419599262326415, -348.6739635108323228 ) ) ;
#6354=CARTESIAN_POINT ( 'NONE',  ( 814.2001403089898304, -425.3618753856919170, -347.4397851343538264 ) ) ;
#6360=CARTESIAN_POINT ( 'NONE',  ( 755.5713283507202505, -413.3618753856920307, -334.6858677611754729 ) ) ;
#6368=CARTESIAN_POINT ( 'NONE',  ( 799.4546378042377910, -273.0783235625958696, -356.1575198192848006 ) ) ;
#6369=CARTESIAN_POINT ( 'NONE',  ( 757.8323909638827445, -122.6346026584201354, -352.1044303154654358 ) ) ;
#6371=CARTESIAN_POINT ( 'NONE',  ( 786.2056067578752163, -251.8055962898686744, -374.4686193811670023 ) ) ;
#6378=CARTESIAN_POINT ( 'NONE',  ( 766.7756240680305382, -62.53286901714199786, -361.5560724626415663 ) ) ;
#6379=CARTESIAN_POINT ( 'NONE',  ( 805.1927285166397041, -160.8164208402382371, -341.8018195045277707 ) ) ;
#6381=CARTESIAN_POINT ( 'NONE',  ( 796.9462024416508257, -108.4527844766019911, -308.9653473494370246 ) ) ;
#6382=CARTESIAN_POINT ( 'NONE',  ( 804.4286716492782716, -113.3618753856929260, -345.3141322388244703 ) ) ;
#6384=CARTESIAN_POINT ( 'NONE',  ( 772.4468031744293057, -57.82724539060780700, -363.8651313633793620 ) ) ;
#6386=CARTESIAN_POINT ( 'NONE',  ( 804.6971507214547046, -339.2817908451524431, -344.0799538623459739 ) ) ;
#6391=FACE_OUTER_BOUND ( 'NONE', #12985, .T. ) ;
#6393=CARTESIAN_POINT ( 'NONE',  ( 796.9571628226829034, -359.4636090269705164, -321.2382568024804641 ) ) ;
#6394=CARTESIAN_POINT ( 'NONE',  ( 778.1981804954714335, -346.2709662947830793, -314.8072714833589885 ) ) ;
#6396=CARTESIAN_POINT ( 'NONE',  ( 750.9282345327678740, -136.9181544815166376, -319.8311093483690115 ) ) ;
#6401=CARTESIAN_POINT ( 'NONE',  ( 754.9735926884551418, -258.3510508353231785, -340.5236548041000333 ) ) ;
#6402=CARTESIAN_POINT ( 'NONE',  ( 814.8207195650702488, -170.1908817542438328, -336.2433038121456548 ) ) ;
#6408=CARTESIAN_POINT ( 'NONE',  ( 804.7487373415286811, -187.5436935675108430, -364.7487373415288516 ) ) ;
#6411=CARTESIAN_POINT ( 'NONE',  ( 749.2812353651451076, -318.4527844766014368, -323.2262854647983090 ) ) ;
#6417=CARTESIAN_POINT ( 'NONE',  ( 805.9055244015594326, -363.6237781080502032, -315.8990559732753240 ) ) ;
#6419=CARTESIAN_POINT ( 'NONE',  ( 782.4968714119720516, -106.8164208402383935, -305.0891759886411023 ) ) ;
#6421=CARTESIAN_POINT ( 'NONE',  ( 812.7932403749906598, -399.1800572038738437, -327.7687537140311633 ) ) ;
#6427=CARTESIAN_POINT ( 'NONE',  ( 800.1688906516307043, -154.1692326535053894, -369.0717654672308186 ) ) ;
#6433=CARTESIAN_POINT ( 'NONE',  ( 801.3366627262608972, -8.532869017142163059, -353.0897708529566899 ) ) ;
#6435=CARTESIAN_POINT ( 'NONE',  ( 754.9967657858570647, -1.543693567511449150, -365.0032342141425374 ) ) ;
#6439=CARTESIAN_POINT ( 'NONE',  ( 755.8990559732751535, -419.4636090269702891, -365.9055244015606831 ) ) ;
#6440=CARTESIAN_POINT ( 'NONE',  ( 804.6798772138708955, -255.7255117493287742, -334.6312213355107019 ) ) ;
#6443=CARTESIAN_POINT ( 'NONE',  ( 769.0155153010367712, -250.3726999360618208, -362.7791456095907279 ) ) ;
#6444=CARTESIAN_POINT ( 'NONE',  ( 800.0135310231082713, -254.0891481129652334, -325.0180583372163028 ) ) ;
#6445=CARTESIAN_POINT ( 'NONE',  ( 756.5762568750052424, -435.1800572038737869, -348.7366044899774238 ) ) ;
#6446=CARTESIAN_POINT ( 'NONE',  ( 801.9419747391806368, -90.45278447660209054, -351.9812246680014027 ) ) ;
#6451=CARTESIAN_POINT ( 'NONE',  ( 760.0363995740630116, -34.91815448151697154, -368.7758568127991907 ) ) ;
#6457=CARTESIAN_POINT ( 'NONE',  ( 804.6971507214547046, -3.281790845153435221, -344.0799538623459739 ) ) ;
#6458=CARTESIAN_POINT ( 'NONE',  ( 792.2312462859673587, -83.90732993114754379, -307.2067596250082602 ) ) ;
#6461=CARTESIAN_POINT ( 'NONE',  ( 792.1044303154645831, -420.4527844766009252, -317.8323909638837677 ) ) ;
#6462=CARTESIAN_POINT ( 'NONE',  ( 800.2193346964446619, -42.99823902205676518, -355.1360043628816925 ) ) ;
#6464=CARTESIAN_POINT ( 'NONE',  ( 814.9108240113580450, -184.2709662947835909, -337.5031285880265273 ) ) ;
#6469=CARTESIAN_POINT ( 'NONE',  ( 761.9338519418445230, -278.5328690171412518, -370.4231160770881957 ) ) ;
#6471=CARTESIAN_POINT ( 'NONE',  ( 745.4481719005789273, -291.7255117493285752, -347.5162901302853129 ) ) ;
#6475=CARTESIAN_POINT ( 'NONE',  ( 785.3687786644884454, -395.3618753856918602, -315.3201227861279676 ) ) ;
#6477=CARTESIAN_POINT ( 'NONE',  ( 748.3538107759620743, -40.71468719896024879, -355.8262568251490165 ) ) ;
#6478=CARTESIAN_POINT ( 'NONE',  ( 805.0264073115434940, -150.3510508353235480, -339.4763451958999099 ) ) ;
#6482=CARTESIAN_POINT ( 'NONE',  ( 785.3687786644884454, -59.36187538569306810, -315.3201227861279676 ) ) ;
#6483=CARTESIAN_POINT ( 'NONE',  ( 790.8726784830453198, -178.7146871989598083, -362.5472867521010585 ) ) ;
#6485=CARTESIAN_POINT ( 'NONE',  ( 768.8385539511368734, 0.7398582555850804487, -306.4236121716840557 ) ) ;
#6490=CARTESIAN_POINT ( 'NONE',  ( 745.5313806188320314, -303.2817908451525000, -333.7943932421247268 ) ) ;
#6495=CARTESIAN_POINT ( 'NONE',  ( 804.1105419155481968, -147.8272453906075157, -347.6308680596136469 ) ) ;
#6496=CARTESIAN_POINT ( 'NONE',  ( 755.5713283507202505, -125.3618753856928834, -334.6858677611754729 ) ) ;
#6497=CARTESIAN_POINT ( 'NONE',  ( 788.8264449731201466, -309.1800572038740711, -363.6646147819170665 ) ) ;
#6500=CARTESIAN_POINT ( 'NONE',  ( 791.6690787386836519, -454.6466601436378028, -367.6383479129825673 ) ) ;
#6504=CARTESIAN_POINT ( 'NONE',  ( 755.8990559732751535, -371.4636090269705164, -365.9055244015606831 ) ) ;
#6510=CARTESIAN_POINT ( 'NONE',  ( 754.8072714833581358, -340.8164208402376971, -338.1981804954720587 ) ) ;
#6511=CARTESIAN_POINT ( 'NONE',  ( 759.0159684113467620, -184.9181544815165239, -325.8855110935213020 ) ) ;
#6512=DIRECTION ( 'NONE',  ( 0.000000000000000000, 0.000000000000000000, 1.000000000000000000 ) ) ;
#6513=CARTESIAN_POINT ( 'NONE',  ( 815.2698199232962679, -400.8164208402374697, -342.5225473063383674 ) ) ;
#6517=CARTESIAN_POINT ( 'NONE',  ( 810.2700907235021077, -453.7763741861470521, -341.5253149289871999 ) ) ;
#6519=CARTESIAN_POINT ( 'NONE',  ( 767.6429770376289525, -57.18005720387489532, -306.8695393053162093 ) ) ;
#6520=CARTESIAN_POINT ( 'NONE',  ( 803.6646147819161570, -233.9073299311470180, -348.8264449731210561 ) ) ;
#6524=CARTESIAN_POINT ( 'NONE',  ( 757.2208543904082489, -40.71468719896024879, -350.9844846989624330 ) ) ;
#6530=CARTESIAN_POINT ( 'NONE',  ( 756.5762568750052424, -51.18005720387493085, -348.7366044899774238 ) ) ;
#6531=CARTESIAN_POINT ( 'NONE',  ( 803.2186876482843445, -367.9874144716865203, -350.0220218866286928 ) ) ;
#6534=CARTESIAN_POINT ( 'NONE',  ( 805.9055244015594326, -363.6237781080502032, -315.8990559732753240 ) ) ;
#6539=( LENGTH_UNIT ( ) NAMED_UNIT ( * ) SI_UNIT ( .MILLI., .METRE. ) );
#6540=CARTESIAN_POINT ( 'NONE',  ( 800.9747183278959710, -204.9982390220562820, -311.9810565676471583 ) ) ;
#6543=CARTESIAN_POINT ( 'NONE',  ( 788.7366044899766848, -203.9073299311471885, -316.5762568750059813 ) ) ;
#6544=EDGE_CURVE ( 'NONE', #22721, #820, #6790, .T. ) ;
#6547=CARTESIAN_POINT ( 'NONE',  ( 778.2165204200184689, -358.8164208402375834, -364.9363028652563230 ) ) ;
#6548=CARTESIAN_POINT ( 'NONE',  ( 781.8018195045266339, 1.729033705215812011, -365.1927285166406705 ) ) ;
#6554=CARTESIAN_POINT ( 'NONE',  ( 797.6776695296629214, 4.456306432488530866, -357.6776695296636603 ) ) ;
#6555=PLANE ( 'NONE',  #17280 ) ;
#6558=CARTESIAN_POINT ( 'NONE',  ( 773.7305795820266212, -225.2817908451527273, -374.8230680027170365 ) ) ;
#6561=CARTESIAN_POINT ( 'NONE',  ( 759.7806653035534055, -222.9982390220561399, -324.8639956371180801 ) ) ;
#6562=CARTESIAN_POINT ( 'NONE',  ( 766.7756240680305382, -398.5328690171409107, -361.5560724626415663 ) ) ;
#6564=CARTESIAN_POINT ( 'NONE',  ( 778.1981804954715471, 13.72903370521577315, -314.8072714833591021 ) ) ;
#6565=CARTESIAN_POINT ( 'NONE',  ( 798.5707757039680246, -77.46360902697138329, -356.7845633553585003 ) ) ;
#6568=CARTESIAN_POINT ( 'NONE',  ( 778.7502325331095108, 23.64894916467591912, -304.6391490659818828 ) ) ;
#6569=CARTESIAN_POINT ( 'NONE',  ( 813.1304606946831655, -281.9073299311469327, -352.3570229623691716 ) ) ;
#6571=CARTESIAN_POINT ( 'NONE',  ( 788.7366044899766848, -83.90732993114754379, -316.5762568750059813 ) ) ;
#6573=CARTESIAN_POINT ( 'NONE',  ( 766.5853460496234675, -181.9874144716870887, -372.3518521366060554 ) ) ;
#6575=CARTESIAN_POINT ( 'NONE',  ( 782.4968714119720516, -394.8164208402374697, -305.0891759886411023 ) ) ;
#6580=CARTESIAN_POINT ( 'NONE',  ( 762.3223304703356007, -415.5436935675102177, -322.3223304703362828 ) ) ;
#6587=CARTESIAN_POINT ( 'NONE',  ( 804.1601925771018387, -247.4419599262323004, -346.5483106153029098 ) ) ;
#6589=CARTESIAN_POINT ( 'NONE',  ( 813.9316612368132837, -271.4419599262321867, -348.6739635108323228 ) ) ;
#6594=CARTESIAN_POINT ( 'NONE',  ( 779.4709603349208464, -48.35105083532386061, -314.7162404726379918 ) ) ;
#6595=CARTESIAN_POINT ( 'NONE',  ( 767.8955696845333705, -168.4527844766018347, -362.1676090361162323 ) ) ;
#6596=CARTESIAN_POINT ( 'NONE',  ( 757.8323909638827445, -194.6346026584198796, -352.1044303154654358 ) ) ;
#6599=CARTESIAN_POINT ( 'NONE',  ( 744.7301800767019131, -124.8164208402383508, -337.4774526936615757 ) ) ;
#6600=CARTESIAN_POINT ( 'NONE',  ( 762.1405469898973024, -121.5436935675110561, -357.8594530101016176 ) ) ;
#6602=CARTESIAN_POINT ( 'NONE',  ( 755.5913626894240451, -61.64542720878961291, -346.6156483768012890 ) ) ;
#6603=CARTESIAN_POINT ( 'NONE',  ( 790.0220218866281812, -391.0999726633340288, -363.2186876482849129 ) ) ;
#6613=CARTESIAN_POINT ( 'NONE',  ( 755.5913626894240451, -349.6454272087887603, -346.6156483768012890 ) ) ;
#6614=CARTESIAN_POINT ( 'NONE',  ( 755.5713283507202505, -341.3618753856922012, -334.6858677611754729 ) ) ;
#6615=CARTESIAN_POINT ( 'NONE',  ( 745.1792804349281596, -134.1908817542439181, -343.7566961878542884 ) ) ;
#6619=DIRECTION ( 'NONE',  ( 0.000000000000000000, -1.000000000000000000, 0.000000000000000000 ) ) ;
#6620=CARTESIAN_POINT ( 'NONE',  ( 766.7756240680305382, -278.5328690171412518, -361.5560724626415663 ) ) ;
#6621=CARTESIAN_POINT ( 'NONE',  ( 783.7953271457878373, -152.1908817542438612, -375.1787889125761239 ) ) ;
#6626=CARTESIAN_POINT ( 'NONE',  ( 745.4481719005789273, -171.7255117493290868, -347.5162901302853697 ) ) ;
#6627=ADVANCED_FACE ( 'NONE', ( #35644, #558 ), #40036, .F. ) ;
#6631=CARTESIAN_POINT ( 'NONE',  ( 759.0252816721024374, -288.9982390220559978, -368.0189434323527280 ) ) ;
#6635=ORIENTED_EDGE ( 'NONE', *, *, #30587, .T. ) ;
#6637=CARTESIAN_POINT ( 'NONE',  ( 815.0009284576459549, -366.3510508353228374, -338.7629533639073429 ) ) ;
#6638=CARTESIAN_POINT ( 'NONE',  ( 810.7187646348534145, -138.4527844766019200, -356.7737145352016341 ) ) ;
#6640=CARTESIAN_POINT ( 'NONE',  ( 749.2812353651451076, -390.4527844766011526, -323.2262854647983090 ) ) ;
#6644=CARTESIAN_POINT ( 'NONE',  ( 768.8385539511368734, -143.2601417444144829, -306.4236121716840557 ) ) ;
#6652=CARTESIAN_POINT ( 'NONE',  ( 814.2001403089898304, -17.36187538569322086, -347.4397851343538264 ) ) ;
#6654=ORIENTED_EDGE ( 'NONE', *, *, #11087, .F. ) ;
#6655=CARTESIAN_POINT ( 'NONE',  ( 746.4236121716829757, -423.8272453906067199, -328.8385539511384650 ) ) ;
#6657=CARTESIAN_POINT ( 'NONE',  ( 759.7806653035534055, -270.9982390220561115, -324.8639956371180801 ) ) ;
#6662=CARTESIAN_POINT ( 'NONE',  ( 801.5560724626406000, -240.5545181178798941, -326.7756240680316182 ) ) ;
#6663=CARTESIAN_POINT ( 'NONE',  ( 797.8594530101008786, -253.5436935675104735, -322.1405469898980982 ) ) ;
#6664=CARTESIAN_POINT ( 'NONE',  ( 779.9999999999992042, -452.9681489794448339, -309.9999999999998863 ) ) ;
#6665=CARTESIAN_POINT ( 'NONE',  ( 791.9812246680005501, -92.63460265842026331, -361.9419747391813189 ) ) ;
#6668=DIRECTION ( 'NONE',  ( -1.000000000000000000, -0.000000000000000000, -0.000000000000000000 ) ) ;
#6669=CARTESIAN_POINT ( 'NONE',  ( 810.4231160770870019, -48.55451811788057626, -321.9338519418446936 ) ) ;
#6675=CARTESIAN_POINT ( 'NONE',  ( 804.8461984189677878, -26.19088175424427334, -336.9566956441385628 ) ) ;
#6676=CARTESIAN_POINT ( 'NONE',  ( 755.2512626584698410, -55.54369356751127640, -315.2512626584710915 ) ) ;
#6678=CARTESIAN_POINT ( 'NONE',  ( 781.7834795799800531, -442.8164208402372992, -315.0636971347436202 ) ) ;
#6679=CARTESIAN_POINT ( 'NONE',  ( 755.5713283507202505, -53.36187538569310362, -334.6858677611754729 ) ) ;
#6681=CARTESIAN_POINT ( 'NONE',  ( 808.0189434323515343, -206.0891481129653471, -319.0252816721025511 ) ) ;
#6686=CARTESIAN_POINT ( 'NONE',  ( 752.4576283171824116, -285.0783235625958127, -317.7880784355627952 ) ) ;
#6688=CARTESIAN_POINT ( 'NONE',  ( 796.7737145352015204, -284.6346026584196807, -370.7187646348536987 ) ) ;
#6692=CARTESIAN_POINT ( 'NONE',  ( 803.6646147819161570, -401.9073299311463643, -348.8264449731210561 ) ) ;
#6694=CARTESIAN_POINT ( 'NONE',  ( 803.8556311672234642, -57.62377810805111267, -365.6418435158340117 ) ) ;
#6695=CARTESIAN_POINT ( 'NONE',  ( 769.1273215169530886, -190.7146871989597798, -317.4527132478988847 ) ) ;
#6700=CARTESIAN_POINT ( 'NONE',  ( 781.7834795799800531, -58.81642084023854267, -315.0636971347436202 ) ) ;
#6701=CARTESIAN_POINT ( 'NONE',  ( 804.1601925771018387, -199.4419599262324709, -346.5483106153029098 ) ) ;
#6704=CARTESIAN_POINT ( 'NONE',  ( 803.8556311672234642, 14.37622189194867417, -365.6418435158340117 ) ) ;
#6709=CARTESIAN_POINT ( 'NONE',  ( 791.0478386215596629, -309.8272453906070041, -306.7653713866226326 ) ) ;
#6713=CARTESIAN_POINT ( 'NONE',  ( 793.9708237608222134, -142.9181544815166376, -319.2295555964448681 ) ) ;
#6714=CARTESIAN_POINT ( 'NONE',  ( 778.2165204200184689, -142.8164208402382656, -364.9363028652563230 ) ) ;
#6716=CARTESIAN_POINT ( 'NONE',  ( 768.0187753319979720, -320.6346026584195670, -318.0580252608186242 ) ) ;
#6718=CARTESIAN_POINT ( 'NONE',  ( 804.6798772138708955, -447.7255117493280636, -334.6312213355107019 ) ) ;
#6724=CARTESIAN_POINT ( 'NONE',  ( 797.8822607201568644, -366.5545181178795815, -370.1134526219340160 ) ) ;
#6729=CARTESIAN_POINT ( 'NONE',  ( 804.9363028652555840, -328.2709662947831362, -338.2165204200192079 ) ) ;
#6731=CARTESIAN_POINT ( 'NONE',  ( 759.0159684113467620, -208.9181544815164102, -325.8855110935213020 ) ) ;
#6735=CARTESIAN_POINT ( 'NONE',  ( 814.2001403089898304, -425.3618753856919170, -347.4397851343538264 ) ) ;
#6740=CARTESIAN_POINT ( 'NONE',  ( 801.1904061080336987, -68.08914811296575920, -368.3070685750235498 ) ) ;
#6741=CARTESIAN_POINT ( 'NONE',  ( 785.3141322388236176, -285.7255117493286889, -364.4286716492789537 ) ) ;
#6746=CARTESIAN_POINT ( 'NONE',  ( 810.4231160770870019, -24.55451811788064020, -321.9338519418446936 ) ) ;
#6747=CARTESIAN_POINT ( 'NONE',  ( 784.0799538623451781, -35.80559628986934229, -364.6971507214555572 ) ) ;
#6754=CARTESIAN_POINT ( 'NONE',  ( 766.7756240680305382, -110.5328690171418629, -361.5560724626415663 ) ) ;
#6756=CARTESIAN_POINT ( 'NONE',  ( 778.2165204200184689, -46.81642084023858530, -364.9363028652563230 ) ) ;
#6757=CARTESIAN_POINT ( 'NONE',  ( 795.9930595647434757, -363.0783235625955854, -320.7433823573372820 ) ) ;
#6760=EDGE_LOOP ( 'NONE', ( #26798, #39176 ) ) ;
#6761=CARTESIAN_POINT ( 'NONE',  ( 801.9858362298568863, -387.0783235625955285, -312.7379699480935642 ) ) ;
#6766=CARTESIAN_POINT ( 'NONE',  ( 814.9108240113580450, -208.2709662947835341, -337.5031285880265273 ) ) ;
#6769=CARTESIAN_POINT ( 'NONE',  ( 794.9819416627830151, -228.9982390220561683, -319.9864689768909898 ) ) ;
#6771=CARTESIAN_POINT ( 'NONE',  ( 800.0135310231082713, -350.0891481129648923, -325.0180583372163028 ) ) ;
#6772=CARTESIAN_POINT ( 'NONE',  ( 771.1735550268778070, -9.180057203875058747, -316.3353852180827630 ) ) ;
#6777=CARTESIAN_POINT ( 'NONE',  ( 804.6798772138708955, 8.274488250670337663, -334.6312213355107019 ) ) ;
#6780=CARTESIAN_POINT ( 'NONE',  ( 764.1737431748507561, -274.3726999360617356, -371.6461892240376415 ) ) ;
#6784=CARTESIAN_POINT ( 'NONE',  ( 804.4286716492782716, -233.3618753856925423, -345.3141322388244703 ) ) ;
#6785=CARTESIAN_POINT ( 'NONE',  ( 757.2208543904082489, -400.7146871989590977, -350.9844846989624330 ) ) ;
#6786=DIRECTION ( 'NONE',  ( -0.000000000000000000, 1.000000000000000000, -0.000000000000000000 ) ) ;
#6788=CARTESIAN_POINT ( 'NONE',  ( 784.1219089521767955, -117.2817908451530684, -315.0488828828318333 ) ) ;
#6790=LINE ( 'NONE', #24800, #28360 ) ;
#6791=CARTESIAN_POINT ( 'NONE',  ( 790.8726784830453198, -442.7146871989589840, -362.5472867521010585 ) ) ;
#6792=CARTESIAN_POINT ( 'NONE',  ( 763.2262854647970016, -320.6346026584195670, -309.2812353651462445 ) ) ;
#6795=CARTESIAN_POINT ( 'NONE',  ( 797.6776695296629214, -67.54369356751125508, -357.6776695296636603 ) ) ;
#6797=CARTESIAN_POINT ( 'NONE',  ( 781.2497674668890113, -204.3510508353233774, -375.3608509340180603 ) ) ;
#6799=CARTESIAN_POINT ( 'NONE',  ( 745.0891759886404770, -436.2709662947827951, -342.4968714119734159 ) ) ;
#6803=CARTESIAN_POINT ( 'NONE',  ( 803.4237431249931660, -423.1800572038737300, -331.2633955100225194 ) ) ;
#6809=CARTESIAN_POINT ( 'NONE',  ( 789.9200121543843807, -265.9874144716867477, -317.0176451133914384 ) ) ;
#6812=CARTESIAN_POINT ( 'NONE',  ( 766.5853460496234675, -277.9874144716867477, -372.3518521366060554 ) ) ;
#6817=CARTESIAN_POINT ( 'NONE',  ( 758.6633372737375112, -44.53286901714205470, -326.9102291470432533 ) ) ;
#6818=CARTESIAN_POINT ( 'NONE',  ( 762.1405469898971887, -169.5436935675108430, -357.8594530101015607 ) ) ;
#6819=CARTESIAN_POINT ( 'NONE',  ( 756.5762568750052424, -219.1800572038744122, -348.7366044899774238 ) ) ;
#6821=CARTESIAN_POINT ( 'NONE',  ( 767.7687537140311633, -95.90732993114751537, -372.7932403749916830 ) ) ;
#6822=CARTESIAN_POINT ( 'NONE',  ( 762.1405469898973024, -97.54369356751114140, -357.8594530101016176 ) ) ;
#6824=CARTESIAN_POINT ( 'NONE',  ( 790.9844846989617508, -382.3726999360613945, -317.2208543904092721 ) ) ;
#6829=FACE_BOUND ( 'NONE', #13313, .T. ) ;
#6832=CARTESIAN_POINT ( 'NONE',  ( 798.5707757039680246, -365.4636090269705164, -356.7845633553585003 ) ) ;
#6833=CARTESIAN_POINT ( 'NONE',  ( 759.7806653035534055, -342.9982390220557136, -324.8639956371180801 ) ) ;
#6835=CARTESIAN_POINT ( 'NONE',  ( 745.1792804349281596, -182.1908817542437760, -343.7566961878542884 ) ) ;
#6839=CARTESIAN_POINT ( 'NONE',  ( 803.8651313633788504, -293.2601417444139429, -332.4468031744301015 ) ) ;
#6840=CARTESIAN_POINT ( 'NONE',  ( 804.4286716492782716, -449.3618753856918602, -345.3141322388244703 ) ) ;
#6841=CARTESIAN_POINT ( 'NONE',  ( 760.0363995740630116, -154.9181544815165523, -368.7758568127991907 ) ) ;
#6846=CARTESIAN_POINT ( 'NONE',  ( 763.0537975583476964, -216.4527844766016926, -371.0346526505628617 ) ) ;
#6849=CARTESIAN_POINT ( 'NONE',  ( 759.0252816721024374, -336.9982390220558273, -368.0189434323527280 ) ) ;
#6851=CARTESIAN_POINT ( 'NONE',  ( 799.9999999999993179, -462.9681489794448339, -370.0000000000000568 ) ) ;
#6856=CARTESIAN_POINT ( 'NONE',  ( 744.9990715423526808, -378.3510508353227806, -341.2370466360926002 ) ) ;
#6857=CARTESIAN_POINT ( 'NONE',  ( 748.9653473494363425, -122.6346026584201354, -356.9462024416521331 ) ) ;
#6858=CARTESIAN_POINT ( 'NONE',  ( 813.1304606946830518, -425.9073299311463074, -352.3570229623690580 ) ) ;
#6864=CARTESIAN_POINT ( 'NONE',  ( 749.8865473780648472, -140.5328690171417634, -322.1177392798429082 ) ) ;
#6871=CARTESIAN_POINT ( 'NONE',  ( 801.1904061080336987, -20.08914811296592973, -368.3070685750235498 ) ) ;
#6872=FACE_OUTER_BOUND ( 'NONE', #37158, .T. ) ;
#6875=CARTESIAN_POINT ( 'NONE',  ( 792.1044303154645831, -180.4527844766017211, -317.8323909638837677 ) ) ;
#6876=CARTESIAN_POINT ( 'NONE',  ( 799.9636004259356241, -406.9181544815157849, -311.2241431872006956 ) ) ;
#6881=CARTESIAN_POINT ( 'NONE',  ( 791.9812246680005501, -260.6346026584197375, -361.9419747391813189 ) ) ;
#6885=CARTESIAN_POINT ( 'NONE',  ( 773.4516893846965786, -259.6454272087890445, -315.8398074228977066 ) ) ;
#6886=CARTESIAN_POINT ( 'NONE',  ( 794.9819416627830151, -252.9982390220560831, -319.9864689768909898 ) ) ;
#6888=CARTESIAN_POINT ( 'NONE',  ( 778.2165204200184689, -118.8164208402383508, -364.9363028652563230 ) ) ;
#6893=CARTESIAN_POINT ( 'NONE',  ( 749.5768839229115201, -36.55451811788061178, -358.0661480581553064 ) ) ;
#6899=CARTESIAN_POINT ( 'NONE',  ( 772.4468031744293057, -9.827245390607961539, -363.8651313633793620 ) ) ;
#6901=CARTESIAN_POINT ( 'NONE',  ( 792.3570229623691148, -69.18005720387488111, -373.1304606946836770 ) ) ;
#6907=CARTESIAN_POINT ( 'NONE',  ( 767.6429770376289525, -201.1800572038744690, -306.8695393053162093 ) ) ;
#6912=CARTESIAN_POINT ( 'NONE',  ( 764.3348316497523456, -286.7146871989594388, -308.6759233522265617 ) ) ;
#6915=CARTESIAN_POINT ( 'NONE',  ( 772.4837098697144029, -287.3618753856923718, -374.5518280994205611 ) ) ;
#6920=CARTESIAN_POINT ( 'NONE',  ( 804.6798772138708955, -375.7255117493283478, -334.6312213355107019 ) ) ;
#6923=CARTESIAN_POINT ( 'NONE',  ( 786.2056067578752163, -35.80559628986934229, -374.4686193811670023 ) ) ;
#6924=CARTESIAN_POINT ( 'NONE',  ( 759.2295555964440155, -184.1692326535052757, -353.9708237608231229 ) ) ;
#6929=CARTESIAN_POINT ( 'NONE',  ( 756.1348686366196716, -185.2601417444143692, -347.5531968255698416 ) ) ;
#6931=CARTESIAN_POINT ( 'NONE',  ( 807.5423716828161105, -33.07832356259662987, -362.2119215644372048 ) ) ;
#6938=CARTESIAN_POINT ( 'NONE',  ( 807.2620300519052989, -312.0090635724251911, -318.0141637701419768 ) ) ;
#6943=CARTESIAN_POINT ( 'NONE',  ( 801.5560724626406000, -144.5545181178802636, -326.7756240680316182 ) ) ;
#6944=CARTESIAN_POINT ( 'NONE',  ( 765.0180583372156207, -144.9982390220564525, -360.0135310231089534 ) ) ;
#6945=CARTESIAN_POINT ( 'NONE',  ( 795.1360043628808398, -356.0891481129648355, -360.2193346964456282 ) ) ;
#6948=AXIS2_PLACEMENT_3D ( 'NONE', #4159, #33020, #28854 ) ;
#6950=DIRECTION ( 'NONE',  ( 0.000000000000000000, 0.000000000000000000, -1.000000000000000000 ) ) ;
#6955=CARTESIAN_POINT ( 'NONE',  ( 786.2694204179717872, -381.2817908451523294, -305.1769319972829067 ) ) ;
#6960=CARTESIAN_POINT ( 'NONE',  ( 762.1405469898971887, -337.5436935675102177, -357.8594530101015607 ) ) ;
#6961=EDGE_CURVE ( 'NONE', #16350, #3536, #16219, .T. ) ;
#6963=CARTESIAN_POINT ( 'NONE',  ( 769.9779781133707957, -211.0999726633346540, -316.7813123517150871 ) ) ;
#6969=CARTESIAN_POINT ( 'NONE',  ( 767.6429770376291799, -417.1800572038736732, -306.8695393053162093 ) ) ;
#6973=CARTESIAN_POINT ( 'NONE',  ( 793.5337260303429048, -457.7979077669877483, -366.8220830107578649 ) ) ;
#6975=CARTESIAN_POINT ( 'NONE',  ( 814.2001403089898304, -41.36187538569314626, -347.4397851343538264 ) ) ;
#6976=CARTESIAN_POINT ( 'NONE',  ( 754.8072714833581358, -268.8164208402378108, -338.1981804954720587 ) ) ;
#6981=CARTESIAN_POINT ( 'NONE',  ( 762.1177392798416577, -42.55451811788057626, -309.8865473780659272 ) ) ;
#6982=CARTESIAN_POINT ( 'NONE',  ( 798.7617431975189675, -75.62377810805104161, -323.0428371773161871 ) ) ;
#6988=CARTESIAN_POINT ( 'NONE',  ( 778.1981804954714335, -10.27096629478414691, -314.8072714833589885 ) ) ;
#6989=CARTESIAN_POINT ( 'NONE',  ( 790.8726784830453198, -106.7146871989600498, -362.5472867521010585 ) ) ;
#6991=CARTESIAN_POINT ( 'NONE',  ( 785.3141322388236176, -69.72551174932942786, -364.4286716492789537 ) ) ;
#6993=CARTESIAN_POINT ( 'NONE',  ( 757.2208543904082489, -400.7146871989590977, -350.9844846989624330 ) ) ;
#6996=CARTESIAN_POINT ( 'NONE',  ( 776.2433038121456548, -396.8965053807772847, -374.8207195650711014 ) ) ;
#7002=CARTESIAN_POINT ( 'NONE',  ( 772.5602148656447525, -249.7255117493288594, -305.7998596910095443 ) ) ;
#7006=CARTESIAN_POINT ( 'NONE',  ( 801.9419747391806368, -234.4527844766016358, -351.9812246680014027 ) ) ;
#7008=CARTESIAN_POINT ( 'NONE',  ( 785.3141322388236176, -357.7255117493285184, -364.4286716492789537 ) ) ;
#7009=CARTESIAN_POINT ( 'NONE',  ( 792.1044303154645831, -12.45278447660232146, -317.8323909638837677 ) ) ;
#7014=CARTESIAN_POINT ( 'NONE',  ( 805.1927285166397041, -16.81642084023866701, -341.8018195045277707 ) ) ;
#7017=CARTESIAN_POINT ( 'NONE',  ( 814.8207195650702488, -266.1908817542435486, -336.2433038121456548 ) ) ;
#7020=CIRCLE ( 'NONE', #34307, 10.00000000000000888 ) ;
#7022=CARTESIAN_POINT ( 'NONE',  ( 778.2165204200184689, -238.8164208402379813, -364.9363028652563230 ) ) ;
#7023=CARTESIAN_POINT ( 'NONE',  ( 779.4709603349208464, -408.3510508353227806, -314.7162404726379918 ) ) ;
#7026=CARTESIAN_POINT ( 'NONE',  ( 802.5472867521000353, -100.3726999360622187, -350.8726784830461156 ) ) ;
#7027=AXIS2_PLACEMENT_3D ( 'NONE', #45159, #13521, #13756 ) ;
#7031=CARTESIAN_POINT ( 'NONE',  ( 799.4546378042377910, -441.0783235625953580, -356.1575198192848006 ) ) ;
#7032=CARTESIAN_POINT ( 'NONE',  ( 808.0189434323515343, -326.0891481129649492, -319.0252816721025511 ) ) ;
#7034=CYLINDRICAL_SURFACE ( 'NONE', #12830, 10.00000000000000888 ) ;
#7035=CARTESIAN_POINT ( 'NONE',  ( 803.4237431249931660, -87.18005720387481006, -331.2633955100225194 ) ) ;
#7037=CARTESIAN_POINT ( 'NONE',  ( 805.9055244015594326, -219.6237781080506295, -315.8990559732753240 ) ) ;
#7039=CARTESIAN_POINT ( 'NONE',  ( 800.9747183278959710, -444.9982390220554862, -311.9810565676471583 ) ) ;
#7045=CARTESIAN_POINT ( 'NONE',  ( 804.1601925771018387, 16.55804007376685050, -346.5483106153029098 ) ) ;
#7046=AXIS2_PLACEMENT_3D ( 'NONE', #17229, #45422, #21156 ) ;
#7053=CARTESIAN_POINT ( 'NONE',  ( 760.5453621957607311, -261.0783235625959264, -323.8424801807151425 ) ) ;
#7055=CARTESIAN_POINT ( 'NONE',  ( 798.0661480581538854, -290.5328690171412518, -309.5768839229118043 ) ) ;
#7061=CARTESIAN_POINT ( 'NONE',  ( 804.1601925771018387, -31.44195992623299674, -346.5483106153029098 ) ) ;
#7062=CARTESIAN_POINT ( 'NONE',  ( 774.6858677611749044, -177.7255117493290868, -315.5713283507209894 ) ) ;
#7063=CARTESIAN_POINT ( 'NONE',  ( 785.3687786644884454, -203.3618753856925991, -315.3201227861279676 ) ) ;
#7066=CARTESIAN_POINT ( 'NONE',  ( 814.5518280994195948, -159.7255117493291436, -332.4837098697145734 ) ) ;
#7067=CIRCLE ( 'NONE', #8551, 10.00000000000000888 ) ;
#7068=CARTESIAN_POINT ( 'NONE',  ( 795.1360043628808398, -92.08914811296570235, -360.2193346964456282 ) ) ;
#7069=ORIENTED_EDGE ( 'NONE', *, *, #40142, .T. ) ;
#7070=CARTESIAN_POINT ( 'NONE',  ( 787.5531968255692163, -381.8272453906068336, -316.1348686366205811 ) ) ;
#7078=CARTESIAN_POINT ( 'NONE',  ( 790.0220218866281812, -367.0999726633342561, -363.2186876482849129 ) ) ;
#7079=CARTESIAN_POINT ( 'NONE',  ( 804.4286716492782716, -353.3618753856922012, -345.3141322388244703 ) ) ;
#7080=CARTESIAN_POINT ( 'NONE',  ( 760.0363995740630116, -154.9181544815165523, -368.7758568127991907 ) ) ;
#7081=AXIS2_PLACEMENT_3D ( 'NONE', #41899, #7480, #45602 ) ;
#7086=CARTESIAN_POINT ( 'NONE',  ( 776.9566956441375396, -300.8965053807775689, -364.8461984189686405 ) ) ;
#7087=CARTESIAN_POINT ( 'NONE',  ( 791.9812246680005501, -452.6346026584191691, -361.9419747391813189 ) ) ;
#7088=CARTESIAN_POINT ( 'NONE',  ( 745.7194118038753459, -157.6454272087893287, -348.7631598425976449 ) ) ;
#7094=CARTESIAN_POINT ( 'NONE',  ( 814.5518280994195948, -207.7255117493289731, -332.4837098697145166 ) ) ;
#7099=CARTESIAN_POINT ( 'NONE',  ( 783.7566961878529810, -96.89650538077825104, -305.1792804349288417 ) ) ;
#7100=CARTESIAN_POINT ( 'NONE',  ( 812.7932403749906598, -327.1800572038741279, -327.7687537140311633 ) ) ;
#7107=CARTESIAN_POINT ( 'NONE',  ( 771.2368401574024119, -373.4419599262319593, -374.2805881961240857 ) ) ;
#7108=CARTESIAN_POINT ( 'NONE',  ( 747.2067596250078623, -147.1800572038746395, -352.2312462859687230 ) ) ;
#7109=CARTESIAN_POINT ( 'NONE',  ( 811.0346526505616112, -422.6346026584192259, -323.0537975583477532 ) ) ;
#7113=CARTESIAN_POINT ( 'NONE',  ( 752.4576283171824116, -189.0783235625961822, -317.7880784355627952 ) ) ;
#7120=CARTESIAN_POINT ( 'NONE',  ( 745.4481719005789273, -27.72551174932954510, -347.5162901302853129 ) ) ;
#7123=CARTESIAN_POINT ( 'NONE',  ( 799.9636004259356241, -430.9181544815157849, -311.2241431872006956 ) ) ;
#7127=CARTESIAN_POINT ( 'NONE',  ( 785.3687786644884454, -251.3618753856923149, -315.3201227861279676 ) ) ;
#7132=CARTESIAN_POINT ( 'NONE',  ( 766.9102291470427417, -258.5545181178799226, -318.6633372737382501 ) ) ;
#7133=CARTESIAN_POINT ( 'NONE',  ( 781.8018195045266339, -262.2709662947831930, -365.1927285166406705 ) ) ;
#7134=CARTESIAN_POINT ( 'NONE',  ( 803.4237431249931660, -447.1800572038736732, -331.2633955100225194 ) ) ;
#7135=CARTESIAN_POINT ( 'NONE',  ( 788.8264449731200330, -117.1800572038746964, -363.6646147819171233 ) ) ;
#7140=CARTESIAN_POINT ( 'NONE',  ( 747.6481478633932056, -61.09997266333506616, -353.4146539503763620 ) ) ;
#7147=CARTESIAN_POINT ( 'NONE',  ( 779.4763451958990572, -8.736336299698871599, -365.0264073115438919 ) ) ;
#7149=CARTESIAN_POINT ( 'NONE',  ( 810.7187646348534145, -90.45278447660209054, -356.7737145352016341 ) ) ;
#7151=DIRECTION ( 'NONE',  ( 0.000000000000000000, -1.000000000000000000, 0.000000000000000000 ) ) ;
#7154=CARTESIAN_POINT ( 'NONE',  ( 792.2312462859673587, -251.9073299311470748, -307.2067596250082602 ) ) ;
#7159=CARTESIAN_POINT ( 'NONE',  ( 815.1787889125755555, -270.8965053807777394, -343.7953271457877804 ) ) ;
#7160=VECTOR ( 'NONE', #17348, 1000.000000000000000 ) ;
#7162=CARTESIAN_POINT ( 'NONE',  ( 812.7932403749906598, -303.1800572038740711, -327.7687537140311633 ) ) ;
#7166=CARTESIAN_POINT ( 'NONE',  ( 764.8639956371174549, -392.0891481129648355, -319.7806653035542013 ) ) ;
#7169=CARTESIAN_POINT ( 'NONE',  ( 748.3538107759620743, -88.71468719896009247, -355.8262568251490165 ) ) ;
#7174=CARTESIAN_POINT ( 'NONE',  ( 804.6798772138708955, -87.72551174932937101, -334.6312213355107019 ) ) ;
#7175=CARTESIAN_POINT ( 'NONE',  ( 756.1348686366196716, -209.2601417444142839, -347.5531968255698416 ) ) ;
#7177=CARTESIAN_POINT ( 'NONE',  ( 783.7566961878529810, -48.89650538077840025, -305.1792804349288417 ) ) ;
#7181=CARTESIAN_POINT ( 'NONE',  ( 757.7880784355613741, -306.0090635724252479, -312.4576283171834916 ) ) ;
#7183=AXIS2_PLACEMENT_3D ( 'NONE', #4140, #22337, #15444 ) ;
#7187=CARTESIAN_POINT ( 'NONE',  ( 766.0291762391763086, -154.9181544815165523, -360.7704444035551319 ) ) ;
#7188=CARTESIAN_POINT ( 'NONE',  ( 797.8594530101008786, -133.5436935675110135, -322.1405469898980982 ) ) ;
#7189=CARTESIAN_POINT ( 'NONE',  ( 755.0636971347428243, -340.2709662947831362, -341.7834795799807353 ) ) ;
#7201=CARTESIAN_POINT ( 'NONE',  ( 778.7629533639073998, -392.7363362996977116, -375.0009284576466371 ) ) ;
#7202=CARTESIAN_POINT ( 'NONE',  ( 815.2698199232962679, -16.81642084023867412, -342.5225473063383674 ) ) ;
#7205=CARTESIAN_POINT ( 'NONE',  ( 797.8594530101008786, -349.5436935675102745, -322.1405469898980982 ) ) ;
#7208=CARTESIAN_POINT ( 'NONE',  ( 763.8424801807145741, -234.0090635724255037, -320.5453621957614700 ) ) ;
#7212=CARTESIAN_POINT ( 'NONE',  ( 787.5162901302840055, -419.3618753856918602, -305.4481719005793252 ) ) ;
#7219=CARTESIAN_POINT ( 'NONE',  ( 759.0252816721024374, -48.99823902205675807, -368.0189434323527280 ) ) ;
#7220=CARTESIAN_POINT ( 'NONE',  ( 756.5762568750052424, -267.1800572038742985, -348.7366044899774238 ) ) ;
#7225=CARTESIAN_POINT ( 'NONE',  ( 776.2046728542105711, -20.19088175424429110, -304.8212110874238761 ) ) ;
#7226=CARTESIAN_POINT ( 'NONE',  ( 769.1273215169530886, -70.71468719896014932, -317.4527132478988847 ) ) ;
#7234=CARTESIAN_POINT ( 'NONE',  ( 778.1981804954714335, -106.2709662947838467, -314.8072714833589885 ) ) ;
#7235=CARTESIAN_POINT ( 'NONE',  ( 756.7813123517142913, -403.9874144716863498, -329.9779781133712504 ) ) ;
#7238=CARTESIAN_POINT ( 'NONE',  ( 773.7943932421234194, -407.8055962898681628, -305.5313806188329409 ) ) ;
#7240=CARTESIAN_POINT ( 'NONE',  ( 799.9999999999993179, -512.9681489794448908, -370.0000000000000000 ) ) ;
#7245=CARTESIAN_POINT ( 'NONE',  ( 815.2698199232961542, -256.8164208402379245, -342.5225473063383106 ) ) ;
#7250=CARTESIAN_POINT ( 'NONE',  ( 794.9819416627830151, -252.9982390220560831, -319.9864689768909898 ) ) ;
#7252=CARTESIAN_POINT ( 'NONE',  ( 756.5762568750052424, -363.1800572038739006, -348.7366044899774238 ) ) ;
#7253=CARTESIAN_POINT ( 'NONE',  ( 755.5713283507202505, -29.36187538569318178, -334.6858677611754729 ) ) ;
#7258=CARTESIAN_POINT ( 'NONE',  ( 774.6858677611749044, -9.725511749329603717, -315.5713283507209894 ) ) ;
#7262=CARTESIAN_POINT ( 'NONE',  ( 748.6759233522253680, -280.3726999360616787, -324.3348316497537098 ) ) ;
#7266=CARTESIAN_POINT ( 'NONE',  ( 755.3201227861273992, -267.7255117493286320, -345.3687786644892981 ) ) ;
#7267=CARTESIAN_POINT ( 'NONE',  ( 802.7791456095903868, -388.7146871989592114, -329.0155153010375102 ) ) ;
#7269=CARTESIAN_POINT ( 'NONE',  ( 760.7433823573367135, -132.0090635724257595, -355.9930595647440441 ) ) ;
#7272=CARTESIAN_POINT ( 'NONE',  ( 788.7631598425961101, -1.441959926233096656, -305.7194118038759143 ) ) ;
#7273=CARTESIAN_POINT ( 'NONE',  ( 745.4481719005789273, -315.7255117493286320, -347.5162901302853697 ) ) ;
#7276=CARTESIAN_POINT ( 'NONE',  ( 758.0580252608178853, -78.45278447660211896, -328.0187753319985404 ) ) ;
#7278=CARTESIAN_POINT ( 'NONE',  ( 810.1134526219336749, -200.5328690171415644, -357.8822607201570349 ) ) ;
#7280=CARTESIAN_POINT ( 'NONE',  ( 782.4968714119720516, -442.8164208402372992, -305.0891759886411023 ) ) ;
#7284=CARTESIAN_POINT ( 'NONE',  ( 756.1348686366196716, 6.739858255585061464, -347.5531968255698416 ) ) ;
#7290=CARTESIAN_POINT ( 'NONE',  ( 776.9566956441375396, -300.8965053807775689, -364.8461984189686405 ) ) ;
#7292=CARTESIAN_POINT ( 'NONE',  ( 758.0141637701419768, -279.0783235625958127, -367.2620300519063790 ) ) ;
#7297=CARTESIAN_POINT ( 'NONE',  ( 799.4546378042377910, -57.07832356259658013, -356.1575198192848006 ) ) ;
#7298=CARTESIAN_POINT ( 'NONE',  ( 794.9819416627830151, -156.9982390220564241, -319.9864689768909898 ) ) ;
#7299=CARTESIAN_POINT ( 'NONE',  ( 758.0580252608178853, -222.4527844766016642, -328.0187753319985404 ) ) ;
#7301=CARTESIAN_POINT ( 'NONE',  ( 763.2262854647970016, -152.6346026584200786, -309.2812353651462445 ) ) ;
#7303=CARTESIAN_POINT ( 'NONE',  ( 756.3353852180820240, -125.9073299311474159, -331.1735550268787733 ) ) ;
#7305=CARTESIAN_POINT ( 'NONE',  ( 758.4439275373578084, -396.5545181178794678, -353.2243759319684386 ) ) ;
#7313=CARTESIAN_POINT ( 'NONE',  ( 784.1219089521767955, -405.2817908451522158, -315.0488828828318333 ) ) ;
#7314=CARTESIAN_POINT ( 'NONE',  ( 774.6858677611749044, -369.7255117493284615, -315.5713283507209894 ) ) ;
#7315=CARTESIAN_POINT ( 'NONE',  ( 771.3260364891663130, -163.6454272087893003, -306.0683387631859773 ) ) ;
#7318=DIRECTION ( 'NONE',  ( -0.000000000000000000, -1.110223024625155554E-15, -1.000000000000000000 ) ) ;
#7319=CARTESIAN_POINT ( 'NONE',  ( 770.0799878456142551, -301.9874144716867477, -362.9823548866085616 ) ) ;
#7321=CARTESIAN_POINT ( 'NONE',  ( 804.1009440267234822, -191.4636090269709996, -314.0944755984392600 ) ) ;
#7326=CARTESIAN_POINT ( 'NONE',  ( 796.7737145352015204, -212.6346026584198796, -370.7187646348536987 ) ) ;
#7330=CARTESIAN_POINT ( 'NONE',  ( 810.1134526219336749, -80.53286901714194812, -357.8822607201570349 ) ) ;
#7332=CARTESIAN_POINT ( 'NONE',  ( 804.7487373415286811, -355.5436935675103882, -364.7487373415288516 ) ) ;
#7337=CARTESIAN_POINT ( 'NONE',  ( 746.0683387631852383, -427.4419599262317888, -331.3260364891676204 ) ) ;
#7338=CARTESIAN_POINT ( 'NONE',  ( 745.7998596910086917, -437.3618753856919170, -332.5602148656461168 ) ) ;
#7342=CARTESIAN_POINT ( 'NONE',  ( 744.9990715423526808, -186.3510508353234343, -341.2370466360926002 ) ) ;
#7348=CARTESIAN_POINT ( 'NONE',  ( 754.9967657858570647, -49.54369356751129061, -365.0032342141425374 ) ) ;
#7351=CARTESIAN_POINT ( 'NONE',  ( 815.3608509340175488, -458.7363362996973706, -341.2497674668889545 ) ) ;
#7356=CARTESIAN_POINT ( 'NONE',  ( 791.9812246680005501, -308.6346026584195670, -361.9419747391813189 ) ) ;
#7360=CARTESIAN_POINT ( 'NONE',  ( 760.7433823573367135, -300.0090635724252479, -355.9930595647440441 ) ) ;
#7361=CARTESIAN_POINT ( 'NONE',  ( 755.0636971347428243, -244.2709662947834204, -341.7834795799807353 ) ) ;
#7362=CARTESIAN_POINT ( 'NONE',  ( 791.9812246680005501, -452.6346026584191691, -361.9419747391813189 ) ) ;
#7363=CARTESIAN_POINT ( 'NONE',  ( 791.9812246680005501, -116.6346026584201780, -361.9419747391813189 ) ) ;
#7368=CARTESIAN_POINT ( 'NONE',  ( 747.6481478633932056, -37.09997266333514432, -353.4146539503763620 ) ) ;
#7374=CARTESIAN_POINT ( 'NONE',  ( 773.4516893846965786, -19.64542720878974791, -315.8398074228977066 ) ) ;
#7375=CARTESIAN_POINT ( 'NONE',  ( 801.1904061080338124, -92.08914811296570235, -368.3070685750236066 ) ) ;
#7377=FACE_OUTER_BOUND ( 'NONE', #8364, .T. ) ;
#7379=CARTESIAN_POINT ( 'NONE',  ( 767.6429770376289525, -225.1800572038743269, -306.8695393053162093 ) ) ;
#7383=CARTESIAN_POINT ( 'NONE',  ( 805.9055244015594326, -291.6237781080503169, -315.8990559732753240 ) ) ;
#7385=CARTESIAN_POINT ( 'NONE',  ( 767.6429770376289525, -321.1800572038740142, -306.8695393053162093 ) ) ;
#7389=CARTESIAN_POINT ( 'NONE',  ( 791.9812246680005501, -404.6346026584193396, -361.9419747391813189 ) ) ;
#7391=CARTESIAN_POINT ( 'NONE',  ( 797.8594530101008786, -205.5436935675108430, -322.1405469898980982 ) ) ;
#7392=CARTESIAN_POINT ( 'NONE',  ( 746.7653713866222915, -89.26014174441463922, -351.0478386215610271 ) ) ;
#7397=CARTESIAN_POINT ( 'NONE',  ( 758.6633372737375112, -188.5328690171416497, -326.9102291470432533 ) ) ;
#7399=EDGE_CURVE ( 'NONE', #9202, #38196, #44623, .T. ) ;
#7400=CARTESIAN_POINT ( 'NONE',  ( 746.7653713866222915, -17.26014174441486659, -351.0478386215610271 ) ) ;
#7406=CARTESIAN_POINT ( 'NONE',  ( 814.4686193811664907, -339.2817908451524431, -346.2056067578752732 ) ) ;
#7409=CARTESIAN_POINT ( 'NONE',  ( 766.9102291470427417, -162.5545181178802352, -318.6633372737382501 ) ) ;
#7410=CARTESIAN_POINT ( 'NONE',  ( 756.3353852180819104, -149.9073299311473875, -331.1735550268788302 ) ) ;
#7411=CARTESIAN_POINT ( 'NONE',  ( 788.8264449731201466, -357.1800572038739574, -363.6646147819170665 ) ) ;
#7422=CARTESIAN_POINT ( 'NONE',  ( 773.7305795820266212, -369.2817908451523294, -374.8230680027170365 ) ) ;
#7423=CARTESIAN_POINT ( 'NONE',  ( 805.0032342141413437, -13.54369356751140963, -314.9967657858572352 ) ) ;
#7426=CARTESIAN_POINT ( 'NONE',  ( 785.3687786644884454, -347.3618753856922012, -315.3201227861279676 ) ) ;
#7428=CARTESIAN_POINT ( 'NONE',  ( 799.9999999999993179, -462.9681489794448339, -309.9999999999998863 ) ) ;
#7429=CARTESIAN_POINT ( 'NONE',  ( 779.4763451958990572, -224.7363362996982232, -365.0264073115438919 ) ) ;
#7433=CARTESIAN_POINT ( 'NONE',  ( 772.4837098697145166, -431.3618753856918602, -374.5518280994205611 ) ) ;
#7436=CARTESIAN_POINT ( 'NONE',  ( 759.9999999999992042, 205.0000000000000568, -350.0000000000000000 ) ) ;
#7438=CARTESIAN_POINT ( 'NONE',  ( 810.7187646348534145, -66.45278447660216159, -356.7737145352016341 ) ) ;
#7439=CARTESIAN_POINT ( 'NONE',  ( 765.0180583372156207, -288.9982390220559978, -360.0135310231089534 ) ) ;
#7441=CARTESIAN_POINT ( 'NONE',  ( 799.9999999999993179, 205.0000000000000568, -339.9999999999999432 ) ) ;
#7444=CARTESIAN_POINT ( 'NONE',  ( 778.7629533639073998, -56.73633629969872771, -375.0009284576466371 ) ) ;
#7445=CARTESIAN_POINT ( 'NONE',  ( 779.4709603349208464, -72.35105083532378956, -314.7162404726379918 ) ) ;
#7449=CARTESIAN_POINT ( 'NONE',  ( 794.9819416627830151, 11.00176097794305541, -319.9864689768909898 ) ) ;
#7451=CARTESIAN_POINT ( 'NONE',  ( 785.3687786644884454, -83.36187538569296862, -315.3201227861279676 ) ) ;
#7453=CARTESIAN_POINT ( 'NONE',  ( 780.5290396650775619, -396.3510508353228374, -365.2837595273619513 ) ) ;
#7457=CARTESIAN_POINT ( 'NONE',  ( 815.1787889125755555, -414.8965053807771710, -343.7953271457877804 ) ) ;
#7462=CARTESIAN_POINT ( 'NONE',  ( 749.2812353651451076, -246.4527844766016074, -323.2262854647983090 ) ) ;
#7467=CARTESIAN_POINT ( 'NONE',  ( 763.8424801807145741, -42.00906357242603661, -320.5453621957614700 ) ) ;
#7468=CARTESIAN_POINT ( 'NONE',  ( 778.2165204200184689, -262.8164208402379245, -364.9363028652563230 ) ) ;
#7471=CARTESIAN_POINT ( 'NONE',  ( 800.0135310231082713, -374.0891481129647786, -325.0180583372163028 ) ) ;
#7472=CARTESIAN_POINT ( 'NONE',  ( 794.9819416627830151, -12.99823902205686821, -319.9864689768909898 ) ) ;
#7479=CARTESIAN_POINT ( 'NONE',  ( 785.3141322388236176, -21.72551174932956641, -364.4286716492789537 ) ) ;
#7480=DIRECTION ( 'NONE',  ( 0.9164815115825496461, 0.1263042864341401839, 0.3796167358741286413 ) ) ;
#7483=CARTESIAN_POINT ( 'NONE',  ( 762.1177392798416577, -282.5545181178798657, -309.8865473780659272 ) ) ;
#7486=CARTESIAN_POINT ( 'NONE',  ( 764.8639956371174549, -272.0891481129651197, -319.7806653035542013 ) ) ;
#7488=CARTESIAN_POINT ( 'NONE',  ( 755.1538015810308480, -134.1908817542439181, -343.0433043558613804 ) ) ;
#7490=CARTESIAN_POINT ( 'NONE',  ( 776.2433038121456548, 11.10349461922141145, -374.8207195650711014 ) ) ;
#7491=CARTESIAN_POINT ( 'NONE',  ( 811.0346526505617248, -326.6346026584194533, -323.0537975583478101 ) ) ;
#7496=CARTESIAN_POINT ( 'NONE',  ( 807.5423716828161105, -201.0783235625961254, -362.2119215644372048 ) ) ;
#7498=CARTESIAN_POINT ( 'NONE',  ( 792.3570229623688874, -429.1800572038737869, -373.1304606946836202 ) ) ;
#7500=EDGE_CURVE ( 'NONE', #31261, #22826, #5540, .T. ) ;
#7504=CARTESIAN_POINT ( 'NONE',  ( 804.6798772138708955, -447.7255117493280636, -334.6312213355107019 ) ) ;
#7511=CARTESIAN_POINT ( 'NONE',  ( 801.3366627262608972, -296.5328690171411949, -353.0897708529566899 ) ) ;
#7513=CARTESIAN_POINT ( 'NONE',  ( 761.9338519418445230, -302.5328690171411949, -370.4231160770881957 ) ) ;
#7518=CARTESIAN_POINT ( 'NONE',  ( 758.6633372737375112, -92.53286901714190549, -326.9102291470432533 ) ) ;
#7519=CARTESIAN_POINT ( 'NONE',  ( 754.8072714833581358, -148.8164208402382656, -338.1981804954720587 ) ) ;
#7520=CARTESIAN_POINT ( 'NONE',  ( 805.1927285166397041, -208.8164208402380666, -341.8018195045277707 ) ) ;
#7522=CARTESIAN_POINT ( 'NONE',  ( 814.2001403089898304, -161.3618753856927697, -347.4397851343538264 ) ) ;
#7525=CARTESIAN_POINT ( 'NONE',  ( 754.8072714833583632, -148.8164208402382656, -338.1981804954721156 ) ) ;
#7527=CARTESIAN_POINT ( 'NONE',  ( 793.9708237608222134, -406.9181544815157849, -319.2295555964448681 ) ) ;
#7534=CARTESIAN_POINT ( 'NONE',  ( 793.9708237608222134, -382.9181544815159555, -319.2295555964448681 ) ) ;
#7536=CARTESIAN_POINT ( 'NONE',  ( 746.4236121716829757, -183.8272453906074020, -328.8385539511384650 ) ) ;
#7539=CARTESIAN_POINT ( 'NONE',  ( 787.4999999999992042, -462.9681489794447771, -310.9526249034443026 ) ) ;
#7540=CARTESIAN_POINT ( 'NONE',  ( 754.9735926884551418, -306.3510508353230648, -340.5236548041000333 ) ) ;
#7542=CARTESIAN_POINT ( 'NONE',  ( 766.4474001241216001, -187.0999726633346825, -307.3154664389482491 ) ) ;
#7547=CARTESIAN_POINT ( 'NONE',  ( 755.2512626584698410, -223.5436935675107577, -315.2512626584710915 ) ) ;
#7548=PLANE ( 'NONE',  #29072 ) ;
#7549=CARTESIAN_POINT ( 'NONE',  ( 764.8639956371174549, 15.91085188703394238, -319.7806653035542013 ) ) ;
#7552=CARTESIAN_POINT ( 'NONE',  ( 803.8556311672234642, -81.62377810805104161, -365.6418435158340117 ) ) ;
#7554=CARTESIAN_POINT ( 'NONE',  ( 801.1904061080336987, -356.0891481129647218, -368.3070685750235498 ) ) ;
#7560=CARTESIAN_POINT ( 'NONE',  ( 748.3538107759620743, -400.7146871989590977, -355.8262568251490165 ) ) ;
#7561=CARTESIAN_POINT ( 'NONE',  ( 744.7301800767019131, -412.8164208402372992, -337.4774526936615757 ) ) ;
#7566=CARTESIAN_POINT ( 'NONE',  ( 745.1769319972822814, -185.8055962898689302, -346.2694204179732083 ) ) ;
#7572=CARTESIAN_POINT ( 'NONE',  ( 746.8695393053150156, -29.90732993114771787, -327.6429770376306010 ) ) ;
#7576=CARTESIAN_POINT ( 'NONE',  ( 814.8207195650702488, -458.1908817542429802, -336.2433038121456548 ) ) ;
#7577=ORIENTED_EDGE ( 'NONE', *, *, #22046, .F. ) ;
#7580=CARTESIAN_POINT ( 'NONE',  ( 754.8072714833581358, -292.8164208402376971, -338.1981804954720587 ) ) ;
#7584=CARTESIAN_POINT ( 'NONE',  ( 757.0176451133909268, -277.0999726633344267, -349.9200121543848354 ) ) ;
#7585=CARTESIAN_POINT ( 'NONE',  ( 804.6798772138708955, -303.7255117493287457, -334.6312213355107019 ) ) ;
#7586=CARTESIAN_POINT ( 'NONE',  ( 791.0208441182601291, -452.8006503659887585, -362.4663821942984328 ) ) ;
#7587=CARTESIAN_POINT ( 'NONE',  ( 797.8594530101008786, -133.5436935675110135, -322.1405469898980982 ) ) ;
#7592=CARTESIAN_POINT ( 'NONE',  ( 809.0717654672305343, -76.91815448151683654, -360.1688906516309885 ) ) ;
#7598=CARTESIAN_POINT ( 'NONE',  ( 757.0176451133909268, -37.09997266333514432, -349.9200121543848354 ) ) ;
#7599=CARTESIAN_POINT ( 'NONE',  ( 777.5031285880264704, -118.8164208402383508, -374.9108240113588408 ) ) ;
#7603=CARTESIAN_POINT ( 'NONE',  ( 800.9747183278959710, -228.9982390220561683, -311.9810565676471583 ) ) ;
#7607=CARTESIAN_POINT ( 'NONE',  ( 766.5853460496234675, -301.9874144716867477, -372.3518521366060554 ) ) ;
#7610=CARTESIAN_POINT ( 'NONE',  ( 755.2512626584698410, -319.5436935675104451, -315.2512626584710915 ) ) ;
#7614=CARTESIAN_POINT ( 'NONE',  ( 778.2165204200184689, -406.8164208402375266, -364.9363028652563230 ) ) ;
#7616=CARTESIAN_POINT ( 'NONE',  ( 755.3201227861273992, -195.7255117493289731, -345.3687786644892981 ) ) ;
#7617=CARTESIAN_POINT ( 'NONE',  ( 810.1134526219336749, -80.53286901714194812, -357.8822607201570349 ) ) ;
#7621=CARTESIAN_POINT ( 'NONE',  ( 755.8398074228967971, -211.4419599262324709, -333.4516893846970333 ) ) ;
#7623=CARTESIAN_POINT ( 'NONE',  ( 773.7943932421234194, -23.80559628986938847, -305.5313806188329409 ) ) ;
#7625=CARTESIAN_POINT ( 'NONE',  ( 801.0087853405226497, -452.9681489794447202, -354.4092604580203556 ) ) ;
#7629=CARTESIAN_POINT ( 'NONE',  ( 745.5313806188320314, -327.2817908451525000, -333.7943932421247268 ) ) ;
#7632=CARTESIAN_POINT ( 'NONE',  ( 755.3028492785439312, -183.2817908451528695, -335.9200461376539693 ) ) ;
#7633=CARTESIAN_POINT ( 'NONE',  ( 755.0636971347428243, -172.2709662947836478, -341.7834795799807353 ) ) ;
#7635=CARTESIAN_POINT ( 'NONE',  ( 771.1735550268780344, -345.1800572038739574, -316.3353852180828198 ) ) ;
#7638=CARTESIAN_POINT ( 'NONE',  ( 759.2295555964440155, 7.830767346494148740, -353.9708237608231229 ) ) ;
#7645=CARTESIAN_POINT ( 'NONE',  ( 754.3581564841646241, -425.4636090269703459, -316.1443688327762516 ) ) ;
#7646=CARTESIAN_POINT ( 'NONE',  ( 745.7998596910086917, -5.361875385693257279, -332.5602148656461168 ) ) ;
#7649=CARTESIAN_POINT ( 'NONE',  ( 797.6776695296629214, -355.5436935675103882, -357.6776695296636603 ) ) ;
#7653=CARTESIAN_POINT ( 'NONE',  ( 757.0176451133909268, -229.0999726633345404, -349.9200121543848354 ) ) ;
#7663=CARTESIAN_POINT ( 'NONE',  ( 758.8095938919642549, -104.0891481129656881, -311.6929314249763365 ) ) ;
#7664=CARTESIAN_POINT ( 'NONE',  ( 785.3687786644884454, -299.3618753856922581, -315.3201227861279676 ) ) ;
#7669=CARTESIAN_POINT ( 'NONE',  ( 783.7953271457878373, -56.19088175424417386, -375.1787889125761239 ) ) ;
#7670=CARTESIAN_POINT ( 'NONE',  ( 790.8726784830453198, -82.71468719896012090, -362.5472867521010585 ) ) ;
#7673=CARTESIAN_POINT ( 'NONE',  ( 755.3201227861273992, -3.725511749329622813, -345.3687786644892981 ) ) ;
#7674=CARTESIAN_POINT ( 'NONE',  ( 780.5290396650775619, -108.3510508353236759, -365.2837595273619513 ) ) ;
#7676=CARTESIAN_POINT ( 'NONE',  ( 781.7834795799800531, -82.81642084023846451, -315.0636971347436202 ) ) ;
#7677=CARTESIAN_POINT ( 'NONE',  ( 803.8651313633788504, -413.2601417444136018, -332.4468031744301015 ) ) ;
#7681=CARTESIAN_POINT ( 'NONE',  ( 778.7502325331095108, -408.3510508353227806, -304.6391490659818828 ) ) ;
#7687=CARTESIAN_POINT ( 'NONE',  ( 777.5031285880264704, -238.8164208402379813, -374.9108240113588408 ) ) ;
#7691=CARTESIAN_POINT ( 'NONE',  ( 755.3028492785439312, -63.28179084515324604, -335.9200461376539693 ) ) ;
#7692=CARTESIAN_POINT ( 'NONE',  ( 788.8264449731201466, -261.1800572038742416, -363.6646147819170665 ) ) ;
#7694=CARTESIAN_POINT ( 'NONE',  ( 756.5762568750052424, -387.1800572038738437, -348.7366044899774238 ) ) ;
#7695=CARTESIAN_POINT ( 'NONE',  ( 788.7366044899766848, -59.90732993114762905, -316.5762568750059813 ) ) ;
#7701=CARTESIAN_POINT ( 'NONE',  ( 758.0580252608178853, -6.452784476602343666, -328.0187753319985404 ) ) ;
#7704=( GEOMETRIC_REPRESENTATION_CONTEXT ( 3 ) GLOBAL_UNCERTAINTY_ASSIGNED_CONTEXT ( ( #39382 ) ) GLOBAL_UNIT_ASSIGNED_CONTEXT ( ( #6539, #17854, #42788 ) ) REPRESENTATION_CONTEXT ( 'NONE', 'WORKASPACE' ) );
#7706=CARTESIAN_POINT ( 'NONE',  ( 762.1177392798416577, -306.5545181178797520, -309.8865473780659272 ) ) ;
#7709=CARTESIAN_POINT ( 'NONE',  ( 801.9419747391806368, -258.4527844766016074, -351.9812246680014027 ) ) ;
#7711=CARTESIAN_POINT ( 'NONE',  ( 801.5560724626406000, -120.5545181178803205, -326.7756240680316182 ) ) ;
#7714=CARTESIAN_POINT ( 'NONE',  ( 805.0032342141413437, -325.5436935675104451, -314.9967657858572352 ) ) ;
#7717=VECTOR ( 'NONE', #28869, 1000.000000000000000 ) ;
#7719=CARTESIAN_POINT ( 'NONE',  ( 764.3348316497523456, -214.7146871989597230, -308.6759233522265617 ) ) ;
#7721=CARTESIAN_POINT ( 'NONE',  ( 804.7487373415286811, -427.5436935675101040, -364.7487373415288516 ) ) ;
#7727=CARTESIAN_POINT ( 'NONE',  ( 803.2186876482843445, 16.01258552831230375, -350.0220218866286928 ) ) ;
#7735=CARTESIAN_POINT ( 'NONE',  ( 773.3843516231979720, -277.4419599262322436, -364.4086373105754433 ) ) ;
#7738=CARTESIAN_POINT ( 'NONE',  ( 744.9990715423526808, -282.3510508353230080, -341.2370466360926002 ) ) ;
#7744=CARTESIAN_POINT ( 'NONE',  ( 754.8983024940795303, -66.89650538077835051, -336.9254006560228163 ) ) ;
#7746=CARTESIAN_POINT ( 'NONE',  ( 813.1304606946830518, -137.9073299311473875, -352.3570229623690580 ) ) ;
#7748=CARTESIAN_POINT ( 'NONE',  ( 781.7834795799800531, -130.8164208402383224, -315.0636971347436202 ) ) ;
#7750=CARTESIAN_POINT ( 'NONE',  ( 755.1538015810308480, -422.1908817542430370, -343.0433043558613804 ) ) ;
#7754=DIRECTION ( 'NONE',  ( 0.000000000000000000, 0.000000000000000000, 1.000000000000000000 ) ) ;
#7761=CARTESIAN_POINT ( 'NONE',  ( 766.9102291470427417, -378.5545181178795247, -318.6633372737382501 ) ) ;
#7763=CARTESIAN_POINT ( 'NONE',  ( 778.7629533639073998, -176.7363362996983369, -375.0009284576466371 ) ) ;
#7767=CARTESIAN_POINT ( 'NONE',  ( 794.1144889064781864, -322.1692326535048210, -360.9840315886528401 ) ) ;
#7769=CARTESIAN_POINT ( 'NONE',  ( 802.2119215644370342, -198.0090635724255606, -367.5423716828165084 ) ) ;
#7777=VECTOR ( 'NONE', #9489, 1000.000000000000000 ) ;
#7778=CARTESIAN_POINT ( 'NONE',  ( 744.7301800767020268, -220.8164208402380098, -337.4774526936615189 ) ) ;
#7780=CARTESIAN_POINT ( 'NONE',  ( 762.3223304703356007, -31.54369356751135456, -322.3223304703362828 ) ) ;
#7783=CARTESIAN_POINT ( 'NONE',  ( 788.7631598425961101, -97.44195992623281199, -305.7194118038759143 ) ) ;
#7785=CARTESIAN_POINT ( 'NONE',  ( 746.8695393053150156, -341.9073299311465917, -327.6429770376306010 ) ) ;
#7792=CARTESIAN_POINT ( 'NONE',  ( 793.4146539503750546, -409.9874144716863498, -307.6481478633938877 ) ) ;
#7794=CARTESIAN_POINT ( 'NONE',  ( 745.0891759886404770, -412.2709662947829088, -342.4968714119734159 ) ) ;
#7796=EDGE_CURVE ( 'NONE', #33292, #15749, #21734, .T. ) ;
#7800=CARTESIAN_POINT ( 'NONE',  ( 805.0264073115434940, -174.3510508353234627, -339.4763451958999099 ) ) ;
#7802=CARTESIAN_POINT ( 'NONE',  ( 795.6651683502461765, -202.7146871989597514, -371.3240766477733814 ) ) ;
#7808=CARTESIAN_POINT ( 'NONE',  ( 792.3570229623688874, -45.18005720387493085, -373.1304606946836202 ) ) ;
#7812=CARTESIAN_POINT ( 'NONE',  ( 813.5763878283155464, -435.8272453906066062, -351.1614460488615350 ) ) ;
#7819=CARTESIAN_POINT ( 'NONE',  ( 762.3223304703356007, -295.5436935675105588, -322.3223304703362828 ) ) ;
#7824=CARTESIAN_POINT ( 'NONE',  ( 757.4527132478984868, -304.3726999360615082, -329.1273215169538844 ) ) ;
#7825=CARTESIAN_POINT ( 'NONE',  ( 788.8264449731200330, -285.1800572038740711, -363.6646147819171233 ) ) ;
#7827=CARTESIAN_POINT ( 'NONE',  ( 785.3141322388236176, -117.7255117493292715, -364.4286716492789537 ) ) ;
#7834=CARTESIAN_POINT ( 'NONE',  ( 757.7880784355613741, -90.00906357242590161, -312.4576283171834916 ) ) ;
#7842=CARTESIAN_POINT ( 'NONE',  ( 751.9810565676468741, -98.08914811296568814, -360.9747183278973921 ) ) ;
#7846=CARTESIAN_POINT ( 'NONE',  ( 777.5031285880264704, -238.8164208402379813, -374.9108240113588408 ) ) ;
#7850=CARTESIAN_POINT ( 'NONE',  ( 808.7758568127978833, -292.1692326535048210, -320.0363995740631822 ) ) ;
#7853=CARTESIAN_POINT ( 'NONE',  ( 767.7687537140311633, -311.9073299311468759, -372.7932403749916830 ) ) ;
#7857=CYLINDRICAL_SURFACE ( 'NONE', #36491, 10.00000000000000888 ) ;
#7858=CARTESIAN_POINT ( 'NONE',  ( 802.1676090361156639, -422.6346026584192259, -327.8955696845344505 ) ) ;
#7860=CARTESIAN_POINT ( 'NONE',  ( 792.1044303154645831, -204.4527844766016926, -317.8323909638837677 ) ) ;
#7861=CARTESIAN_POINT ( 'NONE',  ( 768.8385539511368734, -95.26014174441461080, -306.4236121716840557 ) ) ;
#7866=CARTESIAN_POINT ( 'NONE',  ( 798.7617431975189675, -219.6237781080506295, -323.0428371773161871 ) ) ;
#7868=AXIS2_PLACEMENT_3D ( 'NONE', #25863, #32580, #39973 ) ;
#7869=CARTESIAN_POINT ( 'NONE',  ( 786.2056067578752163, -35.80559628986934229, -374.4686193811670023 ) ) ;
#7875=CARTESIAN_POINT ( 'NONE',  ( 745.7194118038753459, -325.6454272087888739, -348.7631598425976449 ) ) ;
#7879=CARTESIAN_POINT ( 'NONE',  ( 787.5531968255692163, -189.8272453906073736, -316.1348686366205811 ) ) ;
#7880=CARTESIAN_POINT ( 'NONE',  ( 785.3141322388236176, -189.7255117493290300, -364.4286716492789537 ) ) ;
#7881=CARTESIAN_POINT ( 'NONE',  ( 762.3223304703356007, -343.5436935675103314, -322.3223304703362828 ) ) ;
#7883=CARTESIAN_POINT ( 'NONE',  ( 803.2186876482843445, 16.01258552831230375, -350.0220218866286928 ) ) ;
#7884=AXIS2_PLACEMENT_3D ( 'NONE', #198, #20351, #41162 ) ;
#7893=CARTESIAN_POINT ( 'NONE',  ( 745.5313806188320314, -399.2817908451522726, -333.7943932421247268 ) ) ;
#7894=VECTOR ( 'NONE', #5246, 1000.000000000000000 ) ;
#7895=CARTESIAN_POINT ( 'NONE',  ( 745.0891759886404770, -4.270966294784170003, -342.4968714119734159 ) ) ;
#7899=CARTESIAN_POINT ( 'NONE',  ( 785.3141322388236176, -357.7255117493285184, -364.4286716492789537 ) ) ;
#7903=CARTESIAN_POINT ( 'NONE',  ( 755.5913626894240451, -253.6454272087889876, -346.6156483768012890 ) ) ;
#7910=CARTESIAN_POINT ( 'NONE',  ( 772.4999999999993179, -462.9681489794447771, -309.9999999999998863 ) ) ;
#7912=CARTESIAN_POINT ( 'NONE',  ( 792.1044303154645831, -324.4527844766013231, -317.8323909638837677 ) ) ;
#7916=CARTESIAN_POINT ( 'NONE',  ( 747.6481478633932056, -61.09997266333506616, -353.4146539503763620 ) ) ;
#7917=CARTESIAN_POINT ( 'NONE',  ( 754.8983024940795303, -90.89650538077827946, -336.9254006560228163 ) ) ;
#7920=CARTESIAN_POINT ( 'NONE',  ( 801.9419747391806368, 5.547215523397618142, -351.9812246680014027 ) ) ;
#7921=CARTESIAN_POINT ( 'NONE',  ( 805.0264073115434940, -126.3510508353236048, -339.4763451958999099 ) ) ;
#7923=CARTESIAN_POINT ( 'NONE',  ( 794.9819416627830151, -108.9982390220565804, -319.9864689768909898 ) ) ;
#7925=CARTESIAN_POINT ( 'NONE',  ( 772.3691319403857278, -383.2601417444137155, -315.8894580844506663 ) ) ;
#7931=VECTOR ( 'NONE', #4043, 1000.000000000000000 ) ;
#7938=CARTESIAN_POINT ( 'NONE',  ( 773.4516893846965786, -67.64542720878958448, -315.8398074228977066 ) ) ;
#7940=CARTESIAN_POINT ( 'NONE',  ( 800.0135310231082713, -254.0891481129652334, -325.0180583372163028 ) ) ;
#7942=CARTESIAN_POINT ( 'NONE',  ( 755.3201227861273992, -387.7255117493283478, -345.3687786644892981 ) ) ;
#7943=CARTESIAN_POINT ( 'NONE',  ( 778.1981804954714335, -58.27096629478398171, -314.8072714833589885 ) ) ;
#7947=CARTESIAN_POINT ( 'NONE',  ( 755.0636971347428243, -28.27096629478409540, -341.7834795799807353 ) ) ;
#7950=CARTESIAN_POINT ( 'NONE',  ( 750.9282345327678740, -304.9181544815161828, -319.8311093483690115 ) ) ;
#7953=CARTESIAN_POINT ( 'NONE',  ( 788.7366044899766848, -251.9073299311470748, -316.5762568750059813 ) ) ;
#7955=CARTESIAN_POINT ( 'NONE',  ( 783.0745993439762742, -152.1908817542438612, -365.1016975059196739 ) ) ;
#7958=CARTESIAN_POINT ( 'NONE',  ( 747.3154664389472828, -19.98741447168758256, -326.4474001241230781 ) ) ;
#7959=CARTESIAN_POINT ( 'NONE',  ( 808.3070685750232087, -354.9982390220557136, -361.1904061080339829 ) ) ;
#7964=CARTESIAN_POINT ( 'NONE',  ( 800.1688906516307043, -250.1692326535050199, -369.0717654672308186 ) ) ;
#7966=CARTESIAN_POINT ( 'NONE',  ( 811.6461892240364477, -436.7146871989589272, -324.1737431748509835 ) ) ;
#7968=EDGE_LOOP ( 'NONE', ( #7577, #15368 ) ) ;
#7971=CARTESIAN_POINT ( 'NONE',  ( 791.9812246680005501, -452.6346026584191691, -361.9419747391813189 ) ) ;
#7972=LINE ( 'NONE', #107, #4104 ) ;
#7977=CARTESIAN_POINT ( 'NONE',  ( 755.0488828828309806, -305.8055962898684470, -344.1219089521771934 ) ) ;
#7980=CARTESIAN_POINT ( 'NONE',  ( 798.0661480581538854, -338.5328690171411381, -309.5768839229118043 ) ) ;
#7986=CARTESIAN_POINT ( 'NONE',  ( 769.1273215169530886, -94.71468719896007826, -317.4527132478988847 ) ) ;
#7988=EDGE_CURVE ( 'NONE', #23858, #41096, #22873, .T. ) ;
#7989=CARTESIAN_POINT ( 'NONE',  ( 814.5518280994195948, -135.7255117493291152, -332.4837098697145734 ) ) ;
#7991=CARTESIAN_POINT ( 'NONE',  ( 800.0135310231082713, -158.0891481129655176, -325.0180583372163028 ) ) ;
#7993=CARTESIAN_POINT ( 'NONE',  ( 769.9779781133707957, -427.0999726633338582, -316.7813123517150871 ) ) ;
#8001=CARTESIAN_POINT ( 'NONE',  ( 787.5531968255692163, -405.8272453906067199, -316.1348686366205811 ) ) ;
#8003=CARTESIAN_POINT ( 'NONE',  ( 744.6391490659812007, -206.7363362996982801, -338.7502325331110455 ) ) ;
#8007=CARTESIAN_POINT ( 'NONE',  ( 754.9735926884551418, -330.3510508353229511, -340.5236548041000333 ) ) ;
#8009=CARTESIAN_POINT ( 'NONE',  ( 755.8990559732751535, -179.4636090269710849, -365.9055244015606831 ) ) ;
#8012=CARTESIAN_POINT ( 'NONE',  ( 805.0032342141413437, -229.5436935675107009, -314.9967657858572352 ) ) ;
#8014=CARTESIAN_POINT ( 'NONE',  ( 768.0187753319979720, -8.634602658420517329, -318.0580252608186242 ) ) ;
#8016=CARTESIAN_POINT ( 'NONE',  ( 812.6845335610512393, -103.9874144716873161, -353.5525998758768651 ) ) ;
#8018=CARTESIAN_POINT ( 'NONE',  ( 763.0537975583475827, -360.4527844766010958, -371.0346526505627480 ) ) ;
#8023=CARTESIAN_POINT ( 'NONE',  ( 758.0141637701419768, -423.0783235625953580, -367.2620300519063790 ) ) ;
#8025=CARTESIAN_POINT ( 'NONE',  ( 786.2694204179717872, 2.718209154846545683, -305.1769319972829067 ) ) ;
#8028=ORIENTED_EDGE ( 'NONE', *, *, #38258, .T. ) ;
#8030=CARTESIAN_POINT ( 'NONE',  ( 755.0488828828309806, -185.8055962898689302, -344.1219089521771934 ) ) ;
#8032=CARTESIAN_POINT ( 'NONE',  ( 786.2056067578752163, -203.8055962898688449, -374.4686193811670023 ) ) ;
#8038=CARTESIAN_POINT ( 'NONE',  ( 795.1360043628807261, -140.0891481129654892, -360.2193346964456282 ) ) ;
#8041=CARTESIAN_POINT ( 'NONE',  ( 751.6929314249748586, -54.99823902205672255, -318.8095938919659034 ) ) ;
#8043=CARTESIAN_POINT ( 'NONE',  ( 804.1009440267234822, -455.4636090269701754, -314.0944755984392600 ) ) ;
#8045=CARTESIAN_POINT ( 'NONE',  ( 760.7433823573367135, -324.0090635724251911, -355.9930595647440441 ) ) ;
#8049=CARTESIAN_POINT ( 'NONE',  ( 804.4286716492782716, -305.3618753856922581, -345.3141322388244703 ) ) ;
#8052=CARTESIAN_POINT ( 'NONE',  ( 804.4086373105744769, -289.6454272087889308, -333.3843516231986541 ) ) ;
#8053=CARTESIAN_POINT ( 'NONE',  ( 767.8955696845333705, -288.4527844766014937, -362.1676090361162323 ) ) ;
#8055=CARTESIAN_POINT ( 'NONE',  ( 797.6776695296629214, -163.5436935675109567, -357.6776695296636603 ) ) ;
#8062=CARTESIAN_POINT ( 'NONE',  ( 779.9999999999992042, 16.45630643248849267, -370.0000000000000568 ) ) ;
#8064=CARTESIAN_POINT ( 'NONE',  ( 786.2694204179717872, -93.28179084515315367, -305.1769319972829067 ) ) ;
#8065=FACE_OUTER_BOUND ( 'NONE', #29938, .T. ) ;
#8070=CARTESIAN_POINT ( 'NONE',  ( 805.0032342141413437, -109.5436935675110988, -314.9967657858572352 ) ) ;
#8074=CARTESIAN_POINT ( 'NONE',  ( 763.2262854647970016, -248.6346026584197659, -309.2812353651462445 ) ) ;
#8078=CARTESIAN_POINT ( 'NONE',  ( 788.7631598425961101, -313.4419599262320730, -305.7194118038759143 ) ) ;
#8079=EDGE_CURVE ( 'NONE', #9510, #36235, #3355, .T. ) ;
#8081=CARTESIAN_POINT ( 'NONE',  ( 800.9747183278959710, -324.9982390220559409, -311.9810565676471583 ) ) ;
#8084=ORIENTED_EDGE ( 'NONE', *, *, #42226, .T. ) ;
#8085=CARTESIAN_POINT ( 'NONE',  ( 785.3141322388236176, -429.7255117493282910, -364.4286716492789537 ) ) ;
#8087=CARTESIAN_POINT ( 'NONE',  ( 791.9812246680005501, -212.6346026584198796, -361.9419747391813189 ) ) ;
#8088=CARTESIAN_POINT ( 'NONE',  ( 798.0661480581538854, -74.53286901714196233, -309.5768839229118043 ) ) ;
#8093=CARTESIAN_POINT ( 'NONE',  ( 766.7756240680305382, -230.5328690171415076, -361.5560724626415663 ) ) ;
#8097=CARTESIAN_POINT ( 'NONE',  ( 814.8230680027162407, -77.80559628986920018, -333.7305795820267917 ) ) ;
#8100=CARTESIAN_POINT ( 'NONE',  ( 813.5763878283155464, -339.8272453906069472, -351.1614460488615350 ) ) ;
#8104=CARTESIAN_POINT ( 'NONE',  ( 761.4292242960306112, -185.4636090269710280, -323.2154366446414429 ) ) ;
#8105=CARTESIAN_POINT ( 'NONE',  ( 797.8594530101008786, -181.5436935675108145, -322.1405469898980982 ) ) ;
#8106=CARTESIAN_POINT ( 'NONE',  ( 788.8264449731201466, -381.1800572038739006, -363.6646147819170665 ) ) ;
#8108=ORIENTED_EDGE ( 'NONE', *, *, #11198, .T. ) ;
#8117=CARTESIAN_POINT ( 'NONE',  ( 814.8207195650702488, -410.1908817542430370, -336.2433038121456548 ) ) ;
#8118=CARTESIAN_POINT ( 'NONE',  ( 808.3070685750232087, 5.001760977943074948, -361.1904061080339829 ) ) ;
#8121=CARTESIAN_POINT ( 'NONE',  ( 804.6798772138708955, -375.7255117493283478, -334.6312213355107019 ) ) ;
#8125=CARTESIAN_POINT ( 'NONE',  ( 772.4468031744293057, -249.8272453906072315, -363.8651313633793620 ) ) ;
#8134=CARTESIAN_POINT ( 'NONE',  ( 804.4286716492782716, -305.3618753856922581, -345.3141322388244703 ) ) ;
#8137=CARTESIAN_POINT ( 'NONE',  ( 757.7880784355613741, -66.00906357242595845, -312.4576283171834916 ) ) ;
#8138=CARTESIAN_POINT ( 'NONE',  ( 759.2295555964440155, -136.1692326535053894, -353.9708237608231229 ) ) ;
#8142=CARTESIAN_POINT ( 'NONE',  ( 785.3141322388236176, -45.72551174932949181, -364.4286716492789537 ) ) ;
#8143=CARTESIAN_POINT ( 'NONE',  ( 763.2154366446407039, -117.6237781080509279, -321.4292242960311228 ) ) ;
#8144=CARTESIAN_POINT ( 'NONE',  ( 792.1044303154645831, -84.45278447660206211, -317.8323909638837677 ) ) ;
#8145=CARTESIAN_POINT ( 'NONE',  ( 800.7704444035546203, -436.1692326535044231, -326.0291762391768771 ) ) ;
#8155=CARTESIAN_POINT ( 'NONE',  ( 766.9102291470427417, -66.55451811788050520, -318.6633372737382501 ) ) ;
#8157=CARTESIAN_POINT ( 'NONE',  ( 804.4286716492782716, -281.3618753856923718, -345.3141322388244703 ) ) ;
#8159=CARTESIAN_POINT ( 'NONE',  ( 759.9864689768902508, -386.0891481129647786, -354.9819416627836404 ) ) ;
#8160=CARTESIAN_POINT ( 'NONE',  ( 802.1676090361156639, -62.63460265842031305, -327.8955696845344505 ) ) ;
#8164=CARTESIAN_POINT ( 'NONE',  ( 773.7305795820266212, -9.281790845153418346, -374.8230680027170365 ) ) ;
#8166=ORIENTED_EDGE ( 'NONE', *, *, #28958, .F. ) ;
#8167=CARTESIAN_POINT ( 'NONE',  ( 748.6759233522253680, -304.3726999360615082, -324.3348316497537098 ) ) ;
#8170=CARTESIAN_POINT ( 'NONE',  ( 754.8072714833581358, -244.8164208402378961, -338.1981804954720587 ) ) ;
#8172=CARTESIAN_POINT ( 'NONE',  ( 804.6971507214547046, -147.2817908451529547, -344.0799538623459739 ) ) ;
#8173=CARTESIAN_POINT ( 'NONE',  ( 759.9999999999992042, 205.0000000000000568, -339.9999999999999432 ) ) ;
#8174=CARTESIAN_POINT ( 'NONE',  ( 745.4481719005789273, -363.7255117493284615, -347.5162901302853697 ) ) ;
#8178=CARTESIAN_POINT ( 'NONE',  ( 751.2241431872005251, -232.1692326535051620, -359.9636004259367610 ) ) ;
#8180=CARTESIAN_POINT ( 'NONE',  ( 813.1304606946830518, 6.092670068852159559, -352.3570229623690580 ) ) ;
#8182=EDGE_LOOP ( 'NONE', ( #43776, #31496, #4562, #45449 ) ) ;
#8185=CARTESIAN_POINT ( 'NONE',  ( 784.0799538623451781, -11.80559628986942577, -364.6971507214555572 ) ) ;
#8186=FACE_OUTER_BOUND ( 'NONE', #17296, .T. ) ;
#8191=CARTESIAN_POINT ( 'NONE',  ( 803.2186876482843445, -295.9874144716866908, -350.0220218866286928 ) ) ;
#8193=CARTESIAN_POINT ( 'NONE',  ( 766.5853460496234675, -325.9874144716865771, -372.3518521366060554 ) ) ;
#8198=CARTESIAN_POINT ( 'NONE',  ( 765.8855110935204493, -70.16923265350563099, -319.0159684113471599 ) ) ;
#8201=CARTESIAN_POINT ( 'NONE',  ( 805.0032342141412300, -181.5436935675108145, -314.9967657858571783 ) ) ;
#8202=VERTEX_POINT ( 'NONE', #13397 ) ;
#8203=CARTESIAN_POINT ( 'NONE',  ( 774.6312213355098493, -143.3618753856927697, -364.6798772138717482 ) ) ;
#8205=CARTESIAN_POINT ( 'NONE',  ( 758.4439275373578084, -420.5545181178793541, -353.2243759319684386 ) ) ;
#8210=DIRECTION ( 'NONE',  ( 0.000000000000000000, 0.000000000000000000, -1.000000000000000000 ) ) ;
#8212=CARTESIAN_POINT ( 'NONE',  ( 804.8461984189677878, -410.1908817542430370, -336.9566956441385628 ) ) ;
#8214=CARTESIAN_POINT ( 'NONE',  ( 791.0478386215596629, -213.8272453906073167, -306.7653713866226326 ) ) ;
#8218=CARTESIAN_POINT ( 'NONE',  ( 789.9200121543843807, -337.9874144716865771, -317.0176451133914384 ) ) ;
#8220=CARTESIAN_POINT ( 'NONE',  ( 760.0363995740630116, -178.9181544815165239, -368.7758568127991907 ) ) ;
#8221=CARTESIAN_POINT ( 'NONE',  ( 767.9999999999992042, 240.0000000000000853, -320.0000000000000000 ) ) ;
#8224=CARTESIAN_POINT ( 'NONE',  ( 812.7932403749906598, -255.1800572038742700, -327.7687537140311633 ) ) ;
#8227=CARTESIAN_POINT ( 'NONE',  ( 788.7366044899766848, -11.90732993114778182, -316.5762568750059813 ) ) ;
#8229=CARTESIAN_POINT ( 'NONE',  ( 793.4146539503750546, -145.9874144716871740, -307.6481478633938877 ) ) ;
#8231=CARTESIAN_POINT ( 'NONE',  ( 744.7301800767019131, -364.8164208402374697, -337.4774526936615757 ) ) ;
#8236=CARTESIAN_POINT ( 'NONE',  ( 800.2193346964447755, -378.9982390220555999, -355.1360043628815788 ) ) ;
#8237=CARTESIAN_POINT ( 'NONE',  ( 787.5162901302840055, -443.3618753856917465, -305.4481719005792684 ) ) ;
#8241=CARTESIAN_POINT ( 'NONE',  ( 780.5290396650775619, -204.3510508353233774, -365.2837595273619513 ) ) ;
#8244=CARTESIAN_POINT ( 'NONE',  ( 793.4146539503750546, -241.9874144716869182, -307.6481478633938877 ) ) ;
#8245=( NAMED_UNIT ( * ) SI_UNIT ( $, .STERADIAN. ) SOLID_ANGLE_UNIT ( ) );
#8249=CARTESIAN_POINT ( 'NONE',  ( 755.5713283507202505, -149.3618753856928265, -334.6858677611754729 ) ) ;
#8251=CARTESIAN_POINT ( 'NONE',  ( 813.1304606946830518, -65.90732993114758642, -352.3570229623690580 ) ) ;
#8254=CARTESIAN_POINT ( 'NONE',  ( 799.2566176426618085, -0.009063572426172561425, -324.0069404352559559 ) ) ;
#8256=CARTESIAN_POINT ( 'NONE',  ( 757.0176451133909268, -325.0999726633342561, -349.9200121543848354 ) ) ;
#8259=CARTESIAN_POINT ( 'NONE',  ( 803.4237431249931660, -279.1800572038741848, -331.2633955100225194 ) ) ;
#8263=CARTESIAN_POINT ( 'NONE',  ( 766.9102291470427417, -282.5545181178798657, -318.6633372737382501 ) ) ;
#8264=CARTESIAN_POINT ( 'NONE',  ( 774.6312213355099630, -287.3618753856923718, -364.6798772138717482 ) ) ;
#8266=CARTESIAN_POINT ( 'NONE',  ( 788.8264449731200330, -141.1800572038746395, -363.6646147819171233 ) ) ;
#8271=CARTESIAN_POINT ( 'NONE',  ( 771.3260364891663130, -67.64542720878958448, -306.0683387631859773 ) ) ;
#8272=CARTESIAN_POINT ( 'NONE',  ( 759.9999999999992042, -462.9681489794448339, -362.3606797749978909 ) ) ;
#8279=CARTESIAN_POINT ( 'NONE',  ( 796.9462024416508257, -132.4527844766019200, -308.9653473494370246 ) ) ;
#8284=CARTESIAN_POINT ( 'NONE',  ( 744.7301800767019131, -268.8164208402378108, -337.4774526936615757 ) ) ;
#8289=CARTESIAN_POINT ( 'NONE',  ( 773.7943932421234194, -311.8055962898685038, -305.5313806188329409 ) ) ;
#8291=CARTESIAN_POINT ( 'NONE',  ( 748.9653473494363425, -362.6346026584194533, -356.9462024416521331 ) ) ;
#8295=CARTESIAN_POINT ( 'NONE',  ( 792.1044303154645831, -420.4527844766009252, -317.8323909638837677 ) ) ;
#8296=CARTESIAN_POINT ( 'NONE',  ( 752.4576283171824116, -117.0783235625963528, -317.7880784355627952 ) ) ;
#8302=CARTESIAN_POINT ( 'NONE',  ( 795.9930595647434757, -219.0783235625960401, -320.7433823573372820 ) ) ;
#8304=CARTESIAN_POINT ( 'NONE',  ( 800.1688906516307043, -58.16923265350564520, -369.0717654672308186 ) ) ;
#8306=CARTESIAN_POINT ( 'NONE',  ( 809.4284809582966318, -452.9681489794448339, -335.2276976236387895 ) ) ;
#8309=CARTESIAN_POINT ( 'NONE',  ( 762.1177392798416577, -354.5545181178796383, -309.8865473780659272 ) ) ;
#8312=CARTESIAN_POINT ( 'NONE',  ( 784.1219089521767955, -189.2817908451528979, -315.0488828828318333 ) ) ;
#8313=CARTESIAN_POINT ( 'NONE',  ( 755.5713283507202505, -197.3618753856926560, -334.6858677611754729 ) ) ;
#8314=CARTESIAN_POINT ( 'NONE',  ( 791.9812246680005501, -380.6346026584192828, -361.9419747391813189 ) ) ;
#8316=CARTESIAN_POINT ( 'NONE',  ( 804.9511171171677688, 18.19440371013048008, -335.8780910478229202 ) ) ;
#8327=CARTESIAN_POINT ( 'NONE',  ( 766.4474001241216001, -427.0999726633338582, -307.3154664389482491 ) ) ;
#8329=CARTESIAN_POINT ( 'NONE',  ( 787.4397851343537695, -45.72551174932949181, -374.2001403089903988 ) ) ;
#8331=CARTESIAN_POINT ( 'NONE',  ( 755.0636971347428243, -388.2709662947829656, -341.7834795799807353 ) ) ;
#8332=CARTESIAN_POINT ( 'NONE',  ( 778.2165204200184689, 1.183579159761269040, -364.9363028652563230 ) ) ;
#8335=CARTESIAN_POINT ( 'NONE',  ( 804.8461984189677878, -242.1908817542435770, -336.9566956441385628 ) ) ;
#8336=CARTESIAN_POINT ( 'NONE',  ( 796.9462024416508257, -180.4527844766017211, -308.9653473494370246 ) ) ;
#8340=CARTESIAN_POINT ( 'NONE',  ( 792.4730984305310812, 16.45630643248850333, -314.5980907654948169 ) ) ;
#8345=CARTESIAN_POINT ( 'NONE',  ( 774.6312213355099630, -311.3618753856922581, -364.6798772138717482 ) ) ;
#8347=CARTESIAN_POINT ( 'NONE',  ( 752.7379699480933368, -60.00906357242598688, -361.9858362298580232 ) ) ;
#8348=CARTESIAN_POINT ( 'NONE',  ( 799.4546378042377910, -105.0783235625964096, -356.1575198192848006 ) ) ;
#8353=CARTESIAN_POINT ( 'NONE',  ( 755.5713283507202505, -29.36187538569318178, -334.6858677611754729 ) ) ;
#8354=CARTESIAN_POINT ( 'NONE',  ( 803.8651313633788504, -125.2601417444145255, -332.4468031744301015 ) ) ;
#8355=CARTESIAN_POINT ( 'NONE',  ( 778.2165204200184689, -142.8164208402382656, -364.9363028652563230 ) ) ;
#8356=CARTESIAN_POINT ( 'NONE',  ( 811.6461892240364477, 19.28531280103956647, -324.1737431748509835 ) ) ;
#8364=EDGE_LOOP ( 'NONE', ( #32742, #8997, #18827, #23046 ) ) ;
#8369=CARTESIAN_POINT ( 'NONE',  ( 799.2566176426618085, -96.00906357242585898, -324.0069404352559559 ) ) ;
#8371=CARTESIAN_POINT ( 'NONE',  ( 756.5762568750052424, -291.1800572038741848, -348.7366044899774238 ) ) ;
#8373=CARTESIAN_POINT ( 'NONE',  ( 781.7834795799800531, -394.8164208402374697, -315.0636971347436202 ) ) ;
#8374=CARTESIAN_POINT ( 'NONE',  ( 801.9419747391806368, -42.45278447660223264, -351.9812246680014027 ) ) ;
#8376=EDGE_CURVE ( 'NONE', #8202, #17032, #41807, .T. ) ;
#8381=CARTESIAN_POINT ( 'NONE',  ( 778.7629533639073998, -8.736336299698871599, -375.0009284576466371 ) ) ;
#8384=CARTESIAN_POINT ( 'NONE',  ( 764.1737431748507561, -322.3726999360615082, -371.6461892240376415 ) ) ;
#8387=CARTESIAN_POINT ( 'NONE',  ( 803.6646147819161570, -305.9073299311467622, -348.8264449731210561 ) ) ;
#8389=CARTESIAN_POINT ( 'NONE',  ( 761.4292242960306112, -137.4636090269711985, -323.2154366446414429 ) ) ;
#8393=CARTESIAN_POINT ( 'NONE',  ( 749.2812353651451076, -342.4527844766013231, -323.2262854647983090 ) ) ;
#8394=DIRECTION ( 'NONE',  ( 0.000000000000000000, 0.000000000000000000, -1.000000000000000000 ) ) ;
#8398=CARTESIAN_POINT ( 'NONE',  ( 781.2497674668890113, -252.3510508353232353, -375.3608509340180603 ) ) ;
#8400=CARTESIAN_POINT ( 'NONE',  ( 812.6845335610512393, -439.9874144716862929, -353.5525998758768651 ) ) ;
#8405=CARTESIAN_POINT ( 'NONE',  ( 793.2243759319678702, -2.532869017142183932, -318.4439275373583200 ) ) ;
#8412=CARTESIAN_POINT ( 'NONE',  ( 803.6646147819161570, -41.90732993114767169, -348.8264449731210561 ) ) ;
#8413=CARTESIAN_POINT ( 'NONE',  ( 801.3366627262608972, -320.5328690171411949, -353.0897708529566899 ) ) ;
#8415=CARTESIAN_POINT ( 'NONE',  ( 773.7943932421234194, -335.8055962898683902, -305.5313806188329409 ) ) ;
#8420=CARTESIAN_POINT ( 'NONE',  ( 804.9511171171677688, -77.80559628986920018, -335.8780910478229202 ) ) ;
#8423=CARTESIAN_POINT ( 'NONE',  ( 792.2312462859673587, -179.9073299311472454, -307.2067596250082602 ) ) ;
#8426=CARTESIAN_POINT ( 'NONE',  ( 781.7834795799800531, -178.8164208402381519, -315.0636971347436202 ) ) ;
#8429=CARTESIAN_POINT ( 'NONE',  ( 786.5483106153019435, -439.6454272087884760, -364.1601925771022366 ) ) ;
#8436=CARTESIAN_POINT ( 'NONE',  ( 790.9844846989617508, -430.3726999360611671, -317.2208543904092721 ) ) ;
#8438=CARTESIAN_POINT ( 'NONE',  ( 762.1177392798416577, -186.5545181178801215, -309.8865473780659272 ) ) ;
#8440=LINE ( 'NONE', #22510, #40123 ) ;
#8441=CARTESIAN_POINT ( 'NONE',  ( 774.6858677611749044, -201.7255117493290015, -315.5713283507209894 ) ) ;
#8442=CARTESIAN_POINT ( 'NONE',  ( 804.9511171171677688, -317.8055962898684470, -335.8780910478229202 ) ) ;
#8444=CARTESIAN_POINT ( 'NONE',  ( 791.0478386215596629, -237.8272453906072599, -306.7653713866226326 ) ) ;
#8447=CARTESIAN_POINT ( 'NONE',  ( 784.1219089521767955, -45.28179084515329578, -315.0488828828318333 ) ) ;
#8450=CARTESIAN_POINT ( 'NONE',  ( 792.3570229623691148, -237.1800572038742985, -373.1304606946836770 ) ) ;
#8452=CARTESIAN_POINT ( 'NONE',  ( 800.2193346964447755, -18.99823902205683979, -355.1360043628815788 ) ) ;
#8454=CARTESIAN_POINT ( 'NONE',  ( 781.2497674668890113, -132.3510508353235764, -375.3608509340180603 ) ) ;
#8456=CARTESIAN_POINT ( 'NONE',  ( 800.9747183278959710, -372.9982390220557704, -311.9810565676471583 ) ) ;
#8458=DIRECTION ( 'NONE',  ( 1.000000000000000000, 0.000000000000000000, 0.000000000000000000 ) ) ;
#8463=CARTESIAN_POINT ( 'NONE',  ( 803.6646147819161570, -401.9073299311463643, -348.8264449731210561 ) ) ;
#8465=CARTESIAN_POINT ( 'NONE',  ( 802.2119215644370342, -6.009063572426154742, -367.5423716828165084 ) ) ;
#8470=CARTESIAN_POINT ( 'NONE',  ( 786.6156483768007774, -241.4419599262322720, -315.5913626894246136 ) ) ;
#8472=CARTESIAN_POINT ( 'NONE',  ( 788.7631598425961101, -217.4419599262324141, -305.7194118038759143 ) ) ;
#8475=CARTESIAN_POINT ( 'NONE',  ( 764.8639956371174549, -80.08914811296574499, -319.7806653035542013 ) ) ;
#8481=CARTESIAN_POINT ( 'NONE',  ( 763.0537975583475827, -72.45278447660213317, -371.0346526505627480 ) ) ;
#8482=CARTESIAN_POINT ( 'NONE',  ( 781.8018195045267476, -70.27096629478397460, -365.1927285166407273 ) ) ;
#8484=CARTESIAN_POINT ( 'NONE',  ( 766.9102291470427417, 5.445481882119263872, -318.6633372737382501 ) ) ;
#8486=CARTESIAN_POINT ( 'NONE',  ( 755.8894580844503253, -327.8272453906069472, -332.3691319403863531 ) ) ;
#8489=CARTESIAN_POINT ( 'NONE',  ( 785.3141322388236176, -309.7255117493287457, -364.4286716492789537 ) ) ;
#8494=CARTESIAN_POINT ( 'NONE',  ( 800.9840315886518738, -316.9181544815160692, -354.1144889064786412 ) ) ;
#8495=CARTESIAN_POINT ( 'NONE',  ( 756.3353852180819104, -293.9073299311468759, -331.1735550268788302 ) ) ;
#8496=CARTESIAN_POINT ( 'NONE',  ( 755.0636971347428243, -148.2709662947837330, -341.7834795799807353 ) ) ;
#8504=CARTESIAN_POINT ( 'NONE',  ( 807.2620300519052989, -72.00906357242594424, -318.0141637701419768 ) ) ;
#8509=VERTEX_POINT ( 'NONE', #44494 ) ;
#8511=CARTESIAN_POINT ( 'NONE',  ( 751.9810565676468741, -122.0891481129656171, -360.9747183278973921 ) ) ;
#8515=CARTESIAN_POINT ( 'NONE',  ( 749.2812353651451076, -270.4527844766014937, -323.2262854647983090 ) ) ;
#8520=CARTESIAN_POINT ( 'NONE',  ( 811.6461892240364477, -340.7146871989592114, -324.1737431748509835 ) ) ;
#8521=CARTESIAN_POINT ( 'NONE',  ( 792.2312462859673587, -83.90732993114754379, -307.2067596250082602 ) ) ;
#8523=CARTESIAN_POINT ( 'NONE',  ( 745.0891759886404770, -340.2709662947831362, -342.4968714119734159 ) ) ;
#8527=CARTESIAN_POINT ( 'NONE',  ( 765.0180583372156207, -432.9982390220555999, -360.0135310231089534 ) ) ;
#8528=CARTESIAN_POINT ( 'NONE',  ( 758.0580252608178853, -222.4527844766016642, -328.0187753319985404 ) ) ;
#8530=CARTESIAN_POINT ( 'NONE',  ( 810.1134526219336749, -104.5328690171418913, -357.8822607201570349 ) ) ;
#8534=CARTESIAN_POINT ( 'NONE',  ( 803.2186876482843445, -247.9874144716867761, -350.0220218866286928 ) ) ;
#8536=CARTESIAN_POINT ( 'NONE',  ( 787.5162901302840055, 12.63812461430668321, -305.4481719005792684 ) ) ;
#8537=CARTESIAN_POINT ( 'NONE',  ( 778.7502325331095108, -72.35105083532378956, -304.6391490659818828 ) ) ;
#8541=CARTESIAN_POINT ( 'NONE',  ( 805.6418435158337843, -389.4636090269704027, -363.8556311672236916 ) ) ;
#8543=CARTESIAN_POINT ( 'NONE',  ( 802.1676090361156639, -230.6346026584197659, -327.8955696845344505 ) ) ;
#8545=VECTOR ( 'NONE', #33355, 1000.000000000000000 ) ;
#8548=CARTESIAN_POINT ( 'NONE',  ( 755.1538015810308480, -206.1908817542437191, -343.0433043558613804 ) ) ;
#8549=CARTESIAN_POINT ( 'NONE',  ( 756.5762568750052424, -195.1800572038744974, -348.7366044899774238 ) ) ;
#8550=CARTESIAN_POINT ( 'NONE',  ( 755.3201227861273992, -387.7255117493284047, -345.3687786644892981 ) ) ;
#8551=AXIS2_PLACEMENT_3D ( 'NONE', #31338, #30662, #24178 ) ;
#8554=CARTESIAN_POINT ( 'NONE',  ( 800.7704444035546203, 19.83076734649410966, -326.0291762391768771 ) ) ;
#8563=CARTESIAN_POINT ( 'NONE',  ( 810.4231160770870019, -408.5545181178794110, -321.9338519418446936 ) ) ;
#8564=CARTESIAN_POINT ( 'NONE',  ( 782.4968714119720516, -34.81642084023861372, -305.0891759886411023 ) ) ;
#8567=CARTESIAN_POINT ( 'NONE',  ( 774.6312213355099630, -383.3618753856921444, -364.6798772138717482 ) ) ;
#8568=CARTESIAN_POINT ( 'NONE',  ( 804.4286716492782716, -17.36187538569322086, -345.3141322388244703 ) ) ;
#8572=CARTESIAN_POINT ( 'NONE',  ( 780.5236548040995785, -260.7363362996981095, -314.9735926884559944 ) ) ;
#8573=CARTESIAN_POINT ( 'NONE',  ( 792.3570229623688874, -165.1800572038745258, -373.1304606946836202 ) ) ;
#8582=CARTESIAN_POINT ( 'NONE',  ( 805.1927285166397041, -328.8164208402375834, -341.8018195045277707 ) ) ;
#8585=CARTESIAN_POINT ( 'NONE',  ( 771.3260364891663130, -91.64542720878951343, -306.0683387631859773 ) ) ;
#8586=CARTESIAN_POINT ( 'NONE',  ( 779.4709603349208464, -120.3510508353236048, -314.7162404726379918 ) ) ;
#8589=CARTESIAN_POINT ( 'NONE',  ( 757.8323909638827445, -26.63460265842045871, -352.1044303154654358 ) ) ;
#8590=CARTESIAN_POINT ( 'NONE',  ( 754.8983024940795303, -138.8965053807781374, -336.9254006560228163 ) ) ;
#8591=CARTESIAN_POINT ( 'NONE',  ( 785.3687786644884454, -131.3618753856928834, -315.3201227861279676 ) ) ;
#8594=CARTESIAN_POINT ( 'NONE',  ( 766.7756240680305382, -422.5328690171408539, -361.5560724626415663 ) ) ;
#8600=CARTESIAN_POINT ( 'NONE',  ( 802.2119215644370342, -270.0090635724253048, -367.5423716828165084 ) ) ;
#8609=CARTESIAN_POINT ( 'NONE',  ( 769.0155153010367712, -82.37269993606227558, -362.7791456095907279 ) ) ;
#8610=CARTESIAN_POINT ( 'NONE',  ( 765.0180583372156207, -288.9982390220559978, -360.0135310231089534 ) ) ;
#8612=CARTESIAN_POINT ( 'NONE',  ( 795.1360043628807261, -380.0891481129646650, -360.2193346964456282 ) ) ;
#8613=CARTESIAN_POINT ( 'NONE',  ( 794.9819416627830151, -36.99823902205679360, -319.9864689768909898 ) ) ;
#8618=CARTESIAN_POINT ( 'NONE',  ( 812.3518521366052028, -25.09997266333519050, -326.5853460496235243 ) ) ;
#8621=CARTESIAN_POINT ( 'NONE',  ( 749.5768839229115201, -324.5545181178796952, -358.0661480581553064 ) ) ;
#8625=CARTESIAN_POINT ( 'NONE',  ( 797.8594530101008786, -277.5436935675105019, -322.1405469898980982 ) ) ;
#8628=CARTESIAN_POINT ( 'NONE',  ( 790.9844846989617508, -166.3726999360620198, -317.2208543904092721 ) ) ;
#8631=CARTESIAN_POINT ( 'NONE',  ( 796.7737145352015204, -332.6346026584195101, -370.7187646348536987 ) ) ;
#8636=CARTESIAN_POINT ( 'NONE',  ( 814.8230680027162407, -437.8055962898679923, -333.7305795820267917 ) ) ;
#8643=CARTESIAN_POINT ( 'NONE',  ( 803.2186876482843445, -7.987414471687621642, -350.0220218866286928 ) ) ;
#8651=CARTESIAN_POINT ( 'NONE',  ( 758.6633372737375112, -332.5328690171411381, -326.9102291470432533 ) ) ;
#8653=CARTESIAN_POINT ( 'NONE',  ( 795.6651683502461765, -322.7146871989593819, -371.3240766477733814 ) ) ;
#8661=CARTESIAN_POINT ( 'NONE',  ( 815.2698199232961542, -184.8164208402380950, -342.5225473063383106 ) ) ;
#8664=CARTESIAN_POINT ( 'NONE',  ( 765.0180583372156207, -168.9982390220563673, -360.0135310231089534 ) ) ;
#8667=CARTESIAN_POINT ( 'NONE',  ( 779.4763451958990572, -416.7363362996975980, -365.0264073115438919 ) ) ;
#8671=CARTESIAN_POINT ( 'NONE',  ( 779.9999999999992042, -462.9681489794448339, -339.9999999999999432 ) ) ;
#8674=CARTESIAN_POINT ( 'NONE',  ( 776.9254006560222479, -428.1908817542430938, -314.8983024940802125 ) ) ;
#8676=CARTESIAN_POINT ( 'NONE',  ( 754.3581564841646241, -209.4636090269709996, -316.1443688327762516 ) ) ;
#8680=CARTESIAN_POINT ( 'NONE',  ( 804.6798772138708955, -183.7255117493290015, -334.6312213355107019 ) ) ;
#8681=CARTESIAN_POINT ( 'NONE',  ( 804.1601925771018387, -343.4419599262320162, -346.5483106153029098 ) ) ;
#8683=CARTESIAN_POINT ( 'NONE',  ( 766.4474001241216001, -235.0999726633344835, -307.3154664389482491 ) ) ;
#8686=CARTESIAN_POINT ( 'NONE',  ( 775.8780910478218402, -57.28179084515326736, -364.9511171171680530 ) ) ;
#8688=CARTESIAN_POINT ( 'NONE',  ( 787.4397851343537695, -237.7255117493289163, -374.2001403089903988 ) ) ;
#8691=CARTESIAN_POINT ( 'NONE',  ( 791.9812246680005501, -20.63460265842048003, -361.9419747391813189 ) ) ;
#8693=CARTESIAN_POINT ( 'NONE',  ( 759.8311093483677041, -142.1692326535054178, -310.9282345327691814 ) ) ;
#8695=CARTESIAN_POINT ( 'NONE',  ( 744.7301800767019131, -388.8164208402374129, -337.4774526936615757 ) ) ;
#8700=CARTESIAN_POINT ( 'NONE',  ( 804.9363028652555840, -376.2709662947829656, -338.2165204200192079 ) ) ;
#8702=CARTESIAN_POINT ( 'NONE',  ( 808.0189434323515343, -446.0891481129646081, -319.0252816721025511 ) ) ;
#8706=CARTESIAN_POINT ( 'NONE',  ( 756.1348686366196716, -209.2601417444142839, -347.5531968255698416 ) ) ;
#8708=CARTESIAN_POINT ( 'NONE',  ( 768.8385539511368734, -215.2601417444141987, -306.4236121716840557 ) ) ;
#8709=PLANE ( 'NONE',  #33452 ) ;
#8714=CARTESIAN_POINT ( 'NONE',  ( 759.9864689768902508, -146.0891481129655176, -354.9819416627836404 ) ) ;
#8716=CARTESIAN_POINT ( 'NONE',  ( 772.5602148656447525, -81.72551174932937101, -305.7998596910095443 ) ) ;
#8717=CARTESIAN_POINT ( 'NONE',  ( 800.0135310231082713, -62.08914811296580183, -325.0180583372163028 ) ) ;
#8719=CARTESIAN_POINT ( 'NONE',  ( 804.6971507214547046, -27.28179084515336328, -344.0799538623459739 ) ) ;
#8721=CARTESIAN_POINT ( 'NONE',  ( 798.5707757039680246, -317.4636090269706301, -356.7845633553585003 ) ) ;
#8729=CARTESIAN_POINT ( 'NONE',  ( 773.4516893846965786, -307.6454272087888171, -315.8398074228977066 ) ) ;
#8730=CARTESIAN_POINT ( 'NONE',  ( 792.1044303154645831, -324.4527844766013231, -317.8323909638837677 ) ) ;
#8731=CARTESIAN_POINT ( 'NONE',  ( 804.4286716492782716, -137.3618753856928265, -345.3141322388244703 ) ) ;
#8735=CARTESIAN_POINT ( 'NONE',  ( 757.7880784355613741, -114.0090635724258163, -312.4576283171834916 ) ) ;
#8741=CARTESIAN_POINT ( 'NONE',  ( 787.4397851343537695, -141.7255117493291721, -374.2001403089903988 ) ) ;
#8744=CARTESIAN_POINT ( 'NONE',  ( 782.5225473063381969, -286.2709662947833635, -375.2698199232970637 ) ) ;
#8745=CARTESIAN_POINT ( 'NONE',  ( 815.2698199232962679, -448.8164208402372424, -342.5225473063383674 ) ) ;
#8748=CARTESIAN_POINT ( 'NONE',  ( 744.9990715423526808, -330.3510508353229511, -341.2370466360926002 ) ) ;
#8749=CARTESIAN_POINT ( 'NONE',  ( 782.4968714119720516, -82.81642084023846451, -305.0891759886411023 ) ) ;
#8751=CARTESIAN_POINT ( 'NONE',  ( 777.5031285880264704, -334.8164208402376403, -374.9108240113588408 ) ) ;
#8755=CARTESIAN_POINT ( 'NONE',  ( 811.6461892240364477, -124.7146871989599930, -324.1737431748509835 ) ) ;
#8760=CARTESIAN_POINT ( 'NONE',  ( 759.2295555964440155, -232.1692326535051620, -353.9708237608231229 ) ) ;
#8762=CARTESIAN_POINT ( 'NONE',  ( 810.1134526219336749, -440.5328690171407970, -357.8822607201570349 ) ) ;
#8763=CARTESIAN_POINT ( 'NONE',  ( 759.8311093483677041, -70.16923265350563099, -310.9282345327691814 ) ) ;
#8766=CARTESIAN_POINT ( 'NONE',  ( 805.6418435158337843, -365.4636090269705164, -363.8556311672236916 ) ) ;
#8768=CARTESIAN_POINT ( 'NONE',  ( 800.0135310231082713, -230.0891481129652618, -325.0180583372163028 ) ) ;
#8771=CARTESIAN_POINT ( 'NONE',  ( 776.9254006560222479, -236.1908817542436338, -314.8983024940802125 ) ) ;
#8772=CARTESIAN_POINT ( 'NONE',  ( 755.0636971347428243, -220.2709662947834772, -341.7834795799807353 ) ) ;
#8773=CARTESIAN_POINT ( 'NONE',  ( 785.3141322388236176, -381.7255117493284615, -364.4286716492789537 ) ) ;
#8776=CARTESIAN_POINT ( 'NONE',  ( 797.6776695296629214, -91.54369356751116982, -357.6776695296636603 ) ) ;
#8779=CARTESIAN_POINT ( 'NONE',  ( 782.7696130847263021, 18.14353250567099707, -310.1281195208451322 ) ) ;
#8785=CARTESIAN_POINT ( 'NONE',  ( 773.7305795820266212, -441.2817908451521021, -374.8230680027170365 ) ) ;
#8786=CARTESIAN_POINT ( 'NONE',  ( 745.0891759886404770, -52.27096629478401724, -342.4968714119734159 ) ) ;
#8788=CARTESIAN_POINT ( 'NONE',  ( 778.2165204200184689, -382.8164208402374697, -364.9363028652563230 ) ) ;
#8789=CARTESIAN_POINT ( 'NONE',  ( 797.6776695296629214, 4.456306432488530866, -357.6776695296636603 ) ) ;
#8792=CARTESIAN_POINT ( 'NONE',  ( 804.6971507214547046, -267.2817908451526137, -344.0799538623459739 ) ) ;
#8793=CARTESIAN_POINT ( 'NONE',  ( 805.0032342141412300, -181.5436935675108145, -314.9967657858571783 ) ) ;
#8796=CARTESIAN_POINT ( 'NONE',  ( 778.5401871010416244, 16.45630643248848912, -314.2029270906900251 ) ) ;
#8802=CARTESIAN_POINT ( 'NONE',  ( 755.3201227861273992, -315.7255117493286320, -345.3687786644892981 ) ) ;
#8804=CARTESIAN_POINT ( 'NONE',  ( 805.6418435158337843, -101.4636090269713264, -363.8556311672236916 ) ) ;
#8805=CARTESIAN_POINT ( 'NONE',  ( 776.9566956441375396, -132.8965053807781374, -364.8461984189686405 ) ) ;
#8808=CARTESIAN_POINT ( 'NONE',  ( 788.7366044899766848, -11.90732993114778182, -316.5762568750059813 ) ) ;
#8809=CARTESIAN_POINT ( 'NONE',  ( 763.2154366446407039, -141.6237781080508569, -321.4292242960311228 ) ) ;
#8810=CARTESIAN_POINT ( 'NONE',  ( 804.9363028652555840, -136.2709662947837330, -338.2165204200192079 ) ) ;
#8812=CARTESIAN_POINT ( 'NONE',  ( 757.2208543904082489, -424.7146871989589840, -350.9844846989624330 ) ) ;
#8818=CARTESIAN_POINT ( 'NONE',  ( 814.2805881961230625, -289.6454272087889308, -331.2368401574024119 ) ) ;
#8825=CARTESIAN_POINT ( 'NONE',  ( 800.9840315886518738, -100.9181544815167513, -354.1144889064786412 ) ) ;
#8826=CARTESIAN_POINT ( 'NONE',  ( 791.9812246680005501, -284.6346026584196807, -361.9419747391813189 ) ) ;
#8829=CARTESIAN_POINT ( 'NONE',  ( 762.3223304703356007, -415.5436935675102177, -322.3223304703362828 ) ) ;
#8830=CARTESIAN_POINT ( 'NONE',  ( 754.8072714833581358, -100.8164208402383792, -338.1981804954720587 ) ) ;
#8836=CARTESIAN_POINT ( 'NONE',  ( 766.4474001241216001, -355.0999726633341993, -307.3154664389482491 ) ) ;
#8839=CARTESIAN_POINT ( 'NONE',  ( 797.6776695296629214, -283.5436935675105019, -357.6776695296636603 ) ) ;
#8841=CARTESIAN_POINT ( 'NONE',  ( 796.1575198192839480, -150.0090635724257027, -359.4546378042384163 ) ) ;
#8845=CARTESIAN_POINT ( 'NONE',  ( 801.1904061080338124, -332.0891481129649492, -368.3070685750236066 ) ) ;
#8850=CARTESIAN_POINT ( 'NONE',  ( 777.5031285880264704, 1.183579159761269040, -374.9108240113588408 ) ) ;
#8856=CARTESIAN_POINT ( 'NONE',  ( 760.5453621957607311, -21.07832356259667250, -323.8424801807151425 ) ) ;
#8861=CARTESIAN_POINT ( 'NONE',  ( 779.4709603349208464, -312.3510508353230080, -314.7162404726379918 ) ) ;
#8865=CARTESIAN_POINT ( 'NONE',  ( 783.7566961878529810, -336.8965053807774552, -305.1792804349288417 ) ) ;
#8872=CARTESIAN_POINT ( 'NONE',  ( 751.9810565676468741, -170.0891481129654608, -360.9747183278973921 ) ) ;
#8875=CARTESIAN_POINT ( 'NONE',  ( 774.6312213355098493, -191.3618753856926276, -364.6798772138717482 ) ) ;
#8877=CARTESIAN_POINT ( 'NONE',  ( 754.7162404726377645, -446.7363362996975980, -339.4709603349214717 ) ) ;
#8883=CARTESIAN_POINT ( 'NONE',  ( 757.0176451133909268, -421.0999726633340288, -349.9200121543848354 ) ) ;
#8885=CARTESIAN_POINT ( 'NONE',  ( 747.6481478633932056, -205.0999726633346256, -353.4146539503763620 ) ) ;
#8888=CARTESIAN_POINT ( 'NONE',  ( 803.4237431249931660, -183.1800572038744974, -331.2633955100225194 ) ) ;
#8890=CARTESIAN_POINT ( 'NONE',  ( 775.9200461376533440, -359.8055962898683333, -315.3028492785443291 ) ) ;
#8892=CARTESIAN_POINT ( 'NONE',  ( 802.2119215644370342, -222.0090635724254184, -367.5423716828165084 ) ) ;
#8895=CARTESIAN_POINT ( 'NONE',  ( 804.6971507214547046, -51.28179084515328867, -344.0799538623459739 ) ) ;
#8898=CARTESIAN_POINT ( 'NONE',  ( 810.7187646348534145, -234.4527844766016358, -356.7737145352016341 ) ) ;
#8901=CARTESIAN_POINT ( 'NONE',  ( 755.0636971347428243, -52.27096629478401724, -341.7834795799807353 ) ) ;
#8903=CARTESIAN_POINT ( 'NONE',  ( 764.3348316497523456, -118.7146871989600072, -308.6759233522265617 ) ) ;
#8905=CARTESIAN_POINT ( 'NONE',  ( 792.3570229623688874, -357.1800572038739006, -373.1304606946836202 ) ) ;
#8907=LINE ( 'NONE', #26899, #1056 ) ;
#8910=CARTESIAN_POINT ( 'NONE',  ( 792.1044303154645831, -396.4527844766010389, -317.8323909638837677 ) ) ;
#8912=CARTESIAN_POINT ( 'NONE',  ( 809.0717654672305343, -4.918154481517067467, -360.1688906516309885 ) ) ;
#8916=CARTESIAN_POINT ( 'NONE',  ( 779.4709603349208464, -240.3510508353232069, -314.7162404726379918 ) ) ;
#8918=CARTESIAN_POINT ( 'NONE',  ( 744.8212110874229666, -234.8965053807777963, -336.2046728542121627 ) ) ;
#8924=CARTESIAN_POINT ( 'NONE',  ( 772.4837098697144029, -71.36187538569302546, -374.5518280994205611 ) ) ;
#8925=CARTESIAN_POINT ( 'NONE',  ( 803.4237431249931660, -87.18005720387481006, -331.2633955100225194 ) ) ;
#8927=CARTESIAN_POINT ( 'NONE',  ( 755.3028492785439312, -15.28179084515340058, -335.9200461376539693 ) ) ;
#8929=CARTESIAN_POINT ( 'NONE',  ( 773.4516893846965786, -307.6454272087888171, -315.8398074228977066 ) ) ;
#8936=CARTESIAN_POINT ( 'NONE',  ( 802.9823548866075953, -313.0999726633342561, -330.0799878456151077 ) ) ;
#8937=CARTESIAN_POINT ( 'NONE',  ( 800.2193346964447755, -306.9982390220558273, -355.1360043628815788 ) ) ;
#8938=CARTESIAN_POINT ( 'NONE',  ( 800.2193346964447755, -162.9982390220563673, -355.1360043628815788 ) ) ;
#8944=CARTESIAN_POINT ( 'NONE',  ( 800.7704444035546203, -268.1692326535049347, -326.0291762391768771 ) ) ;
#8945=CARTESIAN_POINT ( 'NONE',  ( 749.5768839229115201, -108.5545181178803915, -358.0661480581553064 ) ) ;
#8953=CARTESIAN_POINT ( 'NONE',  ( 755.2512626584698410, -151.5436935675109851, -315.2512626584710915 ) ) ;
#8956=CARTESIAN_POINT ( 'NONE',  ( 763.0537975583475827, -264.4527844766016074, -371.0346526505627480 ) ) ;
#8960=CARTESIAN_POINT ( 'NONE',  ( 771.2368401574024119, -349.4419599262320162, -374.2805881961240857 ) ) ;
#8961=CARTESIAN_POINT ( 'NONE',  ( 810.7187646348534145, -90.45278447660209054, -356.7737145352016341 ) ) ;
#8963=CARTESIAN_POINT ( 'NONE',  ( 792.3570229623688874, -357.1800572038739006, -373.1304606946836202 ) ) ;
#8967=CARTESIAN_POINT ( 'NONE',  ( 754.8072714833581358, -220.8164208402379529, -338.1981804954720587 ) ) ;
#8968=CARTESIAN_POINT ( 'NONE',  ( 751.2241431872005251, -136.1692326535053894, -359.9636004259367610 ) ) ;
#8972=ORIENTED_EDGE ( 'NONE', *, *, #19296, .F. ) ;
#8973=CARTESIAN_POINT ( 'NONE',  ( 754.9735926884551418, 5.648949164675971524, -340.5236548041000333 ) ) ;
#8975=CARTESIAN_POINT ( 'NONE',  ( 795.6651683502461765, -418.7146871989590409, -371.3240766477733814 ) ) ;
#8979=CARTESIAN_POINT ( 'NONE',  ( 768.9521613784389729, -393.8272453906067199, -373.2346286133773106 ) ) ;
#8980=CARTESIAN_POINT ( 'NONE',  ( 762.1405469898971887, -241.5436935675106156, -357.8594530101015607 ) ) ;
#8983=CARTESIAN_POINT ( 'NONE',  ( 804.4086373105744769, -217.6454272087891582, -333.3843516231986541 ) ) ;
#8984=CARTESIAN_POINT ( 'NONE',  ( 797.8594530101008786, -205.5436935675108430, -322.1405469898980982 ) ) ;
#8986=CARTESIAN_POINT ( 'NONE',  ( 803.4237431249931660, -399.1800572038738437, -331.2633955100225194 ) ) ;
#8989=CARTESIAN_POINT ( 'NONE',  ( 778.2165204200184689, -94.81642084023843609, -364.9363028652563230 ) ) ;
#8997=ORIENTED_EDGE ( 'NONE', *, *, #17059, .T. ) ;
#8998=CARTESIAN_POINT ( 'NONE',  ( 748.6759233522253680, -448.3726999360611103, -324.3348316497537098 ) ) ;
#8999=CARTESIAN_POINT ( 'NONE',  ( 808.3070685750232087, -42.99823902205676518, -361.1904061080339829 ) ) ;
#9001=CARTESIAN_POINT ( 'NONE',  ( 794.9819416627830151, -396.9982390220556567, -319.9864689768909898 ) ) ;
#9002=CARTESIAN_POINT ( 'NONE',  ( 762.1405469898973024, -25.54369356751137232, -357.8594530101016176 ) ) ;
#9005=CARTESIAN_POINT ( 'NONE',  ( 799.2566176426618085, -288.0090635724252479, -324.0069404352559559 ) ) ;
#9006=CARTESIAN_POINT ( 'NONE',  ( 745.4481719005789273, -171.7255117493291152, -347.5162901302853129 ) ) ;
#9009=CARTESIAN_POINT ( 'NONE',  ( 780.7518514355283514, 16.45630643248848912, -313.9393219192966740 ) ) ;
#9013=CARTESIAN_POINT ( 'NONE',  ( 797.8594530101008786, -349.5436935675102745, -322.1405469898980982 ) ) ;
#9016=CARTESIAN_POINT ( 'NONE',  ( 783.7953271457878373, -104.1908817542440175, -375.1787889125761239 ) ) ;
#9017=CARTESIAN_POINT ( 'NONE',  ( 755.0488828828309806, -161.8055962898689870, -344.1219089521771934 ) ) ;
#9020=CARTESIAN_POINT ( 'NONE',  ( 805.1927285166397041, -40.81642084023859951, -341.8018195045277707 ) ) ;
#9021=CARTESIAN_POINT ( 'NONE',  ( 765.8855110935204493, -166.1692326535053041, -319.0159684113471599 ) ) ;
#9022=CARTESIAN_POINT ( 'NONE',  ( 800.2193346964447755, -138.9982390220563957, -355.1360043628815788 ) ) ;
#9024=CARTESIAN_POINT ( 'NONE',  ( 779.4709603349208464, -432.3510508353226669, -314.7162404726379918 ) ) ;
#9030=CARTESIAN_POINT ( 'NONE',  ( 755.8990559732751535, -275.4636090269708575, -365.9055244015606831 ) ) ;
#9037=CARTESIAN_POINT ( 'NONE',  ( 784.1219089521767955, -117.2817908451530684, -315.0488828828318333 ) ) ;
#9038=CARTESIAN_POINT ( 'NONE',  ( 762.3223304703356007, -127.5436935675110561, -322.3223304703362828 ) ) ;
#9040=CARTESIAN_POINT ( 'NONE',  ( 755.0636971347428243, -268.2709662947833067, -341.7834795799807353 ) ) ;
#9041=ORIENTED_EDGE ( 'NONE', *, *, #42791, .F. ) ;
#9042=CARTESIAN_POINT ( 'NONE',  ( 778.2165204200184689, -430.8164208402374129, -364.9363028652563230 ) ) ;
#9043=CARTESIAN_POINT ( 'NONE',  ( 774.6312213355099630, -71.36187538569302546, -364.6798772138717482 ) ) ;
#9049=CARTESIAN_POINT ( 'NONE',  ( 766.4474001241216001, -331.0999726633342561, -307.3154664389482491 ) ) ;
#9054=CARTESIAN_POINT ( 'NONE',  ( 771.2633955100217236, -287.9073299311468759, -363.4237431249939618 ) ) ;
#9056=CARTESIAN_POINT ( 'NONE',  ( 766.0291762391763086, -202.9181544815164386, -360.7704444035551319 ) ) ;
#9059=CARTESIAN_POINT ( 'NONE',  ( 755.2512626584698410, -367.5436935675102745, -315.2512626584710915 ) ) ;
#9064=CARTESIAN_POINT ( 'NONE',  ( 808.0189434323515343, -14.08914811296595460, -319.0252816721025511 ) ) ;
#9065=CARTESIAN_POINT ( 'NONE',  ( 803.4237431249931660, -231.1800572038743553, -331.2633955100225194 ) ) ;
#9067=ADVANCED_FACE ( 'NONE', ( #6391 ), #31766, .F. ) ;
#9071=CARTESIAN_POINT ( 'NONE',  ( 755.0488828828309806, -17.80559628986940979, -344.1219089521771934 ) ) ;
#9078=CARTESIAN_POINT ( 'NONE',  ( 805.0264073115434940, -318.3510508353230080, -339.4763451958999099 ) ) ;
#9081=CARTESIAN_POINT ( 'NONE',  ( 811.6461892240364477, -364.7146871989592114, -324.1737431748509835 ) ) ;
#9087=CARTESIAN_POINT ( 'NONE',  ( 772.4837098697144029, -167.3618753856927412, -374.5518280994205611 ) ) ;
#9090=CARTESIAN_POINT ( 'NONE',  ( 767.8955696845334842, -192.4527844766017211, -362.1676090361161755 ) ) ;
#9092=CARTESIAN_POINT ( 'NONE',  ( 766.0291762391763086, -442.9181544815157849, -360.7704444035551319 ) ) ;
#9100=CARTESIAN_POINT ( 'NONE',  ( 802.5472867521000353, -436.3726999360612240, -350.8726784830461156 ) ) ;
#9102=VECTOR ( 'NONE', #23422, 1000.000000000000000 ) ;
#9104=CARTESIAN_POINT ( 'NONE',  ( 745.5313806188320314, -231.2817908451527558, -333.7943932421247268 ) ) ;
#9108=CARTESIAN_POINT ( 'NONE',  ( 774.6312213355099630, -191.3618753856925991, -364.6798772138717482 ) ) ;
#9109=CARTESIAN_POINT ( 'NONE',  ( 756.1348686366196716, -353.2601417444137724, -347.5531968255698416 ) ) ;
#9111=CARTESIAN_POINT ( 'NONE',  ( 744.6391490659812007, -206.7363362996982801, -338.7502325331110455 ) ) ;
#9114=CARTESIAN_POINT ( 'NONE',  ( 804.8461984189677878, -98.19088175424404596, -336.9566956441385628 ) ) ;
#9118=CARTESIAN_POINT ( 'NONE',  ( 773.3843516231979720, -421.4419599262317888, -364.4086373105754433 ) ) ;
#9119=CARTESIAN_POINT ( 'NONE',  ( 749.2812353651451076, -294.4527844766013800, -323.2262854647983090 ) ) ;
#9122=CARTESIAN_POINT ( 'NONE',  ( 756.3353852180819104, -53.90732993114765037, -331.1735550268788302 ) ) ;
#9125=CARTESIAN_POINT ( 'NONE',  ( 745.1769319972822814, -137.8055962898690154, -346.2694204179732083 ) ) ;
#9127=CARTESIAN_POINT ( 'NONE',  ( 777.4774526936600978, -418.2709662947827383, -304.7301800767027657 ) ) ;
#9131=CARTESIAN_POINT ( 'NONE',  ( 767.8955696845333705, -408.4527844766009252, -362.1676090361162323 ) ) ;
#9133=CARTESIAN_POINT ( 'NONE',  ( 802.2119215644370342, -30.00906357242607925, -367.5423716828165084 ) ) ;
#9137=CARTESIAN_POINT ( 'NONE',  ( 756.7813123517142913, -235.9874144716868898, -329.9779781133712504 ) ) ;
#9141=CARTESIAN_POINT ( 'NONE',  ( 798.0661480581538854, -218.5328690171414792, -309.5768839229118043 ) ) ;
#9147=CARTESIAN_POINT ( 'NONE',  ( 803.6646147819161570, -185.9073299311472454, -348.8264449731210561 ) ) ;
#9149=ADVANCED_FACE ( 'NONE', ( #6829, #2919 ), #17008, .F. ) ;
#9150=CARTESIAN_POINT ( 'NONE',  ( 814.5518280994195948, -87.72551174932937101, -332.4837098697145734 ) ) ;
#9151=CARTESIAN_POINT ( 'NONE',  ( 804.6798772138710092, -63.72551174932941365, -334.6312213355106451 ) ) ;
#9153=CARTESIAN_POINT ( 'NONE',  ( 763.8424801807145741, -18.00906357242611477, -320.5453621957614700 ) ) ;
#9155=CARTESIAN_POINT ( 'NONE',  ( 796.1575198192839480, -342.0090635724251342, -359.4546378042384163 ) ) ;
#9162=CARTESIAN_POINT ( 'NONE',  ( 800.9840315886518738, -340.9181544815160123, -354.1144889064786412 ) ) ;
#9163=CARTESIAN_POINT ( 'NONE',  ( 803.6646147819161570, -305.9073299311467622, -348.8264449731210561 ) ) ;
#9164=CARTESIAN_POINT ( 'NONE',  ( 799.9636004259356241, -142.9181544815166376, -311.2241431872006956 ) ) ;
#9168=CARTESIAN_POINT ( 'NONE',  ( 813.5763878283155464, -123.8272453906076009, -351.1614460488615350 ) ) ;
#9178=CARTESIAN_POINT ( 'NONE',  ( 792.2312462859673587, -155.9073299311473306, -307.2067596250082602 ) ) ;
#9183=CARTESIAN_POINT ( 'NONE',  ( 808.3070685750230950, -282.9982390220558841, -361.1904061080339261 ) ) ;
#9188=CARTESIAN_POINT ( 'NONE',  ( 813.2346286133761168, -341.2601417444138292, -328.9521613784389160 ) ) ;
#9189=CARTESIAN_POINT ( 'NONE',  ( 759.0252816721024374, -96.99823902205660886, -368.0189434323527280 ) ) ;
#9192=CARTESIAN_POINT ( 'NONE',  ( 787.5162901302840055, -347.3618753856922012, -305.4481719005792684 ) ) ;
#9198=CARTESIAN_POINT ( 'NONE',  ( 815.1787889125755555, -126.8965053807781516, -343.7953271457877804 ) ) ;
#9202=VERTEX_POINT ( 'NONE', #29236 ) ;
#9203=EDGE_CURVE ( 'NONE', #20167, #14643, #43922, .T. ) ;
#9204=CARTESIAN_POINT ( 'NONE',  ( 783.0433043558608688, -0.8965053807785533513, -315.1538015810313027 ) ) ;
#9207=CARTESIAN_POINT ( 'NONE',  ( 814.8230680027162407, -437.8055962898679923, -333.7305795820267917 ) ) ;
#9211=CARTESIAN_POINT ( 'NONE',  ( 812.3518521366052028, -361.0999726633341425, -326.5853460496235243 ) ) ;
#9213=CARTESIAN_POINT ( 'NONE',  ( 794.9819416627830151, -228.9982390220561683, -319.9864689768909898 ) ) ;
#9218=CARTESIAN_POINT ( 'NONE',  ( 755.8894580844503253, -207.8272453906073451, -332.3691319403863531 ) ) ;
#9219=CARTESIAN_POINT ( 'NONE',  ( 803.4237431249931660, -231.1800572038743553, -331.2633955100225194 ) ) ;
#9220=CARTESIAN_POINT ( 'NONE',  ( 797.6776695296629214, -427.5436935675101040, -357.6776695296636603 ) ) ;
#9223=CARTESIAN_POINT ( 'NONE',  ( 771.2633955100217236, -95.90732993114751537, -363.4237431249939618 ) ) ;
#9230=AXIS2_PLACEMENT_3D ( 'NONE', #22034, #4702, #19030 ) ;
#9235=CARTESIAN_POINT ( 'NONE',  ( 744.6391490659812007, -446.7363362996975980, -338.7502325331110455 ) ) ;
#9236=CARTESIAN_POINT ( 'NONE',  ( 754.9967657858570647, -25.54369356751137232, -365.0032342141425943 ) ) ;
#9238=CARTESIAN_POINT ( 'NONE',  ( 754.8072714833581358, -436.8164208402372992, -338.1981804954720587 ) ) ;
#9239=CARTESIAN_POINT ( 'NONE',  ( 801.9419747391806368, 5.547215523397618142, -351.9812246680014027 ) ) ;
#9241=CARTESIAN_POINT ( 'NONE',  ( 779.9999999999992042, -462.9681489794448339, -339.9999999999999432 ) ) ;
#9242=CARTESIAN_POINT ( 'NONE',  ( 796.1575198192839480, -294.0090635724253048, -359.4546378042384163 ) ) ;
#9243=CARTESIAN_POINT ( 'NONE',  ( 746.8695393053150156, -173.9073299311472169, -327.6429770376306010 ) ) ;
#9247=CARTESIAN_POINT ( 'NONE',  ( 794.4892657455289964, 16.45630643248850689, -314.6207049315058271 ) ) ;
#9250=CARTESIAN_POINT ( 'NONE',  ( 795.6651683502461765, -226.7146871989596661, -371.3240766477733814 ) ) ;
#9256=CARTESIAN_POINT ( 'NONE',  ( 771.1735550268778070, -369.1800572038739574, -316.3353852180827630 ) ) ;
#9259=CARTESIAN_POINT ( 'NONE',  ( 746.4236121716829757, -87.82724539060770041, -328.8385539511384650 ) ) ;
#9260=CARTESIAN_POINT ( 'NONE',  ( 755.8398074228967971, -163.4419599262325846, -333.4516893846970333 ) ) ;
#9263=CARTESIAN_POINT ( 'NONE',  ( 797.8594530101008786, -61.54369356751124087, -322.1405469898980982 ) ) ;
#9264=CARTESIAN_POINT ( 'NONE',  ( 769.1273215169530886, -166.7146871989598367, -317.4527132478988847 ) ) ;
#9268=CARTESIAN_POINT ( 'NONE',  ( 814.8230680027162407, -5.805596289869448867, -333.7305795820267917 ) ) ;
#9274=CARTESIAN_POINT ( 'NONE',  ( 750.9282345327678740, -256.9181544815163534, -319.8311093483690115 ) ) ;
#9280=CARTESIAN_POINT ( 'NONE',  ( 763.0428371773158460, -107.4636090269713122, -358.7617431975195359 ) ) ;
#9281=CARTESIAN_POINT ( 'NONE',  ( 800.2193346964447755, -114.9982390220565236, -355.1360043628815788 ) ) ;
#9282=CARTESIAN_POINT ( 'NONE',  ( 805.1927285166399315, -304.8164208402376971, -341.8018195045277707 ) ) ;
#9284=CARTESIAN_POINT ( 'NONE',  ( 788.8264449731200330, -429.1800572038737869, -363.6646147819171233 ) ) ;
#9290=EDGE_LOOP ( 'NONE', ( #2276, #4456 ) ) ;
#9291=CARTESIAN_POINT ( 'NONE',  ( 749.5768839229115201, -348.5545181178796383, -358.0661480581553064 ) ) ;
#9294=CARTESIAN_POINT ( 'NONE',  ( 804.4286716492782716, -305.3618753856922581, -345.3141322388244703 ) ) ;
#9296=CARTESIAN_POINT ( 'NONE',  ( 793.0897708529556667, -174.5545181178801784, -361.3366627262616362 ) ) ;
#9298=CARTESIAN_POINT ( 'NONE',  ( 779.9999999999992042, 126.4563064324884465, -339.9999999999999432 ) ) ;
#9299=CARTESIAN_POINT ( 'NONE',  ( 792.2312462859673587, -395.9073299311465348, -307.2067596250082602 ) ) ;
#9304=CARTESIAN_POINT ( 'NONE',  ( 812.7932403749906598, -15.18005720387504631, -327.7687537140311633 ) ) ;
#9305=CARTESIAN_POINT ( 'NONE',  ( 802.1676090361156639, -254.6346026584196238, -327.8955696845344505 ) ) ;
#9309=CARTESIAN_POINT ( 'NONE',  ( 803.8651313633788504, -53.26014174441475291, -332.4468031744301015 ) ) ;
#9317=CARTESIAN_POINT ( 'NONE',  ( 755.8398074228967971, -331.4419599262320162, -333.4516893846970333 ) ) ;
#9321=CARTESIAN_POINT ( 'NONE',  ( 788.7631598425961101, -361.4419599262319593, -305.7194118038759143 ) ) ;
#9327=CARTESIAN_POINT ( 'NONE',  ( 808.3070685750230950, -234.9982390220561683, -361.1904061080339261 ) ) ;
#9330=CARTESIAN_POINT ( 'NONE',  ( 755.0636971347428243, -220.2709662947834772, -341.7834795799807353 ) ) ;
#9332=CARTESIAN_POINT ( 'NONE',  ( 778.2165204200184689, -310.8164208402377540, -364.9363028652563230 ) ) ;
#9333=CARTESIAN_POINT ( 'NONE',  ( 769.9779781133707957, -451.0999726633339151, -316.7813123517150871 ) ) ;
#9340=CARTESIAN_POINT ( 'NONE',  ( 759.0159684113467620, -448.9181544815156144, -325.8855110935213020 ) ) ;
#9341=CARTESIAN_POINT ( 'NONE',  ( 762.3515768340985232, 20.87080523294372014, -315.3598267498177847 ) ) ;
#9344=CARTESIAN_POINT ( 'NONE',  ( 749.5768839229115201, -228.5545181178799794, -358.0661480581553064 ) ) ;
#9348=CARTESIAN_POINT ( 'NONE',  ( 754.8072714833581358, -196.8164208402380950, -338.1981804954720587 ) ) ;
#9349=CARTESIAN_POINT ( 'NONE',  ( 764.0069404352550464, -375.0783235625955285, -359.2566176426627180 ) ) ;
#9350=CARTESIAN_POINT ( 'NONE',  ( 757.7880784355613741, -210.0090635724255321, -312.4576283171834916 ) ) ;
#9352=CARTESIAN_POINT ( 'NONE',  ( 759.9999999999992042, 166.4563064324884465, -319.9999999999999432 ) ) ;
#9353=CARTESIAN_POINT ( 'NONE',  ( 758.4439275373578084, -84.55451811788046257, -353.2243759319684386 ) ) ;
#9358=CARTESIAN_POINT ( 'NONE',  ( 745.7998596910086917, -269.3618753856924286, -332.5602148656461168 ) ) ;
#9361=CARTESIAN_POINT ( 'NONE',  ( 803.6646147819161570, -65.90732993114758642, -348.8264449731210561 ) ) ;
#9364=CARTESIAN_POINT ( 'NONE',  ( 803.8556311672234642, -153.6237781080508000, -365.6418435158340117 ) ) ;
#9366=CARTESIAN_POINT ( 'NONE',  ( 747.2067596250078623, -411.1800572038738437, -352.2312462859687230 ) ) ;
#9368=PLANE ( 'NONE',  #35735 ) ;
#9371=CARTESIAN_POINT ( 'NONE',  ( 759.7806653035534055, -414.9982390220555430, -324.8639956371180801 ) ) ;
#9377=CARTESIAN_POINT ( 'NONE',  ( 772.3691319403857278, -215.2601417444141987, -315.8894580844506663 ) ) ;
#9378=CARTESIAN_POINT ( 'NONE',  ( 771.1735550268778070, -129.1800572038746111, -316.3353852180827630 ) ) ;
#9380=CARTESIAN_POINT ( 'NONE',  ( 813.2346286133761168, -245.2601417444141987, -328.9521613784389160 ) ) ;
#9384=CARTESIAN_POINT ( 'NONE',  ( 804.9363028652555840, -184.2709662947835909, -338.2165204200192079 ) ) ;
#9387=CARTESIAN_POINT ( 'NONE',  ( 814.2001403089898304, -113.3618753856929260, -347.4397851343538264 ) ) ;
#9388=CARTESIAN_POINT ( 'NONE',  ( 778.1981804954715471, -58.27096629478398881, -314.8072714833591021 ) ) ;
#9389=CARTESIAN_POINT ( 'NONE',  ( 758.4439275373578084, -60.55451811788051941, -353.2243759319684386 ) ) ;
#9390=CARTESIAN_POINT ( 'NONE',  ( 790.0220218866281812, -343.0999726633342561, -363.2186876482849129 ) ) ;
#9399=CARTESIAN_POINT ( 'NONE',  ( 754.7162404726377645, -326.7363362996979390, -339.4709603349214717 ) ) ;
#9400=CARTESIAN_POINT ( 'NONE',  ( 803.4237431249931660, -327.1800572038741279, -331.2633955100225194 ) ) ;
#9401=CARTESIAN_POINT ( 'NONE',  ( 807.2620300519052989, -120.0090635724258021, -318.0141637701419768 ) ) ;
#9405=CARTESIAN_POINT ( 'NONE',  ( 810.4231160770870019, -120.5545181178803205, -321.9338519418446936 ) ) ;
#9406=CARTESIAN_POINT ( 'NONE',  ( 779.9999999999992042, 126.4563064324884465, -339.9999999999999432 ) ) ;
#9412=CARTESIAN_POINT ( 'NONE',  ( 808.3070685750232087, -162.9982390220563673, -361.1904061080339829 ) ) ;
#9415=CARTESIAN_POINT ( 'NONE',  ( 808.0189434323515343, -302.0891481129650629, -319.0252816721025511 ) ) ;
#9421=CARTESIAN_POINT ( 'NONE',  ( 747.3154664389472828, -355.9874144716865203, -326.4474001241230781 ) ) ;
#9423=CARTESIAN_POINT ( 'NONE',  ( 754.9967657858570647, -121.5436935675110419, -365.0032342141425374 ) ) ;
#9425=CARTESIAN_POINT ( 'NONE',  ( 812.7932403749906598, -375.1800572038739574, -327.7687537140311633 ) ) ;
#9426=CARTESIAN_POINT ( 'NONE',  ( 779.9999999999992042, -452.9681489794448339, -339.9999999999999432 ) ) ;
#9432=CARTESIAN_POINT ( 'NONE',  ( 793.4146539503750546, -169.9874144716871172, -307.6481478633938877 ) ) ;
#9438=CARTESIAN_POINT ( 'NONE',  ( 758.0141637701419768, -423.0783235625953580, -367.2620300519063790 ) ) ;
#9441=ORIENTED_EDGE ( 'NONE', *, *, #23778, .T. ) ;
#9442=CARTESIAN_POINT ( 'NONE',  ( 794.9819416627830151, -180.9982390220563389, -319.9864689768909898 ) ) ;
#9443=CARTESIAN_POINT ( 'NONE',  ( 776.2046728542105711, -380.1908817542431507, -304.8212110874238761 ) ) ;
#9448=CARTESIAN_POINT ( 'NONE',  ( 761.4292242960306112, -233.4636090269708575, -323.2154366446414429 ) ) ;
#9449=CARTESIAN_POINT ( 'NONE',  ( 795.1360043628807261, -212.0891481129652902, -360.2193346964456282 ) ) ;
#9450=CARTESIAN_POINT ( 'NONE',  ( 802.1676090361155502, -422.6346026584191691, -327.8955696845344505 ) ) ;
#9453=CARTESIAN_POINT ( 'NONE',  ( 788.7366044899766848, -107.9073299311474727, -316.5762568750059813 ) ) ;
#9463=CARTESIAN_POINT ( 'NONE',  ( 813.5763878283155464, -459.8272453906066062, -351.1614460488615350 ) ) ;
#9464=CARTESIAN_POINT ( 'NONE',  ( 746.8695393053151292, -53.90732993114765037, -327.6429770376306578 ) ) ;
#9466=CARTESIAN_POINT ( 'NONE',  ( 802.1676090361156639, -422.6346026584192259, -327.8955696845344505 ) ) ;
#9467=CARTESIAN_POINT ( 'NONE',  ( 788.8264449731201466, -45.18005720387493795, -363.6646147819170665 ) ) ;
#9470=CARTESIAN_POINT ( 'NONE',  ( 791.9812246680005501, 3.365397341579444479, -361.9419747391813189 ) ) ;
#9471=CARTESIAN_POINT ( 'NONE',  ( 801.5560724626406000, -288.5545181178798657, -326.7756240680316182 ) ) ;
#9472=CARTESIAN_POINT ( 'NONE',  ( 748.9653473494363425, -194.6346026584198796, -356.9462024416521331 ) ) ;
#9477=CARTESIAN_POINT ( 'NONE',  ( 759.8311093483677041, -238.1692326535050768, -310.9282345327691814 ) ) ;
#9479=CARTESIAN_POINT ( 'NONE',  ( 777.4774526936600978, -298.2709662947830793, -304.7301800767027657 ) ) ;
#9483=CARTESIAN_POINT ( 'NONE',  ( 797.6776695296629214, -355.5436935675103882, -357.6776695296636603 ) ) ;
#9486=CARTESIAN_POINT ( 'NONE',  ( 764.1737431748507561, -82.37269993606227558, -371.6461892240376415 ) ) ;
#9487=CARTESIAN_POINT ( 'NONE',  ( 793.2243759319678702, -170.5328690171416781, -318.4439275373583200 ) ) ;
#9489=DIRECTION ( 'NONE',  ( 0.000000000000000000, -1.000000000000000000, 0.000000000000000000 ) ) ;
#9492=CARTESIAN_POINT ( 'NONE',  ( 774.6312213355099630, -47.36187538569312494, -364.6798772138717482 ) ) ;
#9493=CARTESIAN_POINT ( 'NONE',  ( 760.5453621957607311, -165.0783235625962391, -323.8424801807151425 ) ) ;
#9495=CARTESIAN_POINT ( 'NONE',  ( 813.2346286133761168, -5.260141744414903897, -328.9521613784389160 ) ) ;
#9500=CARTESIAN_POINT ( 'NONE',  ( 750.9282345327678740, -280.9181544815162965, -319.8311093483690115 ) ) ;
#9507=CARTESIAN_POINT ( 'NONE',  ( 783.0745993439762742, -104.1908817542440175, -365.1016975059196739 ) ) ;
#9508=CARTESIAN_POINT ( 'NONE',  ( 778.2165204200184689, -118.8164208402383508, -364.9363028652563230 ) ) ;
#9509=CARTESIAN_POINT ( 'NONE',  ( 801.9419747391806368, -330.4527844766013231, -351.9812246680014027 ) ) ;
#9510=VERTEX_POINT ( 'NONE', #25531 ) ;
#9511=CARTESIAN_POINT ( 'NONE',  ( 781.7834795799800531, -442.8164208402372992, -315.0636971347436202 ) ) ;
#9518=CARTESIAN_POINT ( 'NONE',  ( 748.6759233522253680, -328.3726999360615650, -324.3348316497537098 ) ) ;
#9521=CARTESIAN_POINT ( 'NONE',  ( 759.9864689768902508, -338.0891481129649492, -354.9819416627836404 ) ) ;
#9524=CARTESIAN_POINT ( 'NONE',  ( 757.0176451133909268, -181.0999726633347109, -349.9200121543848354 ) ) ;
#9526=DIRECTION ( 'NONE',  ( -0.000000000000000000, -1.000000000000000000, -0.000000000000000000 ) ) ;
#9527=CARTESIAN_POINT ( 'NONE',  ( 754.9967657858570647, -385.5436935675102745, -365.0032342141425943 ) ) ;
#9532=CARTESIAN_POINT ( 'NONE',  ( 808.3070685750230950, -18.99823902205683979, -361.1904061080339261 ) ) ;
#9533=CARTESIAN_POINT ( 'NONE',  ( 797.6776695296629214, -235.5436935675107293, -357.6776695296636603 ) ) ;
#9537=CARTESIAN_POINT ( 'NONE',  ( 780.5290396650775619, -36.35105083532390324, -365.2837595273619513 ) ) ;
#9545=CARTESIAN_POINT ( 'NONE',  ( 778.2165204200184689, -70.81642084023850714, -364.9363028652563230 ) ) ;
#9546=CARTESIAN_POINT ( 'NONE',  ( 796.7845633553578182, -369.6237781080500895, -358.5707757039688204 ) ) ;
#9549=CARTESIAN_POINT ( 'NONE',  ( 748.3538107759620743, -352.7146871989593251, -355.8262568251490165 ) ) ;
#9557=CARTESIAN_POINT ( 'NONE',  ( 745.4481719005789273, -219.7255117493289447, -347.5162901302853129 ) ) ;
#9560=CARTESIAN_POINT ( 'NONE',  ( 762.3223304703356007, -223.5436935675107577, -322.3223304703362828 ) ) ;
#9562=CARTESIAN_POINT ( 'NONE',  ( 797.8594530101008786, -325.5436935675105019, -322.1405469898980982 ) ) ;
#9563=CARTESIAN_POINT ( 'NONE',  ( 763.0428371773158460, -443.4636090269702322, -358.7617431975195359 ) ) ;
#9570=CARTESIAN_POINT ( 'NONE',  ( 800.0135310231082713, 9.910851887033969021, -325.0180583372163028 ) ) ;
#9574=CARTESIAN_POINT ( 'NONE',  ( 752.7379699480933368, -228.0090635724254753, -361.9858362298580232 ) ) ;
#9577=CARTESIAN_POINT ( 'NONE',  ( 771.1735550268778070, -225.1800572038743269, -316.3353852180827630 ) ) ;
#9578=CARTESIAN_POINT ( 'NONE',  ( 755.8398074228967971, -355.4419599262319593, -333.4516893846970333 ) ) ;
#9579=CARTESIAN_POINT ( 'NONE',  ( 768.9521613784389729, -249.8272453906072315, -373.2346286133773106 ) ) ;
#9582=CARTESIAN_POINT ( 'NONE',  ( 776.9254006560222479, -68.19088175424413123, -314.8983024940802125 ) ) ;
#9586=CARTESIAN_POINT ( 'NONE',  ( 783.0433043558608688, -432.8965053807771142, -315.1538015810313027 ) ) ;
#9587=CARTESIAN_POINT ( 'NONE',  ( 814.2001403089898304, -281.3618753856923718, -347.4397851343538264 ) ) ;
#9589=DIRECTION ( 'NONE',  ( -1.000000000000000000, -0.000000000000000000, -0.000000000000000000 ) ) ;
#9590=CARTESIAN_POINT ( 'NONE',  ( 771.2633955100217236, -47.90732993114767169, -363.4237431249939618 ) ) ;
#9592=CARTESIAN_POINT ( 'NONE',  ( 781.2497674668890113, -180.3510508353234343, -375.3608509340180603 ) ) ;
#9594=CARTESIAN_POINT ( 'NONE',  ( 812.7932403749906598, -399.1800572038738437, -327.7687537140311633 ) ) ;
#9598=CARTESIAN_POINT ( 'NONE',  ( 800.2193346964447755, -426.9982390220554862, -355.1360043628815788 ) ) ;
#9603=CARTESIAN_POINT ( 'NONE',  ( 786.6156483768007774, -265.4419599262323004, -315.5913626894246136 ) ) ;
#9605=CARTESIAN_POINT ( 'NONE',  ( 793.4146539503750546, -265.9874144716867477, -307.6481478633938877 ) ) ;
#9611=CARTESIAN_POINT ( 'NONE',  ( 786.6156483768007774, -25.44195992623301450, -315.5913626894246136 ) ) ;
#9612=CARTESIAN_POINT ( 'NONE',  ( 804.6798772138708955, -159.7255117493291436, -334.6312213355107019 ) ) ;
#9614=CARTESIAN_POINT ( 'NONE',  ( 787.4397851343537695, -117.7255117493292715, -374.2001403089903988 ) ) ;
#9615=CARTESIAN_POINT ( 'NONE',  ( 762.3223304703356007, -103.5436935675111272, -322.3223304703362828 ) ) ;
#9617=CARTESIAN_POINT ( 'NONE',  ( 804.4086373105744769, -49.64542720878965554, -333.3843516231986541 ) ) ;
#9618=CARTESIAN_POINT ( 'NONE',  ( 787.5531968255692163, -357.8272453906068904, -316.1348686366205811 ) ) ;
#9625=CARTESIAN_POINT ( 'NONE',  ( 758.4439275373578084, -372.5545181178796383, -353.2243759319684386 ) ) ;
#9626=CARTESIAN_POINT ( 'NONE',  ( 762.1405469898971887, -337.5436935675102177, -357.8594530101015607 ) ) ;
#9627=CARTESIAN_POINT ( 'NONE',  ( 799.9636004259356241, -118.9181544815167229, -311.2241431872006956 ) ) ;
#9630=CARTESIAN_POINT ( 'NONE',  ( 805.1016975059191054, -270.8965053807777394, -343.0745993439771837 ) ) ;
#9631=CARTESIAN_POINT ( 'NONE',  ( 755.8990559732751535, -107.4636090269713122, -365.9055244015606831 ) ) ;
#9637=CARTESIAN_POINT ( 'NONE',  ( 787.4397851343537695, -165.7255117493291152, -374.2001403089903988 ) ) ;
#9640=CARTESIAN_POINT ( 'NONE',  ( 814.2001403089898304, -305.3618753856922581, -347.4397851343538264 ) ) ;
#9646=CARTESIAN_POINT ( 'NONE',  ( 815.0009284576459549, -390.3510508353227237, -338.7629533639073429 ) ) ;
#9647=CARTESIAN_POINT ( 'NONE',  ( 744.7301800767019131, -124.8164208402383508, -337.4774526936615757 ) ) ;
#9649=CARTESIAN_POINT ( 'NONE',  ( 792.2312462859673587, -371.9073299311465917, -307.2067596250082602 ) ) ;
#9655=CARTESIAN_POINT ( 'NONE',  ( 756.1443688327750579, -141.6237781080508569, -314.3581564841659315 ) ) ;
#9661=CARTESIAN_POINT ( 'NONE',  ( 792.3570229623688874, -21.18005720387502677, -373.1304606946836202 ) ) ;
#9664=ORIENTED_EDGE ( 'NONE', *, *, #28357, .T. ) ;
#9665=CARTESIAN_POINT ( 'NONE',  ( 752.7379699480933368, -396.0090635724249637, -361.9858362298580232 ) ) ;
#9666=CARTESIAN_POINT ( 'NONE',  ( 794.9819416627830151, -276.9982390220559978, -319.9864689768909898 ) ) ;
#9670=CARTESIAN_POINT ( 'NONE',  ( 802.9823548866075953, -265.0999726633344267, -330.0799878456151077 ) ) ;
#9671=CARTESIAN_POINT ( 'NONE',  ( 778.2165204200184689, -214.8164208402380666, -364.9363028652563230 ) ) ;
#9672=CARTESIAN_POINT ( 'NONE',  ( 804.4286716492782716, -425.3618753856919170, -345.3141322388244703 ) ) ;
#9683=CARTESIAN_POINT ( 'NONE',  ( 754.3581564841646241, -449.4636090269702322, -316.1443688327762516 ) ) ;
#9684=CARTESIAN_POINT ( 'NONE',  ( 755.2512626584698410, -79.54369356751119824, -315.2512626584710915 ) ) ;
#9686=CARTESIAN_POINT ( 'NONE',  ( 765.0180583372156207, -432.9982390220555999, -360.0135310231089534 ) ) ;
#9687=CARTESIAN_POINT ( 'NONE',  ( 778.2165204200184689, -46.81642084023858530, -364.9363028652563230 ) ) ;
#9689=FACE_OUTER_BOUND ( 'NONE', #2379, .T. ) ;
#9690=CARTESIAN_POINT ( 'NONE',  ( 766.0291762391763086, -274.9181544815161828, -360.7704444035551319 ) ) ;
#9691=CARTESIAN_POINT ( 'NONE',  ( 792.2312462859673587, -203.9073299311471885, -307.2067596250082602 ) ) ;
#9695=DIRECTION ( 'NONE',  ( 1.000000000000000000, 0.000000000000000000, -0.000000000000000000 ) ) ;
#9696=CARTESIAN_POINT ( 'NONE',  ( 778.7502325331095108, -288.3510508353231216, -304.6391490659818828 ) ) ;
#9699=CARTESIAN_POINT ( 'NONE',  ( 812.7932403749906598, -279.1800572038741848, -327.7687537140311633 ) ) ;
#9703=CARTESIAN_POINT ( 'NONE',  ( 755.0636971347428243, -340.2709662947831362, -341.7834795799807353 ) ) ;
#9705=EDGE_CURVE ( 'NONE', #14504, #24267, #32164, .T. ) ;
#9706=CARTESIAN_POINT ( 'NONE',  ( 791.1614460488616487, -35.26014174441480264, -373.5763878283158874 ) ) ;
#9707=CARTESIAN_POINT ( 'NONE',  ( 803.8651313633788504, -149.2601417444144261, -332.4468031744301015 ) ) ;
#9711=CARTESIAN_POINT ( 'NONE',  ( 774.6312213355099630, -71.36187538569302546, -364.6798772138717482 ) ) ;
#9712=CARTESIAN_POINT ( 'NONE',  ( 804.9511171171677688, -173.8055962898689302, -335.8780910478229202 ) ) ;
#9714=CARTESIAN_POINT ( 'NONE',  ( 811.6461892240364477, -4.714687198960358039, -324.1737431748509835 ) ) ;
#9720=CARTESIAN_POINT ( 'NONE',  ( 813.5763878283155464, -315.8272453906070609, -351.1614460488615350 ) ) ;
#9727=CARTESIAN_POINT ( 'NONE',  ( 804.6971507214547046, -123.2817908451530542, -344.0799538623459739 ) ) ;
#9728=CARTESIAN_POINT ( 'NONE',  ( 758.0580252608178853, -102.4527844766020337, -328.0187753319985404 ) ) ;
#9729=CARTESIAN_POINT ( 'NONE',  ( 762.1405469898973024, -313.5436935675103882, -357.8594530101016176 ) ) ;
#9730=CARTESIAN_POINT ( 'NONE',  ( 797.8594530101008786, -445.5436935675098766, -322.1405469898980982 ) ) ;
#9733=CARTESIAN_POINT ( 'NONE',  ( 792.0613484971601110, -458.0032201311295807, -367.4685979341032294 ) ) ;
#9738=CARTESIAN_POINT ( 'NONE',  ( 754.3581564841646241, -329.4636090269706870, -316.1443688327762516 ) ) ;
#9740=CARTESIAN_POINT ( 'NONE',  ( 800.0135310231082713, -326.0891481129649492, -325.0180583372163028 ) ) ;
#9742=CARTESIAN_POINT ( 'NONE',  ( 784.1219089521767955, -189.2817908451528979, -315.0488828828318333 ) ) ;
#9746=CARTESIAN_POINT ( 'NONE',  ( 749.2812353651451076, -366.4527844766012095, -323.2262854647983090 ) ) ;
#9753=CARTESIAN_POINT ( 'NONE',  ( 792.3570229623688874, -21.18005720387502677, -373.1304606946836202 ) ) ;
#9754=CARTESIAN_POINT ( 'NONE',  ( 771.2633955100217236, -239.9073299311470748, -363.4237431249939618 ) ) ;
#9758=CARTESIAN_POINT ( 'NONE',  ( 790.8726784830453198, -34.71468719896025590, -362.5472867521010585 ) ) ;
#9764=CARTESIAN_POINT ( 'NONE',  ( 757.8323909638827445, -74.63460265842032015, -352.1044303154654358 ) ) ;
#9765=CARTESIAN_POINT ( 'NONE',  ( 804.1601925771018387, -367.4419599262319025, -346.5483106153029098 ) ) ;
#9769=CARTESIAN_POINT ( 'NONE',  ( 759.8311093483677041, -358.1692326535047641, -310.9282345327691814 ) ) ;
#9774=CARTESIAN_POINT ( 'NONE',  ( 777.4774526936600978, -202.2709662947834772, -304.7301800767027657 ) ) ;
#9779=CARTESIAN_POINT ( 'NONE',  ( 771.1735550268780344, -201.1800572038744690, -316.3353852180828198 ) ) ;
#9781=CARTESIAN_POINT ( 'NONE',  ( 803.4237431249931660, -327.1800572038741279, -331.2633955100225194 ) ) ;
#9782=CARTESIAN_POINT ( 'NONE',  ( 773.4516893846965786, -451.6454272087884192, -315.8398074228977066 ) ) ;
#9785=DIRECTION ( 'NONE',  ( 0.000000000000000000, 0.000000000000000000, 1.000000000000000000 ) ) ;
#9787=FACE_OUTER_BOUND ( 'NONE', #5065, .T. ) ;
#9789=CARTESIAN_POINT ( 'NONE',  ( 769.9779781133707957, -451.0999726633339151, -316.7813123517150871 ) ) ;
#9790=CARTESIAN_POINT ( 'NONE',  ( 759.2380499001254748, 21.41625977839825978, -318.3449445151863415 ) ) ;
#9792=CARTESIAN_POINT ( 'NONE',  ( 809.0717654672305343, -244.9181544815162681, -360.1688906516309885 ) ) ;
#9795=CARTESIAN_POINT ( 'NONE',  ( 756.3353852180819104, -221.9073299311470464, -331.1735550268788302 ) ) ;
#9796=CARTESIAN_POINT ( 'NONE',  ( 773.3843516231979720, -373.4419599262319593, -364.4086373105754433 ) ) ;
#9797=CARTESIAN_POINT ( 'NONE',  ( 745.1792804349281596, -254.1908817542435770, -343.7566961878542884 ) ) ;
#9800=CARTESIAN_POINT ( 'NONE',  ( 772.4468031744293057, -81.82724539060772884, -363.8651313633793620 ) ) ;
#9804=CARTESIAN_POINT ( 'NONE',  ( 796.7845633553578182, -417.6237781080499190, -358.5707757039688204 ) ) ;
#9805=CARTESIAN_POINT ( 'NONE',  ( 763.0537975583476964, -288.4527844766014937, -371.0346526505628617 ) ) ;
#9808=CARTESIAN_POINT ( 'NONE',  ( 802.1676090361156639, -62.63460265842031305, -327.8955696845344505 ) ) ;
#9811=CARTESIAN_POINT ( 'NONE',  ( 766.5853460496234675, -157.9874144716871456, -372.3518521366060554 ) ) ;
#9813=CARTESIAN_POINT ( 'NONE',  ( 814.9108240113580450, -400.2709662947828519, -337.5031285880265273 ) ) ;
#9817=CARTESIAN_POINT ( 'NONE',  ( 765.0180583372156207, -432.9982390220555999, -360.0135310231089534 ) ) ;
#9823=CARTESIAN_POINT ( 'NONE',  ( 801.3366627262608972, -272.5328690171413086, -353.0897708529566899 ) ) ;
#9824=CARTESIAN_POINT ( 'NONE',  ( 794.9819416627830151, -132.9982390220564810, -319.9864689768909898 ) ) ;
#9826=CARTESIAN_POINT ( 'NONE',  ( 815.1787889125755555, -270.8965053807777394, -343.7953271457877804 ) ) ;
#9832=CARTESIAN_POINT ( 'NONE',  ( 775.9200461376533440, -47.80559628986931386, -315.3028492785443291 ) ) ;
#9833=CARTESIAN_POINT ( 'NONE',  ( 800.2193346964447755, -162.9982390220563673, -355.1360043628815788 ) ) ;
#9835=CARTESIAN_POINT ( 'NONE',  ( 748.9653473494363425, -98.63460265842024910, -356.9462024416521331 ) ) ;
#9837=CARTESIAN_POINT ( 'NONE',  ( 778.2165204200184689, -94.81642084023843609, -364.9363028652563230 ) ) ;
#9839=CARTESIAN_POINT ( 'NONE',  ( 805.2837595273609850, -50.73633629969874193, -340.5290396650784714 ) ) ;
#9841=CARTESIAN_POINT ( 'NONE',  ( 793.9708237608222134, -358.9181544815160123, -319.2295555964448681 ) ) ;
#9846=CARTESIAN_POINT ( 'NONE',  ( 796.1575198192839480, -342.0090635724251342, -359.4546378042384163 ) ) ;
#9847=CARTESIAN_POINT ( 'NONE',  ( 757.8323909638827445, -362.6346026584194533, -352.1044303154654358 ) ) ;
#9852=CARTESIAN_POINT ( 'NONE',  ( 755.8398074228967971, -259.4419599262322436, -333.4516893846970333 ) ) ;
#9853=CARTESIAN_POINT ( 'NONE',  ( 766.4474001241216001, -139.0999726633348530, -307.3154664389482491 ) ) ;
#9859=CARTESIAN_POINT ( 'NONE',  ( 813.1304606946831655, -185.9073299311472169, -352.3570229623691716 ) ) ;
#9862=CARTESIAN_POINT ( 'NONE',  ( 801.1904061080336987, -308.0891481129650629, -368.3070685750235498 ) ) ;
#9870=CARTESIAN_POINT ( 'NONE',  ( 766.5853460496234675, -373.9874144716864066, -372.3518521366060554 ) ) ;
#9871=CARTESIAN_POINT ( 'NONE',  ( 792.3570229623688874, -117.1800572038746964, -373.1304606946836202 ) ) ;
#9873=CARTESIAN_POINT ( 'NONE',  ( 796.9462024416508257, -396.4527844766010389, -308.9653473494370246 ) ) ;
#9877=CARTESIAN_POINT ( 'NONE',  ( 771.2368401574024119, -157.4419599262326130, -374.2805881961240857 ) ) ;
#9881=ORIENTED_EDGE ( 'NONE', *, *, #26982, .F. ) ;
#9884=CARTESIAN_POINT ( 'NONE',  ( 792.2312462859673587, -11.90732993114778182, -307.2067596250082602 ) ) ;
#9888=CARTESIAN_POINT ( 'NONE',  ( 760.0363995740630116, -418.9181544815157849, -368.7758568127991907 ) ) ;
#9889=CARTESIAN_POINT ( 'NONE',  ( 754.8072714833581358, -268.8164208402378108, -338.1981804954720587 ) ) ;
#9892=CARTESIAN_POINT ( 'NONE',  ( 787.5531968255692163, -237.8272453906072599, -316.1348686366205811 ) ) ;
#9893=CARTESIAN_POINT ( 'NONE',  ( 788.7366044899766848, -251.9073299311470748, -316.5762568750059813 ) ) ;
#9895=CARTESIAN_POINT ( 'NONE',  ( 785.3141322388236176, -405.7255117493283478, -364.4286716492789537 ) ) ;
#9896=CARTESIAN_POINT ( 'NONE',  ( 803.6646147819161570, -89.90732993114750116, -348.8264449731210561 ) ) ;
#9902=CARTESIAN_POINT ( 'NONE',  ( 762.1177392798416577, -66.55451811788050520, -309.8865473780659272 ) ) ;
#9907=EDGE_CURVE ( 'NONE', #11556, #1648, #3420, .T. ) ;
#9909=CARTESIAN_POINT ( 'NONE',  ( 802.5472867521000353, -28.37269993606244967, -350.8726784830461156 ) ) ;
#9910=CARTESIAN_POINT ( 'NONE',  ( 759.0252816721024374, -72.99823902205667991, -368.0189434323527280 ) ) ;
#9912=CARTESIAN_POINT ( 'NONE',  ( 768.0187753319979720, -416.6346026584192259, -318.0580252608186242 ) ) ;
#9913=CARTESIAN_POINT ( 'NONE',  ( 781.7834795799800531, -34.81642084023861372, -315.0636971347436202 ) ) ;
#9916=CARTESIAN_POINT ( 'NONE',  ( 787.5162901302840055, -203.3618753856925991, -305.4481719005792684 ) ) ;
#9921=CARTESIAN_POINT ( 'NONE',  ( 807.5423716828161105, -273.0783235625958696, -362.2119215644372048 ) ) ;
#9923=CARTESIAN_POINT ( 'NONE',  ( 751.6929314249748586, -270.9982390220561115, -318.8095938919659034 ) ) ;
#9927=CARTESIAN_POINT ( 'NONE',  ( 804.9363028652555840, -352.2709662947830225, -338.2165204200192079 ) ) ;
#9931=CARTESIAN_POINT ( 'NONE',  ( 801.9858362298568863, -51.07832356259657303, -312.7379699480935642 ) ) ;
#9932=CARTESIAN_POINT ( 'NONE',  ( 760.5453621957607311, -141.0783235625962959, -323.8424801807151425 ) ) ;
#9934=CARTESIAN_POINT ( 'NONE',  ( 787.4999999999992042, -512.9681489794448908, -309.9999999999998863 ) ) ;
#9937=CARTESIAN_POINT ( 'NONE',  ( 757.8323909638827445, -50.63460265842036989, -352.1044303154654358 ) ) ;
#9938=CARTESIAN_POINT ( 'NONE',  ( 764.0069404352550464, -159.0783235625962391, -359.2566176426627180 ) ) ;
#9942=CARTESIAN_POINT ( 'NONE',  ( 783.7566961878529810, -0.8965053807785533513, -305.1792804349288417 ) ) ;
#9948=CARTESIAN_POINT ( 'NONE',  ( 795.8262568251477660, -310.3726999360616219, -308.3538107759623585 ) ) ;
#9955=CARTESIAN_POINT ( 'NONE',  ( 776.9254006560222479, -164.1908817542438612, -314.8983024940802125 ) ) ;
#9956=CARTESIAN_POINT ( 'NONE',  ( 797.8594530101008786, -109.5436935675110988, -322.1405469898980982 ) ) ;
#9957=CARTESIAN_POINT ( 'NONE',  ( 797.8594530101009923, -301.5436935675105588, -322.1405469898982119 ) ) ;
#9960=CARTESIAN_POINT ( 'NONE',  ( 769.9999999999992042, 178.9475563372491251, -360.0000000000000000 ) ) ;
#9966=CARTESIAN_POINT ( 'NONE',  ( 814.2805881961230625, -361.6454272087887603, -331.2368401574024119 ) ) ;
#9971=CARTESIAN_POINT ( 'NONE',  ( 757.8323909638827445, -338.6346026584195101, -352.1044303154654358 ) ) ;
#9972=DIRECTION ( 'NONE',  ( -0.000000000000000000, 1.000000000000000000, -1.110223024625155554E-15 ) ) ;
#9973=CARTESIAN_POINT ( 'NONE',  ( 793.9708237608222134, -190.9181544815164955, -319.2295555964448681 ) ) ;
#9975=CARTESIAN_POINT ( 'NONE',  ( 758.8095938919644823, -392.0891481129647786, -311.6929314249762797 ) ) ;
#9981=CARTESIAN_POINT ( 'NONE',  ( 777.5031285880264704, -22.81642084023865280, -374.9108240113588408 ) ) ;
#9982=CARTESIAN_POINT ( 'NONE',  ( 795.1360043628807261, -236.0891481129651766, -360.2193346964456282 ) ) ;
#9988=CARTESIAN_POINT ( 'NONE',  ( 766.4474001241216001, -43.09997266333511590, -307.3154664389482491 ) ) ;
#9989=CARTESIAN_POINT ( 'NONE',  ( 801.3366627262608972, -56.53286901714201917, -353.0897708529566899 ) ) ;
#9992=DIRECTION ( 'NONE',  ( -1.000000000000000000, -0.000000000000000000, -0.000000000000000000 ) ) ;
#9996=CARTESIAN_POINT ( 'NONE',  ( 805.1927285166397041, -64.81642084023852135, -341.8018195045277707 ) ) ;
#9998=CARTESIAN_POINT ( 'NONE',  ( 754.8983024940795303, -378.8965053807772847, -336.9254006560228163 ) ) ;
#10003=CARTESIAN_POINT ( 'NONE',  ( 813.2346286133761168, -365.2601417444137155, -328.9521613784389160 ) ) ;
#10010=CARTESIAN_POINT ( 'NONE',  ( 772.5602148656447525, -201.7255117493290015, -305.7998596910095443 ) ) ;
#10013=CARTESIAN_POINT ( 'NONE',  ( 800.2193346964446619, -210.9982390220562252, -355.1360043628816925 ) ) ;
#10014=VERTEX_POINT ( 'NONE', #37968 ) ;
#10016=CARTESIAN_POINT ( 'NONE',  ( 778.1981804954714335, -322.2709662947830225, -314.8072714833589885 ) ) ;
#10017=CARTESIAN_POINT ( 'NONE',  ( 762.1405469898971887, -25.54369356751136877, -357.8594530101015607 ) ) ;
#10025=CARTESIAN_POINT ( 'NONE',  ( 803.6646147819161570, 6.092670068852159559, -348.8264449731210561 ) ) ;
#10030=CARTESIAN_POINT ( 'NONE',  ( 783.7953271457878373, -248.1908817542435202, -375.1787889125761239 ) ) ;
#10033=CARTESIAN_POINT ( 'NONE',  ( 788.8264449731200330, -213.1800572038743553, -363.6646147819171233 ) ) ;
#10034=CARTESIAN_POINT ( 'NONE',  ( 799.4546378042377910, -393.0783235625954717, -356.1575198192848006 ) ) ;
#10036=CARTESIAN_POINT ( 'NONE',  ( 800.0135310231082713, 9.910851887033969021, -325.0180583372163028 ) ) ;
#10037=CARTESIAN_POINT ( 'NONE',  ( 784.1219089521767955, -93.28179084515315367, -315.0488828828318333 ) ) ;
#10040=CARTESIAN_POINT ( 'NONE',  ( 749.8865473780648472, 3.467130982857797417, -322.1177392798429082 ) ) ;
#10041=CARTESIAN_POINT ( 'NONE',  ( 754.9967657858570647, -265.5436935675106156, -365.0032342141425943 ) ) ;
#10043=CARTESIAN_POINT ( 'NONE',  ( 804.4286716492782716, -89.36187538569299704, -345.3141322388244703 ) ) ;
#10047=CARTESIAN_POINT ( 'NONE',  ( 810.1134526219336749, -176.5328690171416213, -357.8822607201570349 ) ) ;
#10050=CARTESIAN_POINT ( 'NONE',  ( 812.7932403749906598, -423.1800572038737300, -327.7687537140311633 ) ) ;
#10051=CARTESIAN_POINT ( 'NONE',  ( 787.4999999999992042, -462.9681489794448339, -370.0000000000000568 ) ) ;
#10055=CARTESIAN_POINT ( 'NONE',  ( 791.9812246680005501, -428.6346026584192259, -361.9419747391813189 ) ) ;
#10063=CARTESIAN_POINT ( 'NONE',  ( 772.3691319403857278, -263.2601417444141134, -315.8894580844506663 ) ) ;
#10065=CARTESIAN_POINT ( 'NONE',  ( 758.0141637701419768, -255.0783235625958980, -367.2620300519063790 ) ) ;
#10068=EDGE_LOOP ( 'NONE', ( #30437, #6635, #23152, #33092 ) ) ;
#10070=CARTESIAN_POINT ( 'NONE',  ( 754.8983024940795303, -42.89650538077842157, -336.9254006560228163 ) ) ;
#10071=CARTESIAN_POINT ( 'NONE',  ( 800.0135310231082713, -206.0891481129653471, -325.0180583372163028 ) ) ;
#10073=CARTESIAN_POINT ( 'NONE',  ( 747.2067596250078623, -123.1800572038747106, -352.2312462859687230 ) ) ;
#10074=CARTESIAN_POINT ( 'NONE',  ( 759.7806653035535192, -102.9982390220565662, -324.8639956371181370 ) ) ;
#10076=CARTESIAN_POINT ( 'NONE',  ( 793.0897708529556667, -30.55451811788062244, -361.3366627262616362 ) ) ;
#10077=CARTESIAN_POINT ( 'NONE',  ( 766.9102291470427417, -354.5545181178796383, -318.6633372737382501 ) ) ;
#10084=CARTESIAN_POINT ( 'NONE',  ( 790.0220218866281812, -343.0999726633342561, -363.2186876482849129 ) ) ;
#10085=CARTESIAN_POINT ( 'NONE',  ( 762.3223304703356007, -343.5436935675103314, -322.3223304703362828 ) ) ;
#10086=CARTESIAN_POINT ( 'NONE',  ( 797.8822607201568644, -126.5545181178803205, -370.1134526219340160 ) ) ;
#10090=CARTESIAN_POINT ( 'NONE',  ( 763.2154366446407039, -309.6237781080502600, -321.4292242960311228 ) ) ;
#10091=CARTESIAN_POINT ( 'NONE',  ( 814.2805881961230625, -145.6454272087893287, -331.2368401574024119 ) ) ;
#10097=CARTESIAN_POINT ( 'NONE',  ( 763.0537975583476964, -168.4527844766018347, -371.0346526505628617 ) ) ;
#10101=CARTESIAN_POINT ( 'NONE',  ( 782.5225473063381969, -310.2709662947832499, -375.2698199232970637 ) ) ;
#10102=CARTESIAN_POINT ( 'NONE',  ( 790.0183182880230106, -452.9681489794449476, -362.9048749981275250 ) ) ;
#10107=CARTESIAN_POINT ( 'NONE',  ( 776.2433038121456548, -372.8965053807773415, -374.8207195650711014 ) ) ;
#10108=CARTESIAN_POINT ( 'NONE',  ( 808.0189434323515343, -134.0891481129655745, -319.0252816721025511 ) ) ;
#10110=CARTESIAN_POINT ( 'NONE',  ( 767.6429770376289525, -393.1800572038737300, -306.8695393053162093 ) ) ;
#10111=CYLINDRICAL_SURFACE ( 'NONE', #32804, 20.00000000000001776 ) ;
#10115=CARTESIAN_POINT ( 'NONE',  ( 815.1787889125755555, -150.8965053807781089, -343.7953271457877804 ) ) ;
#10122=CARTESIAN_POINT ( 'NONE',  ( 758.8095938919642549, -8.089148112965974136, -311.6929314249763365 ) ) ;
#10125=CARTESIAN_POINT ( 'NONE',  ( 797.6776695296629214, -187.5436935675108430, -357.6776695296636603 ) ) ;
#10126=CARTESIAN_POINT ( 'NONE',  ( 754.3581564841646241, -401.4636090269704027, -316.1443688327762516 ) ) ;
#10128=CARTESIAN_POINT ( 'NONE',  ( 759.9864689768902508, -266.0891481129651197, -354.9819416627836404 ) ) ;
#10132=CARTESIAN_POINT ( 'NONE',  ( 804.1105419155481968, -243.8272453906072030, -347.6308680596136469 ) ) ;
#10133=CARTESIAN_POINT ( 'NONE',  ( 756.5762568750052424, -267.1800572038742985, -348.7366044899774238 ) ) ;
#10134=CARTESIAN_POINT ( 'NONE',  ( 802.1676090361155502, -446.6346026584191122, -327.8955696845344505 ) ) ;
#10135=CARTESIAN_POINT ( 'NONE',  ( 802.1676090361156639, -86.63460265842023489, -327.8955696845344505 ) ) ;
#10140=CARTESIAN_POINT ( 'NONE',  ( 748.6759233522253680, -40.37269993606240348, -324.3348316497537098 ) ) ;
#10146=CARTESIAN_POINT ( 'NONE',  ( 804.8461984189677878, -2.190881754244347945, -336.9566956441385628 ) ) ;
#10147=CARTESIAN_POINT ( 'NONE',  ( 745.7998596910086917, -77.36187538569302546, -332.5602148656461168 ) ) ;
#10149=CARTESIAN_POINT ( 'NONE',  ( 805.1927285166397041, -448.8164208402371855, -341.8018195045277707 ) ) ;
#10150=CARTESIAN_POINT ( 'NONE',  ( 757.8323909638828582, -26.63460265842046226, -352.1044303154654358 ) ) ;
#10152=CARTESIAN_POINT ( 'NONE',  ( 745.4481719005789273, -195.7255117493289731, -347.5162901302853129 ) ) ;
#10156=CARTESIAN_POINT ( 'NONE',  ( 754.0944755984390895, -279.6237781080503737, -364.1009440267246760 ) ) ;
#10158=CARTESIAN_POINT ( 'NONE',  ( 808.3070685750230950, -282.9982390220558841, -361.1904061080339261 ) ) ;
#10162=CARTESIAN_POINT ( 'NONE',  ( 759.9864689768902508, -386.0891481129647786, -354.9819416627836404 ) ) ;
#10164=CARTESIAN_POINT ( 'NONE',  ( 781.2497674668890113, -60.35105083532383219, -375.3608509340180603 ) ) ;
#10165=CARTESIAN_POINT ( 'NONE',  ( 757.2208543904082489, -184.7146871989598083, -350.9844846989624330 ) ) ;
#10168=ORIENTED_EDGE ( 'NONE', *, *, #21300, .T. ) ;
#10169=CARTESIAN_POINT ( 'NONE',  ( 762.1405469898971887, -73.54369356751118403, -357.8594530101015607 ) ) ;
#10170=CARTESIAN_POINT ( 'NONE',  ( 793.2243759319678702, -194.5328690171415644, -318.4439275373583200 ) ) ;
#10172=CARTESIAN_POINT ( 'NONE',  ( 747.3154664389472828, 4.012585528312341054, -326.4474001241230781 ) ) ;
#10178=CARTESIAN_POINT ( 'NONE',  ( 745.7194118038753459, -301.6454272087889308, -348.7631598425976449 ) ) ;
#10183=CARTESIAN_POINT ( 'NONE',  ( 780.5236548040995785, -140.7363362996984506, -314.9735926884559944 ) ) ;
#10184=CARTESIAN_POINT ( 'NONE',  ( 804.4286716492782716, -137.3618753856928265, -345.3141322388244703 ) ) ;
#10185=CARTESIAN_POINT ( 'NONE',  ( 759.7806653035535192, -318.9982390220558841, -324.8639956371181370 ) ) ;
#10192=CARTESIAN_POINT ( 'NONE',  ( 804.1009440267234822, -383.4636090269704596, -314.0944755984392600 ) ) ;
#10197=CARTESIAN_POINT ( 'NONE',  ( 805.1927285166397041, -328.8164208402375834, -341.8018195045277707 ) ) ;
#10199=CARTESIAN_POINT ( 'NONE',  ( 766.0291762391763086, -226.9181544815163534, -360.7704444035551319 ) ) ;
#10202=CARTESIAN_POINT ( 'NONE',  ( 751.9810565676468741, -410.0891481129647218, -360.9747183278973921 ) ) ;
#10206=CARTESIAN_POINT ( 'NONE',  ( 804.6401732501814195, -455.9581923679652391, -357.6484231659003967 ) ) ;
#10208=CARTESIAN_POINT ( 'NONE',  ( 814.5518280994195948, -63.72551174932939233, -332.4837098697145734 ) ) ;
#10209=CARTESIAN_POINT ( 'NONE',  ( 801.9419747391806368, -282.4527844766014937, -351.9812246680014027 ) ) ;
#10213=CARTESIAN_POINT ( 'NONE',  ( 807.2620300519052989, -24.00906357242609346, -318.0141637701419768 ) ) ;
#10214=CARTESIAN_POINT ( 'NONE',  ( 754.8983024940795303, -66.89650538077835051, -336.9254006560228163 ) ) ;
#10218=DIRECTION ( 'NONE',  ( 0.000000000000000000, 0.000000000000000000, -1.000000000000000000 ) ) ;
#10221=CARTESIAN_POINT ( 'NONE',  ( 759.9864689768902508, -74.08914811296577341, -354.9819416627836404 ) ) ;
#10222=CARTESIAN_POINT ( 'NONE',  ( 756.7813123517142913, -355.9874144716865203, -329.9779781133712504 ) ) ;
#10225=CARTESIAN_POINT ( 'NONE',  ( 813.9316612368132837, -391.4419599262317888, -348.6739635108323228 ) ) ;
#10230=CARTESIAN_POINT ( 'NONE',  ( 744.7301800767019131, -220.8164208402379529, -337.4774526936615757 ) ) ;
#10234=CARTESIAN_POINT ( 'NONE',  ( 756.3353852180820240, -197.9073299311472169, -331.1735550268787733 ) ) ;
#10237=CARTESIAN_POINT ( 'NONE',  ( 765.0180583372156207, -360.9982390220557704, -360.0135310231089534 ) ) ;
#10238=CARTESIAN_POINT ( 'NONE',  ( 771.2633955100217236, -23.90732993114773919, -363.4237431249939618 ) ) ;
#10244=CARTESIAN_POINT ( 'NONE',  ( 771.2633955100217236, 0.09267006885218045942, -363.4237431249939618 ) ) ;
#10245=DIRECTION ( 'NONE',  ( -0.7014439490181307857, 0.1263042864341424876, -0.7014439490181749726 ) ) ;
#10248=CARTESIAN_POINT ( 'NONE',  ( 812.3518521366052028, -289.0999726633343698, -326.5853460496235243 ) ) ;
#10251=CARTESIAN_POINT ( 'NONE',  ( 792.1044303154645831, -228.4527844766015789, -317.8323909638837677 ) ) ;
#10252=CARTESIAN_POINT ( 'NONE',  ( 776.9566956441375396, -396.8965053807772847, -364.8461984189686405 ) ) ;
#10254=CARTESIAN_POINT ( 'NONE',  ( 803.4237431249931660, 8.819942796124882634, -331.2633955100225194 ) ) ;
#10255=CARTESIAN_POINT ( 'NONE',  ( 760.7433823573367135, -108.0090635724258448, -355.9930595647440441 ) ) ;
#10259=CARTESIAN_POINT ( 'NONE',  ( 793.4146539503750546, -1.987414471687640294, -307.6481478633938877 ) ) ;
#10260=CARTESIAN_POINT ( 'NONE',  ( 747.2067596250078623, -315.1800572038740711, -352.2312462859687230 ) ) ;
#10263=CARTESIAN_POINT ( 'NONE',  ( 800.2193346964447755, -66.99823902205672255, -355.1360043628815788 ) ) ;
#10265=CARTESIAN_POINT ( 'NONE',  ( 746.7653713866222915, -161.2601417444143976, -351.0478386215610271 ) ) ;
#10267=CARTESIAN_POINT ( 'NONE',  ( 810.4231160770870019, -0.5545181178807169209, -321.9338519418446936 ) ) ;
#10272=CARTESIAN_POINT ( 'NONE',  ( 762.1405469898971887, -409.5436935675101040, -357.8594530101015607 ) ) ;
#10280=CARTESIAN_POINT ( 'NONE',  ( 775.9200461376533440, -263.8055962898686175, -315.3028492785443291 ) ) ;
#10282=CARTESIAN_POINT ( 'NONE',  ( 791.1614460488616487, -275.2601417444140566, -373.5763878283158874 ) ) ;
#10287=CARTESIAN_POINT ( 'NONE',  ( 769.1273215169530886, -46.71468719896022748, -317.4527132478988847 ) ) ;
#10288=CARTESIAN_POINT ( 'NONE',  ( 755.5713283507202505, -197.3618753856926560, -334.6858677611754729 ) ) ;
#10290=CARTESIAN_POINT ( 'NONE',  ( 754.9967657858570647, -97.54369356751112718, -365.0032342141425374 ) ) ;
#10291=CARTESIAN_POINT ( 'NONE',  ( 755.3201227861273992, -99.72551174932931417, -345.3687786644892981 ) ) ;
#10293=CARTESIAN_POINT ( 'NONE',  ( 800.9840315886518738, -52.91815448151692891, -354.1144889064786412 ) ) ;
#10294=CARTESIAN_POINT ( 'NONE',  ( 754.7162404726377645, -374.7363362996978253, -339.4709603349214717 ) ) ;
#10303=ORIENTED_EDGE ( 'NONE', *, *, #17898, .T. ) ;
#10304=CARTESIAN_POINT ( 'NONE',  ( 804.1105419155481968, -363.8272453906068336, -347.6308680596136469 ) ) ;
#10305=CARTESIAN_POINT ( 'NONE',  ( 797.8594530101008786, -349.5436935675102745, -322.1405469898980982 ) ) ;
#10306=CARTESIAN_POINT ( 'NONE',  ( 748.6759233522253680, -160.3726999360620482, -324.3348316497537098 ) ) ;
#10311=CARTESIAN_POINT ( 'NONE',  ( 759.2295555964440155, -280.1692326535049347, -353.9708237608231229 ) ) ;
#10312=CARTESIAN_POINT ( 'NONE',  ( 800.0135310231082713, -446.0891481129646081, -325.0180583372163028 ) ) ;
#10313=CARTESIAN_POINT ( 'NONE',  ( 812.3518521366052028, -145.0999726633347677, -326.5853460496235243 ) ) ;
#10319=CARTESIAN_POINT ( 'NONE',  ( 745.7998596910086917, -197.3618753856926560, -332.5602148656461168 ) ) ;
#10322=CARTESIAN_POINT ( 'NONE',  ( 748.9653473494363425, -314.6346026584194533, -356.9462024416521331 ) ) ;
#10326=ORIENTED_EDGE ( 'NONE', *, *, #38314, .T. ) ;
#10328=CARTESIAN_POINT ( 'NONE',  ( 798.0661480581538854, -362.5328690171410813, -309.5768839229118043 ) ) ;
#10329=CARTESIAN_POINT ( 'NONE',  ( 813.1304606946830518, -137.9073299311473875, -352.3570229623690580 ) ) ;
#10330=CARTESIAN_POINT ( 'NONE',  ( 796.7737145352015204, -428.6346026584192259, -370.7187646348536987 ) ) ;
#10335=CARTESIAN_POINT ( 'NONE',  ( 744.9990715423526808, -162.3510508353235196, -341.2370466360926002 ) ) ;
#10341=CARTESIAN_POINT ( 'NONE',  ( 763.0537975583475827, -24.45278447660229304, -371.0346526505627480 ) ) ;
#10344=CARTESIAN_POINT ( 'NONE',  ( 791.0478386215596629, -405.8272453906067199, -306.7653713866226326 ) ) ;
#10348=CARTESIAN_POINT ( 'NONE',  ( 755.5713283507202505, -245.3618753856925139, -334.6858677611754729 ) ) ;
#10352=CARTESIAN_POINT ( 'NONE',  ( 772.4468031744293057, -249.8272453906072315, -363.8651313633793620 ) ) ;
#10353=CARTESIAN_POINT ( 'NONE',  ( 754.8072714833581358, -268.8164208402378108, -338.1981804954720587 ) ) ;
#10354=CARTESIAN_POINT ( 'NONE',  ( 795.1360043628808398, -452.0891481129646081, -360.2193346964456282 ) ) ;
#10355=CARTESIAN_POINT ( 'NONE',  ( 792.1044303154645831, -84.45278447660206211, -317.8323909638837677 ) ) ;
#10359=DIRECTION ( 'NONE',  ( -1.000000000000000000, 0.000000000000000000, 0.000000000000000000 ) ) ;
#10360=CARTESIAN_POINT ( 'NONE',  ( 771.3260364891663130, -43.64542720878966975, -306.0683387631859773 ) ) ;
#10367=CARTESIAN_POINT ( 'NONE',  ( 800.9840315886518738, -4.918154481517067467, -354.1144889064786412 ) ) ;
#10368=CARTESIAN_POINT ( 'NONE',  ( 792.2312462859673587, -59.90732993114762905, -307.2067596250082602 ) ) ;
#10370=CARTESIAN_POINT ( 'NONE',  ( 800.2193346964447755, -450.9982390220554294, -355.1360043628815788 ) ) ;
#10372=CARTESIAN_POINT ( 'NONE',  ( 772.4837098697144029, -215.3618753856925423, -374.5518280994205611 ) ) ;
#10376=CARTESIAN_POINT ( 'NONE',  ( 746.0683387631852383, -259.4419599262322436, -331.3260364891676204 ) ) ;
#10378=CARTESIAN_POINT ( 'NONE',  ( 749.2812353651451076, -294.4527844766013800, -323.2262854647983090 ) ) ;
#10382=CARTESIAN_POINT ( 'NONE',  ( 812.6845335610512393, -31.98741447168754348, -353.5525998758768651 ) ) ;
#10383=CARTESIAN_POINT ( 'NONE',  ( 754.8072714833581358, -388.8164208402374129, -338.1981804954720587 ) ) ;
#10385=CARTESIAN_POINT ( 'NONE',  ( 755.5713283507202505, -197.3618753856926560, -334.6858677611754729 ) ) ;
#10386=CARTESIAN_POINT ( 'NONE',  ( 766.5853460496234675, -37.98741447168752927, -372.3518521366060554 ) ) ;
#10387=CARTESIAN_POINT ( 'NONE',  ( 799.4546378042377910, -201.0783235625961254, -356.1575198192848006 ) ) ;
#10391=CARTESIAN_POINT ( 'NONE',  ( 805.1927285166397041, -88.81642084023842187, -341.8018195045277707 ) ) ;
#10392=CARTESIAN_POINT ( 'NONE',  ( 757.2208543904082489, -208.7146871989596946, -350.9844846989624330 ) ) ;
#10395=CARTESIAN_POINT ( 'NONE',  ( 771.2368401574024119, -37.44195992623299674, -374.2805881961240857 ) ) ;
#10400=CARTESIAN_POINT ( 'NONE',  ( 744.6391490659812007, -302.7363362996979959, -338.7502325331110455 ) ) ;
#10404=CARTESIAN_POINT ( 'NONE',  ( 790.0220218866281812, -151.0999726633347677, -363.2186876482849129 ) ) ;
#10405=CARTESIAN_POINT ( 'NONE',  ( 785.3687786644884454, -131.3618753856928834, -315.3201227861279676 ) ) ;
#10406=CARTESIAN_POINT ( 'NONE',  ( 804.6798772138710092, -351.7255117493284615, -334.6312213355106451 ) ) ;
#10408=CARTESIAN_POINT ( 'NONE',  ( 805.1927285166397041, -448.8164208402371855, -341.8018195045277707 ) ) ;
#10415=CARTESIAN_POINT ( 'NONE',  ( 752.7379699480933368, -372.0090635724250205, -361.9858362298580232 ) ) ;
#10420=CARTESIAN_POINT ( 'NONE',  ( 767.8955696845333705, -336.4527844766012095, -362.1676090361162323 ) ) ;
#10421=CARTESIAN_POINT ( 'NONE',  ( 758.4439275373578084, -204.5545181178800931, -353.2243759319684386 ) ) ;
#10425=CARTESIAN_POINT ( 'NONE',  ( 763.2262854647970016, -416.6346026584192259, -309.2812353651462445 ) ) ;
#10430=CARTESIAN_POINT ( 'NONE',  ( 804.7487373415286811, -43.54369356751131903, -364.7487373415288516 ) ) ;
#10431=CARTESIAN_POINT ( 'NONE',  ( 781.7834795799800531, -274.8164208402378108, -315.0636971347436202 ) ) ;
#10437=CARTESIAN_POINT ( 'NONE',  ( 745.7194118038753459, -37.64542720878968396, -348.7631598425976449 ) ) ;
#10438=CARTESIAN_POINT ( 'NONE',  ( 798.7617431975189675, -99.62377810805098477, -323.0428371773161871 ) ) ;
#10443=CARTESIAN_POINT ( 'NONE',  ( 805.1927285166397041, 7.183579159761247723, -341.8018195045277707 ) ) ;
#10444=CARTESIAN_POINT ( 'NONE',  ( 803.2186876482843445, -103.9874144716873161, -350.0220218866286928 ) ) ;
#10446=CARTESIAN_POINT ( 'NONE',  ( 800.0135310231082713, -62.08914811296580183, -325.0180583372163028 ) ) ;
#10447=CARTESIAN_POINT ( 'NONE',  ( 800.7704444035546203, -388.1692326535045936, -326.0291762391768771 ) ) ;
#10450=CARTESIAN_POINT ( 'NONE',  ( 759.8311093483677041, -382.1692326535045936, -310.9282345327691814 ) ) ;
#10455=CARTESIAN_POINT ( 'NONE',  ( 772.4837098697144029, -239.3618753856924570, -374.5518280994205611 ) ) ;
#10458=CARTESIAN_POINT ( 'NONE',  ( 762.1405469898973024, -241.5436935675106440, -357.8594530101016176 ) ) ;
#10461=CARTESIAN_POINT ( 'NONE',  ( 762.3223304703356007, -367.5436935675102745, -322.3223304703362828 ) ) ;
#10462=CARTESIAN_POINT ( 'NONE',  ( 797.8594530101008786, -13.54369356751140785, -322.1405469898980982 ) ) ;
#10467=CARTESIAN_POINT ( 'NONE',  ( 774.6312213355099630, -23.36187538569318889, -364.6798772138717482 ) ) ;
#10471=CARTESIAN_POINT ( 'NONE',  ( 771.3260364891663130, -259.6454272087890445, -306.0683387631859773 ) ) ;
#10475=CARTESIAN_POINT ( 'NONE',  ( 785.3141322388236176, -237.7255117493289163, -364.4286716492789537 ) ) ;
#10476=CARTESIAN_POINT ( 'NONE',  ( 775.9200461376533440, -407.8055962898681628, -315.3028492785443291 ) ) ;
#10479=CARTESIAN_POINT ( 'NONE',  ( 766.0291762391763086, -106.9181544815167371, -360.7704444035551319 ) ) ;
#10482=CARTESIAN_POINT ( 'NONE',  ( 803.8556311672234642, 14.37622189194867417, -365.6418435158340117 ) ) ;
#10483=CARTESIAN_POINT ( 'NONE',  ( 814.2001403089898304, -305.3618753856922581, -347.4397851343538264 ) ) ;
#10486=CARTESIAN_POINT ( 'NONE',  ( 791.9812246680005501, -92.63460265842026331, -361.9419747391813189 ) ) ;
#10488=CARTESIAN_POINT ( 'NONE',  ( 801.9858362298568863, -195.0783235625961538, -312.7379699480935642 ) ) ;
#10490=CARTESIAN_POINT ( 'NONE',  ( 801.1904061080336987, -452.0891481129646650, -368.3070685750235498 ) ) ;
#10495=CARTESIAN_POINT ( 'NONE',  ( 794.9819416627830151, -444.9982390220554862, -319.9864689768909898 ) ) ;
#10501=CARTESIAN_POINT ( 'NONE',  ( 803.8651313633788504, -245.2601417444141987, -332.4468031744301015 ) ) ;
#10503=CARTESIAN_POINT ( 'NONE',  ( 768.8385539511368734, -287.2601417444140566, -306.4236121716840557 ) ) ;
#10508=CARTESIAN_POINT ( 'NONE',  ( 786.6156483768007774, -49.44195992623295410, -315.5913626894246136 ) ) ;
#10509=CARTESIAN_POINT ( 'NONE',  ( 768.0187753319979720, -152.6346026584200786, -318.0580252608186242 ) ) ;
#10510=CARTESIAN_POINT ( 'NONE',  ( 764.8639956371174549, -200.0891481129653187, -319.7806653035542013 ) ) ;
#10513=CARTESIAN_POINT ( 'NONE',  ( 800.9747183278959710, -132.9982390220564810, -311.9810565676471583 ) ) ;
#10514=CARTESIAN_POINT ( 'NONE',  ( 755.0636971347428243, -100.2709662947838609, -341.7834795799807353 ) ) ;
#10515=ORIENTED_EDGE ( 'NONE', *, *, #28565, .F. ) ;
#10516=CARTESIAN_POINT ( 'NONE',  ( 766.0291762391763086, -394.9181544815158418, -360.7704444035551319 ) ) ;
#10524=CARTESIAN_POINT ( 'NONE',  ( 800.9840315886518738, -364.9181544815158986, -354.1144889064786412 ) ) ;
#10525=CARTESIAN_POINT ( 'NONE',  ( 762.3223304703356007, -367.5436935675102745, -322.3223304703362828 ) ) ;
#10527=CARTESIAN_POINT ( 'NONE',  ( 802.2119215644370342, -174.0090635724256742, -367.5423716828165084 ) ) ;
#10531=CARTESIAN_POINT ( 'NONE',  ( 765.8855110935204493, -286.1692326535048778, -319.0159684113471599 ) ) ;
#10533=CARTESIAN_POINT ( 'NONE',  ( 791.0478386215596629, -165.8272453906074873, -306.7653713866226326 ) ) ;
#10538=CARTESIAN_POINT ( 'NONE',  ( 810.7187646348534145, -210.4527844766016926, -356.7737145352016341 ) ) ;
#10542=CARTESIAN_POINT ( 'NONE',  ( 751.2241431872005251, -112.1692326535054889, -359.9636004259367610 ) ) ;
#10543=CARTESIAN_POINT ( 'NONE',  ( 747.2067596250078623, -339.1800572038740142, -352.2312462859687230 ) ) ;
#10549=CARTESIAN_POINT ( 'NONE',  ( 814.8230680027162407, -389.8055962898682765, -333.7305795820267917 ) ) ;
#10550=CARTESIAN_POINT ( 'NONE',  ( 767.7687537140311633, -143.9073299311473590, -372.7932403749916830 ) ) ;
#10552=CARTESIAN_POINT ( 'NONE',  ( 751.6929314249748586, -438.9982390220553157, -318.8095938919659034 ) ) ;
#10553=CARTESIAN_POINT ( 'NONE',  ( 779.9999999999992042, -462.9681489794448339, -339.9999999999999432 ) ) ;
#10558=CARTESIAN_POINT ( 'NONE',  ( 801.9858362298568863, -195.0783235625961538, -312.7379699480935642 ) ) ;
#10562=CARTESIAN_POINT ( 'NONE',  ( 779.9999999999992042, 126.4563064324884465, -370.0000000000000568 ) ) ;
#10567=CARTESIAN_POINT ( 'NONE',  ( 745.7998596910086917, -5.361875385693257279, -332.5602148656461168 ) ) ;
#10570=ADVANCED_BREP_SHAPE_REPRESENTATION ( '', ( #33039, #26858 ), #7704 ) ;
#10571=CARTESIAN_POINT ( 'NONE',  ( 752.7379699480933368, -420.0090635724249069, -361.9858362298580232 ) ) ;
#10576=CARTESIAN_POINT ( 'NONE',  ( 788.8264449731200330, -261.1800572038741848, -363.6646147819171233 ) ) ;
#10580=CARTESIAN_POINT ( 'NONE',  ( 766.0291762391763086, -250.9181544815163534, -360.7704444035551319 ) ) ;
#10581=CARTESIAN_POINT ( 'NONE',  ( 764.8639956371174549, -248.0891481129651481, -319.7806653035542013 ) ) ;
#10583=CARTESIAN_POINT ( 'NONE',  ( 778.1981804954714335, -106.2709662947838467, -314.8072714833589885 ) ) ;
#10589=DIRECTION ( 'NONE',  ( 0.000000000000000000, 0.000000000000000000, -1.000000000000000000 ) ) ;
#10591=CARTESIAN_POINT ( 'NONE',  ( 762.1177392798416577, -42.55451811788057626, -309.8865473780659272 ) ) ;
#10596=EDGE_LOOP ( 'NONE', ( #11366, #2720 ) ) ;
#10597=CARTESIAN_POINT ( 'NONE',  ( 793.9708237608222134, -22.91815448151701062, -319.2295555964448681 ) ) ;
#10599=CARTESIAN_POINT ( 'NONE',  ( 813.1304606946831655, -113.9073299311474585, -352.3570229623691716 ) ) ;
#10602=FACE_OUTER_BOUND ( 'NONE', #657, .T. ) ;
#10604=CARTESIAN_POINT ( 'NONE',  ( 787.5162901302840055, -251.3618753856923149, -305.4481719005792684 ) ) ;
#10608=CARTESIAN_POINT ( 'NONE',  ( 751.2241431872005251, -280.1692326535049347, -359.9636004259367610 ) ) ;
#10611=CARTESIAN_POINT ( 'NONE',  ( 782.5225473063381969, -334.2709662947829656, -375.2698199232970637 ) ) ;
#10615=CARTESIAN_POINT ( 'NONE',  ( 805.1927285166397041, -376.8164208402375834, -341.8018195045277707 ) ) ;
#10618=CARTESIAN_POINT ( 'NONE',  ( 774.6858677611749044, -201.7255117493290015, -315.5713283507209894 ) ) ;
#10619=CARTESIAN_POINT ( 'NONE',  ( 795.6651683502461765, -34.71468719896025590, -371.3240766477733814 ) ) ;
#10624=CARTESIAN_POINT ( 'NONE',  ( 794.1144889064781864, -202.1692326535051905, -360.9840315886528401 ) ) ;
#10626=CARTESIAN_POINT ( 'NONE',  ( 759.8311093483677041, -46.16923265350568784, -310.9282345327691814 ) ) ;
#10632=CARTESIAN_POINT ( 'NONE',  ( 745.1792804349281596, -302.1908817542433781, -343.7566961878542884 ) ) ;
#10635=CARTESIAN_POINT ( 'NONE',  ( 754.7162404726377645, -158.7363362996984222, -339.4709603349214717 ) ) ;
#10636=CARTESIAN_POINT ( 'NONE',  ( 785.3141322388236176, -141.7255117493291721, -364.4286716492789537 ) ) ;
#10637=CARTESIAN_POINT ( 'NONE',  ( 758.0580252608178853, -342.4527844766013231, -328.0187753319985404 ) ) ;
#10648=CARTESIAN_POINT ( 'NONE',  ( 811.3240766477731540, -388.3726999360613945, -355.6651683502462902 ) ) ;
#10649=CARTESIAN_POINT ( 'NONE',  ( 754.9967657858570647, -1.543693567511449594, -365.0032342141425943 ) ) ;
#10653=CARTESIAN_POINT ( 'NONE',  ( 800.2193346964447755, -378.9982390220555999, -355.1360043628815788 ) ) ;
#10656=CARTESIAN_POINT ( 'NONE',  ( 755.1538015810308480, -206.1908817542437191, -343.0433043558613804 ) ) ;
#10660=CARTESIAN_POINT ( 'NONE',  ( 758.8095938919644823, -416.0891481129646650, -311.6929314249762797 ) ) ;
#10666=CARTESIAN_POINT ( 'NONE',  ( 767.7687537140311633, -47.90732993114767169, -372.7932403749916830 ) ) ;
#10667=CARTESIAN_POINT ( 'NONE',  ( 795.1360043628807261, -284.0891481129650629, -360.2193346964456282 ) ) ;
#10671=CARTESIAN_POINT ( 'NONE',  ( 748.6759233522253680, -16.37269993606248519, -324.3348316497537098 ) ) ;
#10672=CARTESIAN_POINT ( 'NONE',  ( 783.0433043558608688, -72.89650538077830788, -315.1538015810313027 ) ) ;
#10675=CIRCLE ( 'NONE', #31345, 30.00000000000008171 ) ;
#10677=CARTESIAN_POINT ( 'NONE',  ( 778.2165204200184689, 1.183579159761269040, -364.9363028652563230 ) ) ;
#10679=CARTESIAN_POINT ( 'NONE',  ( 803.6646147819161570, -89.90732993114750116, -348.8264449731210561 ) ) ;
#10680=VECTOR ( 'NONE', #24349, 1000.000000000000000 ) ;
#10681=CARTESIAN_POINT ( 'NONE',  ( 795.9930595647434757, -411.0783235625954717, -320.7433823573372820 ) ) ;
#10684=CARTESIAN_POINT ( 'NONE',  ( 798.0661480581538854, -386.5328690171409676, -309.5768839229118043 ) ) ;
#10690=CARTESIAN_POINT ( 'NONE',  ( 767.6429770376289525, -249.1800572038742416, -306.8695393053162093 ) ) ;
#10695=CARTESIAN_POINT ( 'NONE',  ( 768.0187753319979720, -248.6346026584197659, -318.0580252608186242 ) ) ;
#10698=CARTESIAN_POINT ( 'NONE',  ( 756.3353852180819104, -365.9073299311465917, -331.1735550268788302 ) ) ;
#10699=CARTESIAN_POINT ( 'NONE',  ( 759.9864689768902508, -26.08914811296592262, -354.9819416627836404 ) ) ;
#10705=CARTESIAN_POINT ( 'NONE',  ( 756.5762568750052424, -3.180057203875080063, -348.7366044899774238 ) ) ;
#10708=CARTESIAN_POINT ( 'NONE',  ( 744.6391490659812007, -278.7363362996980527, -338.7502325331110455 ) ) ;
#10713=CARTESIAN_POINT ( 'NONE',  ( 795.1360043628807261, -260.0891481129650060, -360.2193346964456282 ) ) ;
#10714=CARTESIAN_POINT ( 'NONE',  ( 786.6156483768007774, -409.4419599262317320, -315.5913626894246136 ) ) ;
#10716=CARTESIAN_POINT ( 'NONE',  ( 757.0176451133909268, -109.0999726633349241, -349.9200121543848354 ) ) ;
#10721=CARTESIAN_POINT ( 'NONE',  ( 768.8385539511368734, 0.7398582555850804487, -306.4236121716840557 ) ) ;
#10722=CARTESIAN_POINT ( 'NONE',  ( 808.3070685750232087, -306.9982390220558841, -361.1904061080339829 ) ) ;
#10725=CARTESIAN_POINT ( 'NONE',  ( 774.6312213355099630, -95.36187538569294020, -364.6798772138717482 ) ) ;
#10727=CARTESIAN_POINT ( 'NONE',  ( 771.2368401574024119, -205.4419599262324425, -374.2805881961240857 ) ) ;
#10729=CARTESIAN_POINT ( 'NONE',  ( 791.0478386215596629, 2.172754609392001601, -306.7653713866226326 ) ) ;
#10734=CARTESIAN_POINT ( 'NONE',  ( 784.0799538623451781, 12.19440371013049784, -364.6971507214555572 ) ) ;
#10741=CARTESIAN_POINT ( 'NONE',  ( 755.0488828828309806, -281.8055962898686175, -344.1219089521771934 ) ) ;
#10744=CARTESIAN_POINT ( 'NONE',  ( 801.9858362298568863, -291.0783235625957559, -312.7379699480935642 ) ) ;
#10750=CARTESIAN_POINT ( 'NONE',  ( 757.2208543904082489, -40.71468719896024879, -350.9844846989624330 ) ) ;
#10751=CARTESIAN_POINT ( 'NONE',  ( 792.1044303154645831, -156.4527844766018916, -317.8323909638837677 ) ) ;
#10752=CARTESIAN_POINT ( 'NONE',  ( 755.0636971347428243, -220.2709662947834772, -341.7834795799807353 ) ) ;
#10755=CARTESIAN_POINT ( 'NONE',  ( 813.1304606946830518, -161.9073299311472454, -352.3570229623690580 ) ) ;
#10757=CARTESIAN_POINT ( 'NONE',  ( 800.0135310231082713, -134.0891481129655745, -325.0180583372163028 ) ) ;
#10759=CARTESIAN_POINT ( 'NONE',  ( 757.0176451133909268, -397.0999726633340288, -349.9200121543848354 ) ) ;
#10767=CARTESIAN_POINT ( 'NONE',  ( 796.9571628226829034, -407.4636090269703459, -321.2382568024804641 ) ) ;
#10768=CARTESIAN_POINT ( 'NONE',  ( 803.6646147819161570, -353.9073299311467053, -348.8264449731210561 ) ) ;
#10769=CARTESIAN_POINT ( 'NONE',  ( 812.3518521366052028, -169.0999726633347393, -326.5853460496235243 ) ) ;
#10774=CARTESIAN_POINT ( 'NONE',  ( 801.3366627262608972, -296.5328690171411949, -353.0897708529566899 ) ) ;
#10775=CARTESIAN_POINT ( 'NONE',  ( 789.5670355615794733, -453.0432664090020012, -363.0970091259334822 ) ) ;
#10776=CARTESIAN_POINT ( 'NONE',  ( 809.0717654672305343, -172.9181544815165239, -360.1688906516309885 ) ) ;
#10782=CARTESIAN_POINT ( 'NONE',  ( 782.4968714119720516, -202.8164208402380950, -305.0891759886411023 ) ) ;
#10783=ADVANCED_FACE ( 'NONE', ( #29841, #1214 ), #15322, .T. ) ;
#10785=CARTESIAN_POINT ( 'NONE',  ( 794.9819416627830151, 11.00176097794305541, -319.9864689768909898 ) ) ;
#10788=CARTESIAN_POINT ( 'NONE',  ( 759.8311093483677041, -94.16923265350555994, -310.9282345327691814 ) ) ;
#10790=CARTESIAN_POINT ( 'NONE',  ( 792.2312462859673587, -347.9073299311467053, -307.2067596250082602 ) ) ;
#10793=CARTESIAN_POINT ( 'NONE',  ( 799.9999999999993179, -512.9681489794448908, -339.9999999999999432 ) ) ;
#10797=CARTESIAN_POINT ( 'NONE',  ( 776.2433038121456548, -396.8965053807772847, -374.8207195650711014 ) ) ;
#10798=CARTESIAN_POINT ( 'NONE',  ( 767.7687537140311633, -407.9073299311465348, -372.7932403749916830 ) ) ;
#10802=CARTESIAN_POINT ( 'NONE',  ( 759.8311093483677041, -190.1692326535052189, -310.9282345327691814 ) ) ;
#10810=CARTESIAN_POINT ( 'NONE',  ( 751.6929314249748586, -30.99823902205680071, -318.8095938919659034 ) ) ;
#10814=CARTESIAN_POINT ( 'NONE',  ( 802.2119215644370342, -462.0090635724247932, -367.5423716828165084 ) ) ;
#10818=CARTESIAN_POINT ( 'NONE',  ( 797.6776695296629214, -307.5436935675104451, -357.6776695296636603 ) ) ;
#10823=CARTESIAN_POINT ( 'NONE',  ( 758.4439275373578084, -276.5545181178798657, -353.2243759319684386 ) ) ;
#10824=CARTESIAN_POINT ( 'NONE',  ( 756.3353852180819104, -245.9073299311469896, -331.1735550268788302 ) ) ;
#10826=CARTESIAN_POINT ( 'NONE',  ( 792.1044303154645831, -108.4527844766019911, -317.8323909638837677 ) ) ;
#10830=CARTESIAN_POINT ( 'NONE',  ( 799.9999999999993179, -462.9681489794448339, -309.9999999999998863 ) ) ;
#10831=CARTESIAN_POINT ( 'NONE',  ( 812.3518521366052028, -49.09997266333511590, -326.5853460496235243 ) ) ;
#10838=CARTESIAN_POINT ( 'NONE',  ( 801.5560724626406000, -0.5545181178807169209, -326.7756240680316182 ) ) ;
#10839=CARTESIAN_POINT ( 'NONE',  ( 744.7301800767020268, -100.8164208402383935, -337.4774526936615189 ) ) ;
#10841=CARTESIAN_POINT ( 'NONE',  ( 803.6646147819161570, -449.9073299311463643, -348.8264449731210561 ) ) ;
#10843=CARTESIAN_POINT ( 'NONE',  ( 812.7932403749906598, -231.1800572038743553, -327.7687537140311633 ) ) ;
#10850=CARTESIAN_POINT ( 'NONE',  ( 745.1769319972822814, -305.8055962898684470, -346.2694204179732083 ) ) ;
#10853=CARTESIAN_POINT ( 'NONE',  ( 815.2698199232961542, -304.8164208402376403, -342.5225473063383106 ) ) ;
#10854=CARTESIAN_POINT ( 'NONE',  ( 799.9999999999993179, 205.0000000000000568, -339.9999999999999432 ) ) ;
#10857=CARTESIAN_POINT ( 'NONE',  ( 781.8018195045266339, -382.2709662947828519, -365.1927285166406705 ) ) ;
#10860=CARTESIAN_POINT ( 'NONE',  ( 762.1405469898971887, -193.5436935675108714, -357.8594530101015607 ) ) ;
#10861=CARTESIAN_POINT ( 'NONE',  ( 786.2056067578752163, -83.80559628986920018, -374.4686193811670023 ) ) ;
#10867=CARTESIAN_POINT ( 'NONE',  ( 763.2154366446407039, -213.6237781080506011, -321.4292242960311228 ) ) ;
#10869=CARTESIAN_POINT ( 'NONE',  ( 764.3348316497523456, -22.71468719896029853, -308.6759233522265617 ) ) ;
#10871=CARTESIAN_POINT ( 'NONE',  ( 808.6629988358042738, -452.9681489794447771, -336.2505073875255448 ) ) ;
#10875=CARTESIAN_POINT ( 'NONE',  ( 791.0478386215596629, -357.8272453906068904, -306.7653713866226326 ) ) ;
#10878=CARTESIAN_POINT ( 'NONE',  ( 763.0428371773158460, -155.4636090269711417, -358.7617431975195359 ) ) ;
#10879=CARTESIAN_POINT ( 'NONE',  ( 754.8072714833581358, -148.8164208402382656, -338.1981804954720587 ) ) ;
#10880=CARTESIAN_POINT ( 'NONE',  ( 759.9864689768902508, -338.0891481129649492, -354.9819416627836404 ) ) ;
#10892=CARTESIAN_POINT ( 'NONE',  ( 760.0363995740630116, -370.9181544815159555, -368.7758568127991907 ) ) ;
#10893=CARTESIAN_POINT ( 'NONE',  ( 805.0032342141413437, 10.45630643248851044, -314.9967657858572352 ) ) ;
#10896=CARTESIAN_POINT ( 'NONE',  ( 759.9864689768902508, -362.0891481129648923, -354.9819416627836404 ) ) ;
#10899=CARTESIAN_POINT ( 'NONE',  ( 790.0220218866281812, -223.0999726633346256, -363.2186876482849129 ) ) ;
#10901=ADVANCED_FACE ( 'NONE', ( #36552 ), #19220, .T. ) ;
#10905=CARTESIAN_POINT ( 'NONE',  ( 801.1904061080338124, -428.0891481129645513, -368.3070685750236066 ) ) ;
#10910=CARTESIAN_POINT ( 'NONE',  ( 811.0346526505616112, -62.63460265842031305, -323.0537975583477532 ) ) ;
#10911=CARTESIAN_POINT ( 'NONE',  ( 792.1044303154645831, -276.4527844766013800, -317.8323909638837677 ) ) ;
#10915=CARTESIAN_POINT ( 'NONE',  ( 805.6418435158337843, -77.46360902697138329, -363.8556311672236916 ) ) ;
#10916=CARTESIAN_POINT ( 'NONE',  ( 805.1016975059191054, -78.89650538077832209, -343.0745993439771837 ) ) ;
#10921=CARTESIAN_POINT ( 'NONE',  ( 801.3366627262608972, -104.5328690171418913, -353.0897708529566899 ) ) ;
#10923=CARTESIAN_POINT ( 'NONE',  ( 803.4237431249931660, -87.18005720387481006, -331.2633955100225194 ) ) ;
#10924=CARTESIAN_POINT ( 'NONE',  ( 786.6156483768007774, -385.4419599262319593, -315.5913626894246136 ) ) ;
#10928=CARTESIAN_POINT ( 'NONE',  ( 813.2346286133761168, -413.2601417444136018, -328.9521613784389160 ) ) ;
#10933=CARTESIAN_POINT ( 'NONE',  ( 787.4397851343537695, -261.7255117493288026, -374.2001403089903988 ) ) ;
#10937=CARTESIAN_POINT ( 'NONE',  ( 800.2193346964446619, -258.9982390220561115, -355.1360043628816925 ) ) ;
#10939=CARTESIAN_POINT ( 'NONE',  ( 774.6312213355099630, -359.3618753856920875, -364.6798772138717482 ) ) ;
#10940=CARTESIAN_POINT ( 'NONE',  ( 759.7806653035534055, -6.998239022056885972, -324.8639956371180801 ) ) ;
#10947=CARTESIAN_POINT ( 'NONE',  ( 764.8639956371174549, -32.08914811296588709, -319.7806653035542013 ) ) ;
#10951=CARTESIAN_POINT ( 'NONE',  ( 760.0363995740630116, -274.9181544815161828, -368.7758568127991907 ) ) ;
#10955=CARTESIAN_POINT ( 'NONE',  ( 765.0180583372156207, -264.9982390220561115, -360.0135310231089534 ) ) ;
#10957=CARTESIAN_POINT ( 'NONE',  ( 755.5913626894240451, -133.6454272087893571, -346.6156483768012890 ) ) ;
#10961=CARTESIAN_POINT ( 'NONE',  ( 807.5423716828161105, 14.92167643740321381, -362.2119215644372048 ) ) ;
#10962=CARTESIAN_POINT ( 'NONE',  ( 745.7998596910086917, -317.3618753856922581, -332.5602148656461168 ) ) ;
#10966=CARTESIAN_POINT ( 'NONE',  ( 745.1769319972822814, -185.8055962898689302, -346.2694204179732083 ) ) ;
#10968=CARTESIAN_POINT ( 'NONE',  ( 796.7737145352015204, -452.6346026584191691, -370.7187646348536987 ) ) ;
#10973=CARTESIAN_POINT ( 'NONE',  ( 758.6633372737375112, 3.467130982857797417, -326.9102291470432533 ) ) ;
#10978=ORIENTED_EDGE ( 'NONE', *, *, #1528, .F. ) ;
#10979=CARTESIAN_POINT ( 'NONE',  ( 800.0135310231082713, -38.08914811296587999, -325.0180583372163028 ) ) ;
#10980=CARTESIAN_POINT ( 'NONE',  ( 758.6633372737375112, -284.5328690171412518, -326.9102291470432533 ) ) ;
#10982=CARTESIAN_POINT ( 'NONE',  ( 749.8865473780648472, -308.5328690171412518, -322.1177392798429082 ) ) ;
#10988=CARTESIAN_POINT ( 'NONE',  ( 805.1016975059191054, -78.89650538077832209, -343.0745993439771837 ) ) ;
#10989=CARTESIAN_POINT ( 'NONE',  ( 802.1676090361156639, -158.6346026584199933, -327.8955696845344505 ) ) ;
#10990=CARTESIAN_POINT ( 'NONE',  ( 754.8072714833581358, -220.8164208402379529, -338.1981804954720587 ) ) ;
#10992=CARTESIAN_POINT ( 'NONE',  ( 808.3070685750230950, -162.9982390220563673, -361.1904061080339261 ) ) ;
#10994=CARTESIAN_POINT ( 'NONE',  ( 804.6798772138710092, -135.7255117493291721, -334.6312213355106451 ) ) ;
#10996=CARTESIAN_POINT ( 'NONE',  ( 786.5483106153019435, -391.6454272087885897, -364.1601925771022366 ) ) ;
#11003=CARTESIAN_POINT ( 'NONE',  ( 804.8461984189677878, -386.1908817542432075, -336.9566956441385628 ) ) ;
#11005=CARTESIAN_POINT ( 'NONE',  ( 783.7953271457878373, -152.1908817542438612, -375.1787889125761239 ) ) ;
#11009=CARTESIAN_POINT ( 'NONE',  ( 779.4709603349208464, -288.3510508353231216, -314.7162404726379918 ) ) ;
#11010=CARTESIAN_POINT ( 'NONE',  ( 797.6776695296629214, -451.5436935675099903, -357.6776695296636603 ) ) ;
#11011=CARTESIAN_POINT ( 'NONE',  ( 778.7629533639073998, -200.7363362996982801, -375.0009284576466371 ) ) ;
#11012=CARTESIAN_POINT ( 'NONE',  ( 779.9999999999992042, 166.4563064324884465, -329.9999999999999432 ) ) ;
#11016=CARTESIAN_POINT ( 'NONE',  ( 751.9810565676468741, -194.0891481129654039, -360.9747183278973921 ) ) ;
#11018=CARTESIAN_POINT ( 'NONE',  ( 792.1044303154645831, 11.54721552339760038, -317.8323909638837677 ) ) ;
#11021=CARTESIAN_POINT ( 'NONE',  ( 807.5423716828161105, -81.07832356259649487, -362.2119215644372048 ) ) ;
#11023=CARTESIAN_POINT ( 'NONE',  ( 808.3070685750230950, -354.9982390220557704, -361.1904061080339261 ) ) ;
#11025=DIRECTION ( 'NONE',  ( 0.7014439490181308967, -0.1263042864341425708, 0.7014439490181749726 ) ) ;
#11028=CARTESIAN_POINT ( 'NONE',  ( 798.0661480581538854, -410.5328690171408539, -309.5768839229118043 ) ) ;
#11029=CARTESIAN_POINT ( 'NONE',  ( 808.3070685750230950, -426.9982390220554862, -361.1904061080339261 ) ) ;
#11033=CARTESIAN_POINT ( 'NONE',  ( 781.2497674668890113, -180.3510508353234343, -375.3608509340180603 ) ) ;
#11039=CARTESIAN_POINT ( 'NONE',  ( 767.6429770376289525, -33.18005720387498769, -306.8695393053162093 ) ) ;
#11043=CARTESIAN_POINT ( 'NONE',  ( 752.7379699480933368, -444.0090635724249069, -361.9858362298580232 ) ) ;
#11048=CARTESIAN_POINT ( 'NONE',  ( 755.0636971347428243, -292.2709662947831930, -341.7834795799807353 ) ) ;
#11052=CARTESIAN_POINT ( 'NONE',  ( 755.1538015810308480, -278.1908817542434917, -343.0433043558613804 ) ) ;
#11053=CARTESIAN_POINT ( 'NONE',  ( 800.0135310231082713, -302.0891481129650629, -325.0180583372163028 ) ) ;
#11055=CARTESIAN_POINT ( 'NONE',  ( 785.3687786644884454, -131.3618753856928834, -315.3201227861279676 ) ) ;
#11057=DIRECTION ( 'NONE',  ( -0.000000000000000000, 1.000000000000000000, -0.000000000000000000 ) ) ;
#11059=CARTESIAN_POINT ( 'NONE',  ( 812.3518521366052028, -73.09997266333502353, -326.5853460496235243 ) ) ;
#11065=CARTESIAN_POINT ( 'NONE',  ( 754.7162404726377645, -38.73633629969877035, -339.4709603349214717 ) ) ;
#11066=CARTESIAN_POINT ( 'NONE',  ( 814.9108240113580450, -112.2709662947838325, -337.5031285880265273 ) ) ;
#11070=CARTESIAN_POINT ( 'NONE',  ( 810.7187646348534145, -234.4527844766016358, -356.7737145352016341 ) ) ;
#11072=CARTESIAN_POINT ( 'NONE',  ( 799.9999999999993179, -512.9681489794448908, -309.9999999999998863 ) ) ;
#11073=CARTESIAN_POINT ( 'NONE',  ( 746.7653713866222915, -305.2601417444139429, -351.0478386215610271 ) ) ;
#11075=CARTESIAN_POINT ( 'NONE',  ( 744.7301800767019131, -316.8164208402377540, -337.4774526936615757 ) ) ;
#11079=CARTESIAN_POINT ( 'NONE',  ( 785.3141322388236176, -381.7255117493284615, -364.4286716492789537 ) ) ;
#11081=CARTESIAN_POINT ( 'NONE',  ( 749.8865473780648472, -68.53286901714197654, -322.1177392798429082 ) ) ;
#11085=CARTESIAN_POINT ( 'NONE',  ( 780.5290396650775619, -204.3510508353233774, -365.2837595273619513 ) ) ;
#11087=EDGE_CURVE ( 'NONE', #3816, #40052, #1944, .T. ) ;
#11088=CARTESIAN_POINT ( 'NONE',  ( 783.7566961878529810, -24.89650538077847486, -305.1792804349288417 ) ) ;
#11090=CARTESIAN_POINT ( 'NONE',  ( 803.8904222555790966, -452.9681489794450044, -350.1048529224749473 ) ) ;
#11094=CARTESIAN_POINT ( 'NONE',  ( 810.4231160770870019, -336.5545181178796952, -321.9338519418446936 ) ) ;
#11095=ADVANCED_FACE ( 'NONE', ( #12980 ), #38782, .F. ) ;
#11098=CARTESIAN_POINT ( 'NONE',  ( 804.6971507214547046, -171.2817908451529263, -344.0799538623459739 ) ) ;
#11099=CARTESIAN_POINT ( 'NONE',  ( 797.6776695296629214, -163.5436935675109567, -357.6776695296636603 ) ) ;
#11100=CARTESIAN_POINT ( 'NONE',  ( 754.8072714833583632, -364.8164208402375266, -338.1981804954721156 ) ) ;
#11102=CARTESIAN_POINT ( 'NONE',  ( 766.7756240680305382, 9.467130982857780097, -361.5560724626415663 ) ) ;
#11109=CARTESIAN_POINT ( 'NONE',  ( 773.7305795820266212, -417.2817908451522158, -374.8230680027170365 ) ) ;
#11110=CARTESIAN_POINT ( 'NONE',  ( 748.9653473494365699, -2.634602658420536425, -356.9462024416520762 ) ) ;
#11113=CARTESIAN_POINT ( 'NONE',  ( 764.8639956371174549, -368.0891481129647786, -319.7806653035542013 ) ) ;
#11117=CARTESIAN_POINT ( 'NONE',  ( 786.5483106153019435, -223.6454272087891013, -364.1601925771022366 ) ) ;
#11121=CARTESIAN_POINT ( 'NONE',  ( 811.0346526505617248, -446.6346026584191122, -323.0537975583478101 ) ) ;
#11126=CARTESIAN_POINT ( 'NONE',  ( 796.7737145352015204, -44.63460265842040542, -370.7187646348536987 ) ) ;
#11127=CARTESIAN_POINT ( 'NONE',  ( 759.7806653035534055, -294.9982390220560546, -324.8639956371180801 ) ) ;
#11128=CARTESIAN_POINT ( 'NONE',  ( 787.4999999999992042, -512.9681489794448908, -329.9999999999999432 ) ) ;
#11131=CARTESIAN_POINT ( 'NONE',  ( 795.8262568251477660, -70.37269993606230400, -308.3538107759623585 ) ) ;
#11132=CARTESIAN_POINT ( 'NONE',  ( 758.6633372737375112, -92.53286901714190549, -326.9102291470432533 ) ) ;
#11136=CARTESIAN_POINT ( 'NONE',  ( 781.8018195045266339, 1.729033705215812011, -365.1927285166406705 ) ) ;
#11137=CARTESIAN_POINT ( 'NONE',  ( 805.0264073115434940, -102.3510508353236901, -339.4763451958999099 ) ) ;
#11139=CARTESIAN_POINT ( 'NONE',  ( 774.6312213355099630, -95.36187538569294020, -364.6798772138717482 ) ) ;
#11141=CARTESIAN_POINT ( 'NONE',  ( 763.2154366446407039, -405.6237781080500326, -321.4292242960311228 ) ) ;
#11144=CARTESIAN_POINT ( 'NONE',  ( 744.9990715423526808, -402.3510508353228374, -341.2370466360926002 ) ) ;
#11148=VERTEX_POINT ( 'NONE', #32060 ) ;
#11151=CARTESIAN_POINT ( 'NONE',  ( 748.9653473494363425, -242.6346026584197659, -356.9462024416521331 ) ) ;
#11155=CARTESIAN_POINT ( 'NONE',  ( 775.8780910478218402, -81.28179084515319630, -364.9511171171680530 ) ) ;
#11157=CARTESIAN_POINT ( 'NONE',  ( 803.4237431249931660, -255.1800572038742700, -331.2633955100225194 ) ) ;
#11159=CARTESIAN_POINT ( 'NONE',  ( 788.7366044899766848, -347.9073299311467053, -316.5762568750059813 ) ) ;
#11160=CARTESIAN_POINT ( 'NONE',  ( 781.7834795799800531, -58.81642084023854267, -315.0636971347436202 ) ) ;
#11165=CARTESIAN_POINT ( 'NONE',  ( 803.4237431249931660, -15.18005720387504631, -331.2633955100225194 ) ) ;
#11166=CYLINDRICAL_SURFACE ( 'NONE', #38801, 30.00000000000002842 ) ;
#11169=CARTESIAN_POINT ( 'NONE',  ( 778.7629533639073998, -272.7363362996981095, -375.0009284576466371 ) ) ;
#11173=CARTESIAN_POINT ( 'NONE',  ( 758.0580252608178853, -246.4527844766016074, -328.0187753319985404 ) ) ;
#11176=CARTESIAN_POINT ( 'NONE',  ( 783.0745993439762742, -104.1908817542440175, -365.1016975059196739 ) ) ;
#11180=CARTESIAN_POINT ( 'NONE',  ( 787.4397851343537695, -309.7255117493287457, -374.2001403089903988 ) ) ;
#11184=CARTESIAN_POINT ( 'NONE',  ( 768.8385539511368734, -191.2601417444143976, -306.4236121716840557 ) ) ;
#11186=CARTESIAN_POINT ( 'NONE',  ( 796.9462024416508257, -444.4527844766009821, -308.9653473494370246 ) ) ;
#11191=CARTESIAN_POINT ( 'NONE',  ( 766.7756240680305382, 9.467130982857780097, -361.5560724626415663 ) ) ;
#11194=DIRECTION ( 'NONE',  ( -1.000000000000000000, -0.000000000000000000, 0.000000000000000000 ) ) ;
#11198=EDGE_CURVE ( 'NONE', #36235, #16032, #28514, .T. ) ;
#11199=CARTESIAN_POINT ( 'NONE',  ( 763.2154366446407039, -285.6237781080502600, -321.4292242960311228 ) ) ;
#11202=CARTESIAN_POINT ( 'NONE',  ( 744.9990715423526808, -306.3510508353230648, -341.2370466360926002 ) ) ;
#11207=CARTESIAN_POINT ( 'NONE',  ( 761.2382568024794409, -63.62377810805107714, -356.9571628226838129 ) ) ;
#11208=CARTESIAN_POINT ( 'NONE',  ( 801.9419747391806368, -162.4527844766018632, -351.9812246680014027 ) ) ;
#11211=CARTESIAN_POINT ( 'NONE',  ( 811.0346526505616112, -134.6346026584201070, -323.0537975583477532 ) ) ;
#11215=CARTESIAN_POINT ( 'NONE',  ( 788.7366044899766848, -155.9073299311473306, -316.5762568750059813 ) ) ;
#11217=CARTESIAN_POINT ( 'NONE',  ( 776.9254006560222479, -380.1908817542431507, -314.8983024940802125 ) ) ;
#11224=CARTESIAN_POINT ( 'NONE',  ( 804.4086373105744769, -385.6454272087888171, -333.3843516231986541 ) ) ;
#11226=CARTESIAN_POINT ( 'NONE',  ( 797.8822607201568644, -174.5545181178801784, -370.1134526219340160 ) ) ;
#11229=CARTESIAN_POINT ( 'NONE',  ( 799.9999999999993179, 205.0000000000000568, -339.9999999999999432 ) ) ;
#11230=CARTESIAN_POINT ( 'NONE',  ( 801.3366627262608972, -344.5328690171410813, -353.0897708529566899 ) ) ;
#11231=CARTESIAN_POINT ( 'NONE',  ( 778.1981804954714335, -442.2709662947826814, -314.8072714833589885 ) ) ;
#11232=CARTESIAN_POINT ( 'NONE',  ( 805.6418435158337843, -197.4636090269709996, -363.8556311672236916 ) ) ;
#11237=CARTESIAN_POINT ( 'NONE',  ( 745.7998596910086917, -221.3618753856925707, -332.5602148656461168 ) ) ;
#11239=CARTESIAN_POINT ( 'NONE',  ( 785.3141322388236176, 2.274488250670355871, -364.4286716492789537 ) ) ;
#11241=CARTESIAN_POINT ( 'NONE',  ( 811.6461892240364477, -100.7146871989600356, -324.1737431748509835 ) ) ;
#11243=CARTESIAN_POINT ( 'NONE',  ( 777.5031285880264704, -334.8164208402376403, -374.9108240113588408 ) ) ;
#11249=CARTESIAN_POINT ( 'NONE',  ( 761.9338519418445230, -398.5328690171409107, -370.4231160770881957 ) ) ;
#11250=CARTESIAN_POINT ( 'NONE',  ( 805.0032342141412300, -421.5436935675101040, -314.9967657858571783 ) ) ;
#11254=CARTESIAN_POINT ( 'NONE',  ( 790.8726784830453198, -178.7146871989598083, -362.5472867521010585 ) ) ;
#11256=CARTESIAN_POINT ( 'NONE',  ( 776.2433038121456548, -204.8965053807779100, -374.8207195650711014 ) ) ;
#11261=CARTESIAN_POINT ( 'NONE',  ( 782.5225473063381969, -46.27096629478404566, -375.2698199232970637 ) ) ;
#11265=CARTESIAN_POINT ( 'NONE',  ( 794.5607502887775127, -462.9631818684622999, -371.8524697363486666 ) ) ;
#11270=CARTESIAN_POINT ( 'NONE',  ( 771.1735550268778070, -297.1800572038740711, -316.3353852180827630 ) ) ;
#11274=CARTESIAN_POINT ( 'NONE',  ( 755.8894580844503253, -303.8272453906071178, -332.3691319403863531 ) ) ;
#11275=CARTESIAN_POINT ( 'NONE',  ( 805.1927285166397041, -304.8164208402376403, -341.8018195045277707 ) ) ;
#11277=CARTESIAN_POINT ( 'NONE',  ( 757.8323909638827445, -122.6346026584201354, -352.1044303154654358 ) ) ;
#11282=CARTESIAN_POINT ( 'NONE',  ( 814.8207195650702488, -74.19088175424410281, -336.2433038121456548 ) ) ;
#11288=CARTESIAN_POINT ( 'NONE',  ( 763.0428371773158460, -59.46360902697142592, -358.7617431975195359 ) ) ;
#11289=CARTESIAN_POINT ( 'NONE',  ( 758.8095938919644823, -104.0891481129656739, -311.6929314249762797 ) ) ;
#11291=FACE_OUTER_BOUND ( 'NONE', #24582, .T. ) ;
#11293=CARTESIAN_POINT ( 'NONE',  ( 767.7687537140311633, -239.9073299311470748, -372.7932403749916830 ) ) ;
#11298=CARTESIAN_POINT ( 'NONE',  ( 815.0009284576459549, -294.3510508353230648, -338.7629533639073429 ) ) ;
#11299=CARTESIAN_POINT ( 'NONE',  ( 796.7737145352015204, -332.6346026584195101, -370.7187646348536987 ) ) ;
#11301=CARTESIAN_POINT ( 'NONE',  ( 801.1904061080336987, -332.0891481129649492, -368.3070685750235498 ) ) ;
#11305=CARTESIAN_POINT ( 'NONE',  ( 762.3223304703356007, -415.5436935675102177, -322.3223304703362828 ) ) ;
#11307=CARTESIAN_POINT ( 'NONE',  ( 759.7806653035534055, -198.9982390220562252, -324.8639956371180801 ) ) ;
#11309=CARTESIAN_POINT ( 'NONE',  ( 764.3348316497523456, -94.71468719896007826, -308.6759233522265617 ) ) ;
#11313=CARTESIAN_POINT ( 'NONE',  ( 783.0433043558608688, -240.8965053807777963, -315.1538015810313027 ) ) ;
#11315=CARTESIAN_POINT ( 'NONE',  ( 795.6651683502461765, -34.71468719896025590, -371.3240766477733814 ) ) ;
#11321=CARTESIAN_POINT ( 'NONE',  ( 788.6739635108323228, -343.6454272087887603, -373.9316612368139090 ) ) ;
#11324=CARTESIAN_POINT ( 'NONE',  ( 786.5483106153019435, -199.6454272087891582, -364.1601925771022366 ) ) ;
#11325=CARTESIAN_POINT ( 'NONE',  ( 800.2193346964447755, -186.9982390220563104, -355.1360043628815788 ) ) ;
#11327=CARTESIAN_POINT ( 'NONE',  ( 759.7806653035535192, -366.9982390220557136, -324.8639956371181370 ) ) ;
#11329=CARTESIAN_POINT ( 'NONE',  ( 803.8651313633788504, 18.73985825558501972, -332.4468031744301015 ) ) ;
#11337=CARTESIAN_POINT ( 'NONE',  ( 745.7194118038753459, -421.6454272087885329, -348.7631598425976449 ) ) ;
#11338=CARTESIAN_POINT ( 'NONE',  ( 812.7932403749906598, 8.819942796124882634, -327.7687537140311633 ) ) ;
#11341=CARTESIAN_POINT ( 'NONE',  ( 804.6798772138708955, -351.7255117493284047, -334.6312213355107019 ) ) ;
#11342=CARTESIAN_POINT ( 'NONE',  ( 774.6858677611749044, 14.27448825067031812, -315.5713283507209894 ) ) ;
#11346=CARTESIAN_POINT ( 'NONE',  ( 772.4468031744293057, -273.8272453906071746, -363.8651313633793620 ) ) ;
#11355=CARTESIAN_POINT ( 'NONE',  ( 788.8264449731200330, -333.1800572038740142, -363.6646147819171233 ) ) ;
#11356=CARTESIAN_POINT ( 'NONE',  ( 791.4716058693660443, -452.9681489794448339, -367.7200696026887954 ) ) ;
#11361=CARTESIAN_POINT ( 'NONE',  ( 810.4231160770870019, -72.55451811788049099, -321.9338519418446936 ) ) ;
#11362=CARTESIAN_POINT ( 'NONE',  ( 787.6308680596127942, -83.26014174441466764, -364.1105419155492768 ) ) ;
#11365=CARTESIAN_POINT ( 'NONE',  ( 759.7806653035534055, -6.998239022056885972, -324.8639956371180801 ) ) ;
#11366=ORIENTED_EDGE ( 'NONE', *, *, #14813, .T. ) ;
#11367=CARTESIAN_POINT ( 'NONE',  ( 771.1735550268778070, -105.1800572038747248, -316.3353852180827630 ) ) ;
#11368=CARTESIAN_POINT ( 'NONE',  ( 789.9200121543843807, -409.9874144716863498, -317.0176451133914384 ) ) ;
#11372=VERTEX_POINT ( 'NONE', #8062 ) ;
#11380=CARTESIAN_POINT ( 'NONE',  ( 758.4439275373578084, -84.55451811788046257, -353.2243759319684386 ) ) ;
#11382=CARTESIAN_POINT ( 'NONE',  ( 756.3353852180820240, -245.9073299311469896, -331.1735550268787733 ) ) ;
#11384=CARTESIAN_POINT ( 'NONE',  ( 762.3223304703356007, -391.5436935675101608, -322.3223304703362828 ) ) ;
#11385=CARTESIAN_POINT ( 'NONE',  ( 754.8072714833581358, -52.81642084023856398, -338.1981804954720587 ) ) ;
#11390=CARTESIAN_POINT ( 'NONE',  ( 803.6646147819161570, -17.90732993114776406, -348.8264449731210561 ) ) ;
#11393=CARTESIAN_POINT ( 'NONE',  ( 797.8822607201568644, -294.5545181178797520, -370.1134526219340160 ) ) ;
#11397=CARTESIAN_POINT ( 'NONE',  ( 762.3223304703356007, -271.5436935675106156, -322.3223304703362828 ) ) ;
#11399=CARTESIAN_POINT ( 'NONE',  ( 766.9102291470427417, -138.5545181178802636, -318.6633372737382501 ) ) ;
#11402=CARTESIAN_POINT ( 'NONE',  ( 781.2497674668890113, -12.35105083532396897, -375.3608509340180603 ) ) ;
#11403=CARTESIAN_POINT ( 'NONE',  ( 782.4968714119720516, -346.8164208402376971, -305.0891759886411023 ) ) ;
#11408=CARTESIAN_POINT ( 'NONE',  ( 759.8311093483677041, -214.1692326535052189, -310.9282345327691814 ) ) ;
#11410=CARTESIAN_POINT ( 'NONE',  ( 759.0252816721024374, -0.9982390220569063999, -368.0189434323527280 ) ) ;
#11417=CARTESIAN_POINT ( 'NONE',  ( 797.8594530101008786, -445.5436935675098766, -322.1405469898980982 ) ) ;
#11424=CARTESIAN_POINT ( 'NONE',  ( 784.0799538623451781, -299.8055962898685038, -364.6971507214555572 ) ) ;
#11426=CARTESIAN_POINT ( 'NONE',  ( 771.2368401574024119, -277.4419599262322436, -374.2805881961240857 ) ) ;
#11434=CARTESIAN_POINT ( 'NONE',  ( 754.8983024940795303, -90.89650538077827946, -336.9254006560228163 ) ) ;
#11436=CARTESIAN_POINT ( 'NONE',  ( 814.9108240113580450, -136.2709662947837330, -337.5031285880265273 ) ) ;
#11439=CARTESIAN_POINT ( 'NONE',  ( 788.8264449731201466, -141.1800572038746395, -363.6646147819170665 ) ) ;
#11441=CARTESIAN_POINT ( 'NONE',  ( 804.6971507214547046, -411.2817908451521589, -344.0799538623459739 ) ) ;
#11446=DIRECTION ( 'NONE',  ( -0.000000000000000000, 1.000000000000000000, -0.000000000000000000 ) ) ;
#11452=CARTESIAN_POINT ( 'NONE',  ( 769.9779781133707957, -403.0999726633339719, -316.7813123517150871 ) ) ;
#11454=CARTESIAN_POINT ( 'NONE',  ( 804.1009440267234822, -215.4636090269709712, -314.0944755984392600 ) ) ;
#11459=CARTESIAN_POINT ( 'NONE',  ( 798.7617431975189675, -315.6237781080503169, -323.0428371773161871 ) ) ;
#11460=DIRECTION ( 'NONE',  ( 0.000000000000000000, 0.000000000000000000, -1.000000000000000000 ) ) ;
#11461=CARTESIAN_POINT ( 'NONE',  ( 814.8207195650702488, -194.1908817542437475, -336.2433038121456548 ) ) ;
#11469=CARTESIAN_POINT ( 'NONE',  ( 745.4481719005789273, -243.7255117493288310, -347.5162901302853697 ) ) ;
#11471=CARTESIAN_POINT ( 'NONE',  ( 792.1044303154645831, -12.45278447660232146, -317.8323909638837677 ) ) ;
#11474=CARTESIAN_POINT ( 'NONE',  ( 815.1787889125755555, -102.8965053807782368, -343.7953271457877804 ) ) ;
#11476=CARTESIAN_POINT ( 'NONE',  ( 782.4968714119720516, -370.8164208402375834, -305.0891759886411023 ) ) ;
#11483=CARTESIAN_POINT ( 'NONE',  ( 766.5853460496234675, -421.9874144716863498, -372.3518521366060554 ) ) ;
#11485=CARTESIAN_POINT ( 'NONE',  ( 762.1177392798416577, 5.445481882119263872, -309.8865473780659272 ) ) ;
#11489=CARTESIAN_POINT ( 'NONE',  ( 754.9735926884551418, -186.3510508353234343, -340.5236548041000333 ) ) ;
#11491=CARTESIAN_POINT ( 'NONE',  ( 783.7566961878529810, -192.8965053807779668, -305.1792804349288417 ) ) ;
#11496=CARTESIAN_POINT ( 'NONE',  ( 755.0636971347428243, -148.2709662947837330, -341.7834795799807353 ) ) ;
#11498=CARTESIAN_POINT ( 'NONE',  ( 782.4968714119720516, -34.81642084023861372, -305.0891759886411023 ) ) ;
#11500=CARTESIAN_POINT ( 'NONE',  ( 814.4686193811664907, -435.2817908451521021, -346.2056067578752732 ) ) ;
#11502=CARTESIAN_POINT ( 'NONE',  ( 804.4086373105744769, -337.6454272087888171, -333.3843516231986541 ) ) ;
#11505=CARTESIAN_POINT ( 'NONE',  ( 804.4286716492782716, -281.3618753856923718, -345.3141322388244703 ) ) ;
#11509=CARTESIAN_POINT ( 'NONE',  ( 786.5483106153019435, -295.6454272087888739, -364.1601925771022366 ) ) ;
#11510=CARTESIAN_POINT ( 'NONE',  ( 792.1044303154645831, -276.4527844766013800, -317.8323909638837677 ) ) ;
#11512=CARTESIAN_POINT ( 'NONE',  ( 759.7806653035534055, -126.9982390220565094, -324.8639956371180801 ) ) ;
#11514=ORIENTED_EDGE ( 'NONE', *, *, #3815, .F. ) ;
#11520=CARTESIAN_POINT ( 'NONE',  ( 788.6739635108323228, -79.64542720878957027, -373.9316612368139090 ) ) ;
#11527=CARTESIAN_POINT ( 'NONE',  ( 772.5602148656447525, -105.7255117493293000, -305.7998596910095443 ) ) ;
#11531=CARTESIAN_POINT ( 'NONE',  ( 813.1304606946830518, -233.9073299311470180, -352.3570229623690580 ) ) ;
#11536=CARTESIAN_POINT ( 'NONE',  ( 744.8212110874229666, -306.8965053807775689, -336.2046728542121627 ) ) ;
#11539=CARTESIAN_POINT ( 'NONE',  ( 751.9810565676468741, -314.0891481129650629, -360.9747183278973921 ) ) ;
#11543=CARTESIAN_POINT ( 'NONE',  ( 805.1927285166397041, -424.8164208402372992, -341.8018195045277707 ) ) ;
#11544=CARTESIAN_POINT ( 'NONE',  ( 781.7834795799800531, -226.8164208402380098, -315.0636971347436202 ) ) ;
#11545=CARTESIAN_POINT ( 'NONE',  ( 773.7943932421234194, -95.80559628986917176, -305.5313806188329409 ) ) ;
#11550=EDGE_LOOP ( 'NONE', ( #28272, #17853, #45584, #72 ) ) ;
#11551=CARTESIAN_POINT ( 'NONE',  ( 784.0799538623451781, -251.8055962898686744, -364.6971507214555572 ) ) ;
#11554=CARTESIAN_POINT ( 'NONE',  ( 758.0141637701419768, -63.07832356259653750, -367.2620300519063790 ) ) ;
#11556=VERTEX_POINT ( 'NONE', #25358 ) ;
#11557=CARTESIAN_POINT ( 'NONE',  ( 793.5525998758768083, -343.0999726633342561, -372.6845335610516941 ) ) ;
#11560=CARTESIAN_POINT ( 'NONE',  ( 755.5913626894240451, -181.6454272087892434, -346.6156483768012890 ) ) ;
#11561=CARTESIAN_POINT ( 'NONE',  ( 771.2633955100217236, -167.9073299311473022, -363.4237431249939618 ) ) ;
#11562=CARTESIAN_POINT ( 'NONE',  ( 778.1981804954715471, -370.2709662947830793, -314.8072714833591021 ) ) ;
#11564=CARTESIAN_POINT ( 'NONE',  ( 801.3366627262608972, 15.46713098285775878, -353.0897708529566899 ) ) ;
#11575=CARTESIAN_POINT ( 'NONE',  ( 750.9282345327678740, -400.9181544815159555, -319.8311093483690115 ) ) ;
#11577=CARTESIAN_POINT ( 'NONE',  ( 749.2812353651451076, -6.452784476602343666, -323.2262854647983090 ) ) ;
#11581=CARTESIAN_POINT ( 'NONE',  ( 778.2165204200184689, -358.8164208402375834, -364.9363028652563230 ) ) ;
#11582=CARTESIAN_POINT ( 'NONE',  ( 788.7366044899766848, 12.09267006885214180, -316.5762568750059813 ) ) ;
#11585=CARTESIAN_POINT ( 'NONE',  ( 766.9102291470427417, -258.5545181178799226, -318.6633372737382501 ) ) ;
#11594=CARTESIAN_POINT ( 'NONE',  ( 803.6646147819161570, -329.9073299311467053, -348.8264449731210561 ) ) ;
#11598=CARTESIAN_POINT ( 'NONE',  ( 788.6739635108323228, -55.64542720878963422, -373.9316612368139090 ) ) ;
#11599=CARTESIAN_POINT ( 'NONE',  ( 770.0799878456142551, -109.9874144716873019, -362.9823548866085616 ) ) ;
#11603=CARTESIAN_POINT ( 'NONE',  ( 755.0636971347428243, -28.27096629478409540, -341.7834795799807353 ) ) ;
#11604=CARTESIAN_POINT ( 'NONE',  ( 787.6308680596127942, -131.2601417444144829, -364.1105419155492768 ) ) ;
#11605=CARTESIAN_POINT ( 'NONE',  ( 757.8323909638827445, -98.63460265842024910, -352.1044303154654358 ) ) ;
#11607=CARTESIAN_POINT ( 'NONE',  ( 759.2295555964440155, -424.1692326535044799, -353.9708237608231229 ) ) ;
#11613=CIRCLE ( 'NONE', #22667, 10.00000000000000888 ) ;
#11619=CARTESIAN_POINT ( 'NONE',  ( 800.9840315886518738, -76.91815448151683654, -354.1144889064786412 ) ) ;
#11621=CARTESIAN_POINT ( 'NONE',  ( 754.8072714833583632, -268.8164208402378677, -338.1981804954721156 ) ) ;
#11623=CARTESIAN_POINT ( 'NONE',  ( 757.8323909638827445, -386.6346026584191691, -352.1044303154654358 ) ) ;
#11624=CARTESIAN_POINT ( 'NONE',  ( 797.8594530101008786, -61.54369356751124087, -322.1405469898980982 ) ) ;
#11628=CARTESIAN_POINT ( 'NONE',  ( 793.5525998758768083, -7.099972663335241130, -372.6845335610516941 ) ) ;
#11631=CARTESIAN_POINT ( 'NONE',  ( 778.7629533639073998, -296.7363362996979390, -375.0009284576466371 ) ) ;
#11635=CARTESIAN_POINT ( 'NONE',  ( 778.1981804954714335, -250.2709662947832783, -314.8072714833589885 ) ) ;
#11637=CARTESIAN_POINT ( 'NONE',  ( 760.7433823573367135, -156.0090635724256742, -355.9930595647440441 ) ) ;
#11641=CARTESIAN_POINT ( 'NONE',  ( 747.2067596250078623, -339.1800572038740142, -352.2312462859687230 ) ) ;
#11646=CARTESIAN_POINT ( 'NONE',  ( 768.8385539511368734, -239.2601417444141987, -306.4236121716840557 ) ) ;
#11648=CARTESIAN_POINT ( 'NONE',  ( 772.5602148656447525, 14.27448825067031812, -305.7998596910095443 ) ) ;
#11654=CARTESIAN_POINT ( 'NONE',  ( 783.0433043558608688, -24.89650538077847486, -315.1538015810313027 ) ) ;
#11660=CARTESIAN_POINT ( 'NONE',  ( 766.7756240680305382, -302.5328690171411949, -361.5560724626415663 ) ) ;
#11662=CARTESIAN_POINT ( 'NONE',  ( 800.1688906516307043, -322.1692326535048210, -369.0717654672308186 ) ) ;
#11667=CARTESIAN_POINT ( 'NONE',  ( 801.3366627262608972, -80.53286901714194812, -353.0897708529566899 ) ) ;
#11671=CARTESIAN_POINT ( 'NONE',  ( 755.2512626584698410, -199.5436935675108430, -315.2512626584710915 ) ) ;
#11673=CARTESIAN_POINT ( 'NONE',  ( 803.4237431249931660, -135.1800572038746679, -331.2633955100225194 ) ) ;
#11676=CARTESIAN_POINT ( 'NONE',  ( 759.0159684113467620, -424.9181544815158986, -325.8855110935213020 ) ) ;
#11686=CARTESIAN_POINT ( 'NONE',  ( 804.6971507214547046, -387.2817908451522726, -344.0799538623459739 ) ) ;
#11688=CARTESIAN_POINT ( 'NONE',  ( 815.3608509340175488, -194.7363362996982517, -341.2497674668889545 ) ) ;
#11692=CARTESIAN_POINT ( 'NONE',  ( 773.3843516231979720, -325.4419599262320162, -364.4086373105754433 ) ) ;
#11694=CARTESIAN_POINT ( 'NONE',  ( 776.2046728542105711, -188.1908817542437760, -304.8212110874238761 ) ) ;
#11696=DIRECTION ( 'NONE',  ( 0.7014439490181308967, -0.1263042864341425708, 0.7014439490181749726 ) ) ;
#11698=CARTESIAN_POINT ( 'NONE',  ( 772.5602148656447525, -225.7255117493289163, -305.7998596910095443 ) ) ;
#11701=CARTESIAN_POINT ( 'NONE',  ( 781.8018195045266339, 1.729033705215812011, -365.1927285166406705 ) ) ;
#11704=CARTESIAN_POINT ( 'NONE',  ( 815.0009284576459549, -126.3510508353236048, -338.7629533639073429 ) ) ;
#11706=CARTESIAN_POINT ( 'NONE',  ( 787.4397851343537695, -357.7255117493285184, -374.2001403089903988 ) ) ;
#11711=CARTESIAN_POINT ( 'NONE',  ( 758.0141637701419768, -399.0783235625955285, -367.2620300519063790 ) ) ;
#11712=CARTESIAN_POINT ( 'NONE',  ( 793.5525998758768083, -7.099972663335241130, -372.6845335610516941 ) ) ;
#11716=CARTESIAN_POINT ( 'NONE',  ( 784.0799538623451781, -203.8055962898688449, -364.6971507214555572 ) ) ;
#11718=CARTESIAN_POINT ( 'NONE',  ( 778.7502325331095108, -240.3510508353232069, -304.6391490659818828 ) ) ;
#11722=ORIENTED_EDGE ( 'NONE', *, *, #34065, .F. ) ;
#11727=CARTESIAN_POINT ( 'NONE',  ( 767.6429770376289525, -57.18005720387489532, -306.8695393053162093 ) ) ;
#11729=CARTESIAN_POINT ( 'NONE',  ( 807.2620300519052989, -456.0090635724247932, -318.0141637701419768 ) ) ;
#11731=CARTESIAN_POINT ( 'NONE',  ( 755.1538015810308480, -326.1908817542433781, -343.0433043558613804 ) ) ;
#11734=CARTESIAN_POINT ( 'NONE',  ( 774.6858677611749044, -297.7255117493286889, -315.5713283507209894 ) ) ;
#11740=CARTESIAN_POINT ( 'NONE',  ( 761.4292242960306112, -281.4636090269706870, -323.2154366446414429 ) ) ;
#11741=CARTESIAN_POINT ( 'NONE',  ( 802.1676090361156639, -278.6346026584196807, -327.8955696845344505 ) ) ;
#11743=CARTESIAN_POINT ( 'NONE',  ( 762.3223304703356007, -151.5436935675109851, -322.3223304703362828 ) ) ;
#11749=CARTESIAN_POINT ( 'NONE',  ( 809.0717654672305343, -100.9181544815167513, -360.1688906516309885 ) ) ;
#11755=CARTESIAN_POINT ( 'NONE',  ( 755.2512626584698410, -127.5436935675110561, -315.2512626584710915 ) ) ;
#11758=CARTESIAN_POINT ( 'NONE',  ( 800.7704444035546203, -436.1692326535044231, -326.0291762391768771 ) ) ;
#11761=CARTESIAN_POINT ( 'NONE',  ( 814.5518280994195948, -255.7255117493287742, -332.4837098697145734 ) ) ;
#11764=CARTESIAN_POINT ( 'NONE',  ( 764.3348316497523456, -310.7146871989593251, -308.6759233522265617 ) ) ;
#11766=CARTESIAN_POINT ( 'NONE',  ( 801.1904061080336987, -356.0891481129647218, -368.3070685750235498 ) ) ;
#11770=CARTESIAN_POINT ( 'NONE',  ( 781.8018195045266339, -406.2709662947829088, -365.1927285166406705 ) ) ;
#11771=CARTESIAN_POINT ( 'NONE',  ( 747.3154664389472828, -115.9874144716872877, -326.4474001241230781 ) ) ;
#11776=EDGE_CURVE ( 'NONE', #34365, #14643, #44502, .T. ) ;
#11778=EDGE_CURVE ( 'NONE', #16020, #37557, #2005, .T. ) ;
#11779=CARTESIAN_POINT ( 'NONE',  ( 805.9055244015594326, -51.62377810805111267, -315.8990559732753240 ) ) ;
#11780=CARTESIAN_POINT ( 'NONE',  ( 791.3800697268461590, -452.9681489794449476, -362.3092612109132915 ) ) ;
#11783=CARTESIAN_POINT ( 'NONE',  ( 764.1737431748507561, -346.3726999360614514, -371.6461892240376415 ) ) ;
#11786=CARTESIAN_POINT ( 'NONE',  ( 802.5472867521000353, -172.3726999360619914, -350.8726784830461156 ) ) ;
#11787=CARTESIAN_POINT ( 'NONE',  ( 778.2165204200184689, -190.8164208402381234, -364.9363028652563230 ) ) ;
#11788=CARTESIAN_POINT ( 'NONE',  ( 755.0636971347428243, -388.2709662947829656, -341.7834795799807353 ) ) ;
#11790=CARTESIAN_POINT ( 'NONE',  ( 797.6776695296629214, -451.5436935675099903, -357.6776695296636603 ) ) ;
#11799=CARTESIAN_POINT ( 'NONE',  ( 746.4236121716829757, -423.8272453906067199, -328.8385539511384650 ) ) ;
#11800=CARTESIAN_POINT ( 'NONE',  ( 777.4774526936600978, -34.27096629478407408, -304.7301800767028226 ) ) ;
#11802=CARTESIAN_POINT ( 'NONE',  ( 757.8323909638827445, -386.6346026584191691, -352.1044303154654358 ) ) ;
#11803=CARTESIAN_POINT ( 'NONE',  ( 805.1927285166399315, 7.183579159761249500, -341.8018195045277707 ) ) ;
#11806=CARTESIAN_POINT ( 'NONE',  ( 759.0159684113467620, -256.9181544815163534, -325.8855110935213020 ) ) ;
#11807=CARTESIAN_POINT ( 'NONE',  ( 787.5162901302840055, -179.3618753856927128, -305.4481719005792684 ) ) ;
#11811=DIRECTION ( 'NONE',  ( 0.000000000000000000, 0.000000000000000000, 1.000000000000000000 ) ) ;
#11815=CARTESIAN_POINT ( 'NONE',  ( 756.3353852180819104, -317.9073299311468190, -331.1735550268788302 ) ) ;
#11818=CARTESIAN_POINT ( 'NONE',  ( 805.6418435158337843, -53.46360902697146855, -363.8556311672236916 ) ) ;
#11819=CARTESIAN_POINT ( 'NONE',  ( 772.3691319403857278, -119.2601417444145397, -315.8894580844506663 ) ) ;
#11822=CARTESIAN_POINT ( 'NONE',  ( 754.8072714833581358, -28.81642084023863148, -338.1981804954720587 ) ) ;
#11823=CARTESIAN_POINT ( 'NONE',  ( 759.2295555964440155, -136.1692326535053894, -353.9708237608231229 ) ) ;
#11824=CARTESIAN_POINT ( 'NONE',  ( 785.3141322388236176, -141.7255117493291721, -364.4286716492789537 ) ) ;
#11825=CARTESIAN_POINT ( 'NONE',  ( 778.7502325331095108, 23.64894916467591912, -304.6391490659818828 ) ) ;
#11837=CARTESIAN_POINT ( 'NONE',  ( 787.5531968255692163, -93.82724539060770041, -316.1348686366205811 ) ) ;
#11839=CARTESIAN_POINT ( 'NONE',  ( 759.9864689768902508, -266.0891481129651197, -354.9819416627836404 ) ) ;
#11841=CARTESIAN_POINT ( 'NONE',  ( 771.1735550268778070, -393.1800572038737300, -316.3353852180827630 ) ) ;
#11842=CARTESIAN_POINT ( 'NONE',  ( 800.2193346964447755, -42.99823902205675807, -355.1360043628815788 ) ) ;
#11846=CARTESIAN_POINT ( 'NONE',  ( 805.6418435158337843, -29.46360902697153250, -363.8556311672236916 ) ) ;
#11849=CARTESIAN_POINT ( 'NONE',  ( 778.7629533639073998, -320.7363362996979390, -375.0009284576466371 ) ) ;
#11852=CARTESIAN_POINT ( 'NONE',  ( 791.9812246680005501, -284.6346026584196807, -361.9419747391813189 ) ) ;
#11854=CARTESIAN_POINT ( 'NONE',  ( 779.4763451958990572, -152.7363362996983938, -365.0264073115438919 ) ) ;
#11857=CARTESIAN_POINT ( 'NONE',  ( 754.9967657858570647, -337.5436935675102745, -365.0032342141425943 ) ) ;
#11858=CARTESIAN_POINT ( 'NONE',  ( 793.3938497862117174, -453.0432664090020580, -372.3358127763068524 ) ) ;
#11861=CARTESIAN_POINT ( 'NONE',  ( 793.4146539503750546, -241.9874144716869182, -307.6481478633938877 ) ) ;
#11863=CARTESIAN_POINT ( 'NONE',  ( 800.9747183278959710, 11.00176097794305541, -311.9810565676471583 ) ) ;
#11868=CARTESIAN_POINT ( 'NONE',  ( 772.3691319403857278, 0.7398582555850804487, -315.8894580844506663 ) ) ;
#11874=CARTESIAN_POINT ( 'NONE',  ( 803.2186876482843445, -343.9874144716865771, -350.0220218866286928 ) ) ;
#11877=CARTESIAN_POINT ( 'NONE',  ( 813.2346286133761168, -317.2601417444139429, -328.9521613784389160 ) ) ;
#11882=CARTESIAN_POINT ( 'NONE',  ( 804.1601925771018387, -79.44195992623286884, -346.5483106153029098 ) ) ;
#11883=ORIENTED_EDGE ( 'NONE', *, *, #35064, .T. ) ;
#11885=CARTESIAN_POINT ( 'NONE',  ( 763.0537975583475827, -168.4527844766018347, -371.0346526505627480 ) ) ;
#11887=CARTESIAN_POINT ( 'NONE',  ( 805.1927285166399315, -160.8164208402382371, -341.8018195045277707 ) ) ;
#11889=CARTESIAN_POINT ( 'NONE',  ( 793.0897708529556667, -438.5545181178793541, -361.3366627262616362 ) ) ;
#11892=CARTESIAN_POINT ( 'NONE',  ( 772.4999999999993179, -462.9681489794447202, -270.0000000000000568 ) ) ;
#11893=DIRECTION ( 'NONE',  ( 0.000000000000000000, -1.000000000000000000, 0.000000000000000000 ) ) ;
#11896=CARTESIAN_POINT ( 'NONE',  ( 759.0159684113467620, -424.9181544815158986, -325.8855110935213020 ) ) ;
#11898=CARTESIAN_POINT ( 'NONE',  ( 788.6739635108323228, -199.6454272087891582, -373.9316612368139090 ) ) ;
#11903=CARTESIAN_POINT ( 'NONE',  ( 772.3691319403857278, -335.2601417444137724, -315.8894580844506663 ) ) ;
#11904=DIRECTION ( 'NONE',  ( 0.000000000000000000, -1.000000000000000000, 0.000000000000000000 ) ) ;
#11905=CARTESIAN_POINT ( 'NONE',  ( 805.6418435158337843, -221.4636090269709428, -363.8556311672236916 ) ) ;
#11909=CARTESIAN_POINT ( 'NONE',  ( 772.4837098697145166, -239.3618753856924855, -374.5518280994205611 ) ) ;
#11912=CARTESIAN_POINT ( 'NONE',  ( 759.9864689768902508, -26.08914811296592262, -354.9819416627836404 ) ) ;
#11914=CARTESIAN_POINT ( 'NONE',  ( 791.1614460488616487, -131.2601417444144829, -373.5763878283158874 ) ) ;
#11916=CARTESIAN_POINT ( 'NONE',  ( 801.1904061080336987, -380.0891481129646650, -368.3070685750235498 ) ) ;
#11921=CARTESIAN_POINT ( 'NONE',  ( 781.8018195045266339, -382.2709662947828519, -365.1927285166406705 ) ) ;
#11922=CARTESIAN_POINT ( 'NONE',  ( 807.2620300519052989, -0.009063572426172561425, -318.0141637701419768 ) ) ;
#11927=APPLICATION_CONTEXT ( 'automotive_design' ) ;
#11928=CARTESIAN_POINT ( 'NONE',  ( 772.3691319403857278, -239.2601417444141987, -315.8894580844506663 ) ) ;
#11932=CARTESIAN_POINT ( 'NONE',  ( 748.3538107759620743, -208.7146871989596946, -355.8262568251490165 ) ) ;
#11935=ORIENTED_EDGE ( 'NONE', *, *, #26956, .F. ) ;
#11937=CARTESIAN_POINT ( 'NONE',  ( 802.1676090361156639, -134.6346026584201070, -327.8955696845344505 ) ) ;
#11939=CARTESIAN_POINT ( 'NONE',  ( 801.1904061080336987, -68.08914811296575920, -368.3070685750235498 ) ) ;
#11940=CARTESIAN_POINT ( 'NONE',  ( 788.8264449731201466, -69.18005720387488111, -363.6646147819170665 ) ) ;
#11942=CARTESIAN_POINT ( 'NONE',  ( 776.9254006560222479, 3.809118245755632959, -314.8983024940802125 ) ) ;
#11944=CARTESIAN_POINT ( 'NONE',  ( 761.4292242960306112, -305.4636090269706870, -323.2154366446414429 ) ) ;
#11948=CARTESIAN_POINT ( 'NONE',  ( 755.3201227861273992, -315.7255117493286320, -345.3687786644892981 ) ) ;
#11952=CARTESIAN_POINT ( 'NONE',  ( 763.8424801807145741, -330.0090635724251342, -320.5453621957614700 ) ) ;
#11953=CARTESIAN_POINT ( 'NONE',  ( 791.9812246680005501, -284.6346026584196807, -361.9419747391813189 ) ) ;
#11955=CARTESIAN_POINT ( 'NONE',  ( 755.3201227861273992, -147.7255117493291152, -345.3687786644892981 ) ) ;
#11960=CARTESIAN_POINT ( 'NONE',  ( 797.8822607201568644, -78.55451811788046257, -370.1134526219340160 ) ) ;
#11967=CARTESIAN_POINT ( 'NONE',  ( 745.4481719005789273, -123.7255117493292289, -347.5162901302853697 ) ) ;
#11971=CARTESIAN_POINT ( 'NONE',  ( 758.8095938919642549, -272.0891481129651197, -311.6929314249763365 ) ) ;
#11976=CARTESIAN_POINT ( 'NONE',  ( 764.3348316497523456, -358.7146871989592114, -308.6759233522265617 ) ) ;
#11977=CARTESIAN_POINT ( 'NONE',  ( 767.7687537140311633, -95.90732993114751537, -372.7932403749916830 ) ) ;
#11979=CARTESIAN_POINT ( 'NONE',  ( 767.7687537140311633, -359.9073299311467053, -372.7932403749916830 ) ) ;
#11984=CARTESIAN_POINT ( 'NONE',  ( 767.8955696845333705, -408.4527844766009252, -362.1676090361162323 ) ) ;
#11986=CARTESIAN_POINT ( 'NONE',  ( 771.2633955100217236, -215.9073299311471317, -363.4237431249939618 ) ) ;
#11988=CARTESIAN_POINT ( 'NONE',  ( 744.9990715423526808, -114.3510508353236617, -341.2370466360926002 ) ) ;
#11993=CARTESIAN_POINT ( 'NONE',  ( 804.9511171171677688, -245.8055962898686460, -335.8780910478229202 ) ) ;
#11995=CARTESIAN_POINT ( 'NONE',  ( 751.2241431872005251, -424.1692326535044799, -359.9636004259367610 ) ) ;
#11996=CARTESIAN_POINT ( 'NONE',  ( 744.8212110874229666, -66.89650538077835051, -336.2046728542121627 ) ) ;
#12001=CARTESIAN_POINT ( 'NONE',  ( 778.7629533639073998, -368.7363362996977685, -375.0009284576466371 ) ) ;
#12006=CARTESIAN_POINT ( 'NONE',  ( 796.1575198192839480, -174.0090635724256742, -359.4546378042384163 ) ) ;
#12007=CARTESIAN_POINT ( 'NONE',  ( 778.1981804954714335, -178.2709662947835625, -314.8072714833589885 ) ) ;
#12008=CARTESIAN_POINT ( 'NONE',  ( 797.6776695296629214, -379.5436935675102745, -357.6776695296636603 ) ) ;
#12011=CARTESIAN_POINT ( 'NONE',  ( 763.2154366446407039, 26.37622189194863509, -321.4292242960311228 ) ) ;
#12015=LINE ( 'NONE', #36941, #27776 ) ;
#12020=CARTESIAN_POINT ( 'NONE',  ( 795.8262568251477660, -406.3726999360612808, -308.3538107759623585 ) ) ;
#12022=CARTESIAN_POINT ( 'NONE',  ( 755.2512626584698410, -31.54369356751135456, -315.2512626584710915 ) ) ;
#12024=CARTESIAN_POINT ( 'NONE',  ( 765.0180583372156207, -408.9982390220556567, -360.0135310231089534 ) ) ;
#12025=CARTESIAN_POINT ( 'NONE',  ( 804.6798772138710092, -15.72551174932958951, -334.6312213355106451 ) ) ;
#12029=CARTESIAN_POINT ( 'NONE',  ( 755.1538015810308480, -254.1908817542435770, -343.0433043558613804 ) ) ;
#12030=CARTESIAN_POINT ( 'NONE',  ( 800.9747183278959710, -156.9982390220564241, -311.9810565676471583 ) ) ;
#12031=EDGE_CURVE ( 'NONE', #45689, #41099, #24850, .T. ) ;
#12040=CARTESIAN_POINT ( 'NONE',  ( 771.1735550268778070, -321.1800572038740142, -316.3353852180827630 ) ) ;
#12042=CARTESIAN_POINT ( 'NONE',  ( 745.1792804349281596, -110.1908817542440033, -343.7566961878542884 ) ) ;
#12043=CARTESIAN_POINT ( 'NONE',  ( 761.2382568024794409, -111.6237781080509279, -356.9571628226838129 ) ) ;
#12046=CARTESIAN_POINT ( 'NONE',  ( 756.5762568750052424, -27.18005720387500901, -348.7366044899774238 ) ) ;
#12047=CARTESIAN_POINT ( 'NONE',  ( 770.0799878456142551, -133.9874144716872024, -362.9823548866085616 ) ) ;
#12048=CARTESIAN_POINT ( 'NONE',  ( 756.5762568750052424, -123.1800572038747106, -348.7366044899774238 ) ) ;
#12050=CARTESIAN_POINT ( 'NONE',  ( 793.2243759319678702, -434.5328690171407970, -318.4439275373583200 ) ) ;
#12063=CARTESIAN_POINT ( 'NONE',  ( 755.8894580844503253, -63.82724539060779279, -332.3691319403863531 ) ) ;
#12064=CARTESIAN_POINT ( 'NONE',  ( 792.1044303154646968, -276.4527844766014368, -317.8323909638837677 ) ) ;
#12066=CARTESIAN_POINT ( 'NONE',  ( 797.6776695296629214, -403.5436935675101608, -357.6776695296636603 ) ) ;
#12067=CARTESIAN_POINT ( 'NONE',  ( 800.0135310231082713, -38.08914811296587999, -325.0180583372163028 ) ) ;
#12071=CARTESIAN_POINT ( 'NONE',  ( 759.9999999999992042, 166.4563064324884465, -360.0000000000000000 ) ) ;
#12072=CARTESIAN_POINT ( 'NONE',  ( 807.2620300519052989, -24.00906357242609346, -318.0141637701419768 ) ) ;
#12075=CARTESIAN_POINT ( 'NONE',  ( 795.8262568251477660, -310.3726999360616219, -308.3538107759623585 ) ) ;
#12078=CARTESIAN_POINT ( 'NONE',  ( 805.1927285166397041, -280.8164208402378677, -341.8018195045277707 ) ) ;
#12081=CARTESIAN_POINT ( 'NONE',  ( 773.4516893846965786, -163.6454272087893003, -315.8398074228977066 ) ) ;
#12085=CARTESIAN_POINT ( 'NONE',  ( 815.2698199232962679, -352.8164208402375266, -342.5225473063383674 ) ) ;
#12091=CARTESIAN_POINT ( 'NONE',  ( 749.8865473780648472, -428.5328690171409107, -322.1177392798429082 ) ) ;
#12096=CARTESIAN_POINT ( 'NONE',  ( 804.1601925771018387, -7.441959926233078448, -346.5483106153029098 ) ) ;
#12103=CARTESIAN_POINT ( 'NONE',  ( 787.6308680596127942, -323.2601417444138860, -364.1105419155492768 ) ) ;
#12106=CARTESIAN_POINT ( 'NONE',  ( 811.6461892240364477, -316.7146871989593819, -324.1737431748509835 ) ) ;
#12112=CARTESIAN_POINT ( 'NONE',  ( 808.0189434323515343, -182.0891481129654323, -319.0252816721025511 ) ) ;
#12115=CARTESIAN_POINT ( 'NONE',  ( 785.3141322388236176, -165.7255117493291152, -364.4286716492789537 ) ) ;
#12116=AXIS2_PLACEMENT_3D ( 'NONE', #11858, #4482, #25931 ) ;
#12118=CARTESIAN_POINT ( 'NONE',  ( 804.6971507214547046, -435.2817908451521021, -344.0799538623459739 ) ) ;
#12124=CARTESIAN_POINT ( 'NONE',  ( 766.0291762391763086, -418.9181544815157849, -360.7704444035551319 ) ) ;
#12126=CARTESIAN_POINT ( 'NONE',  ( 812.3518521366052028, -193.0999726633346256, -326.5853460496235243 ) ) ;
#12130=CARTESIAN_POINT ( 'NONE',  ( 757.8323909638827445, -170.6346026584199649, -352.1044303154654358 ) ) ;
#12131=CARTESIAN_POINT ( 'NONE',  ( 805.0264073115434940, -342.3510508353228943, -339.4763451958999099 ) ) ;
#12133=CARTESIAN_POINT ( 'NONE',  ( 809.0717654672305343, -220.9181544815164102, -360.1688906516309885 ) ) ;
#12136=CARTESIAN_POINT ( 'NONE',  ( 766.0291762391763086, -34.91815448151697154, -360.7704444035551319 ) ) ;
#12139=CARTESIAN_POINT ( 'NONE',  ( 792.2312462859673587, -227.9073299311471033, -307.2067596250082602 ) ) ;
#12142=CARTESIAN_POINT ( 'NONE',  ( 756.3353852180819104, -5.907329931147798696, -331.1735550268788302 ) ) ;
#12144=CARTESIAN_POINT ( 'NONE',  ( 783.7566961878529810, -120.8965053807781800, -305.1792804349288417 ) ) ;
#12146=CARTESIAN_POINT ( 'NONE',  ( 745.4481719005789273, -363.7255117493284047, -347.5162901302853129 ) ) ;
#12152=CARTESIAN_POINT ( 'NONE',  ( 785.3687786644884454, -395.3618753856918602, -315.3201227861279676 ) ) ;
#12155=CARTESIAN_POINT ( 'NONE',  ( 791.0478386215596629, 2.172754609392001601, -306.7653713866226326 ) ) ;
#12159=CARTESIAN_POINT ( 'NONE',  ( 803.8651313633788504, -221.2601417444142271, -332.4468031744301015 ) ) ;
#12161=CARTESIAN_POINT ( 'NONE',  ( 791.1614460488616487, -227.2601417444141987, -373.5763878283158874 ) ) ;
#12162=CARTESIAN_POINT ( 'NONE',  ( 772.4999999999993179, -462.9681489794447202, -270.0000000000000568 ) ) ;
#12166=CARTESIAN_POINT ( 'NONE',  ( 768.0187753319979720, -152.6346026584200786, -318.0580252608186242 ) ) ;
#12169=CARTESIAN_POINT ( 'NONE',  ( 792.2312462859673587, -83.90732993114754379, -307.2067596250082602 ) ) ;
#12170=AXIS2_PLACEMENT_3D ( 'NONE', #36840, #26442, #22513 ) ;
#12171=CARTESIAN_POINT ( 'NONE',  ( 755.5713283507202505, -77.36187538569302546, -334.6858677611754729 ) ) ;
#12173=CARTESIAN_POINT ( 'NONE',  ( 796.9571628226829034, 0.5363909730283709099, -321.2382568024804641 ) ) ;
#12175=CARTESIAN_POINT ( 'NONE',  ( 787.5531968255692163, -309.8272453906070041, -316.1348686366205811 ) ) ;
#12183=CARTESIAN_POINT ( 'NONE',  ( 776.9254006560222479, -332.1908817542433781, -314.8983024940802125 ) ) ;
#12184=CARTESIAN_POINT ( 'NONE',  ( 768.0187753319979720, -320.6346026584195670, -318.0580252608186242 ) ) ;
#12185=CARTESIAN_POINT ( 'NONE',  ( 795.1360043628807261, -140.0891481129654892, -360.2193346964456282 ) ) ;
#12191=CARTESIAN_POINT ( 'NONE',  ( 807.2620300519052989, -120.0090635724258021, -318.0141637701419768 ) ) ;
#12198=CARTESIAN_POINT ( 'NONE',  ( 747.2067596250078623, -123.1800572038747106, -352.2312462859687230 ) ) ;
#12202=CARTESIAN_POINT ( 'NONE',  ( 782.5225473063381969, -262.2709662947831930, -375.2698199232970637 ) ) ;
#12204=CARTESIAN_POINT ( 'NONE',  ( 792.2312462859673587, -443.9073299311464780, -307.2067596250082602 ) ) ;
#12206=CARTESIAN_POINT ( 'NONE',  ( 793.4146539503750546, -337.9874144716865771, -307.6481478633938877 ) ) ;
#12207=CARTESIAN_POINT ( 'NONE',  ( 745.4481719005789273, -75.72551174932937101, -347.5162901302853129 ) ) ;
#12209=CARTESIAN_POINT ( 'NONE',  ( 746.8695393053150156, -341.9073299311465917, -327.6429770376306010 ) ) ;
#12213=CARTESIAN_POINT ( 'NONE',  ( 771.1735550268778070, -225.1800572038743269, -316.3353852180827630 ) ) ;
#12215=CARTESIAN_POINT ( 'NONE',  ( 745.1769319972822814, -113.8055962898691149, -346.2694204179732083 ) ) ;
#12221=CARTESIAN_POINT ( 'NONE',  ( 780.5290396650775619, -228.3510508353232922, -365.2837595273619513 ) ) ;
#12223=CARTESIAN_POINT ( 'NONE',  ( 815.0009284576459549, -438.3510508353226669, -338.7629533639073429 ) ) ;
#12224=CARTESIAN_POINT ( 'NONE',  ( 754.0944755984390895, -63.62377810805107714, -364.1009440267246760 ) ) ;
#12228=CARTESIAN_POINT ( 'NONE',  ( 745.7194118038753459, -373.6454272087887034, -348.7631598425976449 ) ) ;
#12234=CARTESIAN_POINT ( 'NONE',  ( 757.0176451133909268, -229.0999726633345404, -349.9200121543848354 ) ) ;
#12235=CARTESIAN_POINT ( 'NONE',  ( 802.1676090361156639, -182.6346026584199649, -327.8955696845344505 ) ) ;
#12236=CARTESIAN_POINT ( 'NONE',  ( 795.1360043628808398, -380.0891481129647218, -360.2193346964456282 ) ) ;
#12239=CARTESIAN_POINT ( 'NONE',  ( 785.3141322388236176, -117.7255117493292715, -364.4286716492789537 ) ) ;
#12249=CARTESIAN_POINT ( 'NONE',  ( 814.8207195650702488, -458.1908817542429802, -336.2433038121456548 ) ) ;
#12250=CARTESIAN_POINT ( 'NONE',  ( 754.9967657858570647, -49.54369356751129772, -365.0032342141425943 ) ) ;
#12252=CARTESIAN_POINT ( 'NONE',  ( 755.5713283507202505, -413.3618753856920307, -334.6858677611754729 ) ) ;
#12253=CARTESIAN_POINT ( 'NONE',  ( 767.8955696845334842, -24.45278447660228949, -362.1676090361161755 ) ) ;
#12256=CARTESIAN_POINT ( 'NONE',  ( 769.9779781133707957, -259.0999726633343698, -316.7813123517150871 ) ) ;
#12257=CARTESIAN_POINT ( 'NONE',  ( 808.3070685750230950, -162.9982390220563673, -361.1904061080339261 ) ) ;
#12260=CARTESIAN_POINT ( 'NONE',  ( 795.2725662613897839, 16.45630643248849267, -314.1785221222716586 ) ) ;
#12264=EDGE_CURVE ( 'NONE', #12399, #36235, #38968, .T. ) ;
#12267=CARTESIAN_POINT ( 'NONE',  ( 803.6646147819161570, -305.9073299311467622, -348.8264449731210561 ) ) ;
#12271=CARTESIAN_POINT ( 'NONE',  ( 762.1177392798416577, -90.55451811788041994, -309.8865473780659272 ) ) ;
#12272=CARTESIAN_POINT ( 'NONE',  ( 787.6308680596127942, -131.2601417444144829, -364.1105419155492768 ) ) ;
#12276=CARTESIAN_POINT ( 'NONE',  ( 788.7366044899766848, -35.90732993114770011, -316.5762568750059813 ) ) ;
#12277=CARTESIAN_POINT ( 'NONE',  ( 805.1016975059191054, -126.8965053807781516, -343.0745993439771837 ) ) ;
#12278=CARTESIAN_POINT ( 'NONE',  ( 758.0580252608178853, -126.4527844766019626, -328.0187753319985404 ) ) ;
#12280=CARTESIAN_POINT ( 'NONE',  ( 759.8311093483677041, 25.83076734649409545, -310.9282345327691814 ) ) ;
#12286=CARTESIAN_POINT ( 'NONE',  ( 795.8262568251477660, -262.3726999360617924, -308.3538107759623585 ) ) ;
#12288=EDGE_LOOP ( 'NONE', ( #4769, #3761, #2153, #27457 ) ) ;
#12289=VECTOR ( 'NONE', #3324, 1000.000000000000000 ) ;
#12295=CARTESIAN_POINT ( 'NONE',  ( 776.9254006560222479, -116.1908817542440033, -314.8983024940802125 ) ) ;
#12297=CARTESIAN_POINT ( 'NONE',  ( 764.8639956371174549, -296.0891481129650629, -319.7806653035542581 ) ) ;
#12299=CARTESIAN_POINT ( 'NONE',  ( 794.9819416627830151, -420.9982390220555999, -319.9864689768909898 ) ) ;
#12300=CARTESIAN_POINT ( 'NONE',  ( 755.0636971347428243, -100.2709662947838609, -341.7834795799807353 ) ) ;
#12307=CARTESIAN_POINT ( 'NONE',  ( 745.7194118038753459, -13.64542720878976390, -348.7631598425976449 ) ) ;
#12310=CARTESIAN_POINT ( 'NONE',  ( 815.3608509340175488, -314.7363362996979959, -341.2497674668889545 ) ) ;
#12313=CARTESIAN_POINT ( 'NONE',  ( 804.6798772138708955, -279.7255117493288026, -334.6312213355107019 ) ) ;
#12315=CARTESIAN_POINT ( 'NONE',  ( 786.5483106153019435, -151.6454272087892718, -364.1601925771022366 ) ) ;
#12317=CARTESIAN_POINT ( 'NONE',  ( 751.9810565676468741, -362.0891481129648923, -360.9747183278973921 ) ) ;
#12324=CARTESIAN_POINT ( 'NONE',  ( 815.0009284576459549, -438.3510508353226669, -338.7629533639073429 ) ) ;
#12330=CARTESIAN_POINT ( 'NONE',  ( 793.2243759319678702, -26.53286901714210799, -318.4439275373583200 ) ) ;
#12337=CARTESIAN_POINT ( 'NONE',  ( 794.1144889064781864, -346.1692326535047641, -360.9840315886528401 ) ) ;
#12339=CARTESIAN_POINT ( 'NONE',  ( 744.9990715423526808, -330.3510508353229511, -341.2370466360926002 ) ) ;
#12345=CARTESIAN_POINT ( 'NONE',  ( 787.5162901302840055, -179.3618753856927128, -305.4481719005792684 ) ) ;
#12348=CARTESIAN_POINT ( 'NONE',  ( 788.8264449731201466, -189.1800572038744690, -363.6646147819170665 ) ) ;
#12350=CARTESIAN_POINT ( 'NONE',  ( 791.9812246680005501, 3.365397341579444479, -361.9419747391813189 ) ) ;
#12357=CARTESIAN_POINT ( 'NONE',  ( 784.1219089521767955, -429.2817908451521021, -315.0488828828318333 ) ) ;
#12360=CARTESIAN_POINT ( 'NONE',  ( 797.8822607201568644, -198.5545181178800647, -370.1134526219340160 ) ) ;
#12364=CARTESIAN_POINT ( 'NONE',  ( 781.7834795799800531, -178.8164208402381519, -315.0636971347436202 ) ) ;
#12365=CARTESIAN_POINT ( 'NONE',  ( 783.0433043558608688, -360.8965053807773984, -315.1538015810313027 ) ) ;
#12367=CARTESIAN_POINT ( 'NONE',  ( 807.2620300519052989, -216.0090635724255037, -318.0141637701419768 ) ) ;
#12370=CARTESIAN_POINT ( 'NONE',  ( 760.7433823573367135, -36.00906357242605793, -355.9930595647440441 ) ) ;
#12372=CARTESIAN_POINT ( 'NONE',  ( 811.0346526505617248, -230.6346026584197944, -323.0537975583478101 ) ) ;
#12375=CARTESIAN_POINT ( 'NONE',  ( 803.4237431249931660, -39.18005720387496638, -331.2633955100225194 ) ) ;
#12377=CARTESIAN_POINT ( 'NONE',  ( 815.1787889125755555, -126.8965053807781516, -343.7953271457877804 ) ) ;
#12379=CARTESIAN_POINT ( 'NONE',  ( 751.6929314249748586, -390.9982390220557136, -318.8095938919659034 ) ) ;
#12383=CARTESIAN_POINT ( 'NONE',  ( 801.9419747391806368, -402.4527844766010389, -351.9812246680014027 ) ) ;
#12385=CARTESIAN_POINT ( 'NONE',  ( 747.6481478633932056, -13.09997266333522248, -353.4146539503763620 ) ) ;
#12389=CARTESIAN_POINT ( 'NONE',  ( 800.7704444035546203, -220.1692326535051052, -326.0291762391768771 ) ) ;
#12391=CARTESIAN_POINT ( 'NONE',  ( 745.1769319972822814, -233.8055962898687028, -346.2694204179732083 ) ) ;
#12397=CARTESIAN_POINT ( 'NONE',  ( 814.2001403089898304, -89.36187538569299704, -347.4397851343538264 ) ) ;
#12398=CARTESIAN_POINT ( 'NONE',  ( 762.3223304703356007, -55.54369356751127640, -322.3223304703362828 ) ) ;
#12399=VERTEX_POINT ( 'NONE', #7539 ) ;
#12400=CARTESIAN_POINT ( 'NONE',  ( 804.8461984189677878, -2.190881754244347945, -336.9566956441385628 ) ) ;
#12402=CARTESIAN_POINT ( 'NONE',  ( 790.9844846989617508, -334.3726999360615082, -317.2208543904092721 ) ) ;
#12409=CARTESIAN_POINT ( 'NONE',  ( 801.5560724626406000, -312.5545181178797520, -326.7756240680316182 ) ) ;
#12410=CARTESIAN_POINT ( 'NONE',  ( 765.0180583372156207, -312.9982390220559409, -360.0135310231089534 ) ) ;
#12411=CARTESIAN_POINT ( 'NONE',  ( 785.3687786644884454, -155.3618753856927128, -315.3201227861279676 ) ) ;
#12415=CARTESIAN_POINT ( 'NONE',  ( 752.7379699480933368, -132.0090635724257595, -361.9858362298580232 ) ) ;
#12421=CARTESIAN_POINT ( 'NONE',  ( 805.0032342141413437, -133.5436935675110419, -314.9967657858572352 ) ) ;
#12425=CARTESIAN_POINT ( 'NONE',  ( 808.3070685750230950, -258.9982390220561115, -361.1904061080339261 ) ) ;
#12426=CARTESIAN_POINT ( 'NONE',  ( 758.8095938919644823, -440.0891481129645513, -311.6929314249762797 ) ) ;
#12429=CARTESIAN_POINT ( 'NONE',  ( 781.2497674668890113, -348.3510508353228943, -375.3608509340180603 ) ) ;
#12430=CARTESIAN_POINT ( 'NONE',  ( 814.9108240113580450, -88.27096629478390355, -337.5031285880265273 ) ) ;
#12432=CARTESIAN_POINT ( 'NONE',  ( 767.7687537140311633, -335.9073299311468190, -372.7932403749916830 ) ) ;
#12433=CARTESIAN_POINT ( 'NONE',  ( 759.9999999999992042, -512.9681489794448908, -350.0000000000000000 ) ) ;
#12436=CARTESIAN_POINT ( 'NONE',  ( 781.8018195045266339, -214.2709662947834488, -365.1927285166406705 ) ) ;
#12437=CARTESIAN_POINT ( 'NONE',  ( 754.0944755984390895, -135.6237781080508853, -364.1009440267246760 ) ) ;
#12443=CARTESIAN_POINT ( 'NONE',  ( 773.3843516231979720, -13.44195992623305713, -364.4086373105754433 ) ) ;
#12445=CARTESIAN_POINT ( 'NONE',  ( 758.8095938919642549, 15.91085188703394238, -311.6929314249763365 ) ) ;
#12449=CARTESIAN_POINT ( 'NONE',  ( 810.4231160770870019, -384.5545181178795247, -321.9338519418446936 ) ) ;
#12451=CARTESIAN_POINT ( 'NONE',  ( 803.6646147819161570, -233.9073299311470180, -348.8264449731210561 ) ) ;
#12454=CARTESIAN_POINT ( 'NONE',  ( 755.8894580844503253, -231.8272453906072315, -332.3691319403863531 ) ) ;
#12455=CARTESIAN_POINT ( 'NONE',  ( 803.4237431249931660, -207.1800572038744406, -331.2633955100225194 ) ) ;
#12456=CARTESIAN_POINT ( 'NONE',  ( 801.9419747391806368, -378.4527844766011526, -351.9812246680014027 ) ) ;
#12459=CARTESIAN_POINT ( 'NONE',  ( 792.1044303154645831, -108.4527844766019911, -317.8323909638837677 ) ) ;
#12468=CARTESIAN_POINT ( 'NONE',  ( 795.8262568251477660, -454.3726999360611103, -308.3538107759623585 ) ) ;
#12469=CARTESIAN_POINT ( 'NONE',  ( 808.0189434323515343, -38.08914811296587999, -319.0252816721025511 ) ) ;
#12471=CARTESIAN_POINT ( 'NONE',  ( 771.2633955100217236, -383.9073299311466485, -363.4237431249939618 ) ) ;
#12472=CARTESIAN_POINT ( 'NONE',  ( 758.0580252608178853, -6.452784476602343666, -328.0187753319985404 ) ) ;
#12475=CARTESIAN_POINT ( 'NONE',  ( 759.0159684113467620, -280.9181544815162965, -325.8855110935213020 ) ) ;
#12476=CARTESIAN_POINT ( 'NONE',  ( 811.0346526505616112, -158.6346026584199933, -323.0537975583477532 ) ) ;
#12479=CARTESIAN_POINT ( 'NONE',  ( 785.1593951492109227, 16.45630643248848912, -313.8313994339321766 ) ) ;
#12480=DIRECTION ( 'NONE',  ( -0.000000000000000000, 1.000000000000000000, -0.000000000000000000 ) ) ;
#12481=AXIS2_PLACEMENT_3D ( 'NONE', #10854, #38344, #24235 ) ;
#12484=CARTESIAN_POINT ( 'NONE',  ( 755.0636971347428243, -364.2709662947830793, -341.7834795799807353 ) ) ;
#12485=EDGE_CURVE ( 'NONE', #19801, #13016, #13709, .T. ) ;
#12487=CARTESIAN_POINT ( 'NONE',  ( 797.8822607201568644, -102.5545181178804057, -370.1134526219340160 ) ) ;
#12488=CARTESIAN_POINT ( 'NONE',  ( 803.2186876482843445, -103.9874144716873161, -350.0220218866286928 ) ) ;
#12491=CARTESIAN_POINT ( 'NONE',  ( 788.8264449731200330, -21.18005720387502677, -363.6646147819171233 ) ) ;
#12492=CARTESIAN_POINT ( 'NONE',  ( 764.0069404352550464, -135.0783235625962959, -359.2566176426627180 ) ) ;
#12493=CARTESIAN_POINT ( 'NONE',  ( 755.5713283507202505, -125.3618753856928834, -334.6858677611754729 ) ) ;
#12496=CARTESIAN_POINT ( 'NONE',  ( 790.8726784830453198, -418.7146871989590409, -362.5472867521010585 ) ) ;
#12502=CARTESIAN_POINT ( 'NONE',  ( 809.0717654672305343, -268.9181544815162397, -360.1688906516309885 ) ) ;
#12509=CARTESIAN_POINT ( 'NONE',  ( 766.0291762391763086, -130.9181544815166660, -360.7704444035551319 ) ) ;
#12510=CARTESIAN_POINT ( 'NONE',  ( 800.0135310231082713, -110.0891481129656597, -325.0180583372163028 ) ) ;
#12511=CARTESIAN_POINT ( 'NONE',  ( 762.1405469898973024, -289.5436935675105019, -357.8594530101016176 ) ) ;
#12514=CARTESIAN_POINT ( 'NONE',  ( 754.8072714833581358, -412.8164208402372992, -338.1981804954720587 ) ) ;
#12515=CARTESIAN_POINT ( 'NONE',  ( 755.0636971347428243, -76.27096629478394618, -341.7834795799807353 ) ) ;
#12522=CARTESIAN_POINT ( 'NONE',  ( 762.1177392798416577, -354.5545181178796383, -309.8865473780659272 ) ) ;
#12525=CARTESIAN_POINT ( 'NONE',  ( 804.4286716492782716, -281.3618753856923718, -345.3141322388244703 ) ) ;
#12527=CARTESIAN_POINT ( 'NONE',  ( 763.8424801807145741, -186.0090635724255890, -320.5453621957614700 ) ) ;
#12531=CARTESIAN_POINT ( 'NONE',  ( 800.9747183278959710, -372.9982390220557704, -311.9810565676471583 ) ) ;
#12536=CARTESIAN_POINT ( 'NONE',  ( 751.6929314249748586, -30.99823902205680071, -318.8095938919659034 ) ) ;
#12537=CARTESIAN_POINT ( 'NONE',  ( 788.8264449731200330, -261.1800572038741848, -363.6646147819171233 ) ) ;
#12542=CARTESIAN_POINT ( 'NONE',  ( 780.5290396650775619, -12.35105083532396897, -365.2837595273619513 ) ) ;
#12543=CARTESIAN_POINT ( 'NONE',  ( 779.9911637788978851, -452.9681489794448339, -340.0036600600989232 ) ) ;
#12548=CARTESIAN_POINT ( 'NONE',  ( 780.5290396650775619, -324.3510508353229511, -365.2837595273619513 ) ) ;
#12552=CARTESIAN_POINT ( 'NONE',  ( 751.2241431872005251, -352.1692326535046504, -359.9636004259367610 ) ) ;
#12558=CARTESIAN_POINT ( 'NONE',  ( 792.3570229623688874, -189.1800572038744122, -373.1304606946836202 ) ) ;
#12561=CARTESIAN_POINT ( 'NONE',  ( 771.2633955100217236, -167.9073299311473022, -363.4237431249939618 ) ) ;
#12564=CARTESIAN_POINT ( 'NONE',  ( 793.0897708529556667, -462.5545181178792973, -361.3366627262616362 ) ) ;
#12570=ORIENTED_EDGE ( 'NONE', *, *, #25566, .F. ) ;
#12571=CARTESIAN_POINT ( 'NONE',  ( 796.9571628226829034, -431.4636090269702322, -321.2382568024804641 ) ) ;
#12573=CARTESIAN_POINT ( 'NONE',  ( 786.2694204179717872, -237.2817908451526421, -305.1769319972829067 ) ) ;
#12576=CARTESIAN_POINT ( 'NONE',  ( 804.4286716492782716, -185.3618753856926844, -345.3141322388244703 ) ) ;
#12577=CARTESIAN_POINT ( 'NONE',  ( 757.2208543904082489, -352.7146871989593251, -350.9844846989624330 ) ) ;
#12579=CARTESIAN_POINT ( 'NONE',  ( 786.2694204179717872, -237.2817908451526421, -305.1769319972829067 ) ) ;
#12580=CARTESIAN_POINT ( 'NONE',  ( 772.4999999999993179, -512.9681489794448908, -309.9999999999998863 ) ) ;
#12581=CARTESIAN_POINT ( 'NONE',  ( 779.9999999999992042, -452.9681489794448339, -329.9999999999999432 ) ) ;
#12582=CARTESIAN_POINT ( 'NONE',  ( 796.1575198192839480, -30.00906357242607925, -359.4546378042384163 ) ) ;
#12584=CARTESIAN_POINT ( 'NONE',  ( 803.8651313633788504, -437.2601417444135450, -332.4468031744301015 ) ) ;
#12585=CARTESIAN_POINT ( 'NONE',  ( 814.9108240113580450, -280.2709662947833067, -337.5031285880265273 ) ) ;
#12590=CARTESIAN_POINT ( 'NONE',  ( 762.3223304703356007, -55.54369356751127640, -322.3223304703362828 ) ) ;
#12593=CARTESIAN_POINT ( 'NONE',  ( 768.8385539511368734, -119.2601417444145397, -306.4236121716840557 ) ) ;
#12595=CARTESIAN_POINT ( 'NONE',  ( 810.7187646348534145, -402.4527844766010389, -356.7737145352016341 ) ) ;
#12597=ADVANCED_FACE ( 'NONE', ( #18616, #32938 ), #43535, .F. ) ;
#12600=CARTESIAN_POINT ( 'NONE',  ( 788.7366044899766848, -395.9073299311465348, -316.5762568750059813 ) ) ;
#12602=CARTESIAN_POINT ( 'NONE',  ( 757.7880784355613741, -42.00906357242603661, -312.4576283171834916 ) ) ;
#12608=CARTESIAN_POINT ( 'NONE',  ( 755.8398074228967971, -235.4419599262323857, -333.4516893846970333 ) ) ;
#12609=CARTESIAN_POINT ( 'NONE',  ( 758.0580252608178853, -126.4527844766019626, -328.0187753319985404 ) ) ;
#12611=CARTESIAN_POINT ( 'NONE',  ( 752.4576283171824116, -237.0783235625960117, -317.7880784355627952 ) ) ;
#12615=CARTESIAN_POINT ( 'NONE',  ( 762.3223304703356007, -175.5436935675108998, -322.3223304703362828 ) ) ;
#12617=CARTESIAN_POINT ( 'NONE',  ( 758.8095938919642549, -80.08914811296574499, -311.6929314249763365 ) ) ;
#12618=CARTESIAN_POINT ( 'NONE',  ( 756.5762568750052424, -75.18005720387485269, -348.7366044899774238 ) ) ;
#12620=CARTESIAN_POINT ( 'NONE',  ( 783.0745993439762742, -8.190881754244330182, -365.1016975059196739 ) ) ;
#12622=CARTESIAN_POINT ( 'NONE',  ( 760.7433823573367135, -348.0090635724251342, -355.9930595647440441 ) ) ;
#12628=CARTESIAN_POINT ( 'NONE',  ( 802.5472867521000353, -340.3726999360615082, -350.8726784830461156 ) ) ;
#12629=CARTESIAN_POINT ( 'NONE',  ( 778.1981804954714335, -322.2709662947830225, -314.8072714833589885 ) ) ;
#12630=CARTESIAN_POINT ( 'NONE',  ( 778.2165204200184689, -166.8164208402382087, -364.9363028652563230 ) ) ;
#12634=CARTESIAN_POINT ( 'NONE',  ( 773.3843516231979720, -277.4419599262322436, -364.4086373105754433 ) ) ;
#12635=CARTESIAN_POINT ( 'NONE',  ( 749.5768839229115201, -132.5545181178802920, -358.0661480581553064 ) ) ;
#12641=CARTESIAN_POINT ( 'NONE',  ( 744.7301800767020268, -124.8164208402383366, -337.4774526936615189 ) ) ;
#12644=CARTESIAN_POINT ( 'NONE',  ( 808.0189434323515343, -278.0891481129651197, -319.0252816721025511 ) ) ;
#12648=CARTESIAN_POINT ( 'NONE',  ( 810.1134526219336749, -344.5328690171410813, -357.8822607201570349 ) ) ;
#12649=CARTESIAN_POINT ( 'NONE',  ( 796.7737145352015204, -92.63460265842026331, -370.7187646348536987 ) ) ;
#12651=CARTESIAN_POINT ( 'NONE',  ( 767.6429770376289525, -369.1800572038739574, -306.8695393053162093 ) ) ;
#12656=CARTESIAN_POINT ( 'NONE',  ( 803.8556311672234642, -129.6237781080508853, -365.6418435158340117 ) ) ;
#12661=CARTESIAN_POINT ( 'NONE',  ( 754.8983024940795303, -18.89650538077849617, -336.9254006560228163 ) ) ;
#12663=CARTESIAN_POINT ( 'NONE',  ( 783.7566961878529810, -432.8965053807771142, -305.1792804349288417 ) ) ;
#12667=CARTESIAN_POINT ( 'NONE',  ( 773.7305795820266212, -369.2817908451523294, -374.8230680027170365 ) ) ;
#12668=CARTESIAN_POINT ( 'NONE',  ( 788.7366044899766848, -227.9073299311471033, -316.5762568750059813 ) ) ;
#12672=CARTESIAN_POINT ( 'NONE',  ( 787.5531968255692163, -213.8272453906073167, -316.1348686366205811 ) ) ;
#12673=CARTESIAN_POINT ( 'NONE',  ( 756.5762568750052424, -219.1800572038744122, -348.7366044899774238 ) ) ;
#12674=CARTESIAN_POINT ( 'NONE',  ( 803.6646147819162707, -425.9073299311463643, -348.8264449731211130 ) ) ;
#12677=CARTESIAN_POINT ( 'NONE',  ( 800.0135310231082713, -110.0891481129656597, -325.0180583372163028 ) ) ;
#12686=CARTESIAN_POINT ( 'NONE',  ( 814.8207195650702488, -434.1908817542430370, -336.2433038121456548 ) ) ;
#12687=CARTESIAN_POINT ( 'NONE',  ( 813.1304606946831655, -41.90732993114767879, -352.3570229623691716 ) ) ;
#12689=CARTESIAN_POINT ( 'NONE',  ( 804.4286716492782716, -401.3618753856920307, -345.3141322388244703 ) ) ;
#12690=CARTESIAN_POINT ( 'NONE',  ( 791.9812246680005501, -20.63460265842048003, -361.9419747391813189 ) ) ;
#12693=CARTESIAN_POINT ( 'NONE',  ( 798.5707757039680246, -293.4636090269707438, -356.7845633553585003 ) ) ;
#12694=CARTESIAN_POINT ( 'NONE',  ( 751.9810565676468741, -170.0891481129654608, -360.9747183278973921 ) ) ;
#12700=CARTESIAN_POINT ( 'NONE',  ( 807.5423716828161105, -225.0783235625959833, -362.2119215644372048 ) ) ;
#12704=CARTESIAN_POINT ( 'NONE',  ( 757.8323909638827445, -362.6346026584194533, -352.1044303154654358 ) ) ;
#12707=CARTESIAN_POINT ( 'NONE',  ( 771.3260364891663130, -115.6454272087894424, -306.0683387631859773 ) ) ;
#12708=CARTESIAN_POINT ( 'NONE',  ( 775.9200461376533440, -143.8055962898690154, -315.3028492785443291 ) ) ;
#12711=CARTESIAN_POINT ( 'NONE',  ( 768.0187753319979720, -56.63460265842036279, -318.0580252608186242 ) ) ;
#12712=CARTESIAN_POINT ( 'NONE',  ( 756.1348686366196716, -161.2601417444143976, -347.5531968255698416 ) ) ;
#12714=CARTESIAN_POINT ( 'NONE',  ( 805.9055244015594326, -3.623778108051270319, -315.8990559732753240 ) ) ;
#12720=CARTESIAN_POINT ( 'NONE',  ( 746.4236121716829757, -255.8272453906072315, -328.8385539511384650 ) ) ;
#12727=CARTESIAN_POINT ( 'NONE',  ( 790.0220218866281812, -103.0999726633349525, -363.2186876482849129 ) ) ;
#12728=CARTESIAN_POINT ( 'NONE',  ( 803.6646147819161570, -113.9073299311474301, -348.8264449731210561 ) ) ;
#12730=CARTESIAN_POINT ( 'NONE',  ( 788.7366044899766848, -299.9073299311468759, -316.5762568750059813 ) ) ;
#12732=CARTESIAN_POINT ( 'NONE',  ( 755.0636971347428243, -412.2709662947829088, -341.7834795799807353 ) ) ;
#12733=CARTESIAN_POINT ( 'NONE',  ( 795.1360043628807261, -68.08914811296575920, -360.2193346964456282 ) ) ;
#12739=CARTESIAN_POINT ( 'NONE',  ( 793.5525998758768083, -343.0999726633342561, -372.6845335610516941 ) ) ;
#12741=CARTESIAN_POINT ( 'NONE',  ( 762.1405469898971887, -289.5436935675103882, -357.8594530101015607 ) ) ;
#12743=CARTESIAN_POINT ( 'NONE',  ( 755.8894580844503253, -183.8272453906074020, -332.3691319403863531 ) ) ;
#12747=CARTESIAN_POINT ( 'NONE',  ( 767.7687537140311633, -383.9073299311466485, -372.7932403749916830 ) ) ;
#12752=CARTESIAN_POINT ( 'NONE',  ( 747.2067596250078623, -27.18005720387500901, -352.2312462859687230 ) ) ;
#12753=CARTESIAN_POINT ( 'NONE',  ( 762.3223304703356007, -247.5436935675106724, -322.3223304703362828 ) ) ;
#12758=CARTESIAN_POINT ( 'NONE',  ( 789.9200121543843807, -49.98741447168749374, -317.0176451133914384 ) ) ;
#12765=CARTESIAN_POINT ( 'NONE',  ( 772.3691319403857278, -335.2601417444137724, -315.8894580844506663 ) ) ;
#12768=CARTESIAN_POINT ( 'NONE',  ( 801.9858362298568863, -363.0783235625955854, -312.7379699480935642 ) ) ;
#12772=( GEOMETRIC_REPRESENTATION_CONTEXT ( 3 ) GLOBAL_UNCERTAINTY_ASSIGNED_CONTEXT ( ( #15357 ) ) GLOBAL_UNIT_ASSIGNED_CONTEXT ( ( #25332, #29037, #8245 ) ) REPRESENTATION_CONTEXT ( 'NONE', 'WORKASPACE' ) );
#12773=CARTESIAN_POINT ( 'NONE',  ( 772.3691319403857278, -95.26014174441461080, -315.8894580844506663 ) ) ;
#12775=CARTESIAN_POINT ( 'NONE',  ( 782.4968714119720516, -226.8164208402380098, -305.0891759886411023 ) ) ;
#12777=EDGE_LOOP ( 'NONE', ( #26206, #4904, #41721, #28345 ) ) ;
#12778=CARTESIAN_POINT ( 'NONE',  ( 754.8072714833583632, -172.8164208402381519, -338.1981804954721156 ) ) ;
#12780=CARTESIAN_POINT ( 'NONE',  ( 781.7834795799800531, -322.8164208402377540, -315.0636971347436202 ) ) ;
#12781=CARTESIAN_POINT ( 'NONE',  ( 800.9840315886518738, -460.9181544815156713, -354.1144889064786412 ) ) ;
#12789=CARTESIAN_POINT ( 'NONE',  ( 779.4763451958990572, -440.7363362996975980, -365.0264073115438919 ) ) ;
#12794=CARTESIAN_POINT ( 'NONE',  ( 748.6759233522253680, -232.3726999360617924, -324.3348316497537098 ) ) ;
#12798=CARTESIAN_POINT ( 'NONE',  ( 781.7834795799800531, -202.8164208402380950, -315.0636971347436202 ) ) ;
#12799=CARTESIAN_POINT ( 'NONE',  ( 804.1601925771018387, -367.4419599262319025, -346.5483106153029098 ) ) ;
#12801=CARTESIAN_POINT ( 'NONE',  ( 754.3581564841646241, -209.4636090269709996, -316.1443688327762516 ) ) ;
#12804=CARTESIAN_POINT ( 'NONE',  ( 763.8424801807145741, -66.00906357242595845, -320.5453621957614700 ) ) ;
#12809=CARTESIAN_POINT ( 'NONE',  ( 802.7791456095903868, -436.7146871989589272, -329.0155153010375102 ) ) ;
#12810=CARTESIAN_POINT ( 'NONE',  ( 772.4837098697145166, -287.3618753856923718, -374.5518280994205611 ) ) ;
#12812=CARTESIAN_POINT ( 'NONE',  ( 799.9999999999993179, 205.0000000000000568, -339.9999999999999432 ) ) ;
#12813=CARTESIAN_POINT ( 'NONE',  ( 785.3141322388236176, -45.72551174932949181, -364.4286716492789537 ) ) ;
#12816=CARTESIAN_POINT ( 'NONE',  ( 815.1787889125755555, -174.8965053807779952, -343.7953271457877804 ) ) ;
#12818=CARTESIAN_POINT ( 'NONE',  ( 800.9747183278959710, -396.9982390220556567, -311.9810565676471583 ) ) ;
#12823=CARTESIAN_POINT ( 'NONE',  ( 804.4286716492782716, -377.3618753856920875, -345.3141322388244703 ) ) ;
#12829=CARTESIAN_POINT ( 'NONE',  ( 766.7756240680305382, -230.5328690171415076, -361.5560724626415663 ) ) ;
#12830=AXIS2_PLACEMENT_3D ( 'NONE', #24559, #9589, #27360 ) ;
#12833=CARTESIAN_POINT ( 'NONE',  ( 815.0009284576459549, -246.3510508353232638, -338.7629533639073429 ) ) ;
#12837=CARTESIAN_POINT ( 'NONE',  ( 783.0433043558608688, -24.89650538077847486, -315.1538015810313027 ) ) ;
#12838=CARTESIAN_POINT ( 'NONE',  ( 759.7806653035534055, -174.9982390220563673, -324.8639956371180801 ) ) ;
#12840=CARTESIAN_POINT ( 'NONE',  ( 811.0346526505616112, -86.63460265842023489, -323.0537975583477532 ) ) ;
#12841=CARTESIAN_POINT ( 'NONE',  ( 797.8594530101009923, -61.54369356751124798, -322.1405469898982119 ) ) ;
#12842=EDGE_LOOP ( 'NONE', ( #21763, #36658 ) ) ;
#12843=CARTESIAN_POINT ( 'NONE',  ( 784.1219089521767955, -21.28179084515337749, -315.0488828828318333 ) ) ;
#12845=CARTESIAN_POINT ( 'NONE',  ( 769.9779781133707957, -355.0999726633341993, -316.7813123517150871 ) ) ;
#12857=CARTESIAN_POINT ( 'NONE',  ( 798.5707757039680246, -317.4636090269706301, -356.7845633553585003 ) ) ;
#12858=CARTESIAN_POINT ( 'NONE',  ( 767.8955696845333705, -312.4527844766012663, -362.1676090361162323 ) ) ;
#12859=CARTESIAN_POINT ( 'NONE',  ( 809.0717654672305343, -148.9181544815166092, -360.1688906516309885 ) ) ;
#12863=CARTESIAN_POINT ( 'NONE',  ( 803.2186876482843445, -271.9874144716868045, -350.0220218866286928 ) ) ;
#12864=CARTESIAN_POINT ( 'NONE',  ( 750.9282345327678740, -112.9181544815167229, -319.8311093483690115 ) ) ;
#12873=CARTESIAN_POINT ( 'NONE',  ( 814.2001403089898304, -185.3618753856926844, -347.4397851343538264 ) ) ;
#12876=CARTESIAN_POINT ( 'NONE',  ( 782.4968714119720516, -298.8164208402377540, -305.0891759886411023 ) ) ;
#12881=CARTESIAN_POINT ( 'NONE',  ( 795.6651683502461765, -346.7146871989592682, -371.3240766477733814 ) ) ;
#12882=CARTESIAN_POINT ( 'NONE',  ( 800.9747183278959710, -108.9982390220565804, -311.9810565676471583 ) ) ;
#12885=CARTESIAN_POINT ( 'NONE',  ( 814.5518280994195948, -399.7255117493283478, -332.4837098697145734 ) ) ;
#12891=CARTESIAN_POINT ( 'NONE',  ( 794.9819416627830151, -228.9982390220561683, -319.9864689768909898 ) ) ;
#12892=CARTESIAN_POINT ( 'NONE',  ( 788.7631598425961101, -169.4419599262325562, -305.7194118038759143 ) ) ;
#12893=DIRECTION ( 'NONE',  ( -1.000000000000000000, -0.000000000000000000, -0.000000000000000000 ) ) ;
#12896=ORIENTED_EDGE ( 'NONE', *, *, #40197, .F. ) ;
#12897=CARTESIAN_POINT ( 'NONE',  ( 758.6633372737375112, 3.467130982857797417, -326.9102291470432533 ) ) ;
#12900=CARTESIAN_POINT ( 'NONE',  ( 813.2346286133761168, -437.2601417444135450, -328.9521613784389160 ) ) ;
#12904=CARTESIAN_POINT ( 'NONE',  ( 814.2805881961230625, -361.6454272087887603, -331.2368401574024119 ) ) ;
#12909=CARTESIAN_POINT ( 'NONE',  ( 760.7433823573367135, -204.0090635724255606, -355.9930595647440441 ) ) ;
#12910=CARTESIAN_POINT ( 'NONE',  ( 801.9419747391806368, -234.4527844766016358, -351.9812246680014027 ) ) ;
#12911=CARTESIAN_POINT ( 'NONE',  ( 755.0636971347428243, -412.2709662947829088, -341.7834795799807353 ) ) ;
#12914=CARTESIAN_POINT ( 'NONE',  ( 768.0187753319979720, -104.6346026584202207, -318.0580252608186242 ) ) ;
#12925=CARTESIAN_POINT ( 'NONE',  ( 791.0478386215596629, -453.8272453906066630, -306.7653713866226326 ) ) ;
#12926=CARTESIAN_POINT ( 'NONE',  ( 808.0189434323515343, -62.08914811296580183, -319.0252816721025511 ) ) ;
#12928=CARTESIAN_POINT ( 'NONE',  ( 792.1044303154645831, -444.4527844766009821, -317.8323909638837677 ) ) ;
#12929=CARTESIAN_POINT ( 'NONE',  ( 756.3353852180820240, -29.90732993114772142, -331.1735550268787733 ) ) ;
#12932=CARTESIAN_POINT ( 'NONE',  ( 757.0176451133909268, -301.0999726633342561, -349.9200121543848354 ) ) ;
#12933=CARTESIAN_POINT ( 'NONE',  ( 746.8695393053150156, -197.9073299311472169, -327.6429770376306010 ) ) ;
#12937=VECTOR ( 'NONE', #44435, 1000.000000000000000 ) ;
#12939=CARTESIAN_POINT ( 'NONE',  ( 814.8230680027162407, -221.8055962898687881, -333.7305795820267917 ) ) ;
#12942=CARTESIAN_POINT ( 'NONE',  ( 782.5225473063381969, -286.2709662947833635, -375.2698199232970637 ) ) ;
#12946=CARTESIAN_POINT ( 'NONE',  ( 756.5762568750052424, -339.1800572038740142, -348.7366044899774238 ) ) ;
#12949=CARTESIAN_POINT ( 'NONE',  ( 795.8262568251477660, -94.37269993606224716, -308.3538107759623585 ) ) ;
#12950=CARTESIAN_POINT ( 'NONE',  ( 783.0433043558608688, -144.8965053807781089, -315.1538015810313027 ) ) ;
#12954=CARTESIAN_POINT ( 'NONE',  ( 804.4286716492782716, -65.36187538569306810, -345.3141322388244703 ) ) ;
#12955=CARTESIAN_POINT ( 'NONE',  ( 799.4546378042377910, -153.0783235625962675, -356.1575198192848006 ) ) ;
#12959=CARTESIAN_POINT ( 'NONE',  ( 814.8230680027162407, 18.19440371013048008, -333.7305795820267917 ) ) ;
#12964=CARTESIAN_POINT ( 'NONE',  ( 766.4474001241216001, -283.0999726633344267, -307.3154664389482491 ) ) ;
#12971=CARTESIAN_POINT ( 'NONE',  ( 775.8780910478218402, -105.2817908451530968, -364.9511171171680530 ) ) ;
#12972=CARTESIAN_POINT ( 'NONE',  ( 759.9864689768902508, -98.08914811296568814, -354.9819416627836404 ) ) ;
#12973=CARTESIAN_POINT ( 'NONE',  ( 758.0580252608178853, -318.4527844766014368, -328.0187753319985404 ) ) ;
#12977=CARTESIAN_POINT ( 'NONE',  ( 778.1981804954714335, -442.2709662947826814, -314.8072714833589885 ) ) ;
#12980=FACE_OUTER_BOUND ( 'NONE', #40467, .T. ) ;
#12985=EDGE_LOOP ( 'NONE', ( #182, #583, #15784, #6654 ) ) ;
#12986=CARTESIAN_POINT ( 'NONE',  ( 744.6391490659812007, -326.7363362996979390, -338.7502325331110455 ) ) ;
#12988=CARTESIAN_POINT ( 'NONE',  ( 778.2165204200184689, -334.8164208402376403, -364.9363028652563230 ) ) ;
#12989=CARTESIAN_POINT ( 'NONE',  ( 790.9844846989617508, -190.3726999360619629, -317.2208543904092721 ) ) ;
#12993=CARTESIAN_POINT ( 'NONE',  ( 796.7737145352015204, -380.6346026584192828, -370.7187646348536987 ) ) ;
#12998=CARTESIAN_POINT ( 'NONE',  ( 751.6929314249748586, -6.998239022056885972, -318.8095938919659034 ) ) ;
#12999=CARTESIAN_POINT ( 'NONE',  ( 804.9363028652555840, -256.2709662947834204, -338.2165204200192079 ) ) ;
#13003=CARTESIAN_POINT ( 'NONE',  ( 754.9735926884551418, -42.35105083532388193, -340.5236548041000333 ) ) ;
#13010=CARTESIAN_POINT ( 'NONE',  ( 765.0180583372156207, -72.99823902205667991, -360.0135310231089534 ) ) ;
#13011=CARTESIAN_POINT ( 'NONE',  ( 802.7791456095903868, -364.7146871989592114, -329.0155153010375102 ) ) ;
#13014=CARTESIAN_POINT ( 'NONE',  ( 808.7758568127978833, -364.1692326535046504, -320.0363995740631822 ) ) ;
#13016=VERTEX_POINT ( 'NONE', #4520 ) ;
#13020=CARTESIAN_POINT ( 'NONE',  ( 749.2812353651451076, -222.4527844766016642, -323.2262854647983090 ) ) ;
#13023=CARTESIAN_POINT ( 'NONE',  ( 755.3201227861273992, -219.7255117493289447, -345.3687786644892981 ) ) ;
#13025=CARTESIAN_POINT ( 'NONE',  ( 771.1735550268778070, -321.1800572038740142, -316.3353852180827630 ) ) ;
#13026=CARTESIAN_POINT ( 'NONE',  ( 799.2566176426618085, -456.0090635724247932, -324.0069404352559559 ) ) ;
#13031=DIRECTION ( 'NONE',  ( 0.000000000000000000, -1.000000000000000000, 0.000000000000000000 ) ) ;
#13033=CARTESIAN_POINT ( 'NONE',  ( 776.9254006560222479, -452.1908817542428665, -314.8983024940802125 ) ) ;
#13035=DIRECTION ( 'NONE',  ( 0.000000000000000000, 1.000000000000000000, 0.000000000000000000 ) ) ;
#13037=CARTESIAN_POINT ( 'NONE',  ( 797.8822607201568644, -222.5545181178800362, -370.1134526219340160 ) ) ;
#13041=CARTESIAN_POINT ( 'NONE',  ( 785.3141322388236176, -189.7255117493290300, -364.4286716492789537 ) ) ;
#13042=CARTESIAN_POINT ( 'NONE',  ( 805.1016975059191054, -366.8965053807773984, -343.0745993439771837 ) ) ;
#13043=CARTESIAN_POINT ( 'NONE',  ( 814.4686193811664907, -243.2817908451526705, -346.2056067578752732 ) ) ;
#13044=DIRECTION ( 'NONE',  ( 0.000000000000000000, 0.000000000000000000, -1.000000000000000000 ) ) ;
#13046=CARTESIAN_POINT ( 'NONE',  ( 761.4292242960306112, -89.46360902697134065, -323.2154366446414429 ) ) ;
#13052=CARTESIAN_POINT ( 'NONE',  ( 770.0799878456142551, -421.9874144716863498, -362.9823548866085616 ) ) ;
#13053=CARTESIAN_POINT ( 'NONE',  ( 758.8095938919644823, -272.0891481129651197, -311.6929314249762797 ) ) ;
#13056=CARTESIAN_POINT ( 'NONE',  ( 801.9419747391806368, -42.45278447660223264, -351.9812246680014027 ) ) ;
#13059=CARTESIAN_POINT ( 'NONE',  ( 815.0009284576459549, -150.3510508353235480, -338.7629533639073429 ) ) ;
#13061=CARTESIAN_POINT ( 'NONE',  ( 758.8095938919642549, -416.0891481129645513, -311.6929314249763365 ) ) ;
#13066=CARTESIAN_POINT ( 'NONE',  ( 785.3687786644884454, -419.3618753856918033, -315.3201227861279676 ) ) ;
#13073=CARTESIAN_POINT ( 'NONE',  ( 805.0264073115434940, -246.3510508353232638, -339.4763451958999099 ) ) ;
#13074=CARTESIAN_POINT ( 'NONE',  ( 756.5762568750052424, -123.1800572038747106, -348.7366044899774238 ) ) ;
#13076=CARTESIAN_POINT ( 'NONE',  ( 811.6461892240364477, -244.7146871989596093, -324.1737431748509835 ) ) ;
#13083=CARTESIAN_POINT ( 'NONE',  ( 765.8855110935204493, -22.16923265350575889, -319.0159684113471599 ) ) ;
#13084=CARTESIAN_POINT ( 'NONE',  ( 788.7366044899766848, -179.9073299311472454, -316.5762568750059813 ) ) ;
#13087=CARTESIAN_POINT ( 'NONE',  ( 767.6429770376289525, -105.1800572038747248, -306.8695393053162093 ) ) ;
#13088=CARTESIAN_POINT ( 'NONE',  ( 797.8594530101009923, -109.5436935675110988, -322.1405469898982119 ) ) ;
#13090=CARTESIAN_POINT ( 'NONE',  ( 776.9254006560222479, -44.19088175424421649, -314.8983024940802125 ) ) ;
#13092=CARTESIAN_POINT ( 'NONE',  ( 761.4292242960306112, -353.4636090269705733, -323.2154366446414429 ) ) ;
#13098=CARTESIAN_POINT ( 'NONE',  ( 769.0155153010367712, -370.3726999360613377, -362.7791456095907279 ) ) ;
#13099=CARTESIAN_POINT ( 'NONE',  ( 788.8264449731200330, -333.1800572038740142, -363.6646147819171233 ) ) ;
#13100=CARTESIAN_POINT ( 'NONE',  ( 802.2119215644370342, -150.0090635724257027, -367.5423716828165084 ) ) ;
#13104=CARTESIAN_POINT ( 'NONE',  ( 798.7617431975189675, -267.6237781080504305, -323.0428371773161871 ) ) ;
#13106=CARTESIAN_POINT ( 'NONE',  ( 745.5313806188320314, -111.2817908451530968, -333.7943932421247268 ) ) ;
#13113=CARTESIAN_POINT ( 'NONE',  ( 749.2812353651451076, -174.4527844766018063, -323.2262854647983090 ) ) ;
#13116=CARTESIAN_POINT ( 'NONE',  ( 796.7737145352015204, -308.6346026584195670, -370.7187646348536987 ) ) ;
#13120=ORIENTED_EDGE ( 'NONE', *, *, #1836, .F. ) ;
#13122=CARTESIAN_POINT ( 'NONE',  ( 791.1614460488616487, -371.2601417444136587, -373.5763878283158874 ) ) ;
#13124=CARTESIAN_POINT ( 'NONE',  ( 792.2312462859673587, -131.9073299311473875, -307.2067596250082602 ) ) ;
#13125=EDGE_CURVE ( 'NONE', #15909, #3566, #484, .T. ) ;
#13127=CARTESIAN_POINT ( 'NONE',  ( 782.5225473063381969, -382.2709662947828519, -375.2698199232970637 ) ) ;
#13132=CARTESIAN_POINT ( 'NONE',  ( 744.9990715423526808, -138.3510508353236048, -341.2370466360926002 ) ) ;
#13137=CARTESIAN_POINT ( 'NONE',  ( 804.1601925771018387, -7.441959926233078448, -346.5483106153029098 ) ) ;
#13140=CARTESIAN_POINT ( 'NONE',  ( 804.7487373415286811, -19.54369356751139364, -364.7487373415288516 ) ) ;
#13143=CARTESIAN_POINT ( 'NONE',  ( 809.0717654672305343, -412.9181544815157281, -360.1688906516309885 ) ) ;
#13144=CARTESIAN_POINT ( 'NONE',  ( 797.8594530101008786, -253.5436935675104735, -322.1405469898980982 ) ) ;
#13147=CARTESIAN_POINT ( 'NONE',  ( 763.0428371773158460, -203.4636090269709996, -358.7617431975195359 ) ) ;
#13148=CARTESIAN_POINT ( 'NONE',  ( 794.9819416627830151, -204.9982390220562820, -319.9864689768909898 ) ) ;
#13149=CARTESIAN_POINT ( 'NONE',  ( 774.6312213355098493, -407.3618753856920307, -364.6798772138717482 ) ) ;
#13154=CARTESIAN_POINT ( 'NONE',  ( 789.8657795001898876, -452.9681489794449476, -362.9715936389367812 ) ) ;
#13156=CARTESIAN_POINT ( 'NONE',  ( 812.3518521366052028, -1.099972663335260226, -326.5853460496235243 ) ) ;
#13162=CARTESIAN_POINT ( 'NONE',  ( 805.6418435158337843, -461.4636090269701754, -363.8556311672236916 ) ) ;
#13163=CARTESIAN_POINT ( 'NONE',  ( 815.2698199232962679, -64.81642084023852135, -342.5225473063383674 ) ) ;
#13165=CARTESIAN_POINT ( 'NONE',  ( 785.3687786644884454, -443.3618753856917465, -315.3201227861279676 ) ) ;
#13166=CARTESIAN_POINT ( 'NONE',  ( 758.0580252608178853, -30.45278447660226817, -328.0187753319985404 ) ) ;
#13168=CARTESIAN_POINT ( 'NONE',  ( 804.6798772138708955, 8.274488250670337663, -334.6312213355107019 ) ) ;
#13169=CARTESIAN_POINT ( 'NONE',  ( 766.0291762391763086, -298.9181544815161828, -360.7704444035551319 ) ) ;
#13170=CARTESIAN_POINT ( 'NONE',  ( 759.0252816721024374, -216.9982390220562252, -368.0189434323527280 ) ) ;
#13175=CARTESIAN_POINT ( 'NONE',  ( 812.6845335610512393, -247.9874144716867761, -353.5525998758768651 ) ) ;
#13176=EDGE_CURVE ( 'NONE', #35738, #35219, #44678, .T. ) ;
#13178=CARTESIAN_POINT ( 'NONE',  ( 810.7187646348534145, -282.4527844766014937, -356.7737145352016341 ) ) ;
#13182=CARTESIAN_POINT ( 'NONE',  ( 755.5713283507202505, -341.3618753856922012, -334.6858677611754729 ) ) ;
#13185=CARTESIAN_POINT ( 'NONE',  ( 746.0683387631852383, -67.44195992623289726, -331.3260364891676204 ) ) ;
#13186=CARTESIAN_POINT ( 'NONE',  ( 802.7791456095903868, -148.7146871989598935, -329.0155153010375102 ) ) ;
#13191=CARTESIAN_POINT ( 'NONE',  ( 804.9363028652555840, -64.27096629478397460, -338.2165204200192079 ) ) ;
#13192=CARTESIAN_POINT ( 'NONE',  ( 800.7704444035546203, -172.1692326535052757, -326.0291762391768771 ) ) ;
#13195=CARTESIAN_POINT ( 'NONE',  ( 807.5423716828161105, -9.078323562596708030, -362.2119215644372048 ) ) ;
#13202=CARTESIAN_POINT ( 'NONE',  ( 783.7953271457878373, -296.1908817542434917, -375.1787889125761239 ) ) ;
#13208=CARTESIAN_POINT ( 'NONE',  ( 759.0159684113467620, -112.9181544815167229, -325.8855110935213020 ) ) ;
#13209=CARTESIAN_POINT ( 'NONE',  ( 802.1676090361156639, -110.6346026584201638, -327.8955696845344505 ) ) ;
#13210=CARTESIAN_POINT ( 'NONE',  ( 802.1676090361155502, -302.6346026584195670, -327.8955696845344505 ) ) ;
#13212=CARTESIAN_POINT ( 'NONE',  ( 792.1044303154645831, -444.4527844766009821, -317.8323909638837677 ) ) ;
#13215=LINE ( 'NONE', #20124, #7160 ) ;
#13219=CARTESIAN_POINT ( 'NONE',  ( 757.7880784355613741, -330.0090635724251342, -312.4576283171834916 ) ) ;
#13222=CARTESIAN_POINT ( 'NONE',  ( 767.8955696845333705, -312.4527844766012663, -362.1676090361162323 ) ) ;
#13224=CARTESIAN_POINT ( 'NONE',  ( 796.1575198192839480, -174.0090635724256742, -359.4546378042384163 ) ) ;
#13227=CARTESIAN_POINT ( 'NONE',  ( 758.8095938919644823, -368.0891481129647786, -311.6929314249762797 ) ) ;
#13228=PLANE ( 'NONE',  #342 ) ;
#13232=CARTESIAN_POINT ( 'NONE',  ( 744.7301800767019131, -28.81642084023863148, -337.4774526936615757 ) ) ;
#13233=CARTESIAN_POINT ( 'NONE',  ( 758.0580252608178853, -246.4527844766016074, -328.0187753319985404 ) ) ;
#13237=CARTESIAN_POINT ( 'NONE',  ( 798.7617431975189675, -51.62377810805111267, -323.0428371773161871 ) ) ;
#13244=CARTESIAN_POINT ( 'NONE',  ( 755.3201227861273992, -51.72551174932946338, -345.3687786644892981 ) ) ;
#13245=CARTESIAN_POINT ( 'NONE',  ( 766.7756240680305382, -374.5328690171410813, -361.5560724626415663 ) ) ;
#13248=CARTESIAN_POINT ( 'NONE',  ( 810.1134526219336749, -368.5328690171409676, -357.8822607201570349 ) ) ;
#13254=CARTESIAN_POINT ( 'NONE',  ( 772.5602148656447525, -225.7255117493289163, -305.7998596910095443 ) ) ;
#13257=CARTESIAN_POINT ( 'NONE',  ( 754.8072714833583632, -220.8164208402380098, -338.1981804954721156 ) ) ;
#13259=CARTESIAN_POINT ( 'NONE',  ( 765.0180583372156207, -336.9982390220558273, -360.0135310231089534 ) ) ;
#13260=CARTESIAN_POINT ( 'NONE',  ( 771.1735550268778070, 14.81994279612486309, -316.3353852180827630 ) ) ;
#13264=DIRECTION ( 'NONE',  ( -1.000000000000000000, -0.000000000000000000, -0.000000000000000000 ) ) ;
#13266=CARTESIAN_POINT ( 'NONE',  ( 788.7366044899766848, 12.09267006885214180, -316.5762568750059813 ) ) ;
#13269=CARTESIAN_POINT ( 'NONE',  ( 747.6481478633932056, -253.0999726633345119, -353.4146539503763620 ) ) ;
#13272=CARTESIAN_POINT ( 'NONE',  ( 800.0135310231082713, -230.0891481129652618, -325.0180583372163028 ) ) ;
#13273=CARTESIAN_POINT ( 'NONE',  ( 780.5290396650775619, -348.3510508353228943, -365.2837595273619513 ) ) ;
#13274=CARTESIAN_POINT ( 'NONE',  ( 745.7194118038753459, -253.6454272087889876, -348.7631598425976449 ) ) ;
#13277=CARTESIAN_POINT ( 'NONE',  ( 773.4516893846965786, -91.64542720878951343, -315.8398074228977066 ) ) ;
#13280=CARTESIAN_POINT ( 'NONE',  ( 754.9735926884551418, -426.3510508353226669, -340.5236548041000333 ) ) ;
#13281=CARTESIAN_POINT ( 'NONE',  ( 772.5602148656447525, -273.7255117493288026, -305.7998596910095443 ) ) ;
#13284=CARTESIAN_POINT ( 'NONE',  ( 785.3687786644884454, -59.36187538569306810, -315.3201227861279676 ) ) ;
#13286=CARTESIAN_POINT ( 'NONE',  ( 776.2433038121456548, -180.8965053807779952, -374.8207195650711014 ) ) ;
#13288=CARTESIAN_POINT ( 'NONE',  ( 772.5602148656447525, -417.7255117493283478, -305.7998596910095443 ) ) ;
#13293=CARTESIAN_POINT ( 'NONE',  ( 756.3353852180819104, -413.9073299311465348, -331.1735550268788302 ) ) ;
#13299=CARTESIAN_POINT ( 'NONE',  ( 776.9566956441375396, -276.8965053807776258, -364.8461984189686405 ) ) ;
#13300=CARTESIAN_POINT ( 'NONE',  ( 785.3687786644884454, -131.3618753856928834, -315.3201227861279676 ) ) ;
#13302=CARTESIAN_POINT ( 'NONE',  ( 764.3348316497523456, -262.7146871989594956, -308.6759233522265617 ) ) ;
#13307=CARTESIAN_POINT ( 'NONE',  ( 800.7704444035546203, -28.16923265350574468, -326.0291762391768771 ) ) ;
#13308=CARTESIAN_POINT ( 'NONE',  ( 791.9812246680005501, -164.6346026584200217, -361.9419747391813189 ) ) ;
#13310=CARTESIAN_POINT ( 'NONE',  ( 745.7998596910086917, -101.3618753856929544, -332.5602148656461168 ) ) ;
#13312=CARTESIAN_POINT ( 'NONE',  ( 785.3141322388236176, -117.7255117493292715, -364.4286716492789537 ) ) ;
#13313=EDGE_LOOP ( 'NONE', ( #21092, #22725 ) ) ;
#13314=CARTESIAN_POINT ( 'NONE',  ( 759.0159684113467620, -40.91815448151695023, -325.8855110935213020 ) ) ;
#13315=CARTESIAN_POINT ( 'NONE',  ( 766.0291762391763086, -370.9181544815159555, -360.7704444035551319 ) ) ;
#13322=CARTESIAN_POINT ( 'NONE',  ( 757.4527132478984868, -352.3726999360614514, -329.1273215169538844 ) ) ;
#13323=CARTESIAN_POINT ( 'NONE',  ( 788.7366044899766848, -371.9073299311465917, -316.5762568750059813 ) ) ;
#13324=CARTESIAN_POINT ( 'NONE',  ( 805.6418435158337843, -125.4636090269712412, -363.8556311672236916 ) ) ;
#13328=CARTESIAN_POINT ( 'NONE',  ( 747.6481478633932056, -157.0999726633347962, -353.4146539503763620 ) ) ;
#13334=CARTESIAN_POINT ( 'NONE',  ( 767.6429770376291799, -177.1800572038744974, -306.8695393053162093 ) ) ;
#13338=CARTESIAN_POINT ( 'NONE',  ( 810.7187646348534145, -306.4527844766013800, -356.7737145352016341 ) ) ;
#13346=CARTESIAN_POINT ( 'NONE',  ( 795.6651683502461765, -370.7146871989592114, -371.3240766477733814 ) ) ;
#13347=CARTESIAN_POINT ( 'NONE',  ( 812.7932403749906598, -111.1800572038747532, -327.7687537140311633 ) ) ;
#13349=CARTESIAN_POINT ( 'NONE',  ( 772.5602148656447525, -369.7255117493284615, -305.7998596910095443 ) ) ;
#13353=CARTESIAN_POINT ( 'NONE',  ( 798.0661480581538854, -146.5328690171417350, -309.5768839229118043 ) ) ;
#13358=CARTESIAN_POINT ( 'NONE',  ( 789.9200121543843807, -1.987414471687640294, -317.0176451133914384 ) ) ;
#13360=CARTESIAN_POINT ( 'NONE',  ( 814.5518280994195948, 8.274488250670337663, -332.4837098697145734 ) ) ;
#13361=CYLINDRICAL_SURFACE ( 'NONE', #32775, 30.00000000000008171 ) ;
#13365=CARTESIAN_POINT ( 'NONE',  ( 771.3260364891663130, -403.6454272087884760, -306.0683387631859773 ) ) ;
#13367=CARTESIAN_POINT ( 'NONE',  ( 771.2633955100217236, -263.9073299311469327, -363.4237431249939618 ) ) ;
#13371=CARTESIAN_POINT ( 'NONE',  ( 793.9708237608222134, -238.9181544815163534, -319.2295555964448681 ) ) ;
#13372=CARTESIAN_POINT ( 'NONE',  ( 759.9864689768902508, -218.0891481129653187, -354.9819416627836404 ) ) ;
#13373=CARTESIAN_POINT ( 'NONE',  ( 767.8955696845334842, -432.4527844766009252, -362.1676090361161755 ) ) ;
#13378=CARTESIAN_POINT ( 'NONE',  ( 814.4686193811664907, -51.28179084515328867, -346.2056067578752732 ) ) ;
#13385=CARTESIAN_POINT ( 'NONE',  ( 769.0155153010367712, -10.37269993606250473, -362.7791456095907279 ) ) ;
#13387=CARTESIAN_POINT ( 'NONE',  ( 787.5162901302840055, -59.36187538569307520, -305.4481719005793252 ) ) ;
#13389=CARTESIAN_POINT ( 'NONE',  ( 762.3223304703356007, -439.5436935675101040, -322.3223304703362828 ) ) ;
#13390=CARTESIAN_POINT ( 'NONE',  ( 797.6776695296629214, -43.54369356751131903, -357.6776695296636603 ) ) ;
#13393=CARTESIAN_POINT ( 'NONE',  ( 745.7998596910086917, -197.3618753856926560, -332.5602148656461168 ) ) ;
#13397=CARTESIAN_POINT ( 'NONE',  ( 772.4999999999993179, -512.9681489794448908, -370.0000000000000000 ) ) ;
#13398=FACE_OUTER_BOUND ( 'NONE', #5949, .T. ) ;
#13399=CARTESIAN_POINT ( 'NONE',  ( 805.9055244015594326, -267.6237781080504305, -315.8990559732753240 ) ) ;
#13401=CARTESIAN_POINT ( 'NONE',  ( 751.9810565676468741, -266.0891481129651197, -360.9747183278973921 ) ) ;
#13405=CARTESIAN_POINT ( 'NONE',  ( 774.6312213355099630, -335.3618753856920307, -364.6798772138717482 ) ) ;
#13407=CARTESIAN_POINT ( 'NONE',  ( 805.9055244015594326, -51.62377810805111267, -315.8990559732753240 ) ) ;
#13408=CARTESIAN_POINT ( 'NONE',  ( 805.1016975059191054, -150.8965053807781089, -343.0745993439771837 ) ) ;
#13415=CARTESIAN_POINT ( 'NONE',  ( 755.3201227861273992, -75.72551174932937101, -345.3687786644892981 ) ) ;
#13416=CARTESIAN_POINT ( 'NONE',  ( 803.8651313633788504, -173.2601417444143692, -332.4468031744301015 ) ) ;
#13418=CARTESIAN_POINT ( 'NONE',  ( 773.7943932421234194, 0.1944037101305369775, -305.5313806188329409 ) ) ;
#13424=CARTESIAN_POINT ( 'NONE',  ( 749.5768839229115201, -324.5545181178796952, -358.0661480581553064 ) ) ;
#13429=CARTESIAN_POINT ( 'NONE',  ( 790.9844846989617508, -166.3726999360620198, -317.2208543904092721 ) ) ;
#13430=CARTESIAN_POINT ( 'NONE',  ( 759.7806653035534055, -102.9982390220565520, -324.8639956371180801 ) ) ;
#13431=CARTESIAN_POINT ( 'NONE',  ( 800.2193346964446619, -306.9982390220558841, -355.1360043628816925 ) ) ;
#13440=CARTESIAN_POINT ( 'NONE',  ( 745.1792804349281596, -350.1908817542433212, -343.7566961878542884 ) ) ;
#13442=CARTESIAN_POINT ( 'NONE',  ( 791.9812246680005501, -332.6346026584195101, -361.9419747391813189 ) ) ;
#13443=PLANE ( 'NONE',  #35527 ) ;
#13444=CARTESIAN_POINT ( 'NONE',  ( 798.5707757039680246, -173.4636090269710849, -356.7845633553585003 ) ) ;
#13450=CARTESIAN_POINT ( 'NONE',  ( 796.9462024416508257, -372.4527844766012095, -308.9653473494370246 ) ) ;
#13455=CARTESIAN_POINT ( 'NONE',  ( 796.7737145352015204, -20.63460265842048003, -370.7187646348536987 ) ) ;
#13456=CARTESIAN_POINT ( 'NONE',  ( 801.9419747391806368, -258.4527844766016074, -351.9812246680014027 ) ) ;
#13460=CARTESIAN_POINT ( 'NONE',  ( 812.3518521366052028, -25.09997266333519050, -326.5853460496235243 ) ) ;
#13461=CARTESIAN_POINT ( 'NONE',  ( 756.7813123517142913, -43.98741447168752217, -329.9779781133712504 ) ) ;
#13468=CARTESIAN_POINT ( 'NONE',  ( 788.8264449731200330, -69.18005720387488111, -363.6646147819171233 ) ) ;
#13469=CARTESIAN_POINT ( 'NONE',  ( 784.0799538623451781, -347.8055962898683333, -364.6971507214555572 ) ) ;
#13473=CARTESIAN_POINT ( 'NONE',  ( 778.7502325331095108, -360.3510508353228374, -304.6391490659818828 ) ) ;
#13479=CARTESIAN_POINT ( 'NONE',  ( 812.7932403749906598, -207.1800572038744406, -327.7687537140311633 ) ) ;
#13482=CARTESIAN_POINT ( 'NONE',  ( 801.9419747391806368, -210.4527844766016926, -351.9812246680014027 ) ) ;
#13484=CARTESIAN_POINT ( 'NONE',  ( 759.9864689768902508, -314.0891481129650629, -354.9819416627836404 ) ) ;
#13485=CARTESIAN_POINT ( 'NONE',  ( 805.1927285166397041, -16.81642084023866701, -341.8018195045277707 ) ) ;
#13489=ORIENTED_EDGE ( 'NONE', *, *, #20442, .T. ) ;
#13490=CARTESIAN_POINT ( 'NONE',  ( 797.8594530101008786, 10.45630643248850866, -322.1405469898980982 ) ) ;
#13491=CARTESIAN_POINT ( 'NONE',  ( 774.2415430293718828, 19.23444159658009056, -310.5578503957772796 ) ) ;
#13494=CARTESIAN_POINT ( 'NONE',  ( 766.4474001241216001, -235.0999726633344835, -307.3154664389482491 ) ) ;
#13496=CARTESIAN_POINT ( 'NONE',  ( 804.6798772138708955, -207.7255117493289447, -334.6312213355107019 ) ) ;
#13497=CARTESIAN_POINT ( 'NONE',  ( 795.9930595647434757, -387.0783235625955285, -320.7433823573372820 ) ) ;
#13498=( BOUNDED_CURVE ( )  B_SPLINE_CURVE ( 2, ( #28891, #35574, #25417, #42973, #39770, #42527, #254, #31884, #17816, #491, #38849, #10893, #3951, #14597, #11338, #32365, #39538, #14351, #39074, #32588, #18290, #8118, #28670, #24960, #22179, #18045, #32126, #28429, #36273, #36055, #21496, #35819, #42748, #10649, #720, #11110, #25180, #39292, #7895, #14818, #7646, #4630, #11577, #18726, #21725, #4198, #21969, #1166, #4418, #35353, #42287, #931, #15034, #32814, #29122, #7423, #43206, #24729, #25657, #15275, #3728, #7202, #21273, #36947, #40646, #36729, #33263, #29362, #22854, #43652, #19621, #30240, #23068, #15496, #4859, #2066, #33055, #9236, #1609, #25869, #44332, #1392, #44105, #37167, #19395, #43432, #33934, #33717, #12022, #16158, #40203, #29576, #26089, #11800, #8564, #26548, #22630, #5087, #5526, #5300, #12469, #23307, #30019, #39980, #15707, #33481, #2285, #12687, #19178, #8999, #29791, #26767, #40872, #1827, #8329, #15935, #22392, #26329, #37408, #5766, #43871, #12250, #40434, #19854, #36496, #18960, #8786, #41556, #30709, #9464, #44806, #24222, #6676, #20072, #27694, #38330, #42022, #34393, #16384, #13387, #10368, #34147, #24444, #20302, #12926, #31388, #20981, #38102, #34843, #13163, #30462, #16858, #45493, #17298, #20753, #38548, #44565, #6901, #27459, #41334, #41111, #27242, #2517, #3207, #9910, #31153, #27012, #13849, #23527, #35077, #27927, #37629, #10147, #5980, #23982, #16623, #9684, #23748, #37862, #6209, #2764, #13610, #30938, #45031, #6458, #20537, #34631, #2988, #17075, #45251, #41797, #42473, #32314, #35768, #885, #3684, #7149, #38793, #24674, #7375, #45722, #21677, #28150, #670, #14075, #21226, #32538, #32068, #39247, #39720, #7842, #14987, #35528, #17771, #29074, #10839, #24911, #35307, #43160, #42923, #28371, #11289, #440, #42702, #11527, #25610, #31837, #14772, #14542, #21917, #42242, #8070, #22132, #3449, #28620, #3903, #11066, #17546, #39025, #10599, #31619, #207, #25133, #17998, #14300, #28843, #21451, #36005, #7599, #25368, #4146, #18240, #4368, #18676, #8511, #32767, #12198, #11967, #1557, #12641, #4585, #36446, #39934, #25822, #11755, #40148, #1112, #4809, #43601, #22579, #5253, #26278, #36900, #8279, #33006, #12421, #40390, #36681, #5040, #16110, #29526, #26035, #19132, #22343, #2014, #29970, #15450, #29734, #33220, #15227, #8741, #15657, #43814, #22807, #19343, #33428, #1772, #30195, #43388, #18913, #36221, #15882, #44054, #40822, #26501, #29314, #1346, #40602, #8953, #26722, #23022, #37113, #5473, #19568, #33665, #44285, #9178, #16805, #2712, #37581, #16335, #44754, #41284, #23253, #30885, #5935, #13561, #24173, #17023, #9412, #44513, #41744, #26955, #3155, #9637, #19803, #38281, #27879, #44980, #10097, #20025, #37355, #41977, #27636, #34102, #6626, #2468, #41055, #16575, #5716, #13113, #20490, #23701, #23479, #45199, #13334, #38050, #33887, #20701, #2240, #17247, #27412, #30416, #34792, #37813, #34576, #6162, #2936, #23930, #41509, #12873, #9859, #20251, #34342, #6408, #31100, #31333, #45440, #13802, #17494, #18181, #24390, #14485, #24859, #28312, #42412, #11016, #28564, #31784, #35947, #31572, #24614, #10319, #28094, #154, #17720, #21402, #17942, #38976, #32010, #38733, #32484, #10782, #45672, #14025, #38494, #39423, #18404, #3400, #3851, #35476, #7094, #42188, #21175, #32257, #615, #10538, #21624, #14717, #4313, #7326, #35255, #3633, #28792, #14243, #834, #383, #6846, #25310, #14933, #42654, #42870, #25083, #20926, #39197, #7778, #11237, #21854, #29016, #35023, #7547, #35707, #4083, #40336, #11698, #15164, #19285, #36630, #12139, #39662, #26448, #8012, #22964, #12372, #37059, #36848, #4531, #40088, #40547, #25549, #8898, #1502, #22080, #33166, #36171, #8450, #8688, #15600, #15391, #11909, #18624, #29469, #32710, #19078, #18856, #22520, #19507, #11469, #33604, #1057, #43543, #25981, #4984, #29683, #43760, #29255, #22752, #43332, #25771, #5412, #26221, #5199, #1956, #1716, #16056, #33372, #39883, #43099, #8224, #22293, #36389, #4752, #32946, #1292, #15821, #29912, #43997, #2410, #44923, #20196, #30829, #33835, #26891, #6345, #6107, #34052, #44693, #10041, #23427, #2880, #40998, #2189, #41687, #23872, #9358, #23647, #37528, #44228, #34277, #13053, #16511, #30593, #13281, #2649, #5887, #24110, #37295, #44454, #30140, #16281, #19976, #34739, #27141, #23187, #12585, #41228, #9587, #6569, #37758, #19749, #30360, #26664, #13508, #38222, #5656, #16747, #27358, #12810, #41453, #9805, #37992, #40761, #20429, #34522, #16972, #31048, #45147, #27581, #20647, #3099, #9119, #42819, #21118, #13742, #32197, #21795, #38921, #35646, #31514, #31277, #17664, #21563, #45617, #4018, #28039, #34967, #13965, #45380, #42132, #14424, #10483, #3341, #39141, #10722, #31950, #27819, #559, #41916, #11180, #14662, #25250, #18119, #17434, #28503, #24557, #42601, #17883, #21344, #10260, #7273, #24337, #14186, #10962, #35420, #35202, #31727, #38441, #3578, #6792, #3793, #38673, #320, #25031, #39360, #94, #17190, #28254, #7714, #7032, #7491, #42353, #24802, #28738, #20869, #35888, #19022, #43710, #40037, #4262, #8845, #8631, #40277, #29855, #32435, #40493, #15336, #29191, #28961, #22913, #11857, #25930, #18354, #11641, #18794, #43941, #4924, #783, #22239, #8393, #14883, #22693, #1230, #1665, #43041, #15768, #26162, #11403, #25491, #15551, #1450, #26392, #39603, #22462, #36792, #39831, #22027, #5149, #12085, #36570, #43270, #33113, #7959, #36116, #4481, #36336, #25719, #4694, #29418, #29631, #19233, #18573, #33320, #32656, #998, #12317, #32885, #15101, #8174, #43490, #2823, #23368, #30297, #9746, #2131, #9059, #13227, #37004, #23812, #44168, #44864, #33994, #30529, #6279, #13450, #12531, #2585, #19917, #41398, #30085, #34461, #20367, #5358, #23126, #26826, #44392, #2346, #44628, #16446, #12993, #19687, #27080, #5832, #16915, #34212, #12747, #37922, #27517, #9527, #41173, #30994, #23591, #26605, #5596, #27304, #45092, #40705, #16688, #41619, #37696, #9975, #33780, #6046, #40933, #16220, #20135, #37230, #9299, #30773, #19452, #33546, #1896, #16003, #37470, #14361, #3962, #6513, #14609, #35137, #3274, #3045, #28681, #31670, #37, #42758, #31453, #38610, #18055, #24743, #20592, #42076, #14131, #28442, #10202, #21285, #34909, #35363, #38861, #28203, #34687, #42297, #17136, #21054, #3738, #10660, #10425, #6969, #31219, #24502, #45313, #7212, #45555, #17826, #31894, #21506, #24280, #27756, #13675, #41858, #27981, #38386, #6735, #13907, #3516, #265, #42541, #10905, #20810, #17366, #24971, #39084, #17600, #7433, #35585, #32137, #502, #24046, #38165, #23259, #5477, #36685, #5257, #19136, #25190, #15889, #26282, #29739, #43818, #12426, #29974, #33224, #37360, #26725, #5721, #40394, #12204, #19349, #16339, #5045, #4209, #11121, #1563, #15661, #33891, #8745, #732, #14829, #39303, #40826, #19808, #18301, #33432, #22812, #1777 ),
 .UNSPECIFIED., .F., .T. ) 
 B_SPLINE_CURVE_WITH_KNOTS ( ( 3, 2, 2, 2, 2, 2, 2, 2, 2, 2, 2, 2, 2, 2, 2, 2, 2, 2, 2, 2, 2, 2, 2, 2, 2, 2, 2, 2, 2, 2, 2, 2, 2, 2, 2, 2, 2, 2, 2, 2, 2, 2, 2, 2, 2, 2, 2, 2, 2, 2, 2, 2, 2, 2, 2, 2, 2, 2, 2, 2, 2, 2, 2, 2, 2, 2, 2, 2, 2, 2, 2, 2, 2, 2, 2, 2, 2, 2, 2, 2, 2, 2, 2, 2, 2, 2, 2, 2, 2, 2, 2, 2, 2, 2, 2, 2, 2, 2, 2, 2, 2, 2, 2, 2, 2, 2, 2, 2, 2, 2, 2, 2, 2, 2, 2, 2, 2, 2, 2, 2, 2, 2, 2, 2, 2, 2, 2, 2, 2, 2, 2, 2, 2, 2, 2, 2, 2, 2, 2, 2, 2, 2, 2, 2, 2, 2, 2, 2, 2, 2, 2, 2, 2, 2, 2, 2, 2, 2, 2, 2, 2, 2, 2, 2, 2, 2, 2, 2, 2, 2, 2, 2, 2, 2, 2, 2, 2, 2, 2, 2, 2, 2, 2, 2, 2, 2, 2, 2, 2, 2, 2, 2, 2, 2, 2, 2, 2, 2, 2, 2, 2, 2, 2, 2, 2, 2, 2, 2, 2, 2, 2, 2, 2, 2, 2, 2, 2, 2, 2, 2, 2, 2, 2, 2, 2, 2, 2, 2, 2, 2, 2, 2, 2, 2, 2, 2, 2, 2, 2, 2, 2, 2, 2, 2, 2, 2, 2, 2, 2, 2, 2, 2, 2, 2, 2, 2, 2, 2, 2, 2, 2, 2, 2, 2, 2, 2, 2, 2, 2, 2, 2, 2, 2, 2, 2, 2, 2, 2, 2, 2, 2, 2, 2, 2, 2, 2, 2, 2, 2, 2, 2, 2, 2, 2, 2, 2, 2, 2, 2, 2, 2, 2, 2, 2, 2, 2, 2, 2, 2, 2, 2, 2, 2, 2, 2, 2, 2, 2, 2, 2, 2, 2, 2, 2, 2, 2, 2, 2, 2, 2, 2, 2, 2, 2, 2, 2, 2, 2, 2, 2, 2, 2, 2, 2, 2, 2, 2, 2, 2, 2, 2, 2, 2, 2, 2, 2, 2, 2, 2, 2, 2, 2, 2, 2, 2, 2, 2, 2, 2, 2, 2, 2, 2, 2, 2, 2, 2, 2, 2, 2, 2, 2, 2, 2, 2, 2, 2, 2, 2, 2, 2, 2, 2, 2, 2, 2, 2, 2, 2, 2, 2, 2, 2, 2, 2, 2, 2, 2, 2, 2, 2, 2, 2, 2, 2, 2, 2, 2, 2, 2, 2, 2, 2, 2, 2, 2, 2, 2, 2, 2, 2, 3 ),
 ( 8.755858387967423303E-18, 0.002272727272727281290, 0.004545454545454553907, 0.006818181818181826524, 0.009090909090909099141, 0.01136363636363637263, 0.01363636363636364437, 0.01590909090909091786, 0.01818181818181819134, 0.02045454545454546483, 0.02272727272727273831, 0.02500000000000001180, 0.02727272727272728181, 0.02954545454545455530, 0.03181818181818182184, 0.03409090909090909532, 0.03636363636363636881, 0.03863636363636364229, 0.04090909090909091578, 0.04318181818181818926, 0.04545454545454546275, 0.04772727272727273623, 0.05000000000000000971, 0.05227272727272727626, 0.05454545454545454974, 0.05681818181818182323, 0.05909090909090909671, 0.06136363636363637020, 0.06363636363636364368, 0.06590909090909091717, 0.06818181818181819065, 0.07045454545454546413, 0.07272727272727273762, 0.07500000000000001110, 0.07727272727272728459, 0.07954545454545455807, 0.08181818181818183155, 0.08409090909090910504, 0.08636363636363637852, 0.08863636363636365201, 0.09090909090909092549, 0.09318181818181819898, 0.09545454545454547246, 0.09772727272727274594, 0.1000000000000000194, 0.1022727272727272929, 0.1045454545454545525, 0.1068181818181818260, 0.1090909090909090995, 0.1113636363636363730, 0.1136363636363636465, 0.1159090909090909199, 0.1181818181818181934, 0.1204545454545454669, 0.1227272727272727404, 0.1250000000000000000, 0.1272727272727272596, 0.1295454545454545470, 0.1318181818181818066, 0.1340909090909090939, 0.1363636363636363535, 0.1386363636363636409, 0.1409090909090909005, 0.1431818181818181879, 0.1454545454545454475, 0.1477272727272727348, 0.1499999999999999944, 0.1522727272727272818, 0.1545454545454545414, 0.1568181818181818288, 0.1590909090909090884, 0.1613636363636363757, 0.1636363636363636354, 0.1659090909090909227, 0.1681818181818181823, 0.1704545454545454419, 0.1727272727272727293, 0.1749999999999999889, 0.1772727272727272763, 0.1795454545454545359, 0.1818181818181818232, 0.1840909090909090828, 0.1863636363636363702, 0.1886363636363636298, 0.1909090909090909172, 0.1931818181818181768, 0.1954545454545454641, 0.1977272727272727237, 0.2000000000000000111, 0.2022727272727272707, 0.2045454545454545581, 0.2068181818181818177, 0.2090909090909090773, 0.2113636363636363646, 0.2136363636363636243, 0.2159090909090909116, 0.2181818181818181712, 0.2204545454545454586, 0.2227272727272727182, 0.2250000000000000056, 0.2272727272727272652, 0.2295454545454545525, 0.2318181818181818121, 0.2340909090909090995, 0.2363636363636363591, 0.2386363636363636465, 0.2409090909090909061, 0.2431818181818181934, 0.2454545454545454530, 0.2477272727272727404, 0.2500000000000000000, 0.2522727272727272596, 0.2545454545454545192, 0.2568181818181818343, 0.2590909090909090939, 0.2613636363636363535, 0.2636363636363636131, 0.2659090909090909283, 0.2681818181818181879, 0.2704545454545454475, 0.2727272727272727071, 0.2750000000000000222, 0.2772727272727272818, 0.2795454545454545414, 0.2818181818181818010, 0.2840909090909091161, 0.2863636363636363757, 0.2886363636363636354, 0.2909090909090908950, 0.2931818181818181546, 0.2954545454545454697, 0.2977272727272727293, 0.2999999999999999889, 0.3022727272727272485, 0.3045454545454545636, 0.3068181818181818232, 0.3090909090909090828, 0.3113636363636363424, 0.3136363636363636576, 0.3159090909090909172, 0.3181818181818181768, 0.3204545454545454364, 0.3227272727272727515, 0.3250000000000000111, 0.3272727272727272707, 0.3295454545454545303, 0.3318181818181818454, 0.3340909090909091050, 0.3363636363636363646, 0.3386363636363636243, 0.3409090909090908839, 0.3431818181818181990, 0.3454545454545454586, 0.3477272727272727182, 0.3499999999999999778, 0.3522727272727272929, 0.3545454545454545525, 0.3568181818181818121, 0.3590909090909090717, 0.3613636363636363869, 0.3636363636363636465, 0.3659090909090909061, 0.3681818181818181657, 0.3704545454545454808, 0.3727272727272727404, 0.3749999999999999445, 0.3772727272727272596, 0.3795454545454545192, 0.3818181818181818343, 0.3840909090909090939, 0.3863636363636363535, 0.3886363636363636131, 0.3909090909090909283, 0.3931818181818181879, 0.3954545454545454475, 0.3977272727272727071, 0.4000000000000000222, 0.4022727272727272818, 0.4045454545454545414, 0.4068181818181818010, 0.4090909090909091161, 0.4113636363636363757, 0.4136363636363636354, 0.4159090909090908950, 0.4181818181818181546, 0.4204545454545454697, 0.4227272727272727293, 0.4249999999999999889, 0.4272727272727272485, 0.4295454545454545636, 0.4318181818181818232, 0.4340909090909090828, 0.4363636363636363424, 0.4386363636363636576, 0.4409090909090909172, 0.4431818181818181768, 0.4454545454545454364, 0.4477272727272727515, 0.4500000000000000111, 0.4522727272727272707, 0.4545454545454545303, 0.4568181818181818454, 0.4590909090909091050, 0.4613636363636363646, 0.4636363636363636243, 0.4659090909090908839, 0.4681818181818181990, 0.4704545454545454586, 0.4727272727272727182, 0.4749999999999999778, 0.4772727272727272929, 0.4795454545454545525, 0.4818181818181818121, 0.4840909090909090717, 0.4863636363636363869, 0.4886363636363636465, 0.4909090909090909061, 0.4931818181818181657, 0.4954545454545454808, 0.4977272727272727404, 0.5000000000000000000, 0.5022727272727273151, 0.5045454545454545192, 0.5068181818181818343, 0.5090909090909090384, 0.5113636363636363535, 0.5136363636363636687, 0.5159090909090908728, 0.5181818181818181879, 0.5204545454545455030, 0.5227272727272727071, 0.5250000000000000222, 0.5272727272727272263, 0.5295454545454545414, 0.5318181818181818565, 0.5340909090909090606, 0.5363636363636363757, 0.5386363636363636909, 0.5409090909090908950, 0.5431818181818182101, 0.5454545454545454142, 0.5477272727272727293, 0.5500000000000000444, 0.5522727272727272485, 0.5545454545454545636, 0.5568181818181817677, 0.5590909090909090828, 0.5613636363636363980, 0.5636363636363636020, 0.5659090909090909172, 0.5681818181818182323, 0.5704545454545454364, 0.5727272727272727515, 0.5749999999999999556, 0.5772727272727272707, 0.5795454545454545858, 0.5818181818181817899, 0.5840909090909091050, 0.5863636363636363091, 0.5886363636363636243, 0.5909090909090909394, 0.5931818181818181435, 0.5954545454545454586, 0.5977272727272727737, 0.5999999999999999778, 0.6022727272727272929, 0.6045454545454544970, 0.6068181818181818121, 0.6090909090909091272, 0.6113636363636362203, 0.6136363636363636465, 0.6159090909090909616, 0.6181818181818181657, 0.6204545454545454808, 0.6227272727272726849, 0.6250000000000000000, 0.6272727272727273151, 0.6295454545454546302, 0.6318181818181818343, 0.6340909090909090384, 0.6363636363636363535, 0.6386363636363636687, 0.6409090909090908728, 0.6431818181818181879, 0.6454545454545455030, 0.6477272727272727071, 0.6500000000000000222, 0.6522727272727272263, 0.6545454545454545414, 0.6568181818181818565, 0.6590909090909090606, 0.6613636363636363757, 0.6636363636363636909, 0.6659090909090908950, 0.6681818181818182101, 0.6704545454545454142, 0.6727272727272727293, 0.6750000000000000444, 0.6772727272727272485, 0.6795454545454545636, 0.6818181818181817677, 0.6840909090909090828, 0.6863636363636363980, 0.6886363636363636020, 0.6909090909090909172, 0.6931818181818182323, 0.6954545454545454364, 0.6977272727272727515, 0.6999999999999999556, 0.7022727272727272707, 0.7045454545454545858, 0.7068181818181817899, 0.7090909090909091050, 0.7113636363636363091, 0.7136363636363636243, 0.7159090909090909394, 0.7181818181818181435, 0.7204545454545454586, 0.7227272727272727737, 0.7249999999999999778, 0.7272727272727272929, 0.7295454545454544970, 0.7318181818181818121, 0.7340909090909091272, 0.7363636363636363313, 0.7386363636363636465, 0.7409090909090909616, 0.7431818181818181657, 0.7454545454545454808, 0.7477272727272726849, 0.7499999999999998890, 0.7522727272727273151, 0.7545454545454545192, 0.7568181818181818343, 0.7590909090909090384, 0.7613636363636363535, 0.7636363636363636687, 0.7659090909090908728, 0.7681818181818181879, 0.7704545454545455030, 0.7727272727272727071, 0.7750000000000000222, 0.7772727272727272263, 0.7795454545454545414, 0.7818181818181818565, 0.7840909090909090606, 0.7863636363636363757, 0.7886363636363636909, 0.7909090909090908950, 0.7931818181818182101, 0.7954545454545454142, 0.7977272727272727293, 0.8000000000000000444, 0.8022727272727272485, 0.8045454545454545636, 0.8068181818181817677, 0.8090909090909090828, 0.8113636363636363980, 0.8136363636363636020, 0.8159090909090909172, 0.8181818181818182323, 0.8204545454545454364, 0.8227272727272727515, 0.8249999999999999556, 0.8272727272727272707, 0.8295454545454545858, 0.8318181818181817899, 0.8340909090909091050, 0.8363636363636363091, 0.8386363636363636243, 0.8409090909090909394, 0.8431818181818181435, 0.8454545454545454586, 0.8477272727272727737, 0.8499999999999999778, 0.8522727272727272929, 0.8545454545454544970, 0.8568181818181818121, 0.8590909090909091272, 0.8613636363636363313, 0.8636363636363636465, 0.8659090909090909616, 0.8681818181818181657, 0.8704545454545453698, 0.8727272727272726849, 0.8750000000000000000, 0.8772727272727273151, 0.8795454545454545192, 0.8818181818181818343, 0.8840909090909090384, 0.8863636363636363535, 0.8886363636363637797, 0.8909090909090908728, 0.8931818181818181879, 0.8954545454545455030, 0.8977272727272727071, 0.9000000000000000222, 0.9022727272727272263, 0.9045454545454545414, 0.9068181818181818565, 0.9090909090909090606, 0.9113636363636363757, 0.9136363636363636909, 0.9159090909090908950, 0.9181818181818182101, 0.9204545454545454142, 0.9227272727272727293, 0.9250000000000000444, 0.9272727272727272485, 0.9295454545454545636, 0.9318181818181817677, 0.9340909090909090828, 0.9363636363636363980, 0.9386363636363636020, 0.9409090909090909172, 0.9431818181818182323, 0.9454545454545454364, 0.9477272727272727515, 0.9499999999999999556, 0.9522727272727272707, 0.9545454545454545858, 0.9568181818181817899, 0.9590909090909091050, 0.9613636363636363091, 0.9636363636363636243, 0.9659090909090909394, 0.9681818181818181435, 0.9704545454545454586, 0.9727272727272727737, 0.9749999999999999778, 0.9772727272727272929, 0.9781254700864302487 ),
 .UNSPECIFIED. ) 
 CURVE ( )  GEOMETRIC_REPRESENTATION_ITEM ( )  RATIONAL_B_SPLINE_CURVE ( ( 1.000000000000000000, 0.9898214418809326842, 1.000000000000000000, 0.9898214418809326842, 1.000000000000000000, 0.9898214418809326842, 1.000000000000000000, 0.9898214418809326842, 1.000000000000000000, 0.9898214418809326842, 1.000000000000000000, 0.9898214418809326842, 1.000000000000000000, 0.9898214418809326842, 1.000000000000000000, 0.9898214418809326842, 1.000000000000000000, 0.9898214418809326842, 1.000000000000000000, 0.9898214418809326842, 1.000000000000000000, 0.9898214418809326842, 1.000000000000000000, 0.9898214418809326842, 1.000000000000000000, 0.9898214418809326842, 1.000000000000000000, 0.9898214418809326842, 1.000000000000000000, 0.9898214418809326842, 1.000000000000000000, 0.9898214418809326842, 1.000000000000000000, 0.9898214418809326842, 1.000000000000000000, 0.9898214418809326842, 1.000000000000000000, 0.9898214418809326842, 1.000000000000000000, 0.9898214418809326842, 1.000000000000000000, 0.9898214418809326842, 1.000000000000000000, 0.9898214418809326842, 1.000000000000000000, 0.9898214418809326842, 1.000000000000000000, 0.9898214418809326842, 1.000000000000000000, 0.9898214418809326842, 1.000000000000000000, 0.9898214418809326842, 1.000000000000000000, 0.9898214418809326842, 1.000000000000000000, 0.9898214418809326842, 1.000000000000000000, 0.9898214418809326842, 1.000000000000000000, 0.9898214418809326842, 1.000000000000000000, 0.9898214418809326842, 1.000000000000000000, 0.9898214418809326842, 1.000000000000000000, 0.9898214418809326842, 1.000000000000000000, 0.9898214418809326842, 1.000000000000000000, 0.9898214418809326842, 1.000000000000000000, 0.9898214418809326842, 1.000000000000000000, 0.9898214418809326842, 1.000000000000000000, 0.9898214418809326842, 1.000000000000000000, 0.9898214418809326842, 1.000000000000000000, 0.9898214418809326842, 1.000000000000000000, 0.9898214418809326842, 1.000000000000000000, 0.9898214418809326842, 1.000000000000000000, 0.9898214418809326842, 1.000000000000000000, 0.9898214418809326842, 1.000000000000000000, 0.9898214418809326842, 1.000000000000000000, 0.9898214418809326842, 1.000000000000000000, 0.9898214418809326842, 1.000000000000000000, 0.9898214418809326842, 1.000000000000000000, 0.9898214418809326842, 1.000000000000000000, 0.9898214418809326842, 1.000000000000000000, 0.9898214418809326842, 1.000000000000000000, 0.9898214418809326842, 1.000000000000000000, 0.9898214418809326842, 1.000000000000000000, 0.9898214418809326842, 1.000000000000000000, 0.9898214418809326842, 1.000000000000000000, 0.9898214418809326842, 1.000000000000000000, 0.9898214418809326842, 1.000000000000000000, 0.9898214418809326842, 1.000000000000000000, 0.9898214418809326842, 1.000000000000000000, 0.9898214418809326842, 1.000000000000000000, 0.9898214418809326842, 1.000000000000000000, 0.9898214418809326842, 1.000000000000000000, 0.9898214418809326842, 1.000000000000000000, 0.9898214418809326842, 1.000000000000000000, 0.9898214418809326842, 1.000000000000000000, 0.9898214418809326842, 1.000000000000000000, 0.9898214418809326842, 1.000000000000000000, 0.9898214418809326842, 1.000000000000000000, 0.9898214418809326842, 1.000000000000000000, 0.9898214418809326842, 1.000000000000000000, 0.9898214418809326842, 1.000000000000000000, 0.9898214418809326842, 1.000000000000000000, 0.9898214418809326842, 1.000000000000000000, 0.9898214418809326842, 1.000000000000000000, 0.9898214418809326842, 1.000000000000000000, 0.9898214418809326842, 1.000000000000000000, 0.9898214418809326842, 1.000000000000000000, 0.9898214418809326842, 1.000000000000000000, 0.9898214418809326842, 1.000000000000000000, 0.9898214418809326842, 1.000000000000000000, 0.9898214418809326842, 1.000000000000000000, 0.9898214418809326842, 1.000000000000000000, 0.9898214418809326842, 1.000000000000000000, 0.9898214418809326842, 1.000000000000000000, 0.9898214418809326842, 1.000000000000000000, 0.9898214418809326842, 1.000000000000000000, 0.9898214418809326842, 1.000000000000000000, 0.9898214418809326842, 1.000000000000000000, 0.9898214418809326842, 1.000000000000000000, 0.9898214418809326842, 1.000000000000000000, 0.9898214418809326842, 1.000000000000000000, 0.9898214418809326842, 1.000000000000000000, 0.9898214418809326842, 1.000000000000000000, 0.9898214418809326842, 1.000000000000000000, 0.9898214418809326842, 1.000000000000000000, 0.9898214418809326842, 1.000000000000000000, 0.9898214418809326842, 1.000000000000000000, 0.9898214418809326842, 1.000000000000000000, 0.9898214418809326842, 1.000000000000000000, 0.9898214418809326842, 1.000000000000000000, 0.9898214418809326842, 1.000000000000000000, 0.9898214418809326842, 1.000000000000000000, 0.9898214418809326842, 1.000000000000000000, 0.9898214418809326842, 1.000000000000000000, 0.9898214418809326842, 1.000000000000000000, 0.9898214418809326842, 1.000000000000000000, 0.9898214418809326842, 1.000000000000000000, 0.9898214418809326842, 1.000000000000000000, 0.9898214418809326842, 1.000000000000000000, 0.9898214418809326842, 1.000000000000000000, 0.9898214418809326842, 1.000000000000000000, 0.9898214418809326842, 1.000000000000000000, 0.9898214418809326842, 1.000000000000000000, 0.9898214418809326842, 1.000000000000000000, 0.9898214418809326842, 1.000000000000000000, 0.9898214418809326842, 1.000000000000000000, 0.9898214418809326842, 1.000000000000000000, 0.9898214418809326842, 1.000000000000000000, 0.9898214418809326842, 1.000000000000000000, 0.9898214418809326842, 1.000000000000000000, 0.9898214418809326842, 1.000000000000000000, 0.9898214418809326842, 1.000000000000000000, 0.9898214418809326842, 1.000000000000000000, 0.9898214418809326842, 1.000000000000000000, 0.9898214418809326842, 1.000000000000000000, 0.9898214418809326842, 1.000000000000000000, 0.9898214418809326842, 1.000000000000000000, 0.9898214418809326842, 1.000000000000000000, 0.9898214418809326842, 1.000000000000000000, 0.9898214418809326842, 1.000000000000000000, 0.9898214418809326842, 1.000000000000000000, 0.9898214418809326842, 1.000000000000000000, 0.9898214418809326842, 1.000000000000000000, 0.9898214418809326842, 1.000000000000000000, 0.9898214418809326842, 1.000000000000000000, 0.9898214418809326842, 1.000000000000000000, 0.9898214418809326842, 1.000000000000000000, 0.9898214418809326842, 1.000000000000000000, 0.9898214418809326842, 1.000000000000000000, 0.9898214418809326842, 1.000000000000000000, 0.9898214418809326842, 1.000000000000000000, 0.9898214418809326842, 1.000000000000000000, 0.9898214418809326842, 1.000000000000000000, 0.9898214418809326842, 1.000000000000000000, 0.9898214418809326842, 1.000000000000000000, 0.9898214418809326842, 1.000000000000000000, 0.9898214418809326842, 1.000000000000000000, 0.9898214418809326842, 1.000000000000000000, 0.9898214418809326842, 1.000000000000000000, 0.9898214418809326842, 1.000000000000000000, 0.9898214418809326842, 1.000000000000000000, 0.9898214418809326842, 1.000000000000000000, 0.9898214418809326842, 1.000000000000000000, 0.9898214418809326842, 1.000000000000000000, 0.9898214418809326842, 1.000000000000000000, 0.9898214418809326842, 1.000000000000000000, 0.9898214418809326842, 1.000000000000000000, 0.9898214418809326842, 1.000000000000000000, 0.9898214418809326842, 1.000000000000000000, 0.9898214418809326842, 1.000000000000000000, 0.9898214418809326842, 1.000000000000000000, 0.9898214418809326842, 1.000000000000000000, 0.9898214418809326842, 1.000000000000000000, 0.9898214418809326842, 1.000000000000000000, 0.9898214418809326842, 1.000000000000000000, 0.9898214418809326842, 1.000000000000000000, 0.9898214418809326842, 1.000000000000000000, 0.9898214418809326842, 1.000000000000000000, 0.9898214418809326842, 1.000000000000000000, 0.9898214418809326842, 1.000000000000000000, 0.9898214418809326842, 1.000000000000000000, 0.9898214418809326842, 1.000000000000000000, 0.9898214418809326842, 1.000000000000000000, 0.9898214418809326842, 1.000000000000000000, 0.9898214418809326842, 1.000000000000000000, 0.9898214418809326842, 1.000000000000000000, 0.9898214418809326842, 1.000000000000000000, 0.9898214418809326842, 1.000000000000000000, 0.9898214418809326842, 1.000000000000000000, 0.9898214418809326842, 1.000000000000000000, 0.9898214418809326842, 1.000000000000000000, 0.9898214418809326842, 1.000000000000000000, 0.9898214418809326842, 1.000000000000000000, 0.9898214418809326842, 1.000000000000000000, 0.9898214418809326842, 1.000000000000000000, 0.9898214418809326842, 1.000000000000000000, 0.9898214418809326842, 1.000000000000000000, 0.9898214418809326842, 1.000000000000000000, 0.9898214418809326842, 1.000000000000000000, 0.9898214418809326842, 1.000000000000000000, 0.9898214418809326842, 1.000000000000000000, 0.9898214418809326842, 1.000000000000000000, 0.9898214418809326842, 1.000000000000000000, 0.9898214418809326842, 1.000000000000000000, 0.9898214418809326842, 1.000000000000000000, 0.9898214418809326842, 1.000000000000000000, 0.9898214418809326842, 1.000000000000000000, 0.9898214418809326842, 1.000000000000000000, 0.9898214418809326842, 1.000000000000000000, 0.9898214418809326842, 1.000000000000000000, 0.9898214418809326842, 1.000000000000000000, 0.9898214418809326842, 1.000000000000000000, 0.9898214418809326842, 1.000000000000000000, 0.9898214418809326842, 1.000000000000000000, 0.9898214418809326842, 1.000000000000000000, 0.9898214418809326842, 1.000000000000000000, 0.9898214418809326842, 1.000000000000000000, 0.9898214418809326842, 1.000000000000000000, 0.9898214418809326842, 1.000000000000000000, 0.9898214418809326842, 1.000000000000000000, 0.9898214418809326842, 1.000000000000000000, 0.9898214418809326842, 1.000000000000000000, 0.9898214418809326842, 1.000000000000000000, 0.9898214418809326842, 1.000000000000000000, 0.9898214418809326842, 1.000000000000000000, 0.9898214418809326842, 1.000000000000000000, 0.9898214418809326842, 1.000000000000000000, 0.9898214418809326842, 1.000000000000000000, 0.9898214418809326842, 1.000000000000000000, 0.9898214418809326842, 1.000000000000000000, 0.9898214418809326842, 1.000000000000000000, 0.9898214418809326842, 1.000000000000000000, 0.9898214418809326842, 1.000000000000000000, 0.9898214418809326842, 1.000000000000000000, 0.9898214418809326842, 1.000000000000000000, 0.9898214418809326842, 1.000000000000000000, 0.9898214418809326842, 1.000000000000000000, 0.9898214418809326842, 1.000000000000000000, 0.9898214418809326842, 1.000000000000000000, 0.9898214418809326842, 1.000000000000000000, 0.9898214418809326842, 1.000000000000000000, 0.9898214418809326842, 1.000000000000000000, 0.9898214418809326842, 1.000000000000000000, 0.9898214418809326842, 1.000000000000000000, 0.9898214418809326842, 1.000000000000000000, 0.9898214418809326842, 1.000000000000000000, 0.9898214418809326842, 1.000000000000000000, 0.9898214418809326842, 1.000000000000000000, 0.9898214418809326842, 1.000000000000000000, 0.9898214418809326842, 1.000000000000000000, 0.9898214418809326842, 1.000000000000000000, 0.9898214418809326842, 1.000000000000000000, 0.9898214418809326842, 1.000000000000000000, 0.9898214418809326842, 1.000000000000000000, 0.9898214418809326842, 1.000000000000000000, 0.9898214418809326842, 1.000000000000000000, 0.9898214418809326842, 1.000000000000000000, 0.9898214418809326842, 1.000000000000000000, 0.9898214418809326842, 1.000000000000000000, 0.9898214418809326842, 1.000000000000000000, 0.9898214418809326842, 1.000000000000000000, 0.9898214418809326842, 1.000000000000000000, 0.9898214418809326842, 1.000000000000000000, 0.9898214418809326842, 1.000000000000000000, 0.9898214418809326842, 1.000000000000000000, 0.9898214418809326842, 1.000000000000000000, 0.9898214418809326842, 1.000000000000000000, 0.9898214418809326842, 1.000000000000000000, 0.9898214418809326842, 1.000000000000000000, 0.9898214418809326842, 1.000000000000000000, 0.9898214418809326842, 1.000000000000000000, 0.9898214418809326842, 1.000000000000000000, 0.9898214418809326842, 1.000000000000000000, 0.9898214418809326842, 1.000000000000000000, 0.9898214418809326842, 1.000000000000000000, 0.9898214418809326842, 1.000000000000000000, 0.9898214418809326842, 1.000000000000000000, 0.9898214418809326842, 1.000000000000000000, 0.9898214418809326842, 1.000000000000000000, 0.9898214418809326842, 1.000000000000000000, 0.9898214418809326842, 1.000000000000000000, 0.9898214418809326842, 1.000000000000000000, 0.9898214418809326842, 1.000000000000000000, 0.9898214418809326842, 1.000000000000000000, 0.9898214418809326842, 1.000000000000000000, 0.9898214418809326842, 1.000000000000000000, 0.9898214418809326842, 1.000000000000000000, 0.9898214418809326842, 1.000000000000000000, 0.9898214418809326842, 1.000000000000000000, 0.9898214418809326842, 1.000000000000000000, 0.9898214418809326842, 1.000000000000000000, 0.9898214418809326842, 1.000000000000000000, 0.9898214418809326842, 1.000000000000000000, 0.9898214418809326842, 1.000000000000000000, 0.9898214418809326842, 1.000000000000000000, 0.9898214418809326842, 1.000000000000000000, 0.9898214418809326842, 1.000000000000000000, 0.9898214418809326842, 1.000000000000000000, 0.9898214418809326842, 1.000000000000000000, 0.9898214418809326842, 1.000000000000000000, 0.9898214418809326842, 1.000000000000000000, 0.9898214418809326842, 1.000000000000000000, 0.9898214418809326842, 1.000000000000000000, 0.9898214418809326842, 1.000000000000000000, 0.9898214418809326842, 1.000000000000000000, 0.9898214418809326842, 1.000000000000000000, 0.9898214418809326842, 1.000000000000000000, 0.9898214418809326842, 1.000000000000000000, 0.9898214418809326842, 1.000000000000000000, 0.9898214418809326842, 1.000000000000000000, 0.9898214418809326842, 1.000000000000000000, 0.9898214418809326842, 1.000000000000000000, 0.9898214418809326842, 1.000000000000000000, 0.9898214418809326842, 1.000000000000000000, 0.9898214418809326842, 1.000000000000000000, 0.9898214418809326842, 1.000000000000000000, 0.9898214418809326842, 1.000000000000000000, 0.9898214418809326842, 1.000000000000000000, 0.9898214418809326842, 1.000000000000000000, 0.9898214418809326842, 1.000000000000000000, 0.9898214418809326842, 1.000000000000000000, 0.9898214418809326842, 1.000000000000000000, 0.9898214418809326842, 1.000000000000000000, 0.9898214418809326842, 1.000000000000000000, 0.9898214418809326842, 1.000000000000000000, 0.9898214418809326842, 1.000000000000000000, 0.9898214418809326842, 1.000000000000000000, 0.9898214418809326842, 1.000000000000000000, 0.9898214418809326842, 1.000000000000000000, 0.9898214418809326842, 1.000000000000000000, 0.9898214418809326842, 1.000000000000000000, 0.9898214418809326842, 1.000000000000000000, 0.9898214418809326842, 1.000000000000000000, 0.9898214418809326842, 1.000000000000000000, 0.9898214418809326842, 1.000000000000000000, 0.9898214418809326842, 1.000000000000000000, 0.9898214418809326842, 1.000000000000000000, 0.9898214418809326842, 1.000000000000000000, 0.9898214418809326842, 1.000000000000000000, 0.9898214418809326842, 1.000000000000000000, 0.9898214418809326842, 1.000000000000000000, 0.9898214418809326842, 1.000000000000000000, 0.9898214418809326842, 1.000000000000000000, 0.9898214418809326842, 1.000000000000000000, 0.9898214418809326842, 1.000000000000000000, 0.9898214418809326842, 1.000000000000000000, 0.9898214418809326842, 1.000000000000000000, 0.9898214418809326842, 1.000000000000000000, 0.9898214418809326842, 1.000000000000000000, 0.9898214418809326842, 1.000000000000000000, 0.9898214418809326842, 1.000000000000000000, 0.9898214418809326842, 1.000000000000000000, 0.9898214418809326842, 1.000000000000000000, 0.9898214418809326842, 1.000000000000000000, 0.9898214418809326842, 1.000000000000000000, 0.9898214418809326842, 1.000000000000000000, 0.9898214418809326842, 1.000000000000000000, 0.9898214418809326842, 1.000000000000000000, 0.9898214418809326842, 1.000000000000000000, 0.9898214418809326842, 1.000000000000000000, 0.9898214418809326842, 1.000000000000000000, 0.9898214418809326842, 1.000000000000000000, 0.9898214418809326842, 1.000000000000000000, 0.9898214418809326842, 1.000000000000000000, 0.9898214418809326842, 1.000000000000000000, 0.9898214418809326842, 1.000000000000000000, 0.9898214418809326842, 1.000000000000000000, 0.9898214418809326842, 1.000000000000000000, 0.9898214418809326842, 1.000000000000000000, 0.9898214418809326842, 1.000000000000000000, 0.9898214418809326842, 1.000000000000000000, 0.9898214418809326842, 1.000000000000000000, 0.9898214418809326842, 1.000000000000000000, 0.9898214418809326842, 1.000000000000000000, 0.9898214418809326842, 1.000000000000000000, 0.9898214418809326842, 1.000000000000000000, 0.9898214418809326842, 1.000000000000000000, 0.9898214418809326842, 1.000000000000000000, 0.9898214418809326842, 1.000000000000000000, 0.9898214418809326842, 1.000000000000000000, 0.9898214418809326842, 1.000000000000000000, 0.9898214418809326842, 1.000000000000000000, 0.9898214418809326842, 1.000000000000000000, 0.9898214418809326842, 1.000000000000000000, 0.9898214418809326842, 1.000000000000000000, 0.9898214418809326842, 1.000000000000000000, 0.9898214418809326842, 1.000000000000000000, 0.9898214418809326842, 1.000000000000000000, 0.9898214418809326842, 1.000000000000000000, 0.9898214418809326842, 1.000000000000000000, 0.9898214418809326842, 1.000000000000000000, 0.9898214418809326842, 1.000000000000000000, 0.9898214418809326842, 1.000000000000000000, 0.9898214418809326842, 1.000000000000000000, 0.9898214418809326842, 1.000000000000000000, 0.9898214418809326842, 1.000000000000000000, 0.9898214418809326842, 1.000000000000000000, 0.9898214418809326842, 1.000000000000000000, 0.9898214418809326842, 1.000000000000000000, 0.9898214418809326842, 1.000000000000000000, 0.9898214418809326842, 1.000000000000000000, 0.9898214418809326842, 1.000000000000000000, 0.9898214418809326842, 1.000000000000000000, 0.9898214418809326842, 1.000000000000000000, 0.9898214418809326842, 1.000000000000000000, 0.9898214418809326842, 1.000000000000000000, 0.9898214418809326842, 1.000000000000000000, 0.9898214418809326842, 1.000000000000000000, 0.9898214418809326842, 1.000000000000000000, 0.9898214418809326842, 1.000000000000000000, 0.9898214418809326842, 1.000000000000000000, 0.9898214418809326842, 1.000000000000000000, 0.9898214418809326842, 1.000000000000000000, 0.9898214418809326842, 1.000000000000000000, 0.9898214418809326842, 1.000000000000000000, 0.9898214418809326842, 1.000000000000000000, 0.9898214418809326842, 1.000000000000000000, 0.9898214418809326842, 1.000000000000000000, 0.9898214418809326842, 1.000000000000000000, 0.9898214418809326842, 1.000000000000000000, 0.9898214418809326842, 1.000000000000000000, 0.9898214418809326842, 1.000000000000000000, 0.9898214418809326842, 1.000000000000000000, 0.9898214418809326842, 1.000000000000000000, 0.9898214418809326842, 1.000000000000000000, 0.9898214418809326842, 1.000000000000000000, 0.9898214418809326842, 1.000000000000000000, 0.9898214418809326842, 1.000000000000000000, 0.9898214418809326842, 1.000000000000000000, 0.9898214418809326842, 1.000000000000000000, 0.9898214418809326842, 1.000000000000000000, 0.9898214418809326842, 1.000000000000000000, 0.9898214418809326842, 1.000000000000000000, 0.9898214418809326842, 1.000000000000000000, 0.9898214418809326842, 1.000000000000000000, 0.9898214418809326842, 1.000000000000000000, 0.9898214418809326842, 1.000000000000000000, 0.9898214418809326842, 1.000000000000000000, 0.9898214418809326842, 1.000000000000000000, 0.9898214418809326842, 1.000000000000000000, 0.9961809353924466759, 0.9952277490961531914 ) ) 
 REPRESENTATION_ITEM ( '' )  );
#13500=CARTESIAN_POINT ( 'NONE',  ( 797.8594530101009923, 10.45630643248851044, -322.1405469898982119 ) ) ;
#13501=CARTESIAN_POINT ( 'NONE',  ( 757.0176451133909268, -85.09997266333499510, -349.9200121543848354 ) ) ;
#13507=CARTESIAN_POINT ( 'NONE',  ( 746.7653713866222915, 6.739858255585061464, -351.0478386215610271 ) ) ;
#13508=CARTESIAN_POINT ( 'NONE',  ( 796.7737145352015204, -284.6346026584196807, -370.7187646348536987 ) ) ;
#13511=CARTESIAN_POINT ( 'NONE',  ( 778.1981804954714335, -82.27096629478388934, -314.8072714833589885 ) ) ;
#13514=CARTESIAN_POINT ( 'NONE',  ( 814.8230680027162407, -173.8055962898689302, -333.7305795820267917 ) ) ;
#13516=CARTESIAN_POINT ( 'NONE',  ( 796.9462024416508257, -420.4527844766009252, -308.9653473494370246 ) ) ;
#13520=CARTESIAN_POINT ( 'NONE',  ( 778.1981804954714335, -442.2709662947826814, -314.8072714833589885 ) ) ;
#13521=DIRECTION ( 'NONE',  ( 1.000000000000000000, 0.000000000000000000, 0.000000000000000000 ) ) ;
#13526=CARTESIAN_POINT ( 'NONE',  ( 770.0799878456142551, -253.9874144716868329, -362.9823548866085616 ) ) ;
#13528=CARTESIAN_POINT ( 'NONE',  ( 754.0944755984390895, -255.6237781080504874, -364.1009440267246760 ) ) ;
#13533=CARTESIAN_POINT ( 'NONE',  ( 774.6312213355099630, -167.3618753856927412, -364.6798772138717482 ) ) ;
#13535=CARTESIAN_POINT ( 'NONE',  ( 782.5225473063381969, -118.2709662947837899, -375.2698199232970637 ) ) ;
#13537=CARTESIAN_POINT ( 'NONE',  ( 781.8018195045267476, -94.27096629478387513, -365.1927285166407273 ) ) ;
#13539=CARTESIAN_POINT ( 'NONE',  ( 798.5707757039680246, -29.46360902697153250, -356.7845633553585003 ) ) ;
#13541=CARTESIAN_POINT ( 'NONE',  ( 776.9254006560222479, -356.1908817542432075, -314.8983024940802125 ) ) ;
#13548=CARTESIAN_POINT ( 'NONE',  ( 793.0897708529556667, -342.5545181178796952, -361.3366627262616362 ) ) ;
#13549=CARTESIAN_POINT ( 'NONE',  ( 797.8594530101008786, -373.5436935675101040, -322.1405469898980982 ) ) ;
#13550=CARTESIAN_POINT ( 'NONE',  ( 778.7629533639073998, -128.7363362996984790, -375.0009284576466371 ) ) ;
#13555=CARTESIAN_POINT ( 'NONE',  ( 756.1348686366196716, -305.2601417444139429, -347.5531968255698416 ) ) ;
#13556=CARTESIAN_POINT ( 'NONE',  ( 786.2694204179717872, -165.2817908451529547, -305.1769319972829067 ) ) ;
#13561=CARTESIAN_POINT ( 'NONE',  ( 814.2001403089898304, -161.3618753856927697, -347.4397851343538264 ) ) ;
#13564=CARTESIAN_POINT ( 'NONE',  ( 814.9108240113580450, -304.2709662947832499, -337.5031285880265273 ) ) ;
#13571=CARTESIAN_POINT ( 'NONE',  ( 811.6461892240364477, -364.7146871989592114, -324.1737431748509835 ) ) ;
#13572=CARTESIAN_POINT ( 'NONE',  ( 749.2812353651451076, -126.4527844766019626, -323.2262854647983090 ) ) ;
#13574=CARTESIAN_POINT ( 'NONE',  ( 808.3070685750230950, -402.9982390220555430, -361.1904061080339261 ) ) ;
#13575=FACE_OUTER_BOUND ( 'NONE', #22685, .T. ) ;
#13578=CARTESIAN_POINT ( 'NONE',  ( 815.0009284576459549, -150.3510508353235480, -338.7629533639073429 ) ) ;
#13585=CARTESIAN_POINT ( 'NONE',  ( 763.0537975583475827, -0.4527844766023628176, -371.0346526505627480 ) ) ;
#13589=CARTESIAN_POINT ( 'NONE',  ( 812.3518521366052028, -409.0999726633340288, -326.5853460496235243 ) ) ;
#13591=CARTESIAN_POINT ( 'NONE',  ( 765.0180583372156207, -264.9982390220561115, -360.0135310231089534 ) ) ;
#13594=CARTESIAN_POINT ( 'NONE',  ( 801.5560724626406000, -264.5545181178798657, -326.7756240680316182 ) ) ;
#13595=CARTESIAN_POINT ( 'NONE',  ( 759.9864689768902508, -242.0891481129652618, -354.9819416627836404 ) ) ;
#13596=CARTESIAN_POINT ( 'NONE',  ( 797.6776695296629214, -403.5436935675101608, -357.6776695296636603 ) ) ;
#13597=CARTESIAN_POINT ( 'NONE',  ( 794.9819416627830151, -84.99823902205663728, -319.9864689768909898 ) ) ;
#13603=CARTESIAN_POINT ( 'NONE',  ( 788.6739635108323228, -55.64542720878963422, -373.9316612368139090 ) ) ;
#13609=CARTESIAN_POINT ( 'NONE',  ( 798.5707757039680246, -29.46360902697153250, -356.7845633553585003 ) ) ;
#13610=CARTESIAN_POINT ( 'NONE',  ( 777.4774526936600978, -82.27096629478390355, -304.7301800767028226 ) ) ;
#13612=CARTESIAN_POINT ( 'NONE',  ( 785.3687786644884454, -419.3618753856918033, -315.3201227861279676 ) ) ;
#13613=CARTESIAN_POINT ( 'NONE',  ( 791.9812246680005501, -44.63460265842040542, -361.9419747391813189 ) ) ;
#13616=CARTESIAN_POINT ( 'NONE',  ( 755.2512626584698410, -199.5436935675108430, -315.2512626584710915 ) ) ;
#13622=CARTESIAN_POINT ( 'NONE',  ( 814.8230680027162407, -269.8055962898686175, -333.7305795820267917 ) ) ;
#13624=CARTESIAN_POINT ( 'NONE',  ( 755.2512626584698410, -271.5436935675106156, -315.2512626584710915 ) ) ;
#13625=DIRECTION ( 'NONE',  ( 0.000000000000000000, 0.000000000000000000, -1.000000000000000000 ) ) ;
#13628=CARTESIAN_POINT ( 'NONE',  ( 800.0135310231082713, -374.0891481129647786, -325.0180583372163028 ) ) ;
#13631=CARTESIAN_POINT ( 'NONE',  ( 766.5853460496234675, -61.98741447168745822, -372.3518521366060554 ) ) ;
#13632=CARTESIAN_POINT ( 'NONE',  ( 790.8726784830453198, -154.7146871989598935, -362.5472867521010585 ) ) ;
#13637=CARTESIAN_POINT ( 'NONE',  ( 801.9419747391806368, -66.45278447660216159, -351.9812246680014027 ) ) ;
#13638=CARTESIAN_POINT ( 'NONE',  ( 786.6156483768007774, -193.4419599262325278, -315.5913626894246136 ) ) ;
#13641=CARTESIAN_POINT ( 'NONE',  ( 744.8212110874229666, 5.103494619221427442, -336.2046728542121627 ) ) ;
#13646=CARTESIAN_POINT ( 'NONE',  ( 747.6481478633932056, -325.0999726633342561, -353.4146539503763620 ) ) ;
#13649=CIRCLE ( 'NONE', #43864, 30.00000000000008171 ) ;
#13653=CARTESIAN_POINT ( 'NONE',  ( 773.4516893846965786, -139.6454272087893571, -315.8398074228977066 ) ) ;
#13654=CARTESIAN_POINT ( 'NONE',  ( 788.7366044899766848, -155.9073299311473306, -316.5762568750059813 ) ) ;
#13655=CARTESIAN_POINT ( 'NONE',  ( 803.4237431249931660, -303.1800572038740711, -331.2633955100225194 ) ) ;
#13663=CARTESIAN_POINT ( 'NONE',  ( 762.1177392798416577, -378.5545181178795247, -309.8865473780659272 ) ) ;
#13669=CARTESIAN_POINT ( 'NONE',  ( 768.0187753319979720, -344.6346026584195101, -318.0580252608186242 ) ) ;
#13671=DIRECTION ( 'NONE',  ( 0.000000000000000000, -0.000000000000000000, -1.000000000000000000 ) ) ;
#13672=CARTESIAN_POINT ( 'NONE',  ( 755.3028492785439312, -231.2817908451527558, -335.9200461376539693 ) ) ;
#13674=CARTESIAN_POINT ( 'NONE',  ( 767.9999999999992042, 205.0000000000000568, -339.9999999999999432 ) ) ;
#13675=CARTESIAN_POINT ( 'NONE',  ( 812.7932403749906598, -423.1800572038737300, -327.7687537140311633 ) ) ;
#13680=CARTESIAN_POINT ( 'NONE',  ( 809.8718804791541288, -453.2309196406925480, -337.2303869152726179 ) ) ;
#13682=CARTESIAN_POINT ( 'NONE',  ( 777.4774526936600978, -58.27096629478398171, -304.7301800767027657 ) ) ;
#13683=CARTESIAN_POINT ( 'NONE',  ( 788.8264449731200330, -285.1800572038740711, -363.6646147819171233 ) ) ;
#13688=CARTESIAN_POINT ( 'NONE',  ( 746.4236121716829757, -15.82724539060794200, -328.8385539511384650 ) ) ;
#13689=CARTESIAN_POINT ( 'NONE',  ( 766.7756240680305382, -62.53286901714199786, -361.5560724626415663 ) ) ;
#13693=ADVANCED_FACE ( 'NONE', ( #41670 ), #24093, .F. ) ;
#13696=CARTESIAN_POINT ( 'NONE',  ( 788.7366044899766848, -59.90732993114762905, -316.5762568750059813 ) ) ;
#13697=EDGE_CURVE ( 'NONE', #31813, #12399, #27805, .T. ) ;
#13698=CARTESIAN_POINT ( 'NONE',  ( 754.8983024940795303, -354.8965053807774552, -336.9254006560228163 ) ) ;
#13701=ORIENTED_EDGE ( 'NONE', *, *, #22138, .F. ) ;
#13703=CARTESIAN_POINT ( 'NONE',  ( 811.6461892240364477, -388.7146871989592114, -324.1737431748509835 ) ) ;
#13709=CIRCLE ( 'NONE', #1881, 10.00000000000000888 ) ;
#13711=CARTESIAN_POINT ( 'NONE',  ( 792.2312462859673587, -203.9073299311471885, -307.2067596250082602 ) ) ;
#13715=CARTESIAN_POINT ( 'NONE',  ( 759.9864689768902508, -218.0891481129653187, -354.9819416627836404 ) ) ;
#13717=CARTESIAN_POINT ( 'NONE',  ( 804.9363028652555840, -376.2709662947829656, -338.2165204200192079 ) ) ;
#13718=CARTESIAN_POINT ( 'NONE',  ( 764.8639956371174549, -8.089148112965974136, -319.7806653035542013 ) ) ;
#13726=CARTESIAN_POINT ( 'NONE',  ( 781.8018195045266339, 1.729033705215812011, -365.1927285166406705 ) ) ;
#13728=CARTESIAN_POINT ( 'NONE',  ( 799.9999999999993179, -462.9681489794448339, -370.0000000000000568 ) ) ;
#13730=CARTESIAN_POINT ( 'NONE',  ( 815.3608509340175488, -290.7363362996980527, -341.2497674668889545 ) ) ;
#13733=CARTESIAN_POINT ( 'NONE',  ( 755.3201227861273992, -219.7255117493289447, -345.3687786644892981 ) ) ;
#13734=CARTESIAN_POINT ( 'NONE',  ( 786.6156483768007774, -385.4419599262319593, -315.5913626894246136 ) ) ;
#13738=CARTESIAN_POINT ( 'NONE',  ( 802.9823548866075953, -97.09997266333496668, -330.0799878456151077 ) ) ;
#13741=CARTESIAN_POINT ( 'NONE',  ( 800.1688906516307043, 13.83076734649413098, -369.0717654672308186 ) ) ;
#13742=CARTESIAN_POINT ( 'NONE',  ( 758.8095938919644823, -296.0891481129650629, -311.6929314249762797 ) ) ;
#13743=LINE ( 'NONE', #321, #3242 ) ;
#13745=CARTESIAN_POINT ( 'NONE',  ( 771.2633955100217236, -95.90732993114751537, -363.4237431249939618 ) ) ;
#13748=CARTESIAN_POINT ( 'NONE',  ( 764.3348316497523456, -166.7146871989598367, -308.6759233522265617 ) ) ;
#13750=CARTESIAN_POINT ( 'NONE',  ( 804.1009440267234822, 0.5363909730283709099, -314.0944755984392600 ) ) ;
#13754=CARTESIAN_POINT ( 'NONE',  ( 774.6312213355099630, -431.3618753856918033, -364.6798772138717482 ) ) ;
#13756=DIRECTION ( 'NONE',  ( 0.000000000000000000, 0.000000000000000000, -1.000000000000000000 ) ) ;
#13764=CARTESIAN_POINT ( 'NONE',  ( 796.7845633553578182, -249.6237781080505158, -358.5707757039688204 ) ) ;
#13766=CARTESIAN_POINT ( 'NONE',  ( 795.6651683502461765, -274.7146871989594388, -371.3240766477733814 ) ) ;
#13770=CARTESIAN_POINT ( 'NONE',  ( 790.8726784830453198, -34.71468719896025590, -362.5472867521010585 ) ) ;
#13771=CARTESIAN_POINT ( 'NONE',  ( 762.3223304703356007, -175.5436935675108998, -322.3223304703362828 ) ) ;
#13772=CARTESIAN_POINT ( 'NONE',  ( 801.9419747391806368, -210.4527844766016926, -351.9812246680014027 ) ) ;
#13774=CARTESIAN_POINT ( 'NONE',  ( 759.0252816721024374, -120.9982390220565378, -368.0189434323527280 ) ) ;
#13775=CARTESIAN_POINT ( 'NONE',  ( 791.9812246680005501, -92.63460265842026331, -361.9419747391813189 ) ) ;
#13777=CARTESIAN_POINT ( 'NONE',  ( 787.5531968255692163, -45.82724539060783542, -316.1348686366205811 ) ) ;
#13778=AXIS2_PLACEMENT_3D ( 'NONE', #10830, #42234, #37683 ) ;
#13779=CARTESIAN_POINT ( 'NONE',  ( 796.9571628226829034, -407.4636090269703459, -321.2382568024804641 ) ) ;
#13787=CARTESIAN_POINT ( 'NONE',  ( 804.4086373105744769, -361.6454272087887603, -333.3843516231986541 ) ) ;
#13788=CARTESIAN_POINT ( 'NONE',  ( 795.1360043628807261, -356.0891481129647218, -360.2193346964456282 ) ) ;
#13790=CARTESIAN_POINT ( 'NONE',  ( 813.5763878283155464, -171.8272453906074304, -351.1614460488615350 ) ) ;
#13795=CARTESIAN_POINT ( 'NONE',  ( 802.7791456095903868, -292.7146871989594956, -329.0155153010375102 ) ) ;
#13797=CARTESIAN_POINT ( 'NONE',  ( 799.9636004259356241, -142.9181544815166376, -311.2241431872006956 ) ) ;
#13802=CARTESIAN_POINT ( 'NONE',  ( 787.4397851343537695, -189.7255117493290300, -374.2001403089903988 ) ) ;
#13805=CARTESIAN_POINT ( 'NONE',  ( 751.6929314249748586, -294.9982390220560546, -318.8095938919659034 ) ) ;
#13811=CARTESIAN_POINT ( 'NONE',  ( 756.1443688327750579, -381.6237781080500326, -314.3581564841659315 ) ) ;
#13812=CARTESIAN_POINT ( 'NONE',  ( 796.7737145352015204, -140.6346026584201070, -370.7187646348536987 ) ) ;
#13813=CARTESIAN_POINT ( 'NONE',  ( 777.4774526936600978, -370.2709662947831362, -304.7301800767027657 ) ) ;
#13817=AXIS2_PLACEMENT_3D ( 'NONE', #200, #14292, #28365 ) ;
#13818=CARTESIAN_POINT ( 'NONE',  ( 807.5423716828161105, -153.0783235625962675, -362.2119215644372048 ) ) ;
#13825=CARTESIAN_POINT ( 'NONE',  ( 772.4837098697144029, -23.36187538569318889, -374.5518280994205611 ) ) ;
#13828=CARTESIAN_POINT ( 'NONE',  ( 766.4474001241216001, -427.0999726633338582, -307.3154664389482491 ) ) ;
#13831=CARTESIAN_POINT ( 'NONE',  ( 771.1735550268778070, -273.1800572038742985, -316.3353852180827630 ) ) ;
#13834=CARTESIAN_POINT ( 'NONE',  ( 790.0220218866281812, -247.0999726633344835, -363.2186876482849129 ) ) ;
#13835=CARTESIAN_POINT ( 'NONE',  ( 755.0636971347428243, -268.2709662947833067, -341.7834795799807353 ) ) ;
#13837=CARTESIAN_POINT ( 'NONE',  ( 767.8955696845333705, -96.45278447660203369, -362.1676090361162323 ) ) ;
#13841=CARTESIAN_POINT ( 'NONE',  ( 811.3240766477731540, -52.37269993606237506, -355.6651683502462902 ) ) ;
#13847=ORIENTED_EDGE ( 'NONE', *, *, #28565, .T. ) ;
#13848=CARTESIAN_POINT ( 'NONE',  ( 802.5472867521000353, -4.372699936062523385, -350.8726784830461156 ) ) ;
#13849=CARTESIAN_POINT ( 'NONE',  ( 748.9653473494365699, -74.63460265842030594, -356.9462024416520762 ) ) ;
#13852=CARTESIAN_POINT ( 'NONE',  ( 756.5762568750052424, -435.1800572038737869, -348.7366044899774238 ) ) ;
#13854=CARTESIAN_POINT ( 'NONE',  ( 815.2698199232961542, -208.8164208402380666, -342.5225473063383106 ) ) ;
#13858=CARTESIAN_POINT ( 'NONE',  ( 744.9990715423526808, -258.3510508353231785, -341.2370466360926002 ) ) ;
#13860=CARTESIAN_POINT ( 'NONE',  ( 747.2067596250078623, -291.1800572038741848, -352.2312462859687230 ) ) ;
#13864=CARTESIAN_POINT ( 'NONE',  ( 805.9055244015594326, -27.62377810805120149, -315.8990559732753240 ) ) ;
#13865=CARTESIAN_POINT ( 'NONE',  ( 762.1405469898971887, -385.5436935675102745, -357.8594530101015607 ) ) ;
#13867=CARTESIAN_POINT ( 'NONE',  ( 781.7834795799800531, -202.8164208402380950, -315.0636971347436202 ) ) ;
#13868=CARTESIAN_POINT ( 'NONE',  ( 807.5423716828161105, -33.07832356259662987, -362.2119215644372048 ) ) ;
#13869=CARTESIAN_POINT ( 'NONE',  ( 804.1601925771018387, -199.4419599262324709, -346.5483106153029098 ) ) ;
#13873=CARTESIAN_POINT ( 'NONE',  ( 775.9200461376533440, -191.8055962898689017, -315.3028492785443291 ) ) ;
#13875=CARTESIAN_POINT ( 'NONE',  ( 811.6461892240364477, -28.71468719896028077, -324.1737431748509835 ) ) ;
#13880=CARTESIAN_POINT ( 'NONE',  ( 809.0717654672305343, -292.9181544815162397, -360.1688906516309885 ) ) ;
#13886=CARTESIAN_POINT ( 'NONE',  ( 779.4763451958990572, -152.7363362996983938, -365.0264073115438919 ) ) ;
#13887=CARTESIAN_POINT ( 'NONE',  ( 800.0135310231082713, -134.0891481129655745, -325.0180583372163028 ) ) ;
#13888=CARTESIAN_POINT ( 'NONE',  ( 800.0135310231082713, -350.0891481129648923, -325.0180583372163028 ) ) ;
#13896=CARTESIAN_POINT ( 'NONE',  ( 802.2119215644370342, -366.0090635724250774, -367.5423716828165084 ) ) ;
#13901=CARTESIAN_POINT ( 'NONE',  ( 788.8264449731200330, -333.1800572038740142, -363.6646147819171233 ) ) ;
#13903=CARTESIAN_POINT ( 'NONE',  ( 755.8894580844503253, -207.8272453906073451, -332.3691319403863531 ) ) ;
#13907=CARTESIAN_POINT ( 'NONE',  ( 813.1304606946831655, -425.9073299311463643, -352.3570229623691716 ) ) ;
#13908=DIRECTION ( 'NONE',  ( -1.000000000000000000, 0.000000000000000000, -0.000000000000000000 ) ) ;
#13913=CARTESIAN_POINT ( 'NONE',  ( 755.2512626584698410, -55.54369356751127640, -315.2512626584710915 ) ) ;
#13915=CARTESIAN_POINT ( 'NONE',  ( 764.8639956371174549, -296.0891481129650629, -319.7806653035542013 ) ) ;
#13919=CARTESIAN_POINT ( 'NONE',  ( 764.1737431748507561, -34.37269993606243901, -371.6461892240376415 ) ) ;
#13920=CARTESIAN_POINT ( 'NONE',  ( 779.4709603349208464, -96.35105083532370429, -314.7162404726379918 ) ) ;
#13926=CARTESIAN_POINT ( 'NONE',  ( 767.8955696845333705, -48.45278447660219712, -362.1676090361162323 ) ) ;
#13927=CARTESIAN_POINT ( 'NONE',  ( 761.2382568024794409, -375.6237781080501463, -356.9571628226838129 ) ) ;
#13930=CARTESIAN_POINT ( 'NONE',  ( 788.7631598425961101, -385.4419599262319593, -305.7194118038759143 ) ) ;
#13935=CARTESIAN_POINT ( 'NONE',  ( 804.7487373415286811, -259.5436935675106156, -364.7487373415288516 ) ) ;
#13939=CARTESIAN_POINT ( 'NONE',  ( 792.1044303154646968, -204.4527844766016926, -317.8323909638837677 ) ) ;
#13942=CARTESIAN_POINT ( 'NONE',  ( 804.6798772138708955, -351.7255117493284047, -334.6312213355107019 ) ) ;
#13943=CARTESIAN_POINT ( 'NONE',  ( 762.3223304703356007, -7.543693567511430942, -322.3223304703362828 ) ) ;
#13948=CARTESIAN_POINT ( 'NONE',  ( 755.3028492785439312, -447.2817908451521021, -335.9200461376539693 ) ) ;
#13952=CARTESIAN_POINT ( 'NONE',  ( 810.4231160770870019, -264.5545181178798657, -321.9338519418446936 ) ) ;
#13955=CARTESIAN_POINT ( 'NONE',  ( 768.0187753319979720, -224.6346026584198228, -318.0580252608186242 ) ) ;
#13957=CARTESIAN_POINT ( 'NONE',  ( 772.3691319403857278, -407.2601417444137155, -315.8894580844506663 ) ) ;
#13960=CARTESIAN_POINT ( 'NONE',  ( 800.9840315886518738, -100.9181544815167513, -354.1144889064786412 ) ) ;
#13964=CARTESIAN_POINT ( 'NONE',  ( 789.6640940660590786, -442.9180389616178672, -363.1300863558843162 ) ) ;
#13965=CARTESIAN_POINT ( 'NONE',  ( 812.7932403749906598, -303.1800572038740711, -327.7687537140311633 ) ) ;
#13968=CARTESIAN_POINT ( 'NONE',  ( 801.9419747391806368, -90.45278447660209054, -351.9812246680014027 ) ) ;
#13970=CARTESIAN_POINT ( 'NONE',  ( 791.1614460488616487, -203.2601417444143124, -373.5763878283158874 ) ) ;
#13972=CARTESIAN_POINT ( 'NONE',  ( 811.0346526505616112, -446.6346026584189985, -323.0537975583477532 ) ) ;
#13975=CARTESIAN_POINT ( 'NONE',  ( 799.9999999999993179, 166.4563064324884465, -360.0000000000000000 ) ) ;
#13978=CARTESIAN_POINT ( 'NONE',  ( 754.8072714833581358, -412.8164208402372992, -338.1981804954720587 ) ) ;
#13985=CARTESIAN_POINT ( 'NONE',  ( 803.2186876482843445, -271.9874144716868045, -350.0220218866286928 ) ) ;
#13987=CARTESIAN_POINT ( 'NONE',  ( 744.8212110874229666, -306.8965053807775689, -336.2046728542121627 ) ) ;
#13994=CARTESIAN_POINT ( 'NONE',  ( 804.9511171171677688, -53.80559628986930676, -335.8780910478229202 ) ) ;
#13995=CARTESIAN_POINT ( 'NONE',  ( 791.9812246680005501, -164.6346026584200217, -361.9419747391813189 ) ) ;
#13996=CARTESIAN_POINT ( 'NONE',  ( 759.9864689768902508, -218.0891481129653187, -354.9819416627836404 ) ) ;
#13998=CARTESIAN_POINT ( 'NONE',  ( 792.2312462859673587, -155.9073299311473306, -307.2067596250082602 ) ) ;
#13999=CARTESIAN_POINT ( 'NONE',  ( 765.0180583372156207, -96.99823902205660886, -360.0135310231089534 ) ) ;
#14001=CARTESIAN_POINT ( 'NONE',  ( 799.2566176426618085, -384.0090635724249637, -324.0069404352559559 ) ) ;
#14009=CARTESIAN_POINT ( 'NONE',  ( 801.5560724626406000, -360.5545181178796383, -326.7756240680316182 ) ) ;
#14010=CARTESIAN_POINT ( 'NONE',  ( 758.0580252608178853, -366.4527844766012095, -328.0187753319985404 ) ) ;
#14011=CARTESIAN_POINT ( 'NONE',  ( 764.1737431748507561, -154.3726999360620198, -371.6461892240376415 ) ) ;
#14017=CARTESIAN_POINT ( 'NONE',  ( 784.0799538623451781, -299.8055962898685038, -364.6971507214555572 ) ) ;
#14019=CARTESIAN_POINT ( 'NONE',  ( 781.2370466360911223, -164.7363362996983938, -304.9990715423533629 ) ) ;
#14025=CARTESIAN_POINT ( 'NONE',  ( 792.2312462859673587, -203.9073299311471885, -307.2067596250082602 ) ) ;
#14027=CARTESIAN_POINT ( 'NONE',  ( 774.6858677611749044, 14.27448825067031812, -315.5713283507209894 ) ) ;
#14029=CARTESIAN_POINT ( 'NONE',  ( 786.2056067578752163, -107.8055962898691433, -374.4686193811670023 ) ) ;
#14030=CARTESIAN_POINT ( 'NONE',  ( 813.1304606946830518, -353.9073299311467053, -352.3570229623690580 ) ) ;
#14037=CARTESIAN_POINT ( 'NONE',  ( 801.9858362298568863, -363.0783235625955854, -312.7379699480935642 ) ) ;
#14038=CARTESIAN_POINT ( 'NONE',  ( 751.9810565676468741, -146.0891481129655176, -360.9747183278973921 ) ) ;
#14039=CARTESIAN_POINT ( 'NONE',  ( 814.9108240113580450, -424.2709662947829088, -337.5031285880265273 ) ) ;
#14044=CARTESIAN_POINT ( 'NONE',  ( 771.2368401574024119, -181.4419599262325278, -374.2805881961240857 ) ) ;
#14050=CARTESIAN_POINT ( 'NONE',  ( 805.0032342141412300, -13.54369356751140785, -314.9967657858571783 ) ) ;
#14053=CARTESIAN_POINT ( 'NONE',  ( 744.6391490659812007, -422.7363362996975980, -338.7502325331110455 ) ) ;
#14056=CARTESIAN_POINT ( 'NONE',  ( 800.0135310231082713, -254.0891481129652334, -325.0180583372163028 ) ) ;
#14060=CARTESIAN_POINT ( 'NONE',  ( 796.1575198192839480, -246.0090635724253900, -359.4546378042384163 ) ) ;
#14061=CARTESIAN_POINT ( 'NONE',  ( 795.1360043628807261, -260.0891481129650060, -360.2193346964456282 ) ) ;
#14062=CARTESIAN_POINT ( 'NONE',  ( 804.9363028652555840, -448.2709662947827951, -338.2165204200192079 ) ) ;
#14067=DIRECTION ( 'NONE',  ( 0.000000000000000000, -1.000000000000000000, 0.000000000000000000 ) ) ;
#14068=CARTESIAN_POINT ( 'NONE',  ( 768.9521613784389729, -33.82724539060788516, -373.2346286133773106 ) ) ;
#14073=VERTEX_POINT ( 'NONE', #43646 ) ;
#14074=CARTESIAN_POINT ( 'NONE',  ( 790.9844846989617508, -22.37269993606246743, -317.2208543904092721 ) ) ;
#14075=CARTESIAN_POINT ( 'NONE',  ( 777.5031285880264704, -94.81642084023843609, -374.9108240113588408 ) ) ;
#14077=DIRECTION ( 'NONE',  ( 0.000000000000000000, 0.000000000000000000, 1.000000000000000000 ) ) ;
#14079=CARTESIAN_POINT ( 'NONE',  ( 745.4481719005789273, -243.7255117493287742, -347.5162901302853129 ) ) ;
#14083=CARTESIAN_POINT ( 'NONE',  ( 803.8556311672234642, -273.6237781080504305, -365.6418435158340117 ) ) ;
#14085=CARTESIAN_POINT ( 'NONE',  ( 792.3570229623688874, -333.1800572038740142, -373.1304606946836202 ) ) ;
#14089=CARTESIAN_POINT ( 'NONE',  ( 762.3223304703356007, -391.5436935675101608, -322.3223304703362828 ) ) ;
#14091=CARTESIAN_POINT ( 'NONE',  ( 778.1981804954714335, -202.2709662947834772, -314.8072714833589885 ) ) ;
#14092=CARTESIAN_POINT ( 'NONE',  ( 768.8385539511368734, -47.26014174441477422, -306.4236121716840557 ) ) ;
#14093=CARTESIAN_POINT ( 'NONE',  ( 776.9566956441375396, -180.8965053807779952, -364.8461984189686405 ) ) ;
#14097=CARTESIAN_POINT ( 'NONE',  ( 772.3691319403857278, -191.2601417444143976, -315.8894580844506663 ) ) ;
#14099=PRODUCT_DEFINITION_SHAPE ( 'NONE', 'NONE',  #23335 ) ;
#14100=CARTESIAN_POINT ( 'NONE',  ( 773.7943932421234194, -47.80559628986931386, -305.5313806188329409 ) ) ;
#14105=CARTESIAN_POINT ( 'NONE',  ( 804.1009440267234822, -311.4636090269706870, -314.0944755984392600 ) ) ;
#14108=CARTESIAN_POINT ( 'NONE',  ( 755.5913626894240451, -157.6454272087893287, -346.6156483768012890 ) ) ;
#14109=CARTESIAN_POINT ( 'NONE',  ( 764.8639956371174549, -152.0891481129655460, -319.7806653035542013 ) ) ;
#14111=CARTESIAN_POINT ( 'NONE',  ( 781.7834795799800531, -346.8164208402376971, -315.0636971347436202 ) ) ;
#14120=CARTESIAN_POINT ( 'NONE',  ( 814.4686193811664907, -387.2817908451522726, -346.2056067578752732 ) ) ;
#14121=EDGE_CURVE ( 'NONE', #1648, #11148, #12015, .T. ) ;
#14125=CARTESIAN_POINT ( 'NONE',  ( 803.6646147819161570, -377.9073299311466485, -348.8264449731210561 ) ) ;
#14127=CARTESIAN_POINT ( 'NONE',  ( 755.1538015810308480, -230.1908817542436338, -343.0433043558613804 ) ) ;
#14131=CARTESIAN_POINT ( 'NONE',  ( 759.0252816721024374, -408.9982390220556567, -368.0189434323527280 ) ) ;
#14136=CARTESIAN_POINT ( 'NONE',  ( 814.5518280994195948, -39.72551174932951312, -332.4837098697145734 ) ) ;
#14137=CARTESIAN_POINT ( 'NONE',  ( 755.5713283507202505, -269.3618753856924286, -334.6858677611754729 ) ) ;
#14142=CARTESIAN_POINT ( 'NONE',  ( 771.3260364891663130, -19.64542720878974791, -306.0683387631859773 ) ) ;
#14143=CARTESIAN_POINT ( 'NONE',  ( 805.0264073115434940, -102.3510508353236901, -339.4763451958999099 ) ) ;
#14148=CARTESIAN_POINT ( 'NONE',  ( 770.0799878456142551, -109.9874144716873019, -362.9823548866085616 ) ) ;
#14150=CARTESIAN_POINT ( 'NONE',  ( 771.1735550268778070, -81.18005720387481006, -316.3353852180827630 ) ) ;
#14151=CARTESIAN_POINT ( 'NONE',  ( 804.1601925771018387, -391.4419599262317888, -346.5483106153029098 ) ) ;
#14154=CARTESIAN_POINT ( 'NONE',  ( 744.8212110874229666, -402.8965053807773415, -336.2046728542121627 ) ) ;
#14160=CARTESIAN_POINT ( 'NONE',  ( 814.2001403089898304, -257.3618753856924286, -347.4397851343538264 ) ) ;
#14163=CARTESIAN_POINT ( 'NONE',  ( 800.2193346964446619, -234.9982390220561683, -355.1360043628816925 ) ) ;
#14165=CARTESIAN_POINT ( 'NONE',  ( 755.3201227861273992, -363.7255117493284047, -345.3687786644892981 ) ) ;
#14166=CARTESIAN_POINT ( 'NONE',  ( 774.6312213355099630, -23.36187538569318889, -364.6798772138717482 ) ) ;
#14170=CARTESIAN_POINT ( 'NONE',  ( 799.9999999999993179, -512.9681489794448908, -339.9999999999999432 ) ) ;
#14172=CARTESIAN_POINT ( 'NONE',  ( 778.1981804954714335, -10.27096629478414691, -314.8072714833589885 ) ) ;
#14176=CARTESIAN_POINT ( 'NONE',  ( 748.6759233522253680, -256.3726999360617924, -324.3348316497537098 ) ) ;
#14179=CARTESIAN_POINT ( 'NONE',  ( 778.2165204200184689, -214.8164208402380666, -364.9363028652563230 ) ) ;
#14180=CARTESIAN_POINT ( 'NONE',  ( 760.5453621957607311, -405.0783235625954148, -323.8424801807151425 ) ) ;
#14181=CARTESIAN_POINT ( 'NONE',  ( 759.9999999999992042, -512.9681489794448908, -339.9999999999999432 ) ) ;
#14182=CARTESIAN_POINT ( 'NONE',  ( 780.5236548040995785, -116.7363362996985217, -314.9735926884559944 ) ) ;
#14185=CARTESIAN_POINT ( 'NONE',  ( 764.3348316497523456, 25.28531280103955226, -308.6759233522265617 ) ) ;
#14186=CARTESIAN_POINT ( 'NONE',  ( 744.7301800767020268, -316.8164208402377540, -337.4774526936615189 ) ) ;
#14189=CARTESIAN_POINT ( 'NONE',  ( 765.0180583372156207, -72.99823902205667991, -360.0135310231089534 ) ) ;
#14191=CARTESIAN_POINT ( 'NONE',  ( 798.0661480581538854, -194.5328690171415644, -309.5768839229118043 ) ) ;
#14193=CARTESIAN_POINT ( 'NONE',  ( 795.1271208383656131, -452.8379544210779954, -371.6178728169206238 ) ) ;
#14199=CARTESIAN_POINT ( 'NONE',  ( 800.2193346964447755, -450.9982390220554294, -355.1360043628815788 ) ) ;
#14205=CARTESIAN_POINT ( 'NONE',  ( 765.8855110935204493, -310.1692326535048778, -319.0159684113471599 ) ) ;
#14207=CARTESIAN_POINT ( 'NONE',  ( 793.4146539503750546, -289.9874144716866908, -307.6481478633938877 ) ) ;
#14212=CARTESIAN_POINT ( 'NONE',  ( 805.1016975059191054, -54.89650538077837183, -343.0745993439771837 ) ) ;
#14213=CARTESIAN_POINT ( 'NONE',  ( 800.2193346964447755, -162.9982390220563673, -355.1360043628815788 ) ) ;
#14214=CARTESIAN_POINT ( 'NONE',  ( 781.8018195045266339, -214.2709662947834488, -365.1927285166406705 ) ) ;
#14217=CARTESIAN_POINT ( 'NONE',  ( 758.8095938919642549, -152.0891481129655460, -311.6929314249763365 ) ) ;
#14218=CARTESIAN_POINT ( 'NONE',  ( 759.7806653035535192, -126.9982390220565094, -324.8639956371181370 ) ) ;
#14220=CARTESIAN_POINT ( 'NONE',  ( 796.1575198192839480, -390.0090635724249069, -359.4546378042384163 ) ) ;
#14229=CARTESIAN_POINT ( 'NONE',  ( 780.5236548040995785, -380.7363362996977116, -314.9735926884559944 ) ) ;
#14230=CARTESIAN_POINT ( 'NONE',  ( 764.8639956371174549, -344.0891481129647786, -319.7806653035542013 ) ) ;
#14231=AXIS2_PLACEMENT_3D ( 'NONE', #25546, #11696, #39659 ) ;
#14232=CARTESIAN_POINT ( 'NONE',  ( 791.0478386215596629, -165.8272453906074873, -306.7653713866226326 ) ) ;
#14234=CARTESIAN_POINT ( 'NONE',  ( 767.9999999999992042, 205.0000000000000568, -339.9999999999999432 ) ) ;
#14236=CARTESIAN_POINT ( 'NONE',  ( 793.2243759319678702, -290.5328690171412518, -318.4439275373583200 ) ) ;
#14237=CARTESIAN_POINT ( 'NONE',  ( 803.4237431249931660, -447.1800572038736732, -331.2633955100225194 ) ) ;
#14238=CARTESIAN_POINT ( 'NONE',  ( 793.5525998758768083, -151.0999726633347677, -372.6845335610516941 ) ) ;
#14243=CARTESIAN_POINT ( 'NONE',  ( 777.5031285880264704, -214.8164208402380666, -374.9108240113588408 ) ) ;
#14249=CARTESIAN_POINT ( 'NONE',  ( 745.1769319972822814, -113.8055962898691149, -346.2694204179732083 ) ) ;
#14251=CARTESIAN_POINT ( 'NONE',  ( 814.2001403089898304, -329.3618753856922581, -347.4397851343538264 ) ) ;
#14257=CARTESIAN_POINT ( 'NONE',  ( 744.9990715423526808, -426.3510508353226669, -341.2370466360926002 ) ) ;
#14258=CARTESIAN_POINT ( 'NONE',  ( 814.2001403089898304, -425.3618753856919170, -347.4397851343538264 ) ) ;
#14263=CARTESIAN_POINT ( 'NONE',  ( 747.3154664389472828, -187.9874144716870603, -326.4474001241230781 ) ) ;
#14271=CARTESIAN_POINT ( 'NONE',  ( 792.2312462859673587, -59.90732993114762905, -307.2067596250082602 ) ) ;
#14273=ORIENTED_EDGE ( 'NONE', *, *, #2706, .F. ) ;
#14274=CARTESIAN_POINT ( 'NONE',  ( 762.1177392798416577, -450.5545181178793541, -309.8865473780659272 ) ) ;
#14277=CARTESIAN_POINT ( 'NONE',  ( 800.0135310231082713, -278.0891481129651197, -325.0180583372163028 ) ) ;
#14283=CARTESIAN_POINT ( 'NONE',  ( 804.8461984189677878, -266.1908817542435486, -336.9566956441385628 ) ) ;
#14284=CARTESIAN_POINT ( 'NONE',  ( 756.5762568750052424, -243.1800572038743269, -348.7366044899774238 ) ) ;
#14285=CARTESIAN_POINT ( 'NONE',  ( 792.1044303154646968, -444.4527844766009821, -317.8323909638837677 ) ) ;
#14286=CARTESIAN_POINT ( 'NONE',  ( 756.3353852180819104, -101.9073299311474727, -331.1735550268788302 ) ) ;
#14291=CARTESIAN_POINT ( 'NONE',  ( 746.4236121716829757, -39.82724539060786384, -328.8385539511384650 ) ) ;
#14292=DIRECTION ( 'NONE',  ( 0.000000000000000000, -1.000000000000000000, 0.000000000000000000 ) ) ;
#14298=CARTESIAN_POINT ( 'NONE',  ( 760.7433823573367135, -12.00906357242613609, -355.9930595647440441 ) ) ;
#14300=CARTESIAN_POINT ( 'NONE',  ( 796.7737145352015204, -116.6346026584201780, -370.7187646348536987 ) ) ;
#14303=DIRECTION ( 'NONE',  ( -0.000000000000000000, 1.000000000000000000, -0.000000000000000000 ) ) ;
#14305=CARTESIAN_POINT ( 'NONE',  ( 782.5225473063381969, -238.2709662947833920, -375.2698199232970637 ) ) ;
#14309=CARTESIAN_POINT ( 'NONE',  ( 814.8230680027162407, -293.8055962898685607, -333.7305795820267917 ) ) ;
#14312=CARTESIAN_POINT ( 'NONE',  ( 808.0189434323515343, -326.0891481129649492, -319.0252816721025511 ) ) ;
#14316=CARTESIAN_POINT ( 'NONE',  ( 797.8594530101008786, -397.5436935675100472, -322.1405469898980982 ) ) ;
#14318=CARTESIAN_POINT ( 'NONE',  ( 798.0661480581538854, -98.53286901714187707, -309.5768839229118043 ) ) ;
#14323=CARTESIAN_POINT ( 'NONE',  ( 785.3687786644884454, -83.36187538569296862, -315.3201227861279676 ) ) ;
#14324=CARTESIAN_POINT ( 'NONE',  ( 783.0433043558608688, -216.8965053807778816, -315.1538015810313027 ) ) ;
#14326=CARTESIAN_POINT ( 'NONE',  ( 744.9990715423526808, -18.35105083532395298, -341.2370466360926002 ) ) ;
#14328=CARTESIAN_POINT ( 'NONE',  ( 807.0960494954803153, -452.9681489794450613, -341.9322302743943851 ) ) ;
#14333=CARTESIAN_POINT ( 'NONE',  ( 745.1792804349281596, -350.1908817542433212, -343.7566961878542884 ) ) ;
#14337=CARTESIAN_POINT ( 'NONE',  ( 766.9102291470427417, -138.5545181178802636, -318.6633372737382501 ) ) ;
#14338=CARTESIAN_POINT ( 'NONE',  ( 794.9819416627830151, -132.9982390220564810, -319.9864689768909898 ) ) ;
#14339=CARTESIAN_POINT ( 'NONE',  ( 756.5762568750052424, -363.1800572038739006, -348.7366044899774238 ) ) ;
#14350=CARTESIAN_POINT ( 'NONE',  ( 797.8822607201568644, -390.5545181178794678, -370.1134526219340160 ) ) ;
#14351=CARTESIAN_POINT ( 'NONE',  ( 815.2698199232962679, 7.183579159761249500, -342.5225473063383674 ) ) ;
#14354=CARTESIAN_POINT ( 'NONE',  ( 758.0580252608178853, -366.4527844766012095, -328.0187753319985404 ) ) ;
#14357=CARTESIAN_POINT ( 'NONE',  ( 787.5531968255692163, -237.8272453906072599, -316.1348686366205811 ) ) ;
#14361=CARTESIAN_POINT ( 'NONE',  ( 814.5518280994195948, -399.7255117493283478, -332.4837098697145166 ) ) ;
#14368=CARTESIAN_POINT ( 'NONE',  ( 800.9747183278959710, -60.99823902205671544, -311.9810565676471583 ) ) ;
#14369=CARTESIAN_POINT ( 'NONE',  ( 794.9819416627830151, -276.9982390220559978, -319.9864689768909898 ) ) ;
#14373=CARTESIAN_POINT ( 'NONE',  ( 815.3608509340175488, -50.73633629969874193, -341.2497674668889545 ) ) ;
#14374=CARTESIAN_POINT ( 'NONE',  ( 761.2382568024794409, -87.62377810805102740, -356.9571628226838129 ) ) ;
#14379=CARTESIAN_POINT ( 'NONE',  ( 771.2633955100217236, 0.09267006885218045942, -363.4237431249939618 ) ) ;
#14380=CARTESIAN_POINT ( 'NONE',  ( 795.9930595647434757, -99.07832356259642381, -320.7433823573372820 ) ) ;
#14382=CARTESIAN_POINT ( 'NONE',  ( 781.7834795799800531, -106.8164208402383935, -315.0636971347436202 ) ) ;
#14384=CARTESIAN_POINT ( 'NONE',  ( 758.6633372737375112, -404.5328690171409107, -326.9102291470432533 ) ) ;
#14387=CARTESIAN_POINT ( 'NONE',  ( 812.6845335610512393, -391.9874144716864066, -353.5525998758768651 ) ) ;
#14392=CARTESIAN_POINT ( 'NONE',  ( 792.3570229623688874, -261.1800572038741848, -373.1304606946836202 ) ) ;
#14398=CARTESIAN_POINT ( 'NONE',  ( 802.1676090361155502, -254.6346026584197091, -327.8955696845344505 ) ) ;
#14401=CARTESIAN_POINT ( 'NONE',  ( 803.6646147819161570, -353.9073299311467053, -348.8264449731210561 ) ) ;
#14402=CARTESIAN_POINT ( 'NONE',  ( 762.3223304703356007, -31.54369356751135456, -322.3223304703362828 ) ) ;
#14408=CARTESIAN_POINT ( 'NONE',  ( 781.8018195045266339, -22.27096629478410250, -365.1927285166406705 ) ) ;
#14412=CARTESIAN_POINT ( 'NONE',  ( 773.7305795820266212, -273.2817908451526137, -374.8230680027170365 ) ) ;
#14417=CARTESIAN_POINT ( 'NONE',  ( 756.5762568750052424, -243.1800572038743269, -348.7366044899774238 ) ) ;
#14418=CARTESIAN_POINT ( 'NONE',  ( 760.5453621957607311, -381.0783235625954717, -323.8424801807151425 ) ) ;
#14420=CARTESIAN_POINT ( 'NONE',  ( 790.9844846989617508, -118.3726999360621619, -317.2208543904092721 ) ) ;
#14423=CARTESIAN_POINT ( 'NONE',  ( 811.6461892240364477, -4.714687198960358039, -324.1737431748509835 ) ) ;
#14424=CARTESIAN_POINT ( 'NONE',  ( 815.2698199232962679, -304.8164208402376971, -342.5225473063383674 ) ) ;
#14428=CARTESIAN_POINT ( 'NONE',  ( 758.0141637701419768, -207.0783235625960685, -367.2620300519063790 ) ) ;
#14430=CARTESIAN_POINT ( 'NONE',  ( 759.0252816721024374, -432.9982390220555999, -368.0189434323527280 ) ) ;
#14436=CARTESIAN_POINT ( 'NONE',  ( 805.0264073115434940, 17.64894916467593688, -339.4763451958999099 ) ) ;
#14440=DIRECTION ( 'NONE',  ( -1.000000000000000000, -0.000000000000000000, -0.000000000000000000 ) ) ;
#14443=EDGE_LOOP ( 'NONE', ( #33044, #37887, #18026, #18432 ) ) ;
#14444=CARTESIAN_POINT ( 'NONE',  ( 772.3691319403857278, -311.2601417444139429, -315.8894580844506663 ) ) ;
#14446=CARTESIAN_POINT ( 'NONE',  ( 746.7653713866222915, -305.2601417444139429, -351.0478386215610271 ) ) ;
#14453=CARTESIAN_POINT ( 'NONE',  ( 795.9930595647434757, -75.07832356259649487, -320.7433823573372820 ) ) ;
#14454=CARTESIAN_POINT ( 'NONE',  ( 754.8072714833581358, -172.8164208402381234, -338.1981804954720587 ) ) ;
#14455=CARTESIAN_POINT ( 'NONE',  ( 765.0180583372156207, -192.9982390220562820, -360.0135310231089534 ) ) ;
#14458=CARTESIAN_POINT ( 'NONE',  ( 805.0032342141412300, -157.5436935675108998, -314.9967657858571783 ) ) ;
#14459=VERTEX_POINT ( 'NONE', #45716 ) ;
#14460=CARTESIAN_POINT ( 'NONE',  ( 764.8639956371174549, -128.0891481129655745, -319.7806653035542581 ) ) ;
#14462=CARTESIAN_POINT ( 'NONE',  ( 804.8461984189677878, -386.1908817542432075, -336.9566956441385628 ) ) ;
#14465=CARTESIAN_POINT ( 'NONE',  ( 779.9999999999992042, 126.4563064324884465, -339.9999999999999432 ) ) ;
#14469=CARTESIAN_POINT ( 'NONE',  ( 796.1575198192839480, -390.0090635724249069, -359.4546378042384163 ) ) ;
#14471=CARTESIAN_POINT ( 'NONE',  ( 752.7379699480933368, -180.0090635724255890, -361.9858362298580232 ) ) ;
#14476=CARTESIAN_POINT ( 'NONE',  ( 759.2295555964440155, -304.1692326535048210, -353.9708237608231229 ) ) ;
#14478=CARTESIAN_POINT ( 'NONE',  ( 814.4686193811664907, -195.2817908451528410, -346.2056067578752732 ) ) ;
#14485=CARTESIAN_POINT ( 'NONE',  ( 767.7687537140311633, -191.9073299311471885, -372.7932403749916830 ) ) ;
#14487=CARTESIAN_POINT ( 'NONE',  ( 762.3223304703356007, 16.45630643248849267, -322.3223304703362828 ) ) ;
#14490=CARTESIAN_POINT ( 'NONE',  ( 781.2497674668890113, -84.35105083532374692, -375.3608509340180603 ) ) ;
#14492=CARTESIAN_POINT ( 'NONE',  ( 796.7737145352015204, -332.6346026584195101, -370.7187646348536987 ) ) ;
#14500=CARTESIAN_POINT ( 'NONE',  ( 744.9990715423526808, -402.3510508353228374, -341.2370466360926002 ) ) ;
#14501=CARTESIAN_POINT ( 'NONE',  ( 751.9810565676468741, -434.0891481129646081, -360.9747183278973921 ) ) ;
#14504=VERTEX_POINT ( 'NONE', #24668 ) ;
#14506=CARTESIAN_POINT ( 'NONE',  ( 805.9055244015594326, -195.6237781080506863, -315.8990559732753240 ) ) ;
#14514=CARTESIAN_POINT ( 'NONE',  ( 745.0891759886404770, -28.27096629478409540, -342.4968714119734159 ) ) ;
#14516=ORIENTED_EDGE ( 'NONE', *, *, #37393, .T. ) ;
#14517=CARTESIAN_POINT ( 'NONE',  ( 814.2805881961230625, -433.6454272087884760, -331.2368401574024119 ) ) ;
#14522=CARTESIAN_POINT ( 'NONE',  ( 778.2165204200184689, -286.8164208402378677, -364.9363028652563230 ) ) ;
#14527=CARTESIAN_POINT ( 'NONE',  ( 754.7162404726377645, -278.7363362996980527, -339.4709603349214717 ) ) ;
#14528=CARTESIAN_POINT ( 'NONE',  ( 762.3223304703356007, -295.5436935675105588, -322.3223304703362828 ) ) ;
#14529=CARTESIAN_POINT ( 'NONE',  ( 756.3353852180820240, -437.9073299311464211, -331.1735550268787733 ) ) ;
#14530=CARTESIAN_POINT ( 'NONE',  ( 762.3223304703356007, -103.5436935675111272, -322.3223304703362828 ) ) ;
#14535=CARTESIAN_POINT ( 'NONE',  ( 814.2805881961230625, -97.64542720878949922, -331.2368401574024119 ) ) ;
#14541=CARTESIAN_POINT ( 'NONE',  ( 755.8894580844503253, -63.82724539060779279, -332.3691319403863531 ) ) ;
#14542=CARTESIAN_POINT ( 'NONE',  ( 792.2312462859673587, -107.9073299311474727, -307.2067596250082602 ) ) ;
#14547=CARTESIAN_POINT ( 'NONE',  ( 787.5162901302840055, -227.3618753856925707, -305.4481719005792684 ) ) ;
#14552=CARTESIAN_POINT ( 'NONE',  ( 747.3154664389472828, -307.9874144716866340, -326.4474001241230781 ) ) ;
#14555=CARTESIAN_POINT ( 'NONE',  ( 745.4481719005789273, -315.7255117493286320, -347.5162901302853129 ) ) ;
#14560=CARTESIAN_POINT ( 'NONE',  ( 804.6798772138708955, -399.7255117493283478, -334.6312213355107019 ) ) ;
#14564=CARTESIAN_POINT ( 'NONE',  ( 746.0683387631852383, -91.44195992623282621, -331.3260364891676204 ) ) ;
#14568=CARTESIAN_POINT ( 'NONE',  ( 754.8983024940795303, -210.8965053807778816, -336.9254006560228163 ) ) ;
#14570=CARTESIAN_POINT ( 'NONE',  ( 815.0009284576459549, -30.35105083532391390, -338.7629533639073429 ) ) ;
#14572=CARTESIAN_POINT ( 'NONE',  ( 807.4745771775690173, -452.9681489794449476, -340.5093320845589346 ) ) ;
#14574=EDGE_CURVE ( 'NONE', #11372, #41096, #44024, .T. ) ;
#14577=CARTESIAN_POINT ( 'NONE',  ( 771.3260364891663130, -355.6454272087887603, -306.0683387631859773 ) ) ;
#14578=AXIS2_PLACEMENT_3D ( 'NONE', #34050, #30591, #16509 ) ;
#14582=CARTESIAN_POINT ( 'NONE',  ( 773.4516893846965786, -187.6454272087892434, -315.8398074228977066 ) ) ;
#14583=CARTESIAN_POINT ( 'NONE',  ( 797.8594530101008786, -157.5436935675108998, -322.1405469898980982 ) ) ;
#14584=CARTESIAN_POINT ( 'NONE',  ( 778.1981804954715471, -346.2709662947830225, -314.8072714833591021 ) ) ;
#14586=CARTESIAN_POINT ( 'NONE',  ( 764.0069404352550464, 8.921676437403235127, -359.2566176426627180 ) ) ;
#14589=FACE_OUTER_BOUND ( 'NONE', #12288, .T. ) ;
#14596=CARTESIAN_POINT ( 'NONE',  ( 783.7953271457878373, -416.1908817542430938, -375.1787889125761239 ) ) ;
#14597=CARTESIAN_POINT ( 'NONE',  ( 811.0346526505617248, 9.365397341579424051, -323.0537975583478101 ) ) ;
#14600=CARTESIAN_POINT ( 'NONE',  ( 755.0636971347428243, -364.2709662947830793, -341.7834795799807353 ) ) ;
#14601=ADVANCED_FACE ( 'NONE', ( #8065 ), #29309, .F. ) ;
#14604=CARTESIAN_POINT ( 'NONE',  ( 790.9844846989617508, -238.3726999360617640, -317.2208543904092721 ) ) ;
#14609=CARTESIAN_POINT ( 'NONE',  ( 814.2001403089898304, -401.3618753856920307, -347.4397851343538264 ) ) ;
#14614=CARTESIAN_POINT ( 'NONE',  ( 763.2262854647970016, -56.63460265842036279, -309.2812353651462445 ) ) ;
#14616=CARTESIAN_POINT ( 'NONE',  ( 762.3223304703356007, -295.5436935675105588, -322.3223304703362828 ) ) ;
#14617=DIRECTION ( 'NONE',  ( 0.000000000000000000, 0.000000000000000000, -1.000000000000000000 ) ) ;
#14620=CARTESIAN_POINT ( 'NONE',  ( 804.1009440267234822, -47.46360902697148987, -314.0944755984392600 ) ) ;
#14621=CARTESIAN_POINT ( 'NONE',  ( 757.2208543904082489, -88.71468719896009247, -350.9844846989624330 ) ) ;
#14625=CARTESIAN_POINT ( 'NONE',  ( 799.4546378042377910, -105.0783235625964096, -356.1575198192848006 ) ) ;
#14627=CARTESIAN_POINT ( 'NONE',  ( 791.9812246680005501, -92.63460265842026331, -361.9419747391813189 ) ) ;
#14628=CARTESIAN_POINT ( 'NONE',  ( 798.7617431975189675, -411.6237781080499758, -323.0428371773161871 ) ) ;
#14631=CARTESIAN_POINT ( 'NONE',  ( 810.1134526219336749, -416.5328690171409107, -357.8822607201570349 ) ) ;
#14636=CARTESIAN_POINT ( 'NONE',  ( 758.8095938919642549, -248.0891481129651481, -311.6929314249763365 ) ) ;
#14641=CARTESIAN_POINT ( 'NONE',  ( 780.5236548040995785, -68.73633629969867798, -314.9735926884559944 ) ) ;
#14642=CARTESIAN_POINT ( 'NONE',  ( 771.2633955100217236, -239.9073299311470748, -363.4237431249939618 ) ) ;
#14643=VERTEX_POINT ( 'NONE', #8272 ) ;
#14644=CARTESIAN_POINT ( 'NONE',  ( 788.8264449731200330, -357.1800572038739006, -363.6646147819171233 ) ) ;
#14645=CARTESIAN_POINT ( 'NONE',  ( 759.7806653035534055, -54.99823902205672255, -324.8639956371180801 ) ) ;
#14650=CARTESIAN_POINT ( 'NONE',  ( 759.9864689768902508, -2.089148112965993231, -354.9819416627836404 ) ) ;
#14653=CARTESIAN_POINT ( 'NONE',  ( 791.0478386215596629, -285.8272453906071178, -306.7653713866226326 ) ) ;
#14657=CARTESIAN_POINT ( 'NONE',  ( 785.3141322388236176, -261.7255117493288026, -364.4286716492789537 ) ) ;
#14658=CARTESIAN_POINT ( 'NONE',  ( 804.1105419155481968, -99.82724539060768620, -347.6308680596136469 ) ) ;
#14661=CARTESIAN_POINT ( 'NONE',  ( 786.2056067578752163, -11.80559628986942577, -374.4686193811670023 ) ) ;
#14662=CARTESIAN_POINT ( 'NONE',  ( 782.5225473063383106, -310.2709662947832499, -375.2698199232970637 ) ) ;
#14663=DIRECTION ( 'NONE',  ( 1.000000000000000000, 0.000000000000000000, -0.000000000000000000 ) ) ;
#14666=CARTESIAN_POINT ( 'NONE',  ( 744.8212110874229666, -210.8965053807778816, -336.2046728542121627 ) ) ;
#14668=CARTESIAN_POINT ( 'NONE',  ( 793.3938497862117174, -453.0432664090020012, -372.3358127763067955 ) ) ;
#14673=CARTESIAN_POINT ( 'NONE',  ( 773.3843516231979720, 10.55804007376686826, -364.4086373105754433 ) ) ;
#14674=CARTESIAN_POINT ( 'NONE',  ( 799.9999999999993179, 166.4563064324884465, -319.9999999999999432 ) ) ;
#14679=CARTESIAN_POINT ( 'NONE',  ( 760.5453621957607311, -285.0783235625958127, -323.8424801807151425 ) ) ;
#14681=CARTESIAN_POINT ( 'NONE',  ( 813.9316612368132837, -295.4419599262320730, -348.6739635108323228 ) ) ;
#14686=CIRCLE ( 'NONE', #19805, 10.00000000000000888 ) ;
#14687=CARTESIAN_POINT ( 'NONE',  ( 772.3691319403857278, -71.26014174441469606, -315.8894580844506663 ) ) ;
#14688=CARTESIAN_POINT ( 'NONE',  ( 785.3141322388236176, -165.7255117493291152, -364.4286716492789537 ) ) ;
#14689=CARTESIAN_POINT ( 'NONE',  ( 771.1735550268778070, -201.1800572038744690, -316.3353852180827630 ) ) ;
#14691=CARTESIAN_POINT ( 'NONE',  ( 751.9810565676468741, -146.0891481129655176, -360.9747183278973921 ) ) ;
#14693=CARTESIAN_POINT ( 'NONE',  ( 778.1981804954715471, -154.2709662947836762, -314.8072714833591021 ) ) ;
#14695=CARTESIAN_POINT ( 'NONE',  ( 798.5707757039680246, -389.4636090269704027, -356.7845633553585003 ) ) ;
#14703=CARTESIAN_POINT ( 'NONE',  ( 790.0220218866281812, -391.0999726633340288, -363.2186876482849129 ) ) ;
#14705=CARTESIAN_POINT ( 'NONE',  ( 754.3581564841646241, -185.4636090269710280, -316.1443688327762516 ) ) ;
#14709=CARTESIAN_POINT ( 'NONE',  ( 803.8651313633788504, -341.2601417444138292, -332.4468031744301015 ) ) ;
#14710=CARTESIAN_POINT ( 'NONE',  ( 795.1360043628807261, -452.0891481129646650, -360.2193346964456282 ) ) ;
#14711=CARTESIAN_POINT ( 'NONE',  ( 799.9636004259356241, -190.9181544815164955, -311.2241431872006956 ) ) ;
#14717=CARTESIAN_POINT ( 'NONE',  ( 804.7487373415286811, -211.5436935675107861, -364.7487373415288516 ) ) ;
#14719=CARTESIAN_POINT ( 'NONE',  ( 756.3353852180819104, -29.90732993114771787, -331.1735550268788302 ) ) ;
#14722=CARTESIAN_POINT ( 'NONE',  ( 798.0661480581538854, -98.53286901714187707, -309.5768839229118043 ) ) ;
#14724=CARTESIAN_POINT ( 'NONE',  ( 745.4481719005789273, -339.7255117493285184, -347.5162901302853129 ) ) ;
#14729=CARTESIAN_POINT ( 'NONE',  ( 756.1443688327750579, -405.6237781080500326, -314.3581564841659315 ) ) ;
#14730=( BOUNDED_CURVE ( )  B_SPLINE_CURVE ( 2, ( #9790, #9341, #34506, #27564, #13491, #23411, #37513 ),
 .UNSPECIFIED., .F., .T. ) 
 B_SPLINE_CURVE_WITH_KNOTS ( ( 3, 2, 2, 3 ),
 ( 0.000000000000000000, 0.002272727272727272617, 0.004545454545454545234, 0.006081874955971018626 ),
 .UNSPECIFIED. ) 
 CURVE ( )  GEOMETRIC_REPRESENTATION_ITEM ( )  RATIONAL_B_SPLINE_CURVE ( ( 0.5000002209606653203, 0.4949109396520706694, 0.5000002209606653203, 0.4949109396520706694, 0.5000002209606653203, 0.4965597396626160176, 0.4977709609702910543 ) ) 
 REPRESENTATION_ITEM ( '' )  );
#14731=CARTESIAN_POINT ( 'NONE',  ( 745.4481719005789273, -435.7255117493282341, -347.5162901302853129 ) ) ;
#14736=CARTESIAN_POINT ( 'NONE',  ( 791.1614460488616487, -203.2601417444143124, -373.5763878283158874 ) ) ;
#14741=CARTESIAN_POINT ( 'NONE',  ( 759.0252816721024374, -48.99823902205675807, -368.0189434323527280 ) ) ;
#14744=CARTESIAN_POINT ( 'NONE',  ( 812.3518521366052028, -457.0999726633339151, -326.5853460496235243 ) ) ;
#14750=CARTESIAN_POINT ( 'NONE',  ( 801.9419747391806368, -282.4527844766014937, -351.9812246680014027 ) ) ;
#14753=CARTESIAN_POINT ( 'NONE',  ( 758.4439275373578084, -300.5545181178797520, -353.2243759319684386 ) ) ;
#14754=CARTESIAN_POINT ( 'NONE',  ( 804.9363028652555840, -304.2709662947832499, -338.2165204200192079 ) ) ;
#14755=CARTESIAN_POINT ( 'NONE',  ( 762.3223304703356007, -439.5436935675101040, -322.3223304703362828 ) ) ;
#14756=CARTESIAN_POINT ( 'NONE',  ( 765.0180583372156207, -120.9982390220565378, -360.0135310231089534 ) ) ;
#14763=CARTESIAN_POINT ( 'NONE',  ( 799.9636004259356241, -94.91815448151677970, -311.2241431872006956 ) ) ;
#14770=CARTESIAN_POINT ( 'NONE',  ( 757.4527132478984868, -40.37269993606240348, -329.1273215169538844 ) ) ;
#14772=CARTESIAN_POINT ( 'NONE',  ( 787.5162901302840055, -107.3618753856928976, -305.4481719005793252 ) ) ;
#14774=CYLINDRICAL_SURFACE ( 'NONE', #35922, 10.00000000000000888 ) ;
#14776=CARTESIAN_POINT ( 'NONE',  ( 811.0346526505616112, -230.6346026584197659, -323.0537975583477532 ) ) ;
#14779=CARTESIAN_POINT ( 'NONE',  ( 800.1688906516307043, -322.1692326535048210, -369.0717654672308186 ) ) ;
#14781=CARTESIAN_POINT ( 'NONE',  ( 796.9462024416508257, -324.4527844766013231, -308.9653473494370246 ) ) ;
#14785=CARTESIAN_POINT ( 'NONE',  ( 768.0187753319979720, -416.6346026584192259, -318.0580252608186242 ) ) ;
#14787=CARTESIAN_POINT ( 'NONE',  ( 761.9338519418445230, -86.53286901714194812, -370.4231160770881957 ) ) ;
#14791=CARTESIAN_POINT ( 'NONE',  ( 765.8855110935204493, -238.1692326535050768, -319.0159684113471599 ) ) ;
#14793=CARTESIAN_POINT ( 'NONE',  ( 803.8556311672234642, -33.62377810805116951, -365.6418435158340117 ) ) ;
#14795=LINE ( 'NONE', #3929, #7717 ) ;
#14799=CARTESIAN_POINT ( 'NONE',  ( 746.4236121716829757, -327.8272453906069472, -328.8385539511384650 ) ) ;
#14803=CARTESIAN_POINT ( 'NONE',  ( 802.5472867521000353, -196.3726999360619061, -350.8726784830461156 ) ) ;
#14804=CARTESIAN_POINT ( 'NONE',  ( 755.5713283507202505, -173.3618753856927128, -334.6858677611754729 ) ) ;
#14805=CARTESIAN_POINT ( 'NONE',  ( 797.8594530101009923, -349.5436935675103314, -322.1405469898982119 ) ) ;
#14807=CARTESIAN_POINT ( 'NONE',  ( 779.4709603349208464, 23.64894916467591912, -314.7162404726379918 ) ) ;
#14813=EDGE_CURVE ( 'NONE', #29231, #29607, #34434, .T. ) ;
#14817=CARTESIAN_POINT ( 'NONE',  ( 802.2119215644370342, -414.0090635724249637, -367.5423716828165084 ) ) ;
#14818=CARTESIAN_POINT ( 'NONE',  ( 744.7301800767020268, -4.816420840238714085, -337.4774526936615189 ) ) ;
#14821=CARTESIAN_POINT ( 'NONE',  ( 767.8955696845333705, -360.4527844766010958, -362.1676090361162323 ) ) ;
#14825=CARTESIAN_POINT ( 'NONE',  ( 779.4763451958990572, -272.7363362996981095, -365.0264073115438919 ) ) ;
#14829=CARTESIAN_POINT ( 'NONE',  ( 813.1304606946831655, -449.9073299311464211, -352.3570229623691716 ) ) ;
#14836=CARTESIAN_POINT ( 'NONE',  ( 755.2512626584698410, -103.5436935675111272, -315.2512626584710915 ) ) ;
#14837=CARTESIAN_POINT ( 'NONE',  ( 795.1360043628807261, -332.0891481129649492, -360.2193346964456282 ) ) ;
#14841=CARTESIAN_POINT ( 'NONE',  ( 783.7953271457878373, -80.19088175424411702, -375.1787889125761239 ) ) ;
#14842=CARTESIAN_POINT ( 'NONE',  ( 786.6156483768007774, -73.44195992623286884, -315.5913626894246136 ) ) ;
#14848=CARTESIAN_POINT ( 'NONE',  ( 764.8639956371174549, -104.0891481129656881, -319.7806653035542013 ) ) ;
#14849=CARTESIAN_POINT ( 'NONE',  ( 765.8855110935204493, -382.1692326535045936, -319.0159684113471599 ) ) ;
#14855=EDGE_CURVE ( 'NONE', #35738, #24791, #35999, .T. ) ;
#14862=CARTESIAN_POINT ( 'NONE',  ( 773.4516893846965786, -91.64542720878951343, -315.8398074228977066 ) ) ;
#14864=CARTESIAN_POINT ( 'NONE',  ( 785.3141322388236176, -237.7255117493289163, -364.4286716492789537 ) ) ;
#14866=CARTESIAN_POINT ( 'NONE',  ( 794.9819416627830151, -396.9982390220556567, -319.9864689768909898 ) ) ;
#14867=CARTESIAN_POINT ( 'NONE',  ( 771.2633955100217236, -47.90732993114767169, -363.4237431249939618 ) ) ;
#14872=CARTESIAN_POINT ( 'NONE',  ( 764.8639956371174549, -8.089148112965974136, -319.7806653035542013 ) ) ;
#14875=CARTESIAN_POINT ( 'NONE',  ( 810.4231160770870019, -312.5545181178797520, -321.9338519418446936 ) ) ;
#14878=CARTESIAN_POINT ( 'NONE',  ( 755.5713283507202505, -269.3618753856924286, -334.6858677611754729 ) ) ;
#14880=CARTESIAN_POINT ( 'NONE',  ( 790.0220218866281812, -103.0999726633349525, -363.2186876482849129 ) ) ;
#14883=CARTESIAN_POINT ( 'NONE',  ( 751.6929314249750860, -342.9982390220557704, -318.8095938919659034 ) ) ;
#14887=CARTESIAN_POINT ( 'NONE',  ( 744.9990715423526808, -210.3510508353233490, -341.2370466360926002 ) ) ;
#14889=CARTESIAN_POINT ( 'NONE',  ( 778.7502325331095108, -432.3510508353226669, -304.6391490659818828 ) ) ;
#14894=CARTESIAN_POINT ( 'NONE',  ( 776.9566956441375396, 11.10349461922141145, -364.8461984189686405 ) ) ;
#14900=CARTESIAN_POINT ( 'NONE',  ( 805.0264073115434940, -294.3510508353230648, -339.4763451958999099 ) ) ;
#14901=CARTESIAN_POINT ( 'NONE',  ( 756.1443688327750579, -285.6237781080502600, -314.3581564841659315 ) ) ;
#14907=CARTESIAN_POINT ( 'NONE',  ( 783.0433043558608688, -72.89650538077830788, -315.1538015810313027 ) ) ;
#14908=CARTESIAN_POINT ( 'NONE',  ( 779.9999999999992042, 16.45630643248849267, -339.9999999999999432 ) ) ;
#14909=CARTESIAN_POINT ( 'NONE',  ( 801.1904061080336987, -164.0891481129655176, -368.3070685750235498 ) ) ;
#14912=CARTESIAN_POINT ( 'NONE',  ( 754.8072714833583632, -124.8164208402383366, -338.1981804954721156 ) ) ;
#14914=CARTESIAN_POINT ( 'NONE',  ( 757.0176451133909268, -421.0999726633340288, -349.9200121543848354 ) ) ;
#14921=CARTESIAN_POINT ( 'NONE',  ( 787.5531968255692163, -381.8272453906068336, -316.1348686366205811 ) ) ;
#14923=CARTESIAN_POINT ( 'NONE',  ( 799.9636004259356241, -214.9181544815164386, -311.2241431872006956 ) ) ;
#14927=CARTESIAN_POINT ( 'NONE',  ( 764.0069404352550464, -327.0783235625956991, -359.2566176426627180 ) ) ;
#14929=CARTESIAN_POINT ( 'NONE',  ( 745.1792804349281596, -182.1908817542437760, -343.7566961878542884 ) ) ;
#14933=CARTESIAN_POINT ( 'NONE',  ( 754.9967657858570647, -217.5436935675107293, -365.0032342141425943 ) ) ;
#14935=CARTESIAN_POINT ( 'NONE',  ( 764.8639956371174549, -8.089148112965974136, -319.7806653035542013 ) ) ;
#14937=CARTESIAN_POINT ( 'NONE',  ( 801.9858362298568863, -99.07832356259642381, -312.7379699480935642 ) ) ;
#14939=CARTESIAN_POINT ( 'NONE',  ( 758.8095938919642549, -344.0891481129647786, -311.6929314249763365 ) ) ;
#14945=CARTESIAN_POINT ( 'NONE',  ( 749.8865473780648472, -404.5328690171409107, -322.1177392798429082 ) ) ;
#14946=CARTESIAN_POINT ( 'NONE',  ( 814.5518280994195948, -423.7255117493281205, -332.4837098697145734 ) ) ;
#14950=CARTESIAN_POINT ( 'NONE',  ( 756.1348686366196716, -185.2601417444143692, -347.5531968255698416 ) ) ;
#14952=CARTESIAN_POINT ( 'NONE',  ( 798.0661480581538854, -194.5328690171415644, -309.5768839229118043 ) ) ;
#14957=CARTESIAN_POINT ( 'NONE',  ( 771.2633955100217236, -143.9073299311473590, -363.4237431249939618 ) ) ;
#14959=CARTESIAN_POINT ( 'NONE',  ( 763.0537975583475827, -48.45278447660219712, -371.0346526505627480 ) ) ;
#14963=CARTESIAN_POINT ( 'NONE',  ( 791.0478386215596629, -453.8272453906066630, -306.7653713866226326 ) ) ;
#14965=CARTESIAN_POINT ( 'NONE',  ( 766.9102291470427417, -306.5545181178797520, -318.6633372737382501 ) ) ;
#14968=CARTESIAN_POINT ( 'NONE',  ( 804.6798772138708955, -279.7255117493288026, -334.6312213355107019 ) ) ;
#14972=CARTESIAN_POINT ( 'NONE',  ( 793.0897708529556667, -294.5545181178797520, -361.3366627262616362 ) ) ;
#14973=CARTESIAN_POINT ( 'NONE',  ( 788.7366044899766848, -275.9073299311469896, -316.5762568750059813 ) ) ;
#14975=CARTESIAN_POINT ( 'NONE',  ( 762.1405469898971887, -121.5436935675110419, -357.8594530101015607 ) ) ;
#14981=CARTESIAN_POINT ( 'NONE',  ( 768.9521613784389729, -81.82724539060772884, -373.2346286133773106 ) ) ;
#14987=CARTESIAN_POINT ( 'NONE',  ( 748.9653473494365699, -98.63460265842023489, -356.9462024416520762 ) ) ;
#14991=CARTESIAN_POINT ( 'NONE',  ( 808.0189434323515343, -230.0891481129652618, -319.0252816721025511 ) ) ;
#14995=CARTESIAN_POINT ( 'NONE',  ( 786.2056067578752163, -323.8055962898684470, -374.4686193811670023 ) ) ;
#14997=CARTESIAN_POINT ( 'NONE',  ( 814.2001403089898304, -305.3618753856922581, -347.4397851343538264 ) ) ;
#15001=CARTESIAN_POINT ( 'NONE',  ( 774.6858677611749044, -417.7255117493283478, -315.5713283507209894 ) ) ;
#15002=CARTESIAN_POINT ( 'NONE',  ( 747.3154664389472828, -91.98741447168737295, -326.4474001241230781 ) ) ;
#15009=CARTESIAN_POINT ( 'NONE',  ( 773.3843516231979720, -229.4419599262323572, -364.4086373105754433 ) ) ;
#15011=CARTESIAN_POINT ( 'NONE',  ( 771.2368401574024119, -61.44195992623291147, -374.2805881961240857 ) ) ;
#15013=CARTESIAN_POINT ( 'NONE',  ( 794.5458710602071051, -452.9681489794447771, -360.4198067286714604 ) ) ;
#15015=CARTESIAN_POINT ( 'NONE',  ( 757.7880784355613741, -330.0090635724251342, -312.4576283171834916 ) ) ;
#15018=CARTESIAN_POINT ( 'NONE',  ( 804.1105419155481968, -195.8272453906074304, -347.6308680596136469 ) ) ;
#15019=CARTESIAN_POINT ( 'NONE',  ( 803.4237431249931660, -183.1800572038744974, -331.2633955100225194 ) ) ;
#15021=CARTESIAN_POINT ( 'NONE',  ( 765.0180583372156207, -384.9982390220556567, -360.0135310231089534 ) ) ;
#15024=CARTESIAN_POINT ( 'NONE',  ( 800.2193346964447755, -450.9982390220554294, -355.1360043628815788 ) ) ;
#15033=CARTESIAN_POINT ( 'NONE',  ( 745.7194118038753459, -397.6454272087885329, -348.7631598425976449 ) ) ;
#15034=CARTESIAN_POINT ( 'NONE',  ( 792.2312462859673587, -11.90732993114778182, -307.2067596250082602 ) ) ;
#15037=CARTESIAN_POINT ( 'NONE',  ( 804.9363028652555840, -352.2709662947830225, -338.2165204200192079 ) ) ;
#15042=CARTESIAN_POINT ( 'NONE',  ( 757.0176451133909268, -253.0999726633345119, -349.9200121543848354 ) ) ;
#15050=CARTESIAN_POINT ( 'NONE',  ( 771.2633955100217236, -311.9073299311468759, -363.4237431249939618 ) ) ;
#15057=CARTESIAN_POINT ( 'NONE',  ( 811.3240766477731540, -52.37269993606237506, -355.6651683502462902 ) ) ;
#15058=CARTESIAN_POINT ( 'NONE',  ( 761.2382568024794409, -135.6237781080508853, -356.9571628226838129 ) ) ;
#15061=CARTESIAN_POINT ( 'NONE',  ( 771.1735550268778070, -9.180057203875058747, -316.3353852180827630 ) ) ;
#15062=CARTESIAN_POINT ( 'NONE',  ( 800.7704444035546203, -148.1692326535053610, -326.0291762391768771 ) ) ;
#15064=CARTESIAN_POINT ( 'NONE',  ( 795.1360043628807261, -92.08914811296568814, -360.2193346964456282 ) ) ;
#15065=EDGE_CURVE ( 'NONE', #14459, #33292, #28543, .T. ) ;
#15066=CARTESIAN_POINT ( 'NONE',  ( 793.2243759319678702, -386.5328690171409676, -318.4439275373583200 ) ) ;
#15070=EDGE_LOOP ( 'NONE', ( #21494, #28118, #10303, #40058 ) ) ;
#15077=CARTESIAN_POINT ( 'NONE',  ( 763.8424801807145741, -66.00906357242595845, -320.5453621957614700 ) ) ;
#15079=CARTESIAN_POINT ( 'NONE',  ( 781.8018195045267476, -262.2709662947832499, -365.1927285166407273 ) ) ;
#15082=CARTESIAN_POINT ( 'NONE',  ( 800.0135310231082713, -398.0891481129647218, -325.0180583372163028 ) ) ;
#15083=CARTESIAN_POINT ( 'NONE',  ( 771.1735550268778070, -57.18005720387489532, -316.3353852180827630 ) ) ;
#15089=CARTESIAN_POINT ( 'NONE',  ( 788.8264449731200330, -21.18005720387502677, -363.6646147819171233 ) ) ;
#15092=CARTESIAN_POINT ( 'NONE',  ( 807.2620300519052989, -312.0090635724251911, -318.0141637701419768 ) ) ;
#15096=CARTESIAN_POINT ( 'NONE',  ( 771.1735550268778070, -273.1800572038742985, -316.3353852180827630 ) ) ;
#15098=CARTESIAN_POINT ( 'NONE',  ( 757.4527132478984868, -136.3726999360621051, -329.1273215169538844 ) ) ;
#15100=CARTESIAN_POINT ( 'NONE',  ( 764.3348316497523456, -22.71468719896029853, -308.6759233522265617 ) ) ;
#15101=CARTESIAN_POINT ( 'NONE',  ( 747.2067596250078623, -363.1800572038739006, -352.2312462859687230 ) ) ;
#15107=CARTESIAN_POINT ( 'NONE',  ( 813.2346286133761168, -221.2601417444142271, -328.9521613784389160 ) ) ;
#15109=CARTESIAN_POINT ( 'NONE',  ( 763.0537975583475827, -0.4527844766023628176, -371.0346526505627480 ) ) ;
#15116=CARTESIAN_POINT ( 'NONE',  ( 803.8651313633788504, -5.260141744414903897, -332.4468031744301015 ) ) ;
#15123=CARTESIAN_POINT ( 'NONE',  ( 763.2154366446407039, -309.6237781080502600, -321.4292242960311228 ) ) ;
#15126=CARTESIAN_POINT ( 'NONE',  ( 810.1134526219336749, -320.5328690171411949, -357.8822607201570349 ) ) ;
#15132=CARTESIAN_POINT ( 'NONE',  ( 790.8726784830453198, -82.71468719896012090, -362.5472867521010585 ) ) ;
#15135=CARTESIAN_POINT ( 'NONE',  ( 804.7487373415286811, -187.5436935675108430, -364.7487373415288516 ) ) ;
#15137=CARTESIAN_POINT ( 'NONE',  ( 771.1735550268780344, -129.1800572038746679, -316.3353852180828198 ) ) ;
#15139=CARTESIAN_POINT ( 'NONE',  ( 763.0428371773158460, -419.4636090269702891, -358.7617431975195359 ) ) ;
#15148=CIRCLE ( 'NONE', #40943, 10.00000000000000888 ) ;
#15150=CARTESIAN_POINT ( 'NONE',  ( 761.4292242960306112, -401.4636090269704027, -323.2154366446414429 ) ) ;
#15151=DIRECTION ( 'NONE',  ( 0.000000000000000000, 0.000000000000000000, 1.000000000000000000 ) ) ;
#15152=CARTESIAN_POINT ( 'NONE',  ( 809.0717654672305343, -196.9181544815164386, -360.1688906516309885 ) ) ;
#15156=CARTESIAN_POINT ( 'NONE',  ( 772.3691319403857278, -311.2601417444139429, -315.8894580844506663 ) ) ;
#15158=CARTESIAN_POINT ( 'NONE',  ( 783.7953271457878373, -200.1908817542436907, -375.1787889125761239 ) ) ;
#15164=CARTESIAN_POINT ( 'NONE',  ( 777.4774526936600978, -226.2709662947834488, -304.7301800767028226 ) ) ;
#15166=CARTESIAN_POINT ( 'NONE',  ( 767.8955696845333705, -0.4527844766023628176, -362.1676090361162323 ) ) ;
#15170=CARTESIAN_POINT ( 'NONE',  ( 786.2056067578752163, -131.8055962898690439, -374.4686193811670023 ) ) ;
#15172=CARTESIAN_POINT ( 'NONE',  ( 782.5225473063381969, -358.2709662947829088, -375.2698199232970637 ) ) ;
#15178=CARTESIAN_POINT ( 'NONE',  ( 801.9858362298568863, -411.0783235625954717, -312.7379699480935642 ) ) ;
#15180=CARTESIAN_POINT ( 'NONE',  ( 814.2805881961230625, -1.645427208789804308, -331.2368401574024119 ) ) ;
#15183=VERTEX_POINT ( 'NONE', #30411 ) ;
#15187=CARTESIAN_POINT ( 'NONE',  ( 803.2186876482843445, -199.9874144716870603, -350.0220218866286928 ) ) ;
#15189=CARTESIAN_POINT ( 'NONE',  ( 768.8385539511368734, -239.2601417444141987, -306.4236121716840557 ) ) ;
#15193=CARTESIAN_POINT ( 'NONE',  ( 778.1981804954714335, -82.27096629478388934, -314.8072714833589885 ) ) ;
#15196=CARTESIAN_POINT ( 'NONE',  ( 800.2193346964447755, -138.9982390220563957, -355.1360043628815788 ) ) ;
#15198=CARTESIAN_POINT ( 'NONE',  ( 763.2262854647970016, -32.63460265842044095, -309.2812353651462445 ) ) ;
#15200=CARTESIAN_POINT ( 'NONE',  ( 811.3240766477731540, -436.3726999360612240, -355.6651683502462902 ) ) ;
#15201=AXIS2_PLACEMENT_3D ( 'NONE', #40976, #1276, #29454 ) ;
#15203=CARTESIAN_POINT ( 'NONE',  ( 804.6971507214547046, -315.2817908451525000, -344.0799538623459739 ) ) ;
#15206=CARTESIAN_POINT ( 'NONE',  ( 800.2193346964447755, -282.9982390220558841, -355.1360043628815788 ) ) ;
#15211=CARTESIAN_POINT ( 'NONE',  ( 798.5707757039680246, -293.4636090269707438, -356.7845633553585003 ) ) ;
#15212=CARTESIAN_POINT ( 'NONE',  ( 755.0636971347428243, -292.2709662947831930, -341.7834795799807353 ) ) ;
#15214=CARTESIAN_POINT ( 'NONE',  ( 762.1405469898971887, -169.5436935675108430, -357.8594530101015607 ) ) ;
#15220=CARTESIAN_POINT ( 'NONE',  ( 752.7379699480933368, -84.00906357242590161, -361.9858362298580232 ) ) ;
#15227=CARTESIAN_POINT ( 'NONE',  ( 792.3570229623691148, -141.1800572038746395, -373.1304606946836770 ) ) ;
#15231=CARTESIAN_POINT ( 'NONE',  ( 751.6929314249748586, -270.9982390220561115, -318.8095938919659034 ) ) ;
#15234=CARTESIAN_POINT ( 'NONE',  ( 815.1787889125755555, -318.8965053807775121, -343.7953271457877804 ) ) ;
#15237=CARTESIAN_POINT ( 'NONE',  ( 763.0537975583475827, -360.4527844766010958, -371.0346526505627480 ) ) ;
#15241=CARTESIAN_POINT ( 'NONE',  ( 756.3353852180819104, -413.9073299311465348, -331.1735550268788302 ) ) ;
#15243=CARTESIAN_POINT ( 'NONE',  ( 765.0180583372156207, -216.9982390220562252, -360.0135310231089534 ) ) ;
#15244=CARTESIAN_POINT ( 'NONE',  ( 801.9858362298568863, -75.07832356259649487, -312.7379699480935642 ) ) ;
#15248=CARTESIAN_POINT ( 'NONE',  ( 776.9566956441375396, -228.8965053807778816, -364.8461984189686405 ) ) ;
#15251=CARTESIAN_POINT ( 'NONE',  ( 815.1787889125755555, -54.89650538077837183, -343.7953271457877804 ) ) ;
#15252=CARTESIAN_POINT ( 'NONE',  ( 808.1998602359702772, -452.9681489794448908, -337.6500903519150825 ) ) ;
#15254=CARTESIAN_POINT ( 'NONE',  ( 805.6418435158337843, -341.4636090269705733, -363.8556311672236916 ) ) ;
#15257=CARTESIAN_POINT ( 'NONE',  ( 766.9102291470427417, -186.5545181178801215, -318.6633372737382501 ) ) ;
#15258=CARTESIAN_POINT ( 'NONE',  ( 800.0135310231082713, -182.0891481129654323, -325.0180583372163028 ) ) ;
#15259=CARTESIAN_POINT ( 'NONE',  ( 759.9864689768902508, -386.0891481129647786, -354.9819416627836404 ) ) ;
#15261=CARTESIAN_POINT ( 'NONE',  ( 798.7617431975189675, 20.37622189194865285, -323.0428371773161871 ) ) ;
#15273=CARTESIAN_POINT ( 'NONE',  ( 747.6481478633932056, -421.0999726633340288, -353.4146539503763620 ) ) ;
#15275=CARTESIAN_POINT ( 'NONE',  ( 814.5518280994195948, -15.72551174932958951, -332.4837098697145166 ) ) ;
#15278=CARTESIAN_POINT ( 'NONE',  ( 767.8955696845333705, -408.4527844766009252, -362.1676090361162323 ) ) ;
#15279=CARTESIAN_POINT ( 'NONE',  ( 764.8639956371174549, -8.089148112965974136, -319.7806653035542581 ) ) ;
#15282=CARTESIAN_POINT ( 'NONE',  ( 790.9844846989617508, -262.3726999360617924, -317.2208543904092721 ) ) ;
#15283=VECTOR ( 'NONE', #25357, 1000.000000000000000 ) ;
#15292=CARTESIAN_POINT ( 'NONE',  ( 778.2165204200184689, -310.8164208402377540, -364.9363028652563230 ) ) ;
#15295=CARTESIAN_POINT ( 'NONE',  ( 802.2119215644370342, -54.00906357242601530, -367.5423716828165084 ) ) ;
#15296=CARTESIAN_POINT ( 'NONE',  ( 755.8398074228967971, -115.4419599262327409, -333.4516893846970333 ) ) ;
#15299=CARTESIAN_POINT ( 'NONE',  ( 774.6312213355099630, -23.36187538569318889, -364.6798772138717482 ) ) ;
#15300=CARTESIAN_POINT ( 'NONE',  ( 804.1601925771018387, -127.4419599262326983, -346.5483106153029098 ) ) ;
#15301=CARTESIAN_POINT ( 'NONE',  ( 797.8594530101008786, -133.5436935675110135, -322.1405469898980982 ) ) ;
#15303=CARTESIAN_POINT ( 'NONE',  ( 758.6633372737375112, -428.5328690171409107, -326.9102291470432533 ) ) ;
#15307=ORIENTED_EDGE ( 'NONE', *, *, #45291, .F. ) ;
#15315=CARTESIAN_POINT ( 'NONE',  ( 755.1538015810308480, -86.19088175424408860, -343.0433043558613804 ) ) ;
#15317=CARTESIAN_POINT ( 'NONE',  ( 767.8955696845334842, -288.4527844766014937, -362.1676090361161755 ) ) ;
#15319=CARTESIAN_POINT ( 'NONE',  ( 795.1360043628807261, -404.0891481129646081, -360.2193346964456282 ) ) ;
#15320=CARTESIAN_POINT ( 'NONE',  ( 801.9419747391806368, -66.45278447660216159, -351.9812246680014027 ) ) ;
#15322=PLANE ( 'NONE',  #40325 ) ;
#15324=CARTESIAN_POINT ( 'NONE',  ( 750.9282345327678740, -16.91815448151702839, -319.8311093483690115 ) ) ;
#15327=CARTESIAN_POINT ( 'NONE',  ( 813.5763878283155464, -291.8272453906071746, -351.1614460488615350 ) ) ;
#15330=CARTESIAN_POINT ( 'NONE',  ( 791.9812246680005501, -308.6346026584195670, -361.9419747391813189 ) ) ;
#15332=CARTESIAN_POINT ( 'NONE',  ( 805.2837595273609850, -146.7363362996984506, -340.5290396650784714 ) ) ;
#15334=DIRECTION ( 'NONE',  ( 1.000000000000000000, 0.000000000000000000, 0.000000000000000000 ) ) ;
#15335=CARTESIAN_POINT ( 'NONE',  ( 813.9316612368132837, -7.441959926233078448, -348.6739635108323228 ) ) ;
#15336=CARTESIAN_POINT ( 'NONE',  ( 772.4837098697145166, -335.3618753856921444, -374.5518280994205611 ) ) ;
#15341=CARTESIAN_POINT ( 'NONE',  ( 783.7566961878529810, -240.8965053807777963, -305.1792804349288417 ) ) ;
#15343=CARTESIAN_POINT ( 'NONE',  ( 807.5423716828161105, -441.0783235625953580, -362.2119215644372048 ) ) ;
#15348=CARTESIAN_POINT ( 'NONE',  ( 772.3691319403857278, -23.26014174441484883, -315.8894580844506663 ) ) ;
#15355=CARTESIAN_POINT ( 'NONE',  ( 800.7704444035546203, -316.1692326535048210, -326.0291762391768771 ) ) ;
#15357=UNCERTAINTY_MEASURE_WITH_UNIT (LENGTH_MEASURE( 1.000000000000000082E-05 ), #25332, 'distance_accuracy_value', 'NONE');
#15358=CARTESIAN_POINT ( 'NONE',  ( 746.0683387631852383, -331.4419599262320162, -331.3260364891676204 ) ) ;
#15365=CARTESIAN_POINT ( 'NONE',  ( 751.6929314249748586, -174.9982390220563673, -318.8095938919659034 ) ) ;
#15367=CARTESIAN_POINT ( 'NONE',  ( 774.6858677611749044, -177.7255117493290868, -315.5713283507209894 ) ) ;
#15368=ORIENTED_EDGE ( 'NONE', *, *, #40459, .F. ) ;
#15370=CARTESIAN_POINT ( 'NONE',  ( 798.5707757039680246, -437.4636090269703459, -356.7845633553585003 ) ) ;
#15378=CARTESIAN_POINT ( 'NONE',  ( 775.8780910478218402, -417.2817908451522158, -364.9511171171680530 ) ) ;
#15380=CARTESIAN_POINT ( 'NONE',  ( 776.2046728542105711, -188.1908817542437760, -304.8212110874238761 ) ) ;
#15384=CARTESIAN_POINT ( 'NONE',  ( 798.7617431975189675, -339.6237781080502600, -323.0428371773161871 ) ) ;
#15386=CARTESIAN_POINT ( 'NONE',  ( 760.0363995740630116, -202.9181544815164386, -368.7758568127991907 ) ) ;
#15391=CARTESIAN_POINT ( 'NONE',  ( 777.5031285880264704, -238.8164208402379813, -374.9108240113588408 ) ) ;
#15393=CARTESIAN_POINT ( 'NONE',  ( 804.4286716492782716, -17.36187538569322086, -345.3141322388244703 ) ) ;
#15395=CARTESIAN_POINT ( 'NONE',  ( 793.4146539503750546, -121.9874144716872593, -307.6481478633938877 ) ) ;
#15397=CARTESIAN_POINT ( 'NONE',  ( 767.7687537140311633, -359.9073299311467053, -372.7932403749916830 ) ) ;
#15403=CARTESIAN_POINT ( 'NONE',  ( 767.8955696845333705, -384.4527844766011526, -362.1676090361162323 ) ) ;
#15405=CARTESIAN_POINT ( 'NONE',  ( 763.2262854647970016, -440.6346026584191122, -309.2812353651462445 ) ) ;
#15410=CARTESIAN_POINT ( 'NONE',  ( 796.7845633553578182, -177.6237781080507148, -358.5707757039688204 ) ) ;
#15411=ADVANCED_FACE ( 'NONE', ( #17242 ), #24610, .T. ) ;
#15413=CARTESIAN_POINT ( 'NONE',  ( 781.2497674668890113, -228.3510508353232922, -375.3608509340180603 ) ) ;
#15416=CARTESIAN_POINT ( 'NONE',  ( 781.7834795799800531, -82.81642084023846451, -315.0636971347436202 ) ) ;
#15419=CARTESIAN_POINT ( 'NONE',  ( 767.8955696845333705, -144.4527844766018632, -362.1676090361162323 ) ) ;
#15421=CARTESIAN_POINT ( 'NONE',  ( 751.9810565676468741, -74.08914811296577341, -360.9747183278973921 ) ) ;
#15422=CARTESIAN_POINT ( 'NONE',  ( 759.7806653035535192, -54.99823902205672965, -324.8639956371181370 ) ) ;
#15424=CARTESIAN_POINT ( 'NONE',  ( 804.4086373105744769, -25.64542720878973014, -333.3843516231986541 ) ) ;
#15426=CARTESIAN_POINT ( 'NONE',  ( 793.9708237608222134, -310.9181544815160123, -319.2295555964448681 ) ) ;
#15430=CARTESIAN_POINT ( 'NONE',  ( 791.9812246680005501, -332.6346026584195101, -361.9419747391813189 ) ) ;
#15434=CARTESIAN_POINT ( 'NONE',  ( 790.9844846989617508, -310.3726999360616219, -317.2208543904092721 ) ) ;
#15435=CARTESIAN_POINT ( 'NONE',  ( 792.1044303154645831, -300.4527844766012663, -317.8323909638837677 ) ) ;
#15437=CARTESIAN_POINT ( 'NONE',  ( 788.7366044899766848, -155.9073299311473306, -316.5762568750059813 ) ) ;
#15443=CARTESIAN_POINT ( 'NONE',  ( 791.0478386215596629, -69.82724539060775726, -306.7653713866226326 ) ) ;
#15444=DIRECTION ( 'NONE',  ( 0.000000000000000000, 0.000000000000000000, -1.000000000000000000 ) ) ;
#15450=CARTESIAN_POINT ( 'NONE',  ( 804.7487373415286811, -139.5436935675110135, -364.7487373415288516 ) ) ;
#15453=CARTESIAN_POINT ( 'NONE',  ( 804.1601925771018387, -415.4419599262318457, -346.5483106153029098 ) ) ;
#15455=CARTESIAN_POINT ( 'NONE',  ( 814.5518280994195948, -279.7255117493288026, -332.4837098697145734 ) ) ;
#15458=CARTESIAN_POINT ( 'NONE',  ( 754.0944755984390895, -351.6237781080502032, -364.1009440267246760 ) ) ;
#15460=CARTESIAN_POINT ( 'NONE',  ( 749.2812353651451076, -342.4527844766013231, -323.2262854647983090 ) ) ;
#15465=CARTESIAN_POINT ( 'NONE',  ( 788.8264449731200330, -429.1800572038737869, -363.6646147819171233 ) ) ;
#15466=CARTESIAN_POINT ( 'NONE',  ( 800.2193346964447755, -210.9982390220561967, -355.1360043628815788 ) ) ;
#15467=CARTESIAN_POINT ( 'NONE',  ( 812.6845335610512393, -103.9874144716873161, -353.5525998758768651 ) ) ;
#15472=CARTESIAN_POINT ( 'NONE',  ( 798.7617431975189675, -243.6237781080504590, -323.0428371773161871 ) ) ;
#15474=CARTESIAN_POINT ( 'NONE',  ( 763.2262854647970016, 15.36539734157940629, -309.2812353651462445 ) ) ;
#15475=CARTESIAN_POINT ( 'NONE',  ( 781.2497674668890113, -60.35105083532383219, -375.3608509340180603 ) ) ;
#15478=ORIENTED_EDGE ( 'NONE', *, *, #19296, .T. ) ;
#15479=CARTESIAN_POINT ( 'NONE',  ( 745.1792804349281596, -374.1908817542432075, -343.7566961878542884 ) ) ;
#15482=CARTESIAN_POINT ( 'NONE',  ( 763.0428371773158460, -179.4636090269710849, -358.7617431975195359 ) ) ;
#15483=CARTESIAN_POINT ( 'NONE',  ( 756.3353852180819104, -173.9073299311472169, -331.1735550268788302 ) ) ;
#15484=CARTESIAN_POINT ( 'NONE',  ( 781.7834795799800531, -394.8164208402374697, -315.0636971347436202 ) ) ;
#15486=CARTESIAN_POINT ( 'NONE',  ( 787.6308680596127942, 12.73985825558503926, -364.1105419155492768 ) ) ;
#15495=CARTESIAN_POINT ( 'NONE',  ( 795.8262568251477660, -430.3726999360611671, -308.3538107759623585 ) ) ;
#15496=CARTESIAN_POINT ( 'NONE',  ( 772.4837098697145166, -23.36187538569319244, -374.5518280994205611 ) ) ;
#15498=CARTESIAN_POINT ( 'NONE',  ( 759.7806653035534055, -390.9982390220557136, -324.8639956371180801 ) ) ;
#15499=CARTESIAN_POINT ( 'NONE',  ( 754.8072714833583632, -4.816420840238714085, -338.1981804954721156 ) ) ;
#15502=CARTESIAN_POINT ( 'NONE',  ( 790.0220218866281812, -247.0999726633344835, -363.2186876482849129 ) ) ;
#15503=CARTESIAN_POINT ( 'NONE',  ( 745.7998596910086917, -149.3618753856928265, -332.5602148656461168 ) ) ;
#15506=CARTESIAN_POINT ( 'NONE',  ( 776.3558828440975503, 16.45630643248848557, -314.5934542695748064 ) ) ;
#15511=CARTESIAN_POINT ( 'NONE',  ( 758.0580252608178853, -318.4527844766014368, -328.0187753319985404 ) ) ;
#15513=CARTESIAN_POINT ( 'NONE',  ( 760.0363995740630116, -106.9181544815167371, -368.7758568127991907 ) ) ;
#15514=CARTESIAN_POINT ( 'NONE',  ( 769.1273215169530886, -118.7146871989600072, -317.4527132478988847 ) ) ;
#15517=CARTESIAN_POINT ( 'NONE',  ( 803.4237431249931660, -15.18005720387504631, -331.2633955100225194 ) ) ;
#15518=CARTESIAN_POINT ( 'NONE',  ( 780.5290396650775619, -132.3510508353235764, -365.2837595273619513 ) ) ;
#15519=CARTESIAN_POINT ( 'NONE',  ( 803.6646147819161570, -137.9073299311473875, -348.8264449731210561 ) ) ;
#15521=CARTESIAN_POINT ( 'NONE',  ( 764.0069404352550464, -423.0783235625953580, -359.2566176426627180 ) ) ;
#15527=ORIENTED_EDGE ( 'NONE', *, *, #40142, .F. ) ;
#15532=CARTESIAN_POINT ( 'NONE',  ( 802.9823548866075953, -97.09997266333496668, -330.0799878456151077 ) ) ;
#15533=CARTESIAN_POINT ( 'NONE',  ( 774.6858677611749044, -273.7255117493288026, -315.5713283507209894 ) ) ;
#15535=CARTESIAN_POINT ( 'NONE',  ( 758.0580252608178853, -390.4527844766011526, -328.0187753319985404 ) ) ;
#15536=CARTESIAN_POINT ( 'NONE',  ( 804.6798772138708955, -39.72551174932951312, -334.6312213355107019 ) ) ;
#15540=CARTESIAN_POINT ( 'NONE',  ( 804.1009440267234822, -23.46360902697155026, -314.0944755984392600 ) ) ;
#15543=CARTESIAN_POINT ( 'NONE',  ( 781.2370466360911223, -308.7363362996979390, -304.9990715423533629 ) ) ;
#15546=CARTESIAN_POINT ( 'NONE',  ( 768.0187753319979720, -296.6346026584195670, -318.0580252608186242 ) ) ;
#15547=LINE ( 'NONE', #30293, #1565 ) ;
#15548=CARTESIAN_POINT ( 'NONE',  ( 763.8424801807145741, -162.0090635724256742, -320.5453621957614700 ) ) ;
#15550=CARTESIAN_POINT ( 'NONE',  ( 810.1134526219336749, -8.532869017142163059, -357.8822607201570349 ) ) ;
#15551=CARTESIAN_POINT ( 'NONE',  ( 792.2312462859673587, -347.9073299311467053, -307.2067596250082602 ) ) ;
#15556=CARTESIAN_POINT ( 'NONE',  ( 793.4146539503750546, -433.9874144716862361, -307.6481478633938877 ) ) ;
#15561=CARTESIAN_POINT ( 'NONE',  ( 766.7756240680305382, -14.53286901714214707, -361.5560724626415663 ) ) ;
#15566=CARTESIAN_POINT ( 'NONE',  ( 794.1144889064781864, -322.1692326535048210, -360.9840315886528401 ) ) ;
#15568=CARTESIAN_POINT ( 'NONE',  ( 813.9316612368132837, -343.4419599262320162, -348.6739635108323228 ) ) ;
#15576=CARTESIAN_POINT ( 'NONE',  ( 745.7998596910086917, -173.3618753856927128, -332.5602148656461168 ) ) ;
#15579=CARTESIAN_POINT ( 'NONE',  ( 759.9864689768902508, -170.0891481129654608, -354.9819416627836404 ) ) ;
#15581=CARTESIAN_POINT ( 'NONE',  ( 790.0220218866281812, -439.0999726633339719, -363.2186876482849129 ) ) ;
#15587=CARTESIAN_POINT ( 'NONE',  ( 755.5913626894240451, -421.6454272087885329, -346.6156483768012890 ) ) ;
#15589=CARTESIAN_POINT ( 'NONE',  ( 814.8207195650702488, -194.1908817542437475, -336.2433038121456548 ) ) ;
#15592=CARTESIAN_POINT ( 'NONE',  ( 794.9819416627830151, -204.9982390220562820, -319.9864689768909898 ) ) ;
#15593=CARTESIAN_POINT ( 'NONE',  ( 802.7791456095903868, -316.7146871989593819, -329.0155153010375102 ) ) ;
#15595=CARTESIAN_POINT ( 'NONE',  ( 814.4686193811664907, -219.2817908451527558, -346.2056067578752732 ) ) ;
#15598=CARTESIAN_POINT ( 'NONE',  ( 798.5707757039680246, -53.46360902697146855, -356.7845633553585003 ) ) ;
#15600=CARTESIAN_POINT ( 'NONE',  ( 782.5225473063383106, -238.2709662947833920, -375.2698199232970637 ) ) ;
#15602=CARTESIAN_POINT ( 'NONE',  ( 755.0636971347428243, -28.27096629478409540, -341.7834795799807353 ) ) ;
#15604=CARTESIAN_POINT ( 'NONE',  ( 811.6461892240364477, -148.7146871989598935, -324.1737431748509835 ) ) ;
#15606=CARTESIAN_POINT ( 'NONE',  ( 763.0537975583475827, -384.4527844766011526, -371.0346526505627480 ) ) ;
#15611=CARTESIAN_POINT ( 'NONE',  ( 797.6776695296629214, -379.5436935675102745, -357.6776695296636603 ) ) ;
#15613=CARTESIAN_POINT ( 'NONE',  ( 796.9462024416508257, -444.4527844766009821, -308.9653473494370246 ) ) ;
#15618=ADVANCED_FACE ( 'NONE', ( #45668, #42184 ), #3151, .F. ) ;
#15619=CARTESIAN_POINT ( 'NONE',  ( 773.3843516231979720, -229.4419599262323572, -364.4086373105754433 ) ) ;
#15622=CARTESIAN_POINT ( 'NONE',  ( 815.0009284576459549, -222.3510508353233206, -338.7629533639073429 ) ) ;
#15627=CARTESIAN_POINT ( 'NONE',  ( 748.9653473494363425, -74.63460265842032015, -356.9462024416521331 ) ) ;
#15629=CARTESIAN_POINT ( 'NONE',  ( 755.0636971347428243, -76.27096629478394618, -341.7834795799807353 ) ) ;
#15631=CARTESIAN_POINT ( 'NONE',  ( 766.0291762391763086, -10.91815448151704793, -360.7704444035551319 ) ) ;
#15633=CARTESIAN_POINT ( 'NONE',  ( 755.3028492785439312, -303.2817908451525000, -335.9200461376539693 ) ) ;
#15640=CARTESIAN_POINT ( 'NONE',  ( 755.8894580844503253, -327.8272453906069472, -332.3691319403863531 ) ) ;
#15641=CARTESIAN_POINT ( 'NONE',  ( 785.3687786644884454, -323.3618753856923149, -315.3201227861279676 ) ) ;
#15642=CARTESIAN_POINT ( 'NONE',  ( 803.4237431249931660, -159.1800572038746111, -331.2633955100225194 ) ) ;
#15649=CARTESIAN_POINT ( 'NONE',  ( 815.3608509340175488, -122.7363362996985074, -341.2497674668889545 ) ) ;
#15657=CARTESIAN_POINT ( 'NONE',  ( 782.5225473063383106, -142.2709662947837330, -375.2698199232970637 ) ) ;
#15660=CARTESIAN_POINT ( 'NONE',  ( 813.1304606946830518, -257.9073299311469896, -352.3570229623690580 ) ) ;
#15661=CARTESIAN_POINT ( 'NONE',  ( 814.5518280994195948, -447.7255117493281205, -332.4837098697145166 ) ) ;
#15663=CARTESIAN_POINT ( 'NONE',  ( 745.1769319972822814, -329.8055962898683902, -346.2694204179732083 ) ) ;
#15664=CARTESIAN_POINT ( 'NONE',  ( 763.2262854647970016, -80.63460265842029173, -309.2812353651462445 ) ) ;
#15667=CARTESIAN_POINT ( 'NONE',  ( 813.1304606946830518, -353.9073299311467053, -352.3570229623690580 ) ) ;
#15672=CARTESIAN_POINT ( 'NONE',  ( 788.8264449731200330, -213.1800572038743553, -363.6646147819171233 ) ) ;
#15674=CARTESIAN_POINT ( 'NONE',  ( 800.1688906516307043, -106.1692326535054889, -369.0717654672308186 ) ) ;
#15678=CARTESIAN_POINT ( 'NONE',  ( 787.6308680596127942, -251.2601417444141134, -364.1105419155492768 ) ) ;
#15682=CARTESIAN_POINT ( 'NONE',  ( 791.1614460488616487, -419.2601417444136587, -373.5763878283158874 ) ) ;
#15683=CARTESIAN_POINT ( 'NONE',  ( 805.9055244015594326, -75.62377810805104161, -315.8990559732753240 ) ) ;
#15687=CARTESIAN_POINT ( 'NONE',  ( 811.3240766477731540, -364.3726999360614514, -355.6651683502462902 ) ) ;
#15688=CARTESIAN_POINT ( 'NONE',  ( 785.3687786644884454, -227.3618753856925707, -315.3201227861279676 ) ) ;
#15691=CARTESIAN_POINT ( 'NONE',  ( 802.9823548866075953, -217.0999726633345972, -330.0799878456151077 ) ) ;
#15692=CARTESIAN_POINT ( 'NONE',  ( 788.8264449731200330, -189.1800572038744122, -363.6646147819171233 ) ) ;
#15693=CARTESIAN_POINT ( 'NONE',  ( 803.6646147819162707, -377.9073299311465917, -348.8264449731211130 ) ) ;
#15694=ORIENTED_EDGE ( 'NONE', *, *, #25580, .F. ) ;
#15696=CARTESIAN_POINT ( 'NONE',  ( 794.9819416627830151, -108.9982390220565804, -319.9864689768909898 ) ) ;
#15701=CARTESIAN_POINT ( 'NONE',  ( 799.9999999999993179, -512.9681489794448908, -339.9999999999999432 ) ) ;
#15705=CARTESIAN_POINT ( 'NONE',  ( 761.4292242960306112, 6.536390973028352924, -323.2154366446414429 ) ) ;
#15707=CARTESIAN_POINT ( 'NONE',  ( 814.9108240113580450, -40.27096629478405987, -337.5031285880265273 ) ) ;
#15710=CARTESIAN_POINT ( 'NONE',  ( 797.8594530101008786, -397.5436935675100472, -322.1405469898980982 ) ) ;
#15711=CARTESIAN_POINT ( 'NONE',  ( 778.2165204200184689, -22.81642084023865280, -364.9363028652563230 ) ) ;
#15714=CARTESIAN_POINT ( 'NONE',  ( 793.9708237608222134, -262.9181544815162965, -319.2295555964448681 ) ) ;
#15715=CARTESIAN_POINT ( 'NONE',  ( 808.0189434323515343, -158.0891481129655176, -319.0252816721025511 ) ) ;
#15718=CARTESIAN_POINT ( 'NONE',  ( 770.7832876896738981, 16.45630643248850333, -316.4833103687052471 ) ) ;
#15722=CARTESIAN_POINT ( 'NONE',  ( 794.9819416627830151, -324.9982390220559409, -319.9864689768909898 ) ) ;
#15724=CARTESIAN_POINT ( 'NONE',  ( 762.1177392798416577, -114.5545181178803631, -309.8865473780659272 ) ) ;
#15725=CARTESIAN_POINT ( 'NONE',  ( 763.2154366446407039, -117.6237781080509279, -321.4292242960311228 ) ) ;
#15728=CARTESIAN_POINT ( 'NONE',  ( 778.1981804954714335, -34.27096629478407408, -314.8072714833589885 ) ) ;
#15729=CARTESIAN_POINT ( 'NONE',  ( 786.6156483768007774, -121.4419599262327267, -315.5913626894246136 ) ) ;
#15730=CARTESIAN_POINT ( 'NONE',  ( 803.4237431249931660, -135.1800572038746679, -331.2633955100225194 ) ) ;
#15732=CARTESIAN_POINT ( 'NONE',  ( 789.6640940660590786, -442.9180389616178672, -363.1300863558843162 ) ) ;
#15740=CARTESIAN_POINT ( 'NONE',  ( 748.6759233522253680, -280.3726999360616787, -324.3348316497537098 ) ) ;
#15747=CARTESIAN_POINT ( 'NONE',  ( 779.4763451958990572, -104.7363362996985785, -365.0264073115438919 ) ) ;
#15748=CARTESIAN_POINT ( 'NONE',  ( 757.8323909638828582, -290.6346026584196238, -352.1044303154654358 ) ) ;
#15749=VERTEX_POINT ( 'NONE', #11012 ) ;
#15750=CARTESIAN_POINT ( 'NONE',  ( 791.9812246680005501, -380.6346026584192828, -361.9419747391813189 ) ) ;
#15751=CARTESIAN_POINT ( 'NONE',  ( 785.3687786644884454, -83.36187538569296862, -315.3201227861279676 ) ) ;
#15754=DIRECTION ( 'NONE',  ( 0.000000000000000000, 0.000000000000000000, 1.000000000000000000 ) ) ;
#15756=CARTESIAN_POINT ( 'NONE',  ( 766.4474001241216001, -19.09997266333520116, -307.3154664389482491 ) ) ;
#15759=CARTESIAN_POINT ( 'NONE',  ( 786.2694204179717872, -309.2817908451525568, -305.1769319972829067 ) ) ;
#15762=CARTESIAN_POINT ( 'NONE',  ( 792.1044303154645831, -276.4527844766013800, -317.8323909638837677 ) ) ;
#15764=CARTESIAN_POINT ( 'NONE',  ( 784.1219089521767955, -165.2817908451529547, -315.0488828828318333 ) ) ;
#15768=CARTESIAN_POINT ( 'NONE',  ( 772.5602148656447525, -345.7255117493285184, -305.7998596910095443 ) ) ;
#15774=CARTESIAN_POINT ( 'NONE',  ( 767.6429770376289525, 14.81994279612486309, -306.8695393053162093 ) ) ;
#15779=CARTESIAN_POINT ( 'NONE',  ( 765.8855110935204493, 1.830767346494167391, -319.0159684113471599 ) ) ;
#15784=ORIENTED_EDGE ( 'NONE', *, *, #18463, .T. ) ;
#15785=CARTESIAN_POINT ( 'NONE',  ( 796.7845633553578182, -345.6237781080501463, -358.5707757039688204 ) ) ;
#15788=CARTESIAN_POINT ( 'NONE',  ( 814.8230680027162407, -317.8055962898684470, -333.7305795820267917 ) ) ;
#15792=ORIENTED_EDGE ( 'NONE', *, *, #30587, .F. ) ;
#15793=CARTESIAN_POINT ( 'NONE',  ( 767.6429770376289525, -177.1800572038744690, -306.8695393053162093 ) ) ;
#15796=CARTESIAN_POINT ( 'NONE',  ( 774.6312213355098493, -167.3618753856927412, -364.6798772138717482 ) ) ;
#15799=CARTESIAN_POINT ( 'NONE',  ( 790.0220218866281812, -415.0999726633340288, -363.2186876482849129 ) ) ;
#15803=DIRECTION ( 'NONE',  ( 0.000000000000000000, 0.000000000000000000, -1.000000000000000000 ) ) ;
#15806=CARTESIAN_POINT ( 'NONE',  ( 786.5483106153019435, -439.6454272087884760, -364.1601925771022366 ) ) ;
#15808=CARTESIAN_POINT ( 'NONE',  ( 814.4686193811664907, -195.2817908451528410, -346.2056067578752732 ) ) ;
#15812=CARTESIAN_POINT ( 'NONE',  ( 755.0636971347428243, -172.2709662947836478, -341.7834795799807353 ) ) ;
#15813=CARTESIAN_POINT ( 'NONE',  ( 754.8983024940795303, -378.8965053807772847, -336.9254006560228163 ) ) ;
#15815=CARTESIAN_POINT ( 'NONE',  ( 768.9521613784389729, -225.8272453906072599, -373.2346286133773106 ) ) ;
#15818=CARTESIAN_POINT ( 'NONE',  ( 760.7433823573367135, -60.00906357242598688, -355.9930595647440441 ) ) ;
#15821=CARTESIAN_POINT ( 'NONE',  ( 810.7187646348534145, -258.4527844766016074, -356.7737145352016341 ) ) ;
#15824=CARTESIAN_POINT ( 'NONE',  ( 792.1044303154645831, -36.45278447660223975, -317.8323909638837677 ) ) ;
#15826=CARTESIAN_POINT ( 'NONE',  ( 814.8230680027162407, -149.8055962898689870, -333.7305795820267917 ) ) ;
#15828=CARTESIAN_POINT ( 'NONE',  ( 815.2698199232961542, -376.8164208402375834, -342.5225473063383106 ) ) ;
#15833=CARTESIAN_POINT ( 'NONE',  ( 765.0180583372156207, -384.9982390220556567, -360.0135310231089534 ) ) ;
#15836=CARTESIAN_POINT ( 'NONE',  ( 757.7880784355613741, 5.990936427573807954, -312.4576283171834916 ) ) ;
#15841=CARTESIAN_POINT ( 'NONE',  ( 760.5453621957607311, -213.0783235625960401, -323.8424801807151425 ) ) ;
#15843=CARTESIAN_POINT ( 'NONE',  ( 783.7566961878529810, -216.8965053807778816, -305.1792804349288417 ) ) ;
#15844=LINE ( 'NONE', #2434, #4679 ) ;
#15851=CARTESIAN_POINT ( 'NONE',  ( 805.0032342141412300, -61.54369356751124087, -314.9967657858571783 ) ) ;
#15854=CARTESIAN_POINT ( 'NONE',  ( 771.1735550268780344, -81.18005720387482427, -316.3353852180828198 ) ) ;
#15856=CARTESIAN_POINT ( 'NONE',  ( 754.7162404726377645, -14.73633629969885384, -339.4709603349214717 ) ) ;
#15858=CARTESIAN_POINT ( 'NONE',  ( 796.9571628226829034, -311.4636090269706870, -321.2382568024804641 ) ) ;
#15866=CARTESIAN_POINT ( 'NONE',  ( 786.5483106153019435, -319.6454272087888739, -364.1601925771022366 ) ) ;
#15867=CARTESIAN_POINT ( 'NONE',  ( 781.8018195045266339, -334.2709662947829656, -365.1927285166406705 ) ) ;
#15868=CARTESIAN_POINT ( 'NONE',  ( 804.9363028652555840, -136.2709662947837330, -338.2165204200192079 ) ) ;
#15874=CARTESIAN_POINT ( 'NONE',  ( 760.0363995740630116, -130.9181544815166660, -368.7758568127991907 ) ) ;
#15882=CARTESIAN_POINT ( 'NONE',  ( 745.4481719005789273, -147.7255117493291721, -347.5162901302853697 ) ) ;
#15883=CARTESIAN_POINT ( 'NONE',  ( 799.9999999999993179, 205.0000000000000568, -360.0000000000000000 ) ) ;
#15886=CARTESIAN_POINT ( 'NONE',  ( 801.1904061080336987, -260.0891481129650060, -368.3070685750235498 ) ) ;
#15889=CARTESIAN_POINT ( 'NONE',  ( 746.8695393053151292, -437.9073299311464211, -327.6429770376306578 ) ) ;
#15891=CARTESIAN_POINT ( 'NONE',  ( 773.7943932421234194, -335.8055962898683902, -305.5313806188329409 ) ) ;
#15892=CARTESIAN_POINT ( 'NONE',  ( 796.9462024416508257, -84.45278447660206211, -308.9653473494370246 ) ) ;
#15894=CARTESIAN_POINT ( 'NONE',  ( 772.4837098697144029, -359.3618753856920875, -374.5518280994205611 ) ) ;
#15898=CARTESIAN_POINT ( 'NONE',  ( 786.2056067578752163, -131.8055962898690439, -374.4686193811670023 ) ) ;
#15905=CARTESIAN_POINT ( 'NONE',  ( 765.8855110935204493, 1.830767346494167391, -319.0159684113471599 ) ) ;
#15907=CARTESIAN_POINT ( 'NONE',  ( 800.1688906516307043, -418.1692326535044799, -369.0717654672308186 ) ) ;
#15909=VERTEX_POINT ( 'NONE', #39193 ) ;
#15911=CARTESIAN_POINT ( 'NONE',  ( 778.7629533639073998, -392.7363362996977116, -375.0009284576466371 ) ) ;
#15914=CARTESIAN_POINT ( 'NONE',  ( 771.2633955100217236, -239.9073299311470748, -363.4237431249939618 ) ) ;
#15918=CARTESIAN_POINT ( 'NONE',  ( 758.4439275373578084, -228.5545181178799794, -353.2243759319684386 ) ) ;
#15919=CARTESIAN_POINT ( 'NONE',  ( 804.6798772138708955, -231.7255117493288310, -334.6312213355107019 ) ) ;
#15920=CARTESIAN_POINT ( 'NONE',  ( 756.3353852180820240, -389.9073299311465917, -331.1735550268787733 ) ) ;
#15921=ORIENTED_EDGE ( 'NONE', *, *, #6544, .T. ) ;
#15923=CARTESIAN_POINT ( 'NONE',  ( 803.6646147819161570, -89.90732993114750116, -348.8264449731210561 ) ) ;
#15934=CARTESIAN_POINT ( 'NONE',  ( 804.1009440267234822, -431.4636090269702322, -314.0944755984392600 ) ) ;
#15935=CARTESIAN_POINT ( 'NONE',  ( 782.5225473063383106, -46.27096629478403855, -375.2698199232970637 ) ) ;
#15938=CARTESIAN_POINT ( 'NONE',  ( 781.8018195045266339, -382.2709662947828519, -365.1927285166406705 ) ) ;
#15939=CARTESIAN_POINT ( 'NONE',  ( 774.6312213355098493, -23.36187538569319244, -364.6798772138717482 ) ) ;
#15943=CARTESIAN_POINT ( 'NONE',  ( 755.5913626894240451, -301.6454272087889308, -346.6156483768012890 ) ) ;
#15945=CARTESIAN_POINT ( 'NONE',  ( 751.6929314249748586, -174.9982390220563673, -318.8095938919659034 ) ) ;
#15949=CARTESIAN_POINT ( 'NONE',  ( 793.3891180349545493, 16.45630643248849978, -314.6660875939051607 ) ) ;
#15954=CARTESIAN_POINT ( 'NONE',  ( 771.1735550268778070, -345.1800572038739006, -316.3353852180827630 ) ) ;
#15956=CARTESIAN_POINT ( 'NONE',  ( 799.9636004259356241, -94.91815448151677970, -311.2241431872006956 ) ) ;
#15957=CARTESIAN_POINT ( 'NONE',  ( 800.7704444035546203, -124.1692326535054463, -326.0291762391768771 ) ) ;
#15961=ADVANCED_FACE ( 'NONE', ( #43327, #39880 ), #32252, .F. ) ;
#15963=CARTESIAN_POINT ( 'NONE',  ( 785.3687786644884454, -35.36187538569316047, -315.3201227861279676 ) ) ;
#15964=CARTESIAN_POINT ( 'NONE',  ( 801.3366627262608972, -128.5328690171417634, -353.0897708529566899 ) ) ;
#15965=CARTESIAN_POINT ( 'NONE',  ( 805.1927285166397041, -136.8164208402382371, -341.8018195045277707 ) ) ;
#15967=CARTESIAN_POINT ( 'NONE',  ( 798.0661480581538854, 21.46713098285774279, -309.5768839229118043 ) ) ;
#15972=CARTESIAN_POINT ( 'NONE',  ( 795.8262568251477660, -286.3726999360617356, -308.3538107759623585 ) ) ;
#15980=CARTESIAN_POINT ( 'NONE',  ( 780.5236548040995785, -116.7363362996985217, -314.9735926884559944 ) ) ;
#15982=CARTESIAN_POINT ( 'NONE',  ( 797.6776695296629214, -115.5436935675110988, -357.6776695296636603 ) ) ;
#15983=CARTESIAN_POINT ( 'NONE',  ( 758.0580252608178853, -294.4527844766013800, -328.0187753319985404 ) ) ;
#15986=CARTESIAN_POINT ( 'NONE',  ( 781.7834795799800531, -418.8164208402374129, -315.0636971347436202 ) ) ;
#15987=CARTESIAN_POINT ( 'NONE',  ( 762.3223304703356007, -79.54369356751119824, -322.3223304703362828 ) ) ;
#15995=ORIENTED_EDGE ( 'NONE', *, *, #7399, .T. ) ;
#15996=CARTESIAN_POINT ( 'NONE',  ( 799.9636004259356241, -358.9181544815160123, -311.2241431872006956 ) ) ;
#15999=CARTESIAN_POINT ( 'NONE',  ( 756.3353852180819104, -293.9073299311468759, -331.1735550268788302 ) ) ;
#16000=CARTESIAN_POINT ( 'NONE',  ( 779.4763451958990572, -200.7363362996982801, -365.0264073115438919 ) ) ;
#16003=CARTESIAN_POINT ( 'NONE',  ( 811.0346526505617248, -398.6346026584193396, -323.0537975583478101 ) ) ;
#16009=CARTESIAN_POINT ( 'NONE',  ( 745.7998596910086917, -29.36187538569318178, -332.5602148656461168 ) ) ;
#16010=AXIS2_PLACEMENT_3D ( 'NONE', #9406, #37349, #40814 ) ;
#16015=CARTESIAN_POINT ( 'NONE',  ( 754.9735926884551418, -18.35105083532395298, -340.5236548041000333 ) ) ;
#16020=VERTEX_POINT ( 'NONE', #12580 ) ;
#16021=CARTESIAN_POINT ( 'NONE',  ( 804.4286716492782716, -41.36187538569314626, -345.3141322388244703 ) ) ;
#16022=CARTESIAN_POINT ( 'NONE',  ( 765.8855110935204493, -334.1692326535047073, -319.0159684113471599 ) ) ;
#16025=CARTESIAN_POINT ( 'NONE',  ( 813.2346286133761168, -341.2601417444138292, -328.9521613784389160 ) ) ;
#16030=CARTESIAN_POINT ( 'NONE',  ( 759.0252816721024374, -192.9982390220562820, -368.0189434323527280 ) ) ;
#16032=VERTEX_POINT ( 'NONE', #1712 ) ;
#16033=CARTESIAN_POINT ( 'NONE',  ( 801.9419747391806368, -186.4527844766017779, -351.9812246680014027 ) ) ;
#16035=CARTESIAN_POINT ( 'NONE',  ( 761.4292242960306112, -449.4636090269702322, -323.2154366446414429 ) ) ;
#16041=APPLICATION_CONTEXT ( 'automotive_design' ) ;
#16042=CARTESIAN_POINT ( 'NONE',  ( 793.0897708529556667, -414.5545181178795247, -361.3366627262616362 ) ) ;
#16044=CARTESIAN_POINT ( 'NONE',  ( 788.6739635108323228, -223.6454272087891013, -373.9316612368139090 ) ) ;
#16046=CIRCLE ( 'NONE', #35971, 10.00000000000000888 ) ;
#16048=CARTESIAN_POINT ( 'NONE',  ( 756.3353852180819104, -173.9073299311472169, -331.1735550268788302 ) ) ;
#16049=CARTESIAN_POINT ( 'NONE',  ( 805.0264073115434940, -366.3510508353228374, -339.4763451958999099 ) ) ;
#16051=CARTESIAN_POINT ( 'NONE',  ( 749.5768839229115201, -228.5545181178799794, -358.0661480581553064 ) ) ;
#16054=CARTESIAN_POINT ( 'NONE',  ( 775.8780910478218402, -33.28179084515333130, -364.9511171171680530 ) ) ;
#16056=CARTESIAN_POINT ( 'NONE',  ( 800.9747183278959710, -252.9982390220560831, -311.9810565676471583 ) ) ;
#16058=DIRECTION ( 'NONE',  ( 0.000000000000000000, 0.000000000000000000, -1.000000000000000000 ) ) ;
#16060=CARTESIAN_POINT ( 'NONE',  ( 781.7834795799800531, -58.81642084023854267, -315.0636971347436202 ) ) ;
#16062=CARTESIAN_POINT ( 'NONE',  ( 748.3538107759620743, -136.7146871989600072, -355.8262568251490165 ) ) ;
#16064=CARTESIAN_POINT ( 'NONE',  ( 792.3570229623688874, -381.1800572038737869, -373.1304606946836202 ) ) ;
#16068=CARTESIAN_POINT ( 'NONE',  ( 778.2165204200184689, -406.8164208402375266, -364.9363028652563230 ) ) ;
#16070=CARTESIAN_POINT ( 'NONE',  ( 754.3581564841646241, 6.536390973028352924, -316.1443688327762516 ) ) ;
#16074=CARTESIAN_POINT ( 'NONE',  ( 790.8726784830453198, -226.7146871989596661, -362.5472867521010585 ) ) ;
#16076=CARTESIAN_POINT ( 'NONE',  ( 778.7502325331095108, -216.3510508353233490, -304.6391490659818828 ) ) ;
#16082=CARTESIAN_POINT ( 'NONE',  ( 805.1927285166397041, -184.8164208402380950, -341.8018195045277707 ) ) ;
#16084=CARTESIAN_POINT ( 'NONE',  ( 808.3070685750230950, -66.99823902205672255, -361.1904061080339261 ) ) ;
#16085=CARTESIAN_POINT ( 'NONE',  ( 767.8955696845334842, -72.45278447660213317, -362.1676090361161755 ) ) ;
#16087=CARTESIAN_POINT ( 'NONE',  ( 790.9844846989617508, 1.627300063937458408, -317.2208543904092721 ) ) ;
#16089=CARTESIAN_POINT ( 'NONE',  ( 800.9840315886518738, -364.9181544815158986, -354.1144889064786412 ) ) ;
#16096=CARTESIAN_POINT ( 'NONE',  ( 802.9823548866075953, -337.0999726633342561, -330.0799878456151077 ) ) ;
#16097=CARTESIAN_POINT ( 'NONE',  ( 797.6776695296629214, -307.5436935675104451, -357.6776695296636603 ) ) ;
#16098=CARTESIAN_POINT ( 'NONE',  ( 788.8264449731200330, -165.1800572038745258, -363.6646147819171233 ) ) ;
#16103=CARTESIAN_POINT ( 'NONE',  ( 780.5290396650775619, -276.3510508353231785, -365.2837595273619513 ) ) ;
#16104=CARTESIAN_POINT ( 'NONE',  ( 764.1737431748507561, -130.3726999360621619, -371.6461892240376415 ) ) ;
#16110=CARTESIAN_POINT ( 'NONE',  ( 814.5518280994195948, -135.7255117493291721, -332.4837098697145166 ) ) ;
#16113=CARTESIAN_POINT ( 'NONE',  ( 745.4481719005789273, -267.7255117493286320, -347.5162901302853129 ) ) ;
#16117=CARTESIAN_POINT ( 'NONE',  ( 746.0683387631852383, -331.4419599262320162, -331.3260364891676204 ) ) ;
#16118=CARTESIAN_POINT ( 'NONE',  ( 782.5225473063381969, -94.27096629478386092, -375.2698199232970637 ) ) ;
#16120=CARTESIAN_POINT ( 'NONE',  ( 749.2812353651451076, -366.4527844766012095, -323.2262854647983090 ) ) ;
#16125=CARTESIAN_POINT ( 'NONE',  ( 773.7943932421234194, -119.8055962898690865, -305.5313806188329409 ) ) ;
#16130=CARTESIAN_POINT ( 'NONE',  ( 769.1273215169530886, 1.285312801039623753, -317.4527132478988847 ) ) ;
#16132=CARTESIAN_POINT ( 'NONE',  ( 801.9858362298568863, -435.0783235625953580, -312.7379699480935642 ) ) ;
#16136=CARTESIAN_POINT ( 'NONE',  ( 773.7305795820266212, -393.2817908451522726, -374.8230680027170365 ) ) ;
#16138=CARTESIAN_POINT ( 'NONE',  ( 755.3201227861273992, -243.7255117493287742, -345.3687786644892981 ) ) ;
#16143=CARTESIAN_POINT ( 'NONE',  ( 769.0155153010367712, -226.3726999360617924, -362.7791456095907279 ) ) ;
#16144=CARTESIAN_POINT ( 'NONE',  ( 794.9819416627830151, -228.9982390220561683, -319.9864689768909898 ) ) ;
#16145=CARTESIAN_POINT ( 'NONE',  ( 788.7366044899766848, -419.9073299311465348, -316.5762568750059813 ) ) ;
#16148=CARTESIAN_POINT ( 'NONE',  ( 781.8018195045266339, -94.27096629478386092, -365.1927285166406705 ) ) ;
#16153=FACE_OUTER_BOUND ( 'NONE', #3083, .T. ) ;
#16157=CARTESIAN_POINT ( 'NONE',  ( 750.9282345327678740, -448.9181544815156144, -319.8311093483690115 ) ) ;
#16158=CARTESIAN_POINT ( 'NONE',  ( 758.8095938919644823, -32.08914811296589420, -311.6929314249762797 ) ) ;
#16160=CARTESIAN_POINT ( 'NONE',  ( 801.9419747391806368, -402.4527844766010389, -351.9812246680014027 ) ) ;
#16161=CARTESIAN_POINT ( 'NONE',  ( 800.2193346964446619, -18.99823902205684689, -355.1360043628816925 ) ) ;
#16164=CARTESIAN_POINT ( 'NONE',  ( 755.3028492785439312, -279.2817908451526137, -335.9200461376539693 ) ) ;
#16165=CARTESIAN_POINT ( 'NONE',  ( 796.7737145352015204, -164.6346026584200217, -370.7187646348536987 ) ) ;
#16170=CARTESIAN_POINT ( 'NONE',  ( 761.9338519418445230, -254.5328690171413655, -370.4231160770881957 ) ) ;
#16175=CARTESIAN_POINT ( 'NONE',  ( 759.7806653035534055, -366.9982390220556567, -324.8639956371180801 ) ) ;
#16177=CARTESIAN_POINT ( 'NONE',  ( 744.6391490659812007, -110.7363362996985501, -338.7502325331110455 ) ) ;
#16178=CARTESIAN_POINT ( 'NONE',  ( 769.1273215169530886, -166.7146871989598367, -317.4527132478988847 ) ) ;
#16181=CARTESIAN_POINT ( 'NONE',  ( 762.3223304703356007, -55.54369356751127640, -322.3223304703362828 ) ) ;
#16182=CARTESIAN_POINT ( 'NONE',  ( 803.2186876482843445, -175.9874144716871172, -350.0220218866286928 ) ) ;
#16183=CARTESIAN_POINT ( 'NONE',  ( 757.8323909638827445, -122.6346026584201354, -352.1044303154654358 ) ) ;
#16186=CARTESIAN_POINT ( 'NONE',  ( 770.0799878456142551, -421.9874144716863498, -362.9823548866085616 ) ) ;
#16191=CARTESIAN_POINT ( 'NONE',  ( 814.8207195650702488, -266.1908817542435486, -336.2433038121456548 ) ) ;
#16199=CARTESIAN_POINT ( 'NONE',  ( 805.2837595273609850, -122.7363362996985074, -340.5290396650784714 ) ) ;
#16200=CARTESIAN_POINT ( 'NONE',  ( 774.6858677611749044, -105.7255117493293000, -315.5713283507209894 ) ) ;
#16201=CARTESIAN_POINT ( 'NONE',  ( 802.1676090361155502, -326.6346026584194533, -327.8955696845344505 ) ) ;
#16203=CARTESIAN_POINT ( 'NONE',  ( 801.9419747391806368, -426.4527844766010389, -351.9812246680014027 ) ) ;
#16204=CARTESIAN_POINT ( 'NONE',  ( 758.0580252608178853, -78.45278447660211896, -328.0187753319985404 ) ) ;
#16210=CARTESIAN_POINT ( 'NONE',  ( 776.2046728542105711, -356.1908817542432075, -304.8212110874238761 ) ) ;
#16213=CARTESIAN_POINT ( 'NONE',  ( 804.6798772138708955, -303.7255117493287457, -334.6312213355107019 ) ) ;
#16216=CARTESIAN_POINT ( 'NONE',  ( 796.1575198192839480, -198.0090635724255606, -359.4546378042384163 ) ) ;
#16219=LINE ( 'NONE', #22692, #31335 ) ;
#16220=CARTESIAN_POINT ( 'NONE',  ( 777.4774526936600978, -394.2709662947829088, -304.7301800767028226 ) ) ;
#16225=CARTESIAN_POINT ( 'NONE',  ( 758.8095938919642549, -8.089148112965974136, -311.6929314249763365 ) ) ;
#16226=CARTESIAN_POINT ( 'NONE',  ( 764.8639956371174549, -248.0891481129651481, -319.7806653035542013 ) ) ;
#16230=CARTESIAN_POINT ( 'NONE',  ( 802.7791456095903868, -52.71468719896020616, -329.0155153010375102 ) ) ;
#16240=CARTESIAN_POINT ( 'NONE',  ( 761.2382568024794409, -327.6237781080502600, -356.9571628226838129 ) ) ;
#16243=CARTESIAN_POINT ( 'NONE',  ( 786.2056067578752163, -347.8055962898683333, -374.4686193811670023 ) ) ;
#16250=CARTESIAN_POINT ( 'NONE',  ( 747.2067596250078623, -219.1800572038744122, -352.2312462859687230 ) ) ;
#16253=CARTESIAN_POINT ( 'NONE',  ( 785.3687786644885591, -179.3618753856927128, -315.3201227861280813 ) ) ;
#16255=CARTESIAN_POINT ( 'NONE',  ( 805.1927285166397041, -328.8164208402375834, -341.8018195045277707 ) ) ;
#16256=CARTESIAN_POINT ( 'NONE',  ( 781.7834795799800531, 13.18357915976123174, -315.0636971347436202 ) ) ;
#16264=CARTESIAN_POINT ( 'NONE',  ( 772.4468031744293057, -441.8272453906066630, -363.8651313633793620 ) ) ;
#16268=CARTESIAN_POINT ( 'NONE',  ( 812.3518521366052028, -241.0999726633345119, -326.5853460496235243 ) ) ;
#16271=CARTESIAN_POINT ( 'NONE',  ( 778.1981804954714335, -202.2709662947834772, -314.8072714833589885 ) ) ;
#16272=CARTESIAN_POINT ( 'NONE',  ( 796.7845633553578182, -369.6237781080500895, -358.5707757039688204 ) ) ;
#16274=CARTESIAN_POINT ( 'NONE',  ( 744.6391490659812007, -230.7363362996981664, -338.7502325331110455 ) ) ;
#16277=CARTESIAN_POINT ( 'NONE',  ( 802.5472867521000353, -76.37269993606228979, -350.8726784830461156 ) ) ;
#16280=CARTESIAN_POINT ( 'NONE',  ( 756.7813123517142913, -427.9874144716862929, -329.9779781133712504 ) ) ;
#16281=CARTESIAN_POINT ( 'NONE',  ( 805.0032342141413437, -277.5436935675105588, -314.9967657858572352 ) ) ;
#16284=CARTESIAN_POINT ( 'NONE',  ( 804.4286716492782716, -41.36187538569314626, -345.3141322388244703 ) ) ;
#16286=CARTESIAN_POINT ( 'NONE',  ( 791.1614460488616487, -155.2601417444144261, -373.5763878283158874 ) ) ;
#16288=CARTESIAN_POINT ( 'NONE',  ( 811.0346526505616112, -398.6346026584193396, -323.0537975583477532 ) ) ;
#16292=CARTESIAN_POINT ( 'NONE',  ( 771.2633955100217236, -383.9073299311466485, -363.4237431249939618 ) ) ;
#16294=EDGE_CURVE ( 'NONE', #820, #1585, #20057, .T. ) ;
#16298=CARTESIAN_POINT ( 'NONE',  ( 794.1144889064781864, -226.1692326535051052, -360.9840315886528401 ) ) ;
#16300=CARTESIAN_POINT ( 'NONE',  ( 781.2497674668890113, -276.3510508353231785, -375.3608509340180603 ) ) ;
#16306=CARTESIAN_POINT ( 'NONE',  ( 794.9819416627830151, -156.9982390220564241, -319.9864689768909898 ) ) ;
#16309=CARTESIAN_POINT ( 'NONE',  ( 749.2812353651451076, -78.45278447660211896, -323.2262854647983090 ) ) ;
#16310=CARTESIAN_POINT ( 'NONE',  ( 781.7834795799800531, -82.81642084023846451, -315.0636971347436202 ) ) ;
#16312=CARTESIAN_POINT ( 'NONE',  ( 761.4292242960306112, -17.46360902697157513, -323.2154366446414429 ) ) ;
#16314=CARTESIAN_POINT ( 'NONE',  ( 802.9823548866075953, -361.0999726633341425, -330.0799878456151077 ) ) ;
#16321=CARTESIAN_POINT ( 'NONE',  ( 798.5707757039680246, -341.4636090269705733, -356.7845633553585003 ) ) ;
#16322=CARTESIAN_POINT ( 'NONE',  ( 756.5762568750052424, -315.1800572038740711, -348.7366044899774238 ) ) ;
#16323=CARTESIAN_POINT ( 'NONE',  ( 786.2694204179717872, -141.2817908451530400, -305.1769319972829067 ) ) ;
#16327=CARTESIAN_POINT ( 'NONE',  ( 789.9200121543843807, -265.9874144716867477, -317.0176451133914384 ) ) ;
#16328=CARTESIAN_POINT ( 'NONE',  ( 811.3240766477731540, -124.3726999360621619, -355.6651683502462902 ) ) ;
#16335=CARTESIAN_POINT ( 'NONE',  ( 808.0189434323515343, -158.0891481129655176, -319.0252816721025511 ) ) ;
#16336=CARTESIAN_POINT ( 'NONE',  ( 759.2380499001254748, 21.41625977839825978, -318.3449445151863415 ) ) ;
#16338=CARTESIAN_POINT ( 'NONE',  ( 767.7687537140311633, -311.9073299311468759, -372.7932403749916830 ) ) ;
#16339=CARTESIAN_POINT ( 'NONE',  ( 800.9747183278959710, -444.9982390220554862, -311.9810565676471583 ) ) ;
#16344=CARTESIAN_POINT ( 'NONE',  ( 815.1787889125755555, -342.8965053807773984, -343.7953271457877804 ) ) ;
#16345=CARTESIAN_POINT ( 'NONE',  ( 746.8695393053150156, -101.9073299311474727, -327.6429770376306010 ) ) ;
#16347=CARTESIAN_POINT ( 'NONE',  ( 763.2262854647970016, -392.6346026584193396, -309.2812353651462445 ) ) ;
#16350=VERTEX_POINT ( 'NONE', #5193 ) ;
#16353=CARTESIAN_POINT ( 'NONE',  ( 808.7758568127978833, -124.1692326535054463, -320.0363995740631822 ) ) ;
#16359=CARTESIAN_POINT ( 'NONE',  ( 745.1769319972822814, -425.8055962898680491, -346.2694204179732083 ) ) ;
#16363=CARTESIAN_POINT ( 'NONE',  ( 766.4474001241216001, -379.0999726633341993, -307.3154664389482491 ) ) ;
#16364=CARTESIAN_POINT ( 'NONE',  ( 797.6776695296629214, -235.5436935675107293, -357.6776695296636603 ) ) ;
#16368=CARTESIAN_POINT ( 'NONE',  ( 783.0745993439762742, -224.1908817542436623, -365.1016975059196739 ) ) ;
#16369=CARTESIAN_POINT ( 'NONE',  ( 802.1676090361156639, -230.6346026584197659, -327.8955696845344505 ) ) ;
#16371=CARTESIAN_POINT ( 'NONE',  ( 765.0180583372156207, -408.9982390220556567, -360.0135310231089534 ) ) ;
#16374=CARTESIAN_POINT ( 'NONE',  ( 758.0580252608178853, -102.4527844766020337, -328.0187753319985404 ) ) ;
#16383=CARTESIAN_POINT ( 'NONE',  ( 804.1009440267234822, -455.4636090269701754, -314.0944755984392600 ) ) ;
#16384=CARTESIAN_POINT ( 'NONE',  ( 782.4968714119720516, -58.81642084023854267, -305.0891759886411023 ) ) ;
#16386=CARTESIAN_POINT ( 'NONE',  ( 803.6646147819161570, -425.9073299311463074, -348.8264449731210561 ) ) ;
#16387=CARTESIAN_POINT ( 'NONE',  ( 755.3201227861273992, -51.72551174932947049, -345.3687786644892981 ) ) ;
#16390=CARTESIAN_POINT ( 'NONE',  ( 763.0428371773158460, -299.4636090269707438, -358.7617431975195359 ) ) ;
#16391=CARTESIAN_POINT ( 'NONE',  ( 782.4968714119720516, -178.8164208402381519, -305.0891759886411023 ) ) ;
#16396=CARTESIAN_POINT ( 'NONE',  ( 800.1688906516307043, -226.1692326535051052, -369.0717654672308186 ) ) ;
#16398=CARTESIAN_POINT ( 'NONE',  ( 754.9967657858570647, -265.5436935675106156, -365.0032342141425374 ) ) ;
#16402=CARTESIAN_POINT ( 'NONE',  ( 758.0580252608178853, -366.4527844766012095, -328.0187753319985404 ) ) ;
#16404=CARTESIAN_POINT ( 'NONE',  ( 748.6759233522253680, -88.37269993606226137, -324.3348316497537098 ) ) ;
#16405=CARTESIAN_POINT ( 'NONE',  ( 772.3691319403857278, -167.2601417444143976, -315.8894580844506663 ) ) ;
#16410=CARTESIAN_POINT ( 'NONE',  ( 805.0264073115434940, -174.3510508353234627, -339.4763451958999099 ) ) ;
#16412=CARTESIAN_POINT ( 'NONE',  ( 745.1769319972822814, 6.194403710130517382, -346.2694204179732083 ) ) ;
#16418=CARTESIAN_POINT ( 'NONE',  ( 745.5313806188320314, -279.2817908451526137, -333.7943932421247268 ) ) ;
#16426=CARTESIAN_POINT ( 'NONE',  ( 790.9844846989617508, -118.3726999360621619, -317.2208543904092721 ) ) ;
#16427=CARTESIAN_POINT ( 'NONE',  ( 781.7834795799800531, -130.8164208402383224, -315.0636971347436202 ) ) ;
#16429=CARTESIAN_POINT ( 'NONE',  ( 755.5713283507202505, -317.3618753856922581, -334.6858677611754729 ) ) ;
#16431=CARTESIAN_POINT ( 'NONE',  ( 762.3223304703356007, -439.5436935675101040, -322.3223304703362828 ) ) ;
#16438=CARTESIAN_POINT ( 'NONE',  ( 778.7629533639073998, -344.7363362996978253, -375.0009284576466371 ) ) ;
#16440=CARTESIAN_POINT ( 'NONE',  ( 764.8639956371174549, -320.0891481129648355, -319.7806653035542013 ) ) ;
#16442=CARTESIAN_POINT ( 'NONE',  ( 783.0745993439762742, -200.1908817542436907, -365.1016975059196739 ) ) ;
#16446=CARTESIAN_POINT ( 'NONE',  ( 801.1904061080338124, -380.0891481129647218, -368.3070685750236066 ) ) ;
#16451=CARTESIAN_POINT ( 'NONE',  ( 749.2812353651451076, -6.452784476602343666, -323.2262854647983090 ) ) ;
#16453=CARTESIAN_POINT ( 'NONE',  ( 774.6858677611749044, -249.7255117493288594, -315.5713283507209894 ) ) ;
#16457=CARTESIAN_POINT ( 'NONE',  ( 761.2382568024794409, -63.62377810805107714, -356.9571628226838129 ) ) ;
#16466=CARTESIAN_POINT ( 'NONE',  ( 789.9200121543843807, -361.9874144716864635, -317.0176451133914384 ) ) ;
#16469=CARTESIAN_POINT ( 'NONE',  ( 766.5853460496234675, -349.9874144716865771, -372.3518521366060554 ) ) ;
#16472=ORIENTED_EDGE ( 'NONE', *, *, #4424, .F. ) ;
#16478=CARTESIAN_POINT ( 'NONE',  ( 759.0252816721024374, -216.9982390220562252, -368.0189434323527280 ) ) ;
#16481=CARTESIAN_POINT ( 'NONE',  ( 762.3223304703356007, -199.5436935675108430, -322.3223304703362828 ) ) ;
#16483=CARTESIAN_POINT ( 'NONE',  ( 788.8264449731200330, -333.1800572038740142, -363.6646147819171233 ) ) ;
#16484=CARTESIAN_POINT ( 'NONE',  ( 800.0135310231082713, 9.910851887033969021, -325.0180583372163028 ) ) ;
#16487=CYLINDRICAL_SURFACE ( 'NONE', #18874, 10.00000000000000888 ) ;
#16491=CARTESIAN_POINT ( 'NONE',  ( 790.9844846989617508, -454.3726999360611103, -317.2208543904092721 ) ) ;
#16496=CARTESIAN_POINT ( 'NONE',  ( 791.0478386215596629, -237.8272453906072599, -306.7653713866226326 ) ) ;
#16500=CARTESIAN_POINT ( 'NONE',  ( 797.8594530101008786, -181.5436935675108145, -322.1405469898980982 ) ) ;
#16502=CARTESIAN_POINT ( 'NONE',  ( 780.5290396650775619, -372.3510508353228374, -365.2837595273619513 ) ) ;
#16503=CARTESIAN_POINT ( 'NONE',  ( 810.4231160770870019, -240.5545181178798941, -321.9338519418446936 ) ) ;
#16506=CARTESIAN_POINT ( 'NONE',  ( 805.2837595273609850, -74.73633629969866377, -340.5290396650784714 ) ) ;
#16509=DIRECTION ( 'NONE',  ( -0.000000000000000000, 0.000000000000000000, -1.000000000000000000 ) ) ;
#16510=CARTESIAN_POINT ( 'NONE',  ( 804.1601925771018387, -439.4419599262316751, -346.5483106153029098 ) ) ;
#16511=CARTESIAN_POINT ( 'NONE',  ( 763.2262854647970016, -272.6346026584196807, -309.2812353651462445 ) ) ;
#16514=CARTESIAN_POINT ( 'NONE',  ( 797.6776695296629214, -43.54369356751131903, -357.6776695296636603 ) ) ;
#16517=CARTESIAN_POINT ( 'NONE',  ( 754.0944755984390895, -159.6237781080508285, -364.1009440267246760 ) ) ;
#16519=CARTESIAN_POINT ( 'NONE',  ( 813.1304606946830518, -401.9073299311463643, -352.3570229623690580 ) ) ;
#16525=CARTESIAN_POINT ( 'NONE',  ( 804.4286716492782716, -425.3618753856919170, -345.3141322388244703 ) ) ;
#16526=CARTESIAN_POINT ( 'NONE',  ( 799.9999999999993179, -512.9681489794448908, -339.9999999999999432 ) ) ;
#16531=CARTESIAN_POINT ( 'NONE',  ( 790.8726784830453198, -250.7146871989595809, -362.5472867521010585 ) ) ;
#16533=CARTESIAN_POINT ( 'NONE',  ( 759.9864689768902508, -122.0891481129656171, -354.9819416627836404 ) ) ;
#16535=CARTESIAN_POINT ( 'NONE',  ( 756.1443688327750579, -261.6237781080504305, -314.3581564841659315 ) ) ;
#16541=ADVANCED_FACE ( 'NONE', ( #17183, #38667 ), #37983, .T. ) ;
#16542=CARTESIAN_POINT ( 'NONE',  ( 797.6776695296629214, -163.5436935675109567, -357.6776695296636603 ) ) ;
#16544=CARTESIAN_POINT ( 'NONE',  ( 767.6429770376289525, -129.1800572038746111, -306.8695393053162093 ) ) ;
#16545=CARTESIAN_POINT ( 'NONE',  ( 774.6858677611749044, -105.7255117493293000, -315.5713283507209894 ) ) ;
#16547=CARTESIAN_POINT ( 'NONE',  ( 775.8780910478218402, -33.28179084515333130, -364.9511171171680530 ) ) ;
#16548=CARTESIAN_POINT ( 'NONE',  ( 800.9840315886518738, -340.9181544815160123, -354.1144889064786412 ) ) ;
#16557=CARTESIAN_POINT ( 'NONE',  ( 772.4468031744293057, -369.8272453906068904, -363.8651313633793620 ) ) ;
#16558=CARTESIAN_POINT ( 'NONE',  ( 785.3141322388236176, -333.7255117493286320, -364.4286716492789537 ) ) ;
#16559=CARTESIAN_POINT ( 'NONE',  ( 781.2370466360911223, -140.7363362996984506, -304.9990715423533629 ) ) ;
#16560=CIRCLE ( 'NONE', #28342, 30.00000000000002842 ) ;
#16564=ADVANCED_FACE ( 'NONE', ( #31271 ), #16965, .T. ) ;
#16565=CARTESIAN_POINT ( 'NONE',  ( 779.4709603349208464, -264.3510508353232353, -314.7162404726379918 ) ) ;
#16566=CARTESIAN_POINT ( 'NONE',  ( 788.6739635108323228, -103.6454272087894850, -373.9316612368139090 ) ) ;
#16568=CARTESIAN_POINT ( 'NONE',  ( 779.9999999999992042, -452.9681489794448339, -339.9999999999999432 ) ) ;
#16575=CARTESIAN_POINT ( 'NONE',  ( 745.7998596910086917, -173.3618753856927128, -332.5602148656461168 ) ) ;
#16578=CARTESIAN_POINT ( 'NONE',  ( 745.7998596910086917, -317.3618753856922581, -332.5602148656461168 ) ) ;
#16585=CARTESIAN_POINT ( 'NONE',  ( 749.8865473780648472, -380.5328690171409676, -322.1177392798429082 ) ) ;
#16586=CARTESIAN_POINT ( 'NONE',  ( 814.9108240113580450, -112.2709662947838325, -337.5031285880265273 ) ) ;
#16589=CARTESIAN_POINT ( 'NONE',  ( 805.0032342141412300, -373.5436935675101040, -314.9967657858571783 ) ) ;
#16594=CARTESIAN_POINT ( 'NONE',  ( 811.6461892240364477, -148.7146871989598935, -324.1737431748509835 ) ) ;
#16601=CARTESIAN_POINT ( 'NONE',  ( 792.3570229623688874, 2.819942796124898177, -373.1304606946836202 ) ) ;
#16604=CARTESIAN_POINT ( 'NONE',  ( 745.7194118038753459, -397.6454272087885329, -348.7631598425976449 ) ) ;
#16608=CARTESIAN_POINT ( 'NONE',  ( 769.9779781133707957, -235.0999726633344835, -316.7813123517150871 ) ) ;
#16609=CARTESIAN_POINT ( 'NONE',  ( 800.2193346964447755, -210.9982390220561967, -355.1360043628815788 ) ) ;
#16610=CARTESIAN_POINT ( 'NONE',  ( 803.4237431249931660, -423.1800572038737300, -331.2633955100225194 ) ) ;
#16615=CARTESIAN_POINT ( 'NONE',  ( 791.0733055594794223, 17.05262341476191068, -312.1184307474205184 ) ) ;
#16622=CARTESIAN_POINT ( 'NONE',  ( 811.3240766477731540, -460.3726999360611103, -355.6651683502462902 ) ) ;
#16623=CARTESIAN_POINT ( 'NONE',  ( 751.6929314249750860, -78.99823902205665149, -318.8095938919659034 ) ) ;
#16625=CARTESIAN_POINT ( 'NONE',  ( 759.7806653035534055, -414.9982390220555430, -324.8639956371180801 ) ) ;
#16626=CARTESIAN_POINT ( 'NONE',  ( 771.1735550268780344, -33.18005720387498769, -316.3353852180828198 ) ) ;
#16629=CARTESIAN_POINT ( 'NONE',  ( 766.9102291470427417, -282.5545181178798657, -318.6633372737382501 ) ) ;
#16630=CARTESIAN_POINT ( 'NONE',  ( 782.5225473063381969, -190.2709662947835909, -375.2698199232970637 ) ) ;
#16636=CARTESIAN_POINT ( 'NONE',  ( 815.0009284576459549, -246.3510508353232638, -338.7629533639073429 ) ) ;
#16638=CARTESIAN_POINT ( 'NONE',  ( 801.1904061080336987, -284.0891481129650629, -368.3070685750235498 ) ) ;
#16642=CARTESIAN_POINT ( 'NONE',  ( 781.7834795799800531, -346.8164208402376971, -315.0636971347436202 ) ) ;
#16644=CARTESIAN_POINT ( 'NONE',  ( 785.3141322388236176, -189.7255117493290300, -364.4286716492789537 ) ) ;
#16645=CARTESIAN_POINT ( 'NONE',  ( 813.2346286133761168, -53.26014174441475291, -328.9521613784389160 ) ) ;
#16646=CARTESIAN_POINT ( 'NONE',  ( 770.0799878456142551, -157.9874144716871456, -362.9823548866085616 ) ) ;
#16651=CARTESIAN_POINT ( 'NONE',  ( 755.5713283507202505, -53.36187538569310362, -334.6858677611754729 ) ) ;
#16652=CARTESIAN_POINT ( 'NONE',  ( 802.7791456095903868, -172.7146871989598083, -329.0155153010375102 ) ) ;
#16655=CARTESIAN_POINT ( 'NONE',  ( 761.9338519418445230, -14.53286901714214707, -370.4231160770881957 ) ) ;
#16661=CARTESIAN_POINT ( 'NONE',  ( 764.1737431748507561, -274.3726999360617356, -371.6461892240376415 ) ) ;
#16667=CARTESIAN_POINT ( 'NONE',  ( 804.6971507214547046, -99.28179084515313946, -344.0799538623459739 ) ) ;
#16668=CARTESIAN_POINT ( 'NONE',  ( 778.1981804954714335, -130.2709662947837899, -314.8072714833589885 ) ) ;
#16669=CARTESIAN_POINT ( 'NONE',  ( 755.0636971347428243, -316.2709662947832499, -341.7834795799807353 ) ) ;
#16671=CARTESIAN_POINT ( 'NONE',  ( 795.1360043628807261, -428.0891481129644944, -360.2193346964456282 ) ) ;
#16679=CARTESIAN_POINT ( 'NONE',  ( 815.3608509340175488, -338.7363362996978822, -341.2497674668889545 ) ) ;
#16682=CARTESIAN_POINT ( 'NONE',  ( 759.7806653035534055, -318.9982390220557704, -324.8639956371180801 ) ) ;
#16684=CARTESIAN_POINT ( 'NONE',  ( 801.5560724626406000, -192.5545181178801215, -326.7756240680316182 ) ) ;
#16688=CARTESIAN_POINT ( 'NONE',  ( 749.2812353651451076, -390.4527844766011526, -323.2262854647983090 ) ) ;
#16693=CARTESIAN_POINT ( 'NONE',  ( 814.2001403089898304, -17.36187538569322086, -347.4397851343538264 ) ) ;
#16694=CARTESIAN_POINT ( 'NONE',  ( 791.9812246680005501, -260.6346026584197375, -361.9419747391813189 ) ) ;
#16695=PLANE ( 'NONE',  #42409 ) ;
#16699=CARTESIAN_POINT ( 'NONE',  ( 776.9566956441375396, -36.89650538077844288, -364.8461984189686405 ) ) ;
#16705=CARTESIAN_POINT ( 'NONE',  ( 797.8594530101008786, -61.54369356751124087, -322.1405469898980982 ) ) ;
#16707=CARTESIAN_POINT ( 'NONE',  ( 757.2208543904082489, -352.7146871989593251, -350.9844846989624330 ) ) ;
#16710=CARTESIAN_POINT ( 'NONE',  ( 744.8212110874229666, -378.8965053807772847, -336.2046728542121627 ) ) ;
#16717=CARTESIAN_POINT ( 'NONE',  ( 782.5225473063381969, -214.2709662947834488, -375.2698199232970637 ) ) ;
#16720=CARTESIAN_POINT ( 'NONE',  ( 802.1676090361155502, -206.6346026584198796, -327.8955696845344505 ) ) ;
#16722=CARTESIAN_POINT ( 'NONE',  ( 804.9363028652555840, -328.2709662947831362, -338.2165204200192079 ) ) ;
#16723=CARTESIAN_POINT ( 'NONE',  ( 804.6971507214547046, -459.2817908451519884, -344.0799538623459739 ) ) ;
#16730=CARTESIAN_POINT ( 'NONE',  ( 761.4292242960306112, -449.4636090269702322, -323.2154366446414429 ) ) ;
#16731=DIRECTION ( 'NONE',  ( 0.000000000000000000, -1.000000000000000000, 0.000000000000000000 ) ) ;
#16732=DIRECTION ( 'NONE',  ( 0.000000000000000000, -1.000000000000000000, 1.110223024625155554E-15 ) ) ;
#16734=CARTESIAN_POINT ( 'NONE',  ( 755.8990559732751535, -251.4636090269709143, -365.9055244015606831 ) ) ;
#16737=CARTESIAN_POINT ( 'NONE',  ( 762.3223304703356007, -223.5436935675107577, -322.3223304703362828 ) ) ;
#16738=CARTESIAN_POINT ( 'NONE',  ( 799.4546378042377910, -369.0783235625956422, -356.1575198192848006 ) ) ;
#16739=CARTESIAN_POINT ( 'NONE',  ( 797.8822607201568644, -246.5545181178799510, -370.1134526219340160 ) ) ;
#16742=CARTESIAN_POINT ( 'NONE',  ( 754.7162404726377645, -86.73633629969862113, -339.4709603349214717 ) ) ;
#16747=CARTESIAN_POINT ( 'NONE',  ( 782.5225473063383106, -286.2709662947833067, -375.2698199232970637 ) ) ;
#16750=CARTESIAN_POINT ( 'NONE',  ( 756.5762568750052424, -51.18005720387493085, -348.7366044899774238 ) ) ;
#16753=CARTESIAN_POINT ( 'NONE',  ( 813.9316612368132837, -175.4419599262325562, -348.6739635108323228 ) ) ;
#16755=CARTESIAN_POINT ( 'NONE',  ( 796.7737145352015204, -404.6346026584193396, -370.7187646348536987 ) ) ;
#16760=CARTESIAN_POINT ( 'NONE',  ( 759.9864689768902508, -434.0891481129646081, -354.9819416627836404 ) ) ;
#16766=CARTESIAN_POINT ( 'NONE',  ( 784.0799538623451781, -275.8055962898685038, -364.6971507214555572 ) ) ;
#16767=CARTESIAN_POINT ( 'NONE',  ( 754.8072714833581358, -124.8164208402383508, -338.1981804954720587 ) ) ;
#16769=CARTESIAN_POINT ( 'NONE',  ( 810.1134526219336749, -248.5328690171414223, -357.8822607201570349 ) ) ;
#16776=CARTESIAN_POINT ( 'NONE',  ( 795.9930595647434757, -27.07832356259665474, -320.7433823573372820 ) ) ;
#16777=CARTESIAN_POINT ( 'NONE',  ( 758.0580252608178853, -174.4527844766018063, -328.0187753319985404 ) ) ;
#16780=CARTESIAN_POINT ( 'NONE',  ( 813.1304606946830518, -113.9073299311474301, -352.3570229623690580 ) ) ;
#16781=CARTESIAN_POINT ( 'NONE',  ( 771.1735550268780344, -105.1800572038747390, -316.3353852180828198 ) ) ;
#16783=CARTESIAN_POINT ( 'NONE',  ( 786.5483106153019435, -55.64542720878963422, -364.1601925771022366 ) ) ;
#16785=CARTESIAN_POINT ( 'NONE',  ( 801.5560724626406000, -360.5545181178796383, -326.7756240680316182 ) ) ;
#16793=CARTESIAN_POINT ( 'NONE',  ( 766.9102291470427417, -354.5545181178796383, -318.6633372737382501 ) ) ;
#16794=CARTESIAN_POINT ( 'NONE',  ( 778.1981804954714335, -370.2709662947831362, -314.8072714833589885 ) ) ;
#16795=CARTESIAN_POINT ( 'NONE',  ( 810.4231160770870019, -120.5545181178803205, -321.9338519418446936 ) ) ;
#16799=CARTESIAN_POINT ( 'NONE',  ( 755.8990559732751535, -155.4636090269711417, -365.9055244015606831 ) ) ;
#16805=CARTESIAN_POINT ( 'NONE',  ( 796.9462024416508257, -156.4527844766018916, -308.9653473494370246 ) ) ;
#16810=CARTESIAN_POINT ( 'NONE',  ( 792.2312462859673587, -299.9073299311468759, -307.2067596250082602 ) ) ;
#16811=CARTESIAN_POINT ( 'NONE',  ( 779.9999999999992042, 16.45630643248849267, -339.9999999999999432 ) ) ;
#16817=CARTESIAN_POINT ( 'NONE',  ( 814.8230680027162407, -365.8055962898682765, -333.7305795820267917 ) ) ;
#16819=CARTESIAN_POINT ( 'NONE',  ( 745.7998596910086917, -125.3618753856928834, -332.5602148656461168 ) ) ;
#16821=CARTESIAN_POINT ( 'NONE',  ( 763.0537975583475827, -384.4527844766011526, -371.0346526505627480 ) ) ;
#16822=DIRECTION ( 'NONE',  ( -1.000000000000000000, -0.000000000000000000, -0.000000000000000000 ) ) ;
#16825=CARTESIAN_POINT ( 'NONE',  ( 783.7566961878529810, -144.8965053807781089, -305.1792804349288417 ) ) ;
#16831=CARTESIAN_POINT ( 'NONE',  ( 759.2295555964440155, -16.16923265350578021, -353.9708237608231229 ) ) ;
#16834=CARTESIAN_POINT ( 'NONE',  ( 808.0189434323515343, -14.08914811296595460, -319.0252816721025511 ) ) ;
#16835=LINE ( 'NONE', #34127, #23910 ) ;
#16838=CARTESIAN_POINT ( 'NONE',  ( 800.2193346964447755, -186.9982390220563104, -355.1360043628815788 ) ) ;
#16839=CARTESIAN_POINT ( 'NONE',  ( 748.6759233522253680, -400.3726999360612808, -324.3348316497537098 ) ) ;
#16840=CARTESIAN_POINT ( 'NONE',  ( 801.9419747391806368, -258.4527844766016074, -351.9812246680014027 ) ) ;
#16843=CARTESIAN_POINT ( 'NONE',  ( 755.3028492785439312, -255.2817908451526705, -335.9200461376539693 ) ) ;
#16844=CARTESIAN_POINT ( 'NONE',  ( 756.3353852180819104, -221.9073299311470464, -331.1735550268788302 ) ) ;
#16845=CARTESIAN_POINT ( 'NONE',  ( 800.2193346964446619, -402.9982390220555999, -355.1360043628816925 ) ) ;
#16851=CARTESIAN_POINT ( 'NONE',  ( 745.7194118038753459, -61.64542720878961291, -348.7631598425976449 ) ) ;
#16857=CARTESIAN_POINT ( 'NONE',  ( 796.9571628226829034, -23.46360902697155026, -321.2382568024804641 ) ) ;
#16858=CARTESIAN_POINT ( 'NONE',  ( 813.1304606946831655, -65.90732993114760063, -352.3570229623691716 ) ) ;
#16860=CARTESIAN_POINT ( 'NONE',  ( 759.7806653035534055, -438.9982390220553157, -324.8639956371180801 ) ) ;
#16861=CARTESIAN_POINT ( 'NONE',  ( 764.8639956371174549, -32.08914811296589420, -319.7806653035542581 ) ) ;
#16863=CARTESIAN_POINT ( 'NONE',  ( 744.7301800767019131, -196.8164208402380950, -337.4774526936615757 ) ) ;
#16868=CARTESIAN_POINT ( 'NONE',  ( 759.8311093483677041, -262.1692326535049347, -310.9282345327691814 ) ) ;
#16870=CARTESIAN_POINT ( 'NONE',  ( 808.0189434323515343, -278.0891481129651197, -319.0252816721025511 ) ) ;
#16871=CYLINDRICAL_SURFACE ( 'NONE', #12481, 10.00000000000000888 ) ;
#16874=CARTESIAN_POINT ( 'NONE',  ( 800.0135310231082713, -350.0891481129648923, -325.0180583372163028 ) ) ;
#16876=CARTESIAN_POINT ( 'NONE',  ( 771.2368401574024119, -61.44195992623291147, -374.2805881961240857 ) ) ;
#16877=CARTESIAN_POINT ( 'NONE',  ( 754.8983024940795303, -162.8965053807780521, -336.9254006560228163 ) ) ;
#16882=CARTESIAN_POINT ( 'NONE',  ( 756.3353852180819104, -77.90732993114757221, -331.1735550268788302 ) ) ;
#16883=CARTESIAN_POINT ( 'NONE',  ( 786.6156483768007774, -169.4419599262325562, -315.5913626894246136 ) ) ;
#16885=CARTESIAN_POINT ( 'NONE',  ( 759.8311093483677041, 1.830767346494167391, -310.9282345327691814 ) ) ;
#16891=CARTESIAN_POINT ( 'NONE',  ( 814.8207195650702488, -314.1908817542433781, -336.2433038121456548 ) ) ;
#16895=CARTESIAN_POINT ( 'NONE',  ( 769.9779781133707957, -163.0999726633347677, -316.7813123517150871 ) ) ;
#16896=CARTESIAN_POINT ( 'NONE',  ( 767.8955696845333705, -120.4527844766019484, -362.1676090361162323 ) ) ;
#16897=CARTESIAN_POINT ( 'NONE',  ( 800.0135310231082713, -326.0891481129649492, -325.0180583372163028 ) ) ;
#16899=CARTESIAN_POINT ( 'NONE',  ( 803.6646147819161570, -425.9073299311463074, -348.8264449731210561 ) ) ;
#16906=CARTESIAN_POINT ( 'NONE',  ( 795.8262568251477660, -334.3726999360615082, -308.3538107759623585 ) ) ;
#16909=VECTOR ( 'NONE', #3002, 1000.000000000000000 ) ;
#16910=CARTESIAN_POINT ( 'NONE',  ( 781.8018195045266339, -310.2709662947832499, -365.1927285166406705 ) ) ;
#16912=CARTESIAN_POINT ( 'NONE',  ( 754.7162404726377645, -182.7363362996983369, -339.4709603349214717 ) ) ;
#16915=CARTESIAN_POINT ( 'NONE',  ( 777.5031285880264704, -382.8164208402374697, -374.9108240113588408 ) ) ;
#16920=CARTESIAN_POINT ( 'NONE',  ( 814.9108240113580450, -16.27096629478413092, -337.5031285880265273 ) ) ;
#16921=CARTESIAN_POINT ( 'NONE',  ( 755.3201227861273992, -243.7255117493287742, -345.3687786644892981 ) ) ;
#16925=CARTESIAN_POINT ( 'NONE',  ( 799.9636004259356241, -46.91815448151694312, -311.2241431872006956 ) ) ;
#16926=CARTESIAN_POINT ( 'NONE',  ( 758.6633372737375112, -44.53286901714205470, -326.9102291470432533 ) ) ;
#16930=FACE_OUTER_BOUND ( 'NONE', #36707, .T. ) ;
#16934=CARTESIAN_POINT ( 'NONE',  ( 774.6312213355099630, -71.36187538569302546, -364.6798772138717482 ) ) ;
#16935=CARTESIAN_POINT ( 'NONE',  ( 765.8855110935204493, -358.1692326535047641, -319.0159684113471599 ) ) ;
#16938=CARTESIAN_POINT ( 'NONE',  ( 754.0944755984390895, -351.6237781080502032, -364.1009440267246760 ) ) ;
#16944=CARTESIAN_POINT ( 'NONE',  ( 813.1304606946830518, -233.9073299311470180, -352.3570229623690580 ) ) ;
#16947=CARTESIAN_POINT ( 'NONE',  ( 797.8594530101009923, -205.5436935675108145, -322.1405469898982119 ) ) ;
#16949=CARTESIAN_POINT ( 'NONE',  ( 758.0580252608178853, -342.4527844766013231, -328.0187753319985404 ) ) ;
#16950=CARTESIAN_POINT ( 'NONE',  ( 795.1360043628807261, 3.910851887033985896, -360.2193346964456282 ) ) ;
#16955=CARTESIAN_POINT ( 'NONE',  ( 793.9708237608222134, -454.9181544815156713, -319.2295555964448681 ) ) ;
#16959=CARTESIAN_POINT ( 'NONE',  ( 781.2370466360911223, -236.7363362996981380, -304.9990715423533629 ) ) ;
#16962=CARTESIAN_POINT ( 'NONE',  ( 785.3687786644884454, -227.3618753856925707, -315.3201227861279676 ) ) ;
#16963=CARTESIAN_POINT ( 'NONE',  ( 775.9200461376533440, -383.8055962898682765, -315.3028492785443291 ) ) ;
#16964=CARTESIAN_POINT ( 'NONE',  ( 809.0717654672305343, -244.9181544815162681, -360.1688906516309885 ) ) ;
#16965=CYLINDRICAL_SURFACE ( 'NONE', #35583, 10.00000000000000888 ) ;
#16967=CARTESIAN_POINT ( 'NONE',  ( 759.0159684113467620, -64.91815448151686496, -325.8855110935213020 ) ) ;
#16971=CARTESIAN_POINT ( 'NONE',  ( 789.9200121543843807, -433.9874144716862361, -317.0176451133914384 ) ) ;
#16972=CARTESIAN_POINT ( 'NONE',  ( 747.2067596250078623, -291.1800572038741848, -352.2312462859687230 ) ) ;
#16975=CARTESIAN_POINT ( 'NONE',  ( 774.6312213355099630, -71.36187538569302546, -364.6798772138717482 ) ) ;
#16977=CARTESIAN_POINT ( 'NONE',  ( 768.8385539511368734, -167.2601417444143976, -306.4236121716840557 ) ) ;
#16979=CARTESIAN_POINT ( 'NONE',  ( 748.9653473494363425, -410.6346026584191122, -356.9462024416521331 ) ) ;
#16980=CARTESIAN_POINT ( 'NONE',  ( 799.9999999999993179, -462.9681489794448339, -370.0000000000000568 ) ) ;
#16983=CARTESIAN_POINT ( 'NONE',  ( 771.2633955100217236, -431.9073299311464211, -363.4237431249939618 ) ) ;
#16990=CARTESIAN_POINT ( 'NONE',  ( 756.1348686366196716, -257.2601417444141134, -347.5531968255698416 ) ) ;
#16992=CARTESIAN_POINT ( 'NONE',  ( 768.8385539511368734, -263.2601417444141134, -306.4236121716840557 ) ) ;
#16997=CARTESIAN_POINT ( 'NONE',  ( 796.7845633553578182, -57.62377810805111267, -358.5707757039688204 ) ) ;
#16998=CARTESIAN_POINT ( 'NONE',  ( 759.9864689768902508, -170.0891481129654608, -354.9819416627836404 ) ) ;
#17000=CARTESIAN_POINT ( 'NONE',  ( 747.2067596250078623, -99.18005720387478164, -352.2312462859687230 ) ) ;
#17001=CARTESIAN_POINT ( 'NONE',  ( 771.2633955100217236, -119.9073299311474443, -363.4237431249939618 ) ) ;
#17003=CARTESIAN_POINT ( 'NONE',  ( 755.5913626894240451, -37.64542720878968396, -346.6156483768012890 ) ) ;
#17004=CARTESIAN_POINT ( 'NONE',  ( 760.7433823573367135, -372.0090635724250205, -355.9930595647440441 ) ) ;
#17008=PLANE ( 'NONE',  #7046 ) ;
#17011=CARTESIAN_POINT ( 'NONE',  ( 772.4468031744293057, -345.8272453906069472, -363.8651313633793620 ) ) ;
#17012=CARTESIAN_POINT ( 'NONE',  ( 800.0135310231082713, -350.0891481129648923, -325.0180583372163028 ) ) ;
#17013=CARTESIAN_POINT ( 'NONE',  ( 764.1737431748507561, -130.3726999360621619, -371.6461892240376415 ) ) ;
#17017=CARTESIAN_POINT ( 'NONE',  ( 755.8398074228967971, -307.4419599262320730, -333.4516893846970333 ) ) ;
#17018=CARTESIAN_POINT ( 'NONE',  ( 762.1177392798416577, -162.5545181178802352, -309.8865473780659272 ) ) ;
#17020=DIRECTION ( 'NONE',  ( 0.000000000000000000, -1.000000000000000000, 0.000000000000000000 ) ) ;
#17023=CARTESIAN_POINT ( 'NONE',  ( 810.7187646348534145, -162.4527844766018632, -356.7737145352016341 ) ) ;
#17026=CARTESIAN_POINT ( 'NONE',  ( 763.0537975583475827, -312.4527844766012663, -371.0346526505627480 ) ) ;
#17032=VERTEX_POINT ( 'NONE', #36331 ) ;
#17034=CARTESIAN_POINT ( 'NONE',  ( 793.4146539503750546, -385.9874144716864066, -307.6481478633938877 ) ) ;
#17035=CARTESIAN_POINT ( 'NONE',  ( 811.0346526505616112, -134.6346026584201070, -323.0537975583477532 ) ) ;
#17037=CARTESIAN_POINT ( 'NONE',  ( 813.1304606946830518, -401.9073299311463643, -352.3570229623690580 ) ) ;
#17042=CARTESIAN_POINT ( 'NONE',  ( 746.7653713866222915, -161.2601417444143976, -351.0478386215610271 ) ) ;
#17047=CARTESIAN_POINT ( 'NONE',  ( 746.8695393053150156, -5.907329931147798696, -327.6429770376306010 ) ) ;
#17052=CARTESIAN_POINT ( 'NONE',  ( 805.1927285166397041, -184.8164208402380950, -341.8018195045277707 ) ) ;
#17053=CARTESIAN_POINT ( 'NONE',  ( 810.4231160770870019, -408.5545181178794110, -321.9338519418446936 ) ) ;
#17056=CARTESIAN_POINT ( 'NONE',  ( 781.8018195045266339, -262.2709662947831930, -365.1927285166406705 ) ) ;
#17059=EDGE_CURVE ( 'NONE', #22826, #37323, #15547, .T. ) ;
#17060=CARTESIAN_POINT ( 'NONE',  ( 804.1105419155481968, -267.8272453906071746, -347.6308680596136469 ) ) ;
#17061=CARTESIAN_POINT ( 'NONE',  ( 774.6858677611749044, -249.7255117493288594, -315.5713283507209894 ) ) ;
#17062=CARTESIAN_POINT ( 'NONE',  ( 762.3223304703356007, -415.5436935675102177, -322.3223304703362828 ) ) ;
#17063=CARTESIAN_POINT ( 'NONE',  ( 791.9812246680005501, -68.63460265842033436, -361.9419747391813189 ) ) ;
#17068=CARTESIAN_POINT ( 'NONE',  ( 744.6391490659812007, -62.73633629969871350, -338.7502325331110455 ) ) ;
#17074=CARTESIAN_POINT ( 'NONE',  ( 798.5707757039680246, -5.463609026971610660, -356.7845633553585003 ) ) ;
#17075=CARTESIAN_POINT ( 'NONE',  ( 808.0189434323515343, -86.08914811296573077, -319.0252816721025511 ) ) ;
#17077=CARTESIAN_POINT ( 'NONE',  ( 804.9363028652555840, -448.2709662947827951, -338.2165204200192079 ) ) ;
#17078=CARTESIAN_POINT ( 'NONE',  ( 801.9419747391806368, -42.45278447660223264, -351.9812246680014027 ) ) ;
#17081=CARTESIAN_POINT ( 'NONE',  ( 745.0891759886404770, -196.2709662947835909, -342.4968714119734159 ) ) ;
#17087=CARTESIAN_POINT ( 'NONE',  ( 751.2241431872005251, -256.1692326535049915, -359.9636004259367610 ) ) ;
#17089=CARTESIAN_POINT ( 'NONE',  ( 787.5162901302840055, -275.3618753856923149, -305.4481719005792684 ) ) ;
#17093=CARTESIAN_POINT ( 'NONE',  ( 815.0009284576459549, -30.35105083532391390, -338.7629533639073429 ) ) ;
#17094=CARTESIAN_POINT ( 'NONE',  ( 800.2193346964447755, -378.9982390220555999, -355.1360043628815788 ) ) ;
#17097=CARTESIAN_POINT ( 'NONE',  ( 800.1688906516307043, -58.16923265350564520, -369.0717654672308186 ) ) ;
#17098=CARTESIAN_POINT ( 'NONE',  ( 776.9566956441375396, -156.8965053807780805, -364.8461984189686405 ) ) ;
#17102=CARTESIAN_POINT ( 'NONE',  ( 765.0180583372156207, -72.99823902205667991, -360.0135310231089534 ) ) ;
#17103=CARTESIAN_POINT ( 'NONE',  ( 761.2382568024794409, -159.6237781080508285, -356.9571628226838129 ) ) ;
#17105=CARTESIAN_POINT ( 'NONE',  ( 761.9338519418445230, 9.467130982857780097, -370.4231160770881957 ) ) ;
#17110=CARTESIAN_POINT ( 'NONE',  ( 814.4686193811664907, -315.2817908451525000, -346.2056067578752732 ) ) ;
#17115=CARTESIAN_POINT ( 'NONE',  ( 805.2837595273609850, -146.7363362996984506, -340.5290396650784714 ) ) ;
#17116=CARTESIAN_POINT ( 'NONE',  ( 800.2193346964447755, -138.9982390220563957, -355.1360043628815788 ) ) ;
#17117=CARTESIAN_POINT ( 'NONE',  ( 765.0180583372156207, -312.9982390220559409, -360.0135310231089534 ) ) ;
#17124=CARTESIAN_POINT ( 'NONE',  ( 793.5525998758768083, -391.0999726633340288, -372.6845335610516941 ) ) ;
#17128=CARTESIAN_POINT ( 'NONE',  ( 759.7806653035534055, -342.9982390220557136, -324.8639956371180801 ) ) ;
#17130=LINE ( 'NONE', #17595, #3825 ) ;
#17131=CARTESIAN_POINT ( 'NONE',  ( 798.5707757039680246, -221.4636090269709428, -356.7845633553585003 ) ) ;
#17136=CARTESIAN_POINT ( 'NONE',  ( 749.2812353651451076, -414.4527844766010389, -323.2262854647983090 ) ) ;
#17140=CARTESIAN_POINT ( 'NONE',  ( 808.0189434323515343, -38.08914811296587999, -319.0252816721025511 ) ) ;
#17141=CARTESIAN_POINT ( 'NONE',  ( 795.1360043628807261, -260.0891481129650060, -360.2193346964456282 ) ) ;
#17145=CARTESIAN_POINT ( 'NONE',  ( 786.2694204179717872, -45.28179084515329578, -305.1769319972829067 ) ) ;
#17146=CARTESIAN_POINT ( 'NONE',  ( 764.0069404352550464, -63.07832356259653750, -359.2566176426627180 ) ) ;
#17149=CARTESIAN_POINT ( 'NONE',  ( 799.9999999999993179, -462.9681489794448339, -309.9999999999998863 ) ) ;
#17153=CARTESIAN_POINT ( 'NONE',  ( 778.1981804954714335, -58.27096629478398171, -314.8072714833589885 ) ) ;
#17154=CARTESIAN_POINT ( 'NONE',  ( 760.5453621957607311, -381.0783235625954717, -323.8424801807151425 ) ) ;
#17158=CARTESIAN_POINT ( 'NONE',  ( 766.5853460496234675, -373.9874144716864066, -372.3518521366060554 ) ) ;
#17162=ORIENTED_EDGE ( 'NONE', *, *, #24972, .T. ) ;
#17163=CARTESIAN_POINT ( 'NONE',  ( 754.9967657858570647, -217.5436935675107293, -365.0032342141425374 ) ) ;
#17168=CARTESIAN_POINT ( 'NONE',  ( 755.5713283507202505, -197.3618753856926560, -334.6858677611754729 ) ) ;
#17170=CARTESIAN_POINT ( 'NONE',  ( 767.8955696845333705, -0.4527844766023628176, -362.1676090361162323 ) ) ;
#17175=CARTESIAN_POINT ( 'NONE',  ( 788.8264449731200330, 2.819942796124898177, -363.6646147819171233 ) ) ;
#17178=CARTESIAN_POINT ( 'NONE',  ( 788.6739635108323228, -271.6454272087889876, -373.9316612368139090 ) ) ;
#17181=CARTESIAN_POINT ( 'NONE',  ( 804.4286716492782716, -209.3618753856926276, -345.3141322388244703 ) ) ;
#17182=CARTESIAN_POINT ( 'NONE',  ( 772.3691319403857278, -383.2601417444137155, -315.8894580844506663 ) ) ;
#17183=FACE_OUTER_BOUND ( 'NONE', #19730, .T. ) ;
#17185=CARTESIAN_POINT ( 'NONE',  ( 801.5560724626406000, -96.55451811788039151, -326.7756240680316182 ) ) ;
#17189=CARTESIAN_POINT ( 'NONE',  ( 798.0661480581538854, 21.46713098285774279, -309.5768839229118043 ) ) ;
#17190=CARTESIAN_POINT ( 'NONE',  ( 796.9462024416508257, -324.4527844766013231, -308.9653473494370246 ) ) ;
#17192=CARTESIAN_POINT ( 'NONE',  ( 755.5713283507202505, -77.36187538569302546, -334.6858677611754729 ) ) ;
#17194=CARTESIAN_POINT ( 'NONE',  ( 812.6845335610512393, -151.9874144716871740, -353.5525998758768651 ) ) ;
#17196=CARTESIAN_POINT ( 'NONE',  ( 814.5518280994195948, -423.7255117493281205, -332.4837098697145734 ) ) ;
#17200=CARTESIAN_POINT ( 'NONE',  ( 778.1981804954714335, -418.2709662947827383, -314.8072714833589885 ) ) ;
#17207=CARTESIAN_POINT ( 'NONE',  ( 804.9511171171677688, -245.8055962898686460, -335.8780910478229202 ) ) ;
#17209=CARTESIAN_POINT ( 'NONE',  ( 766.5853460496234675, -253.9874144716868329, -372.3518521366060554 ) ) ;
#17214=CARTESIAN_POINT ( 'NONE',  ( 793.2243759319678702, -50.53286901714203339, -318.4439275373583200 ) ) ;
#17215=CARTESIAN_POINT ( 'NONE',  ( 778.2165204200184689, -166.8164208402382087, -364.9363028652563230 ) ) ;
#17216=CARTESIAN_POINT ( 'NONE',  ( 771.2633955100217236, -191.9073299311471885, -363.4237431249939618 ) ) ;
#17218=CARTESIAN_POINT ( 'NONE',  ( 758.8095938919642549, -128.0891481129655176, -311.6929314249763365 ) ) ;
#17221=CARTESIAN_POINT ( 'NONE',  ( 794.9819416627830151, -108.9982390220565804, -319.9864689768909898 ) ) ;
#17222=CARTESIAN_POINT ( 'NONE',  ( 780.5236548040995785, -44.73633629969875614, -314.9735926884559944 ) ) ;
#17224=CARTESIAN_POINT ( 'NONE',  ( 766.9102291470427417, -378.5545181178795247, -318.6633372737382501 ) ) ;
#17229=CARTESIAN_POINT ( 'NONE',  ( 791.7608162188021197, 240.0000000000000853, -320.0000000000000000 ) ) ;
#17232=CARTESIAN_POINT ( 'NONE',  ( 755.8894580844503253, -351.8272453906068336, -332.3691319403863531 ) ) ;
#17233=CARTESIAN_POINT ( 'NONE',  ( 794.9819416627830151, -348.9982390220558273, -319.9864689768909898 ) ) ;
#17234=CARTESIAN_POINT ( 'NONE',  ( 747.6481478633932056, -133.0999726633348246, -353.4146539503763620 ) ) ;
#17239=CARTESIAN_POINT ( 'NONE',  ( 790.8726784830453198, -298.7146871989593251, -362.5472867521010585 ) ) ;
#17240=CARTESIAN_POINT ( 'NONE',  ( 792.1044303154645831, -444.4527844766009821, -317.8323909638837677 ) ) ;
#17241=CARTESIAN_POINT ( 'NONE',  ( 768.9521613784389729, -153.8272453906075157, -373.2346286133773106 ) ) ;
#17242=FACE_OUTER_BOUND ( 'NONE', #19051, .T. ) ;
#17247=CARTESIAN_POINT ( 'NONE',  ( 792.2312462859673587, -179.9073299311472454, -307.2067596250082602 ) ) ;
#17250=CARTESIAN_POINT ( 'NONE',  ( 815.2698199232961542, -304.8164208402376403, -342.5225473063383106 ) ) ;
#17257=CARTESIAN_POINT ( 'NONE',  ( 759.8311093483677041, -382.1692326535045936, -310.9282345327691814 ) ) ;
#17258=CARTESIAN_POINT ( 'NONE',  ( 746.8695393053150156, -125.9073299311474159, -327.6429770376306010 ) ) ;
#17259=CARTESIAN_POINT ( 'NONE',  ( 772.5602148656447525, -393.7255117493283478, -305.7998596910095443 ) ) ;
#17263=CARTESIAN_POINT ( 'NONE',  ( 803.8556311672234642, -153.6237781080508000, -365.6418435158340117 ) ) ;
#17270=CARTESIAN_POINT ( 'NONE',  ( 787.4397851343537695, -21.72551174932956641, -374.2001403089903988 ) ) ;
#17273=CARTESIAN_POINT ( 'NONE',  ( 754.3581564841646241, -425.4636090269703459, -316.1443688327762516 ) ) ;
#17276=CARTESIAN_POINT ( 'NONE',  ( 768.0187753319979720, -272.6346026584196807, -318.0580252608186242 ) ) ;
#17279=EDGE_CURVE ( 'NONE', #35219, #1648, #17130, .T. ) ;
#17280=AXIS2_PLACEMENT_3D ( 'NONE', #35188, #10245, #3564 ) ;
#17281=CARTESIAN_POINT ( 'NONE',  ( 804.8461984189677878, -242.1908817542435770, -336.9566956441385628 ) ) ;
#17282=CARTESIAN_POINT ( 'NONE',  ( 758.0580252608178853, -270.4527844766014937, -328.0187753319985404 ) ) ;
#17283=CARTESIAN_POINT ( 'NONE',  ( 804.6798772138710092, -447.7255117493281205, -334.6312213355106451 ) ) ;
#17284=CARTESIAN_POINT ( 'NONE',  ( 804.9363028652555840, -88.27096629478390355, -338.2165204200192079 ) ) ;
#17290=CARTESIAN_POINT ( 'NONE',  ( 799.9636004259356241, -46.91815448151694312, -311.2241431872006956 ) ) ;
#17296=EDGE_LOOP ( 'NONE', ( #32673, #8166, #11722, #4712 ) ) ;
#17297=CARTESIAN_POINT ( 'NONE',  ( 776.9254006560222479, 3.809118245755632959, -314.8983024940802125 ) ) ;
#17298=CARTESIAN_POINT ( 'NONE',  ( 808.3070685750232087, -66.99823902205670834, -361.1904061080339829 ) ) ;
#17300=CARTESIAN_POINT ( 'NONE',  ( 794.9819416627830151, -444.9982390220554862, -319.9864689768909898 ) ) ;
#17303=CARTESIAN_POINT ( 'NONE',  ( 813.1304606946830518, -209.9073299311470748, -352.3570229623690580 ) ) ;
#17309=CARTESIAN_POINT ( 'NONE',  ( 798.0661480581538854, -266.5328690171413655, -309.5768839229118043 ) ) ;
#17311=CARTESIAN_POINT ( 'NONE',  ( 754.9967657858570647, -289.5436935675103882, -365.0032342141425374 ) ) ;
#17315=CARTESIAN_POINT ( 'NONE',  ( 795.1360043628807261, -404.0891481129646081, -360.2193346964456282 ) ) ;
#17318=CARTESIAN_POINT ( 'NONE',  ( 803.8556311672234642, -33.62377810805116951, -365.6418435158340117 ) ) ;
#17319=CARTESIAN_POINT ( 'NONE',  ( 793.2243759319678702, -194.5328690171415644, -318.4439275373583200 ) ) ;
#17324=CARTESIAN_POINT ( 'NONE',  ( 802.1676090361156639, -86.63460265842023489, -327.8955696845344505 ) ) ;
#17325=CARTESIAN_POINT ( 'NONE',  ( 804.9511171171677688, -197.8055962898688733, -335.8780910478229202 ) ) ;
#17328=CARTESIAN_POINT ( 'NONE',  ( 747.3154664389472828, -43.98741447168752217, -326.4474001241230781 ) ) ;
#17333=CARTESIAN_POINT ( 'NONE',  ( 815.3608509340175488, -290.7363362996980527, -341.2497674668889545 ) ) ;
#17335=EDGE_CURVE ( 'NONE', #3566, #34365, #24276, .T. ) ;
#17341=CARTESIAN_POINT ( 'NONE',  ( 800.9840315886518738, -148.9181544815166092, -354.1144889064786412 ) ) ;
#17342=CARTESIAN_POINT ( 'NONE',  ( 774.6312213355099630, -143.3618753856927697, -364.6798772138717482 ) ) ;
#17343=CARTESIAN_POINT ( 'NONE',  ( 794.9819416627830151, -348.9982390220558273, -319.9864689768909898 ) ) ;
#17348=DIRECTION ( 'NONE',  ( -0.000000000000000000, 1.000000000000000000, -0.000000000000000000 ) ) ;
#17354=CARTESIAN_POINT ( 'NONE',  ( 750.9282345327678740, -376.9181544815159555, -319.8311093483690115 ) ) ;
#17361=CARTESIAN_POINT ( 'NONE',  ( 755.0636971347428243, -316.2709662947832499, -341.7834795799807353 ) ) ;
#17362=CARTESIAN_POINT ( 'NONE',  ( 802.5472867521000353, -220.3726999360618208, -350.8726784830461156 ) ) ;
#17366=CARTESIAN_POINT ( 'NONE',  ( 792.3570229623691148, -429.1800572038737300, -373.1304606946836770 ) ) ;
#17374=CARTESIAN_POINT ( 'NONE',  ( 805.0032342141412300, -37.54369356751132614, -314.9967657858571783 ) ) ;
#17375=CARTESIAN_POINT ( 'NONE',  ( 755.3201227861273992, -291.7255117493285752, -345.3687786644892981 ) ) ;
#17380=CARTESIAN_POINT ( 'NONE',  ( 797.8822607201568644, -30.55451811788062244, -370.1134526219340160 ) ) ;
#17381=CARTESIAN_POINT ( 'NONE',  ( 763.2154366446407039, -93.62377810805098477, -321.4292242960311228 ) ) ;
#17389=CARTESIAN_POINT ( 'NONE',  ( 757.8323909638827445, -50.63460265842036989, -352.1044303154654358 ) ) ;
#17390=CARTESIAN_POINT ( 'NONE',  ( 776.9566956441375396, -372.8965053807773415, -364.8461984189686405 ) ) ;
#17394=CARTESIAN_POINT ( 'NONE',  ( 786.2056067578752163, -395.8055962898682765, -374.4686193811670023 ) ) ;
#17402=CARTESIAN_POINT ( 'NONE',  ( 796.9462024416508257, -252.4527844766015789, -308.9653473494370246 ) ) ;
#17403=ADVANCED_FACE ( 'NONE', ( #45088 ), #13443, .F. ) ;
#17407=CARTESIAN_POINT ( 'NONE',  ( 759.7806653035535192, -198.9982390220562536, -324.8639956371181370 ) ) ;
#17409=CARTESIAN_POINT ( 'NONE',  ( 794.9819416627830151, -372.9982390220557704, -319.9864689768909898 ) ) ;
#17410=CARTESIAN_POINT ( 'NONE',  ( 791.9812246680005501, -20.63460265842048003, -361.9419747391813189 ) ) ;
#17419=CARTESIAN_POINT ( 'NONE',  ( 787.5531968255692163, -453.8272453906066630, -316.1348686366205811 ) ) ;
#17423=CARTESIAN_POINT ( 'NONE',  ( 813.5763878283155464, -267.8272453906071746, -351.1614460488615350 ) ) ;
#17426=CARTESIAN_POINT ( 'NONE',  ( 795.1360043628807261, -236.0891481129651766, -360.2193346964456282 ) ) ;
#17427=CARTESIAN_POINT ( 'NONE',  ( 773.3843516231979720, -397.4419599262317320, -364.4086373105754433 ) ) ;
#17430=CARTESIAN_POINT ( 'NONE',  ( 783.0745993439762742, -128.1908817542439465, -365.1016975059196739 ) ) ;
#17433=CARTESIAN_POINT ( 'NONE',  ( 747.3154664389472828, 4.012585528312341054, -326.4474001241230781 ) ) ;
#17434=CARTESIAN_POINT ( 'NONE',  ( 767.7687537140311633, -311.9073299311468759, -372.7932403749916830 ) ) ;
#17435=DIRECTION ( 'NONE',  ( 1.000000000000000000, 0.000000000000000000, 0.000000000000000000 ) ) ;
#17437=CARTESIAN_POINT ( 'NONE',  ( 794.9819416627830151, -84.99823902205663728, -319.9864689768909898 ) ) ;
#17439=CARTESIAN_POINT ( 'NONE',  ( 747.3154664389472828, -187.9874144716870603, -326.4474001241230781 ) ) ;
#17441=CARTESIAN_POINT ( 'NONE',  ( 767.6429770376289525, -441.1800572038735027, -306.8695393053162093 ) ) ;
#17446=CARTESIAN_POINT ( 'NONE',  ( 768.0187753319979720, -416.6346026584192259, -318.0580252608186242 ) ) ;
#17451=VERTEX_POINT ( 'NONE', #41614 ) ;
#17453=CARTESIAN_POINT ( 'NONE',  ( 804.9511171171677688, -269.8055962898686175, -335.8780910478229202 ) ) ;
#17455=CARTESIAN_POINT ( 'NONE',  ( 758.0141637701419768, -303.0783235625957559, -367.2620300519063790 ) ) ;
#17460=CARTESIAN_POINT ( 'NONE',  ( 772.3691319403857278, -47.26014174441477422, -315.8894580844506663 ) ) ;
#17461=CARTESIAN_POINT ( 'NONE',  ( 757.8323909638827445, -170.6346026584199649, -352.1044303154654358 ) ) ;
#17462=CARTESIAN_POINT ( 'NONE',  ( 804.4286716492782716, -209.3618753856926276, -345.3141322388244703 ) ) ;
#17464=CARTESIAN_POINT ( 'NONE',  ( 763.0537975583475827, -96.45278447660203369, -371.0346526505627480 ) ) ;
#17466=CARTESIAN_POINT ( 'NONE',  ( 755.5713283507202505, -101.3618753856929544, -334.6858677611754729 ) ) ;
#17469=CARTESIAN_POINT ( 'NONE',  ( 755.5913626894240451, -373.6454272087887034, -346.6156483768012890 ) ) ;
#17475=CARTESIAN_POINT ( 'NONE',  ( 799.9999999999993179, 205.0000000000000568, -339.9999999999999432 ) ) ;
#17478=CARTESIAN_POINT ( 'NONE',  ( 759.0159684113467620, -352.9181544815159555, -325.8855110935213020 ) ) ;
#17479=CARTESIAN_POINT ( 'NONE',  ( 791.9812246680005501, -356.6346026584193964, -361.9419747391813189 ) ) ;
#17481=CARTESIAN_POINT ( 'NONE',  ( 783.7953271457878373, -176.1908817542438328, -375.1787889125761239 ) ) ;
#17483=VECTOR ( 'NONE', #42742, 1000.000000000000000 ) ;
#17486=CARTESIAN_POINT ( 'NONE',  ( 786.6156483768007774, -289.4419599262321299, -315.5913626894246136 ) ) ;
#17488=CARTESIAN_POINT ( 'NONE',  ( 752.7379699480933368, -156.0090635724256742, -361.9858362298580232 ) ) ;
#17494=CARTESIAN_POINT ( 'NONE',  ( 782.5225473063383106, -190.2709662947835625, -375.2698199232970637 ) ) ;
#17497=CARTESIAN_POINT ( 'NONE',  ( 812.7932403749906598, -351.1800572038740142, -327.7687537140311633 ) ) ;
#17503=CARTESIAN_POINT ( 'NONE',  ( 812.6845335610512393, -391.9874144716864066, -353.5525998758768651 ) ) ;
#17505=CARTESIAN_POINT ( 'NONE',  ( 787.5162901302840055, -107.3618753856928976, -305.4481719005792684 ) ) ;
#17506=CARTESIAN_POINT ( 'NONE',  ( 782.5225473063381969, -430.2709662947827383, -375.2698199232970637 ) ) ;
#17510=CARTESIAN_POINT ( 'NONE',  ( 768.8385539511368734, -167.2601417444143976, -306.4236121716840557 ) ) ;
#17516=CARTESIAN_POINT ( 'NONE',  ( 765.0180583372156207, -144.9982390220564525, -360.0135310231089534 ) ) ;
#17519=CARTESIAN_POINT ( 'NONE',  ( 787.5162901302840055, -11.36187538569323863, -305.4481719005792684 ) ) ;
#17523=CARTESIAN_POINT ( 'NONE',  ( 805.6418435158337843, -413.4636090269704027, -363.8556311672236916 ) ) ;
#17527=CARTESIAN_POINT ( 'NONE',  ( 774.6858677611749044, -273.7255117493288026, -315.5713283507209894 ) ) ;
#17531=CARTESIAN_POINT ( 'NONE',  ( 776.9254006560222479, -260.1908817542435486, -314.8983024940802125 ) ) ;
#17532=CARTESIAN_POINT ( 'NONE',  ( 804.6798772138708955, -255.7255117493287742, -334.6312213355107019 ) ) ;
#17533=CARTESIAN_POINT ( 'NONE',  ( 809.6099558218720631, -452.9681489794449476, -335.1781210895659342 ) ) ;
#17534=CARTESIAN_POINT ( 'NONE',  ( 771.1735550268778070, -129.1800572038746111, -316.3353852180827630 ) ) ;
#17538=CARTESIAN_POINT ( 'NONE',  ( 804.1009440267234822, -47.46360902697148987, -314.0944755984392600 ) ) ;
#17545=CARTESIAN_POINT ( 'NONE',  ( 787.5531968255692163, -21.82724539060792424, -316.1348686366205811 ) ) ;
#17546=CARTESIAN_POINT ( 'NONE',  ( 815.2698199232962679, -112.8164208402383650, -342.5225473063383674 ) ) ;
#17550=CARTESIAN_POINT ( 'NONE',  ( 758.8095938919642549, -224.0891481129653187, -311.6929314249763365 ) ) ;
#17554=CARTESIAN_POINT ( 'NONE',  ( 811.6461892240364477, -268.7146871989595525, -324.1737431748509835 ) ) ;
#17556=CARTESIAN_POINT ( 'NONE',  ( 772.4837098697144029, -311.3618753856922581, -374.5518280994205611 ) ) ;
#17560=CARTESIAN_POINT ( 'NONE',  ( 788.7366044899766848, -371.9073299311465917, -316.5762568750059813 ) ) ;
#17562=CARTESIAN_POINT ( 'NONE',  ( 807.5423716828161105, -57.07832356259658013, -362.2119215644372048 ) ) ;
#17563=CARTESIAN_POINT ( 'NONE',  ( 783.0433043558608688, -192.8965053807779668, -315.1538015810313027 ) ) ;
#17566=ORIENTED_EDGE ( 'NONE', *, *, #39078, .T. ) ;
#17567=CARTESIAN_POINT ( 'NONE',  ( 769.1273215169530886, -190.7146871989597798, -317.4527132478988847 ) ) ;
#17570=CARTESIAN_POINT ( 'NONE',  ( 752.4576283171824116, -45.07832356259660145, -317.7880784355627952 ) ) ;
#17575=CARTESIAN_POINT ( 'NONE',  ( 797.8822607201568644, -318.5545181178796952, -370.1134526219340160 ) ) ;
#17579=CARTESIAN_POINT ( 'NONE',  ( 760.7433823573367135, -156.0090635724256742, -355.9930595647440441 ) ) ;
#17580=CARTESIAN_POINT ( 'NONE',  ( 762.3223304703356007, -151.5436935675109851, -322.3223304703362828 ) ) ;
#17581=CARTESIAN_POINT ( 'NONE',  ( 759.9864689768902508, -362.0891481129648923, -354.9819416627836404 ) ) ;
#17589=VERTEX_POINT ( 'NONE', #4426 ) ;
#17590=CARTESIAN_POINT ( 'NONE',  ( 749.5768839229115201, -372.5545181178796383, -358.0661480581553064 ) ) ;
#17594=CARTESIAN_POINT ( 'NONE',  ( 805.1927285166397041, -376.8164208402375834, -341.8018195045277707 ) ) ;
#17595=CARTESIAN_POINT ( 'NONE',  ( 799.9999999999993179, 205.0000000000000568, -319.9999999999999432 ) ) ;
#17596=CARTESIAN_POINT ( 'NONE',  ( 773.4516893846965786, -211.6454272087891582, -315.8398074228977066 ) ) ;
#17600=CARTESIAN_POINT ( 'NONE',  ( 777.5031285880264704, -430.8164208402374129, -374.9108240113588408 ) ) ;
#17601=DIRECTION ( 'NONE',  ( 0.000000000000000000, 0.000000000000000000, -1.000000000000000000 ) ) ;
#17606=CARTESIAN_POINT ( 'NONE',  ( 758.8095938919642549, -56.08914811296580893, -311.6929314249763365 ) ) ;
#17607=CARTESIAN_POINT ( 'NONE',  ( 762.3223304703356007, -271.5436935675106156, -322.3223304703362828 ) ) ;
#17612=CARTESIAN_POINT ( 'NONE',  ( 768.9521613784389729, -33.82724539060788516, -373.2346286133773106 ) ) ;
#17613=CARTESIAN_POINT ( 'NONE',  ( 804.1601925771018387, -79.44195992623286884, -346.5483106153029098 ) ) ;
#17619=CARTESIAN_POINT ( 'NONE',  ( 765.0180583372156207, -0.9982390220569063999, -360.0135310231089534 ) ) ;
#17620=CARTESIAN_POINT ( 'NONE',  ( 784.0799538623451781, -107.8055962898691433, -364.6971507214555572 ) ) ;
#17622=CARTESIAN_POINT ( 'NONE',  ( 795.1360043628807261, -68.08914811296575920, -360.2193346964456282 ) ) ;
#17625=CARTESIAN_POINT ( 'NONE',  ( 798.7617431975189675, -387.6237781080499758, -323.0428371773161871 ) ) ;
#17629=CARTESIAN_POINT ( 'NONE',  ( 813.2346286133761168, -389.2601417444136018, -328.9521613784389160 ) ) ;
#17636=CARTESIAN_POINT ( 'NONE',  ( 747.2067596250078623, -243.1800572038743269, -352.2312462859687230 ) ) ;
#17640=CARTESIAN_POINT ( 'NONE',  ( 757.8323909638828582, -242.6346026584197659, -352.1044303154654358 ) ) ;
#17641=ORIENTED_EDGE ( 'NONE', *, *, #33400, .T. ) ;
#17644=CARTESIAN_POINT ( 'NONE',  ( 791.9812246680005501, -356.6346026584193964, -361.9419747391813189 ) ) ;
#17645=CARTESIAN_POINT ( 'NONE',  ( 788.8264449731200330, -21.18005720387502677, -363.6646147819171233 ) ) ;
#17649=DIRECTION ( 'NONE',  ( 0.000000000000000000, 0.000000000000000000, 1.000000000000000000 ) ) ;
#17651=CARTESIAN_POINT ( 'NONE',  ( 762.3223304703356007, -31.54369356751135456, -322.3223304703362828 ) ) ;
#17655=CARTESIAN_POINT ( 'NONE',  ( 815.3608509340175488, -266.7363362996981095, -341.2497674668889545 ) ) ;
#17658=CARTESIAN_POINT ( 'NONE',  ( 771.2633955100217236, -239.9073299311470748, -363.4237431249939618 ) ) ;
#17659=CARTESIAN_POINT ( 'NONE',  ( 763.2154366446407039, -381.6237781080500326, -321.4292242960311228 ) ) ;
#17661=CARTESIAN_POINT ( 'NONE',  ( 779.4763451958990572, -128.7363362996984790, -365.0264073115438919 ) ) ;
#17663=CARTESIAN_POINT ( 'NONE',  ( 751.2241431872005251, 7.830767346494148740, -359.9636004259367610 ) ) ;
#17664=CARTESIAN_POINT ( 'NONE',  ( 792.2312462859673587, -299.9073299311468759, -307.2067596250082602 ) ) ;
#17667=CARTESIAN_POINT ( 'NONE',  ( 795.1360043628807261, -68.08914811296575920, -360.2193346964456282 ) ) ;
#17670=CARTESIAN_POINT ( 'NONE',  ( 778.7502325331095108, -216.3510508353233490, -304.6391490659818828 ) ) ;
#17672=CARTESIAN_POINT ( 'NONE',  ( 787.5162901302840055, -443.3618753856917465, -305.4481719005792684 ) ) ;
#17677=CARTESIAN_POINT ( 'NONE',  ( 788.7366044899766848, -443.9073299311464780, -316.5762568750059813 ) ) ;
#17685=CARTESIAN_POINT ( 'NONE',  ( 796.7845633553578182, -297.6237781080502600, -358.5707757039688204 ) ) ;
#17687=CARTESIAN_POINT ( 'NONE',  ( 745.1769319972822814, -305.8055962898684470, -346.2694204179732083 ) ) ;
#17692=CARTESIAN_POINT ( 'NONE',  ( 795.9930595647434757, -51.07832356259657303, -320.7433823573372820 ) ) ;
#17693=CARTESIAN_POINT ( 'NONE',  ( 805.1927285166397041, -160.8164208402382371, -341.8018195045277707 ) ) ;
#17694=CARTESIAN_POINT ( 'NONE',  ( 791.9812246680005501, -212.6346026584198796, -361.9419747391813189 ) ) ;
#17696=CARTESIAN_POINT ( 'NONE',  ( 787.5162901302840055, -131.3618753856928834, -305.4481719005792684 ) ) ;
#17698=CARTESIAN_POINT ( 'NONE',  ( 785.3687786644885591, -131.3618753856928549, -315.3201227861280813 ) ) ;
#17700=CARTESIAN_POINT ( 'NONE',  ( 802.5472867521000353, -388.3726999360613945, -350.8726784830461156 ) ) ;
#17708=CARTESIAN_POINT ( 'NONE',  ( 799.2566176426618085, -384.0090635724249637, -324.0069404352559559 ) ) ;
#17709=CARTESIAN_POINT ( 'NONE',  ( 756.5762568750052424, -363.1800572038739006, -348.7366044899774238 ) ) ;
#17710=CARTESIAN_POINT ( 'NONE',  ( 788.6739635108323228, -175.6454272087892718, -373.9316612368139090 ) ) ;
#17714=CARTESIAN_POINT ( 'NONE',  ( 755.5713283507202505, -437.3618753856919170, -334.6858677611754729 ) ) ;
#17715=CARTESIAN_POINT ( 'NONE',  ( 810.4231160770870019, -168.5545181178802352, -321.9338519418446936 ) ) ;
#17720=CARTESIAN_POINT ( 'NONE',  ( 751.6929314249750860, -198.9982390220562536, -318.8095938919659034 ) ) ;
#17725=CARTESIAN_POINT ( 'NONE',  ( 764.3348316497523456, -94.71468719896007826, -308.6759233522265617 ) ) ;
#17727=CARTESIAN_POINT ( 'NONE',  ( 792.3570229623688874, -333.1800572038740142, -373.1304606946836202 ) ) ;
#17729=CARTESIAN_POINT ( 'NONE',  ( 759.9999999999992042, 205.0000000000000568, -339.9999999999999432 ) ) ;
#17732=CARTESIAN_POINT ( 'NONE',  ( 745.1769319972822814, -425.8055962898680491, -346.2694204179732083 ) ) ;
#17733=CARTESIAN_POINT ( 'NONE',  ( 777.5031285880264704, -142.8164208402382656, -374.9108240113588408 ) ) ;
#17734=CARTESIAN_POINT ( 'NONE',  ( 777.5031285880264704, -406.8164208402375266, -374.9108240113588408 ) ) ;
#17735=DIRECTION ( 'NONE',  ( 0.000000000000000000, 0.000000000000000000, -1.000000000000000000 ) ) ;
#17738=EDGE_CURVE ( 'NONE', #19609, #16032, #25663, .T. ) ;
#17739=CARTESIAN_POINT ( 'NONE',  ( 810.1134526219336749, -176.5328690171416213, -357.8822607201570349 ) ) ;
#17745=CARTESIAN_POINT ( 'NONE',  ( 782.4968714119720516, -58.81642084023854267, -305.0891759886411023 ) ) ;
#17748=CARTESIAN_POINT ( 'NONE',  ( 746.4236121716829757, -447.8272453906067199, -328.8385539511384650 ) ) ;
#17752=CARTESIAN_POINT ( 'NONE',  ( 804.9363028652555840, -304.2709662947832499, -338.2165204200192079 ) ) ;
#17756=CARTESIAN_POINT ( 'NONE',  ( 793.0897708529556667, -246.5545181178799510, -361.3366627262616362 ) ) ;
#17757=CARTESIAN_POINT ( 'NONE',  ( 767.8955696845333705, -240.4527844766015221, -362.1676090361162323 ) ) ;
#17758=CARTESIAN_POINT ( 'NONE',  ( 803.6646147819162707, -449.9073299311464211, -348.8264449731211130 ) ) ;
#17759=CARTESIAN_POINT ( 'NONE',  ( 771.1735550268778070, -105.1800572038747248, -316.3353852180827630 ) ) ;
#17764=CARTESIAN_POINT ( 'NONE',  ( 745.5313806188320314, -63.28179084515324604, -333.7943932421247268 ) ) ;
#17770=CARTESIAN_POINT ( 'NONE',  ( 799.2566176426618085, -0.009063572426172561425, -324.0069404352559559 ) ) ;
#17771=CARTESIAN_POINT ( 'NONE',  ( 745.4481719005789273, -99.72551174932931417, -347.5162901302853697 ) ) ;
#17775=CARTESIAN_POINT ( 'NONE',  ( 749.2812353651451076, -246.4527844766016074, -323.2262854647983090 ) ) ;
#17779=CARTESIAN_POINT ( 'NONE',  ( 768.8385539511368734, -287.2601417444140566, -306.4236121716840557 ) ) ;
#17781=CARTESIAN_POINT ( 'NONE',  ( 811.0346526505616112, -302.6346026584196238, -323.0537975583477532 ) ) ;
#17785=CARTESIAN_POINT ( 'NONE',  ( 792.1044303154645831, -396.4527844766010389, -317.8323909638837677 ) ) ;
#17787=CARTESIAN_POINT ( 'NONE',  ( 764.8639956371174549, -200.0891481129653187, -319.7806653035542013 ) ) ;
#17788=CARTESIAN_POINT ( 'NONE',  ( 815.0009284576459549, -102.3510508353236901, -338.7629533639073429 ) ) ;
#17792=CARTESIAN_POINT ( 'NONE',  ( 772.3691319403857278, -215.2601417444141987, -315.8894580844506663 ) ) ;
#17795=CARTESIAN_POINT ( 'NONE',  ( 788.7631598425961101, -49.44195992623295410, -305.7194118038759143 ) ) ;
#17800=CARTESIAN_POINT ( 'NONE',  ( 788.6739635108323228, -319.6454272087888739, -373.9316612368139090 ) ) ;
#17803=CARTESIAN_POINT ( 'NONE',  ( 763.8424801807145741, -162.0090635724256742, -320.5453621957614700 ) ) ;
#17804=CARTESIAN_POINT ( 'NONE',  ( 781.8018195045266339, -142.2709662947837330, -365.1927285166406705 ) ) ;
#17805=CARTESIAN_POINT ( 'NONE',  ( 767.8955696845334842, -336.4527844766012663, -362.1676090361161755 ) ) ;
#17815=CARTESIAN_POINT ( 'NONE',  ( 764.1737431748507561, -394.3726999360613377, -371.6461892240376415 ) ) ;
#17816=CARTESIAN_POINT ( 'NONE',  ( 792.2312462859673587, 12.09267006885214180, -307.2067596250082602 ) ) ;
#17819=CARTESIAN_POINT ( 'NONE',  ( 800.2193346964447755, -354.9982390220557704, -355.1360043628815788 ) ) ;
#17822=CARTESIAN_POINT ( 'NONE',  ( 755.5913626894240451, -205.6454272087891297, -346.6156483768012890 ) ) ;
#17826=CARTESIAN_POINT ( 'NONE',  ( 796.9462024416508257, -420.4527844766009821, -308.9653473494370246 ) ) ;
#17829=CARTESIAN_POINT ( 'NONE',  ( 801.6550554848130332, -456.5036469134198001, -360.7619500998734452 ) ) ;
#17831=CARTESIAN_POINT ( 'NONE',  ( 747.2067596250078623, -51.18005720387493085, -352.2312462859687230 ) ) ;
#17832=CARTESIAN_POINT ( 'NONE',  ( 788.7366044899766848, -275.9073299311469896, -316.5762568750059813 ) ) ;
#17837=CARTESIAN_POINT ( 'NONE',  ( 814.2805881961230625, -73.64542720878957027, -331.2368401574024119 ) ) ;
#17838=CARTESIAN_POINT ( 'NONE',  ( 805.0264073115434940, -78.35105083532376113, -339.4763451958999099 ) ) ;
#17842=CARTESIAN_POINT ( 'NONE',  ( 804.4286716492782716, 6.638124614306706306, -345.3141322388244703 ) ) ;
#17844=CARTESIAN_POINT ( 'NONE',  ( 803.6646147819161570, -113.9073299311474301, -348.8264449731210561 ) ) ;
#17845=CARTESIAN_POINT ( 'NONE',  ( 802.7791456095903868, -388.7146871989592114, -329.0155153010375102 ) ) ;
#17849=CARTESIAN_POINT ( 'NONE',  ( 768.8385539511368734, -383.2601417444137155, -306.4236121716840557 ) ) ;
#17853=ORIENTED_EDGE ( 'NONE', *, *, #12031, .T. ) ;
#17854=( NAMED_UNIT ( * ) PLANE_ANGLE_UNIT ( ) SI_UNIT ( $, .RADIAN. ) );
#17855=CARTESIAN_POINT ( 'NONE',  ( 759.0252816721024374, -240.9982390220561683, -368.0189434323527280 ) ) ;
#17859=CARTESIAN_POINT ( 'NONE',  ( 754.8072714833583632, -244.8164208402379245, -338.1981804954721156 ) ) ;
#17861=CARTESIAN_POINT ( 'NONE',  ( 781.7834795799800531, -370.8164208402375834, -315.0636971347436202 ) ) ;
#17862=CARTESIAN_POINT ( 'NONE',  ( 804.4286716492782716, -17.36187538569322086, -345.3141322388244703 ) ) ;
#17868=CARTESIAN_POINT ( 'NONE',  ( 788.7366044899766848, -11.90732993114778182, -316.5762568750059813 ) ) ;
#17869=CARTESIAN_POINT ( 'NONE',  ( 799.9999999999993179, -512.9681489794448908, -339.9999999999999432 ) ) ;
#17872=CARTESIAN_POINT ( 'NONE',  ( 750.9282345327678740, -256.9181544815163534, -319.8311093483690115 ) ) ;
#17876=CARTESIAN_POINT ( 'NONE',  ( 800.2193346964447755, -258.9982390220561115, -355.1360043628815788 ) ) ;
#17877=CARTESIAN_POINT ( 'NONE',  ( 798.7617431975189675, -411.6237781080499758, -323.0428371773161871 ) ) ;
#17879=CARTESIAN_POINT ( 'NONE',  ( 798.5707757039680246, -125.4636090269712412, -356.7845633553585003 ) ) ;
#17882=CARTESIAN_POINT ( 'NONE',  ( 746.0683387631852383, 4.558040073766884248, -331.3260364891676204 ) ) ;
#17883=CARTESIAN_POINT ( 'NONE',  ( 751.9810565676468741, -314.0891481129650629, -360.9747183278973921 ) ) ;
#17887=CARTESIAN_POINT ( 'NONE',  ( 766.5853460496234675, -205.9874144716870035, -372.3518521366060554 ) ) ;
#17889=CARTESIAN_POINT ( 'NONE',  ( 767.7687537140311633, -431.9073299311464211, -372.7932403749916830 ) ) ;
#17895=CARTESIAN_POINT ( 'NONE',  ( 787.6308680596127942, 12.73985825558503926, -364.1105419155492768 ) ) ;
#17898=EDGE_CURVE ( 'NONE', #15183, #29231, #22636, .T. ) ;
#17902=CARTESIAN_POINT ( 'NONE',  ( 754.9735926884551418, -282.3510508353230080, -340.5236548041000333 ) ) ;
#17904=CARTESIAN_POINT ( 'NONE',  ( 800.1688906516307043, -298.1692326535049347, -369.0717654672308186 ) ) ;
#17909=CARTESIAN_POINT ( 'NONE',  ( 756.1348686366196716, -41.26014174441479554, -347.5531968255698416 ) ) ;
#17910=CARTESIAN_POINT ( 'NONE',  ( 759.9864689768902508, -170.0891481129654608, -354.9819416627836404 ) ) ;
#17911=CARTESIAN_POINT ( 'NONE',  ( 768.0187753319979720, -224.6346026584198228, -318.0580252608186242 ) ) ;
#17913=CARTESIAN_POINT ( 'NONE',  ( 796.9462024416508257, -132.4527844766018916, -308.9653473494370246 ) ) ;
#17915=CARTESIAN_POINT ( 'NONE',  ( 755.3201227861273992, -147.7255117493291721, -345.3687786644892981 ) ) ;
#17917=CARTESIAN_POINT ( 'NONE',  ( 780.5236548040995785, -404.7363362996975980, -314.9735926884559944 ) ) ;
#17925=VERTEX_POINT ( 'NONE', #40651 ) ;
#17926=CARTESIAN_POINT ( 'NONE',  ( 780.5236548040995785, -404.7363362996975980, -314.9735926884559944 ) ) ;
#17929=CARTESIAN_POINT ( 'NONE',  ( 764.1737431748507561, -178.3726999360619629, -371.6461892240376415 ) ) ;
#17934=CARTESIAN_POINT ( 'NONE',  ( 766.7756240680305382, -302.5328690171411949, -361.5560724626415663 ) ) ;
#17936=CARTESIAN_POINT ( 'NONE',  ( 813.5763878283155464, -171.8272453906074304, -351.1614460488615350 ) ) ;
#17942=CARTESIAN_POINT ( 'NONE',  ( 758.8095938919644823, -200.0891481129653471, -311.6929314249762797 ) ) ;
#17944=CARTESIAN_POINT ( 'NONE',  ( 801.9419747391806368, 5.547215523397618142, -351.9812246680014027 ) ) ;
#17946=CARTESIAN_POINT ( 'NONE',  ( 781.2497674668890113, -108.3510508353236759, -375.3608509340180603 ) ) ;
#17948=CARTESIAN_POINT ( 'NONE',  ( 745.0891759886404770, -340.2709662947831362, -342.4968714119734159 ) ) ;
#17954=CARTESIAN_POINT ( 'NONE',  ( 807.5423716828161105, -417.0783235625954148, -362.2119215644372048 ) ) ;
#17955=CARTESIAN_POINT ( 'NONE',  ( 759.0252816721024374, -408.9982390220556567, -368.0189434323527280 ) ) ;
#17961=CARTESIAN_POINT ( 'NONE',  ( 748.3538107759620743, -184.7146871989598083, -355.8262568251490165 ) ) ;
#17968=CARTESIAN_POINT ( 'NONE',  ( 777.5031285880264704, -46.81642084023858530, -374.9108240113588408 ) ) ;
#17971=CARTESIAN_POINT ( 'NONE',  ( 778.7629533639073998, -440.7363362996975980, -375.0009284576466371 ) ) ;
#17976=CARTESIAN_POINT ( 'NONE',  ( 788.8264449731200330, -309.1800572038740711, -363.6646147819171233 ) ) ;
#17981=CARTESIAN_POINT ( 'NONE',  ( 769.0155153010367712, -298.3726999360616787, -362.7791456095907279 ) ) ;
#17982=CARTESIAN_POINT ( 'NONE',  ( 792.1044303154645831, -252.4527844766015789, -317.8323909638837677 ) ) ;
#17984=CARTESIAN_POINT ( 'NONE',  ( 764.8639956371174549, -128.0891481129655176, -319.7806653035542013 ) ) ;
#17986=LINE ( 'NONE', #1336, #20395 ) ;
#17988=CARTESIAN_POINT ( 'NONE',  ( 773.7305795820266212, -81.28179084515319630, -374.8230680027170365 ) ) ;
#17995=CARTESIAN_POINT ( 'NONE',  ( 787.5531968255692163, -45.82724539060783542, -316.1348686366205811 ) ) ;
#17998=CARTESIAN_POINT ( 'NONE',  ( 801.1904061080338124, -116.0891481129656313, -368.3070685750236066 ) ) ;
#18002=CARTESIAN_POINT ( 'NONE',  ( 746.8695393053150156, -245.9073299311469896, -327.6429770376306010 ) ) ;
#18006=CARTESIAN_POINT ( 'NONE',  ( 812.6845335610512393, -295.9874144716866908, -353.5525998758768651 ) ) ;
#18009=CARTESIAN_POINT ( 'NONE',  ( 782.5225473063381969, -310.2709662947832499, -375.2698199232970637 ) ) ;
#18013=CARTESIAN_POINT ( 'NONE',  ( 778.2165204200184689, -382.8164208402374697, -364.9363028652563230 ) ) ;
#18015=CARTESIAN_POINT ( 'NONE',  ( 804.9363028652555840, -208.2709662947835341, -338.2165204200192079 ) ) ;
#18016=CARTESIAN_POINT ( 'NONE',  ( 788.7631598425961101, -97.44195992623281199, -305.7194118038759143 ) ) ;
#18020=CARTESIAN_POINT ( 'NONE',  ( 764.0069404352550464, -207.0783235625960685, -359.2566176426627180 ) ) ;
#18022=CARTESIAN_POINT ( 'NONE',  ( 748.3538107759620743, -16.71468719896031985, -355.8262568251490165 ) ) ;
#18024=CARTESIAN_POINT ( 'NONE',  ( 802.7276637122909051, -452.9681489794449476, -352.0069550970126784 ) ) ;
#18026=ORIENTED_EDGE ( 'NONE', *, *, #33961, .F. ) ;
#18028=CARTESIAN_POINT ( 'NONE',  ( 812.3518521366052028, -337.0999726633342561, -326.5853460496235243 ) ) ;
#18031=CARTESIAN_POINT ( 'NONE',  ( 758.4439275373578084, -180.5545181178801499, -353.2243759319684386 ) ) ;
#18032=CARTESIAN_POINT ( 'NONE',  ( 804.6798772138708955, -135.7255117493291152, -334.6312213355107019 ) ) ;
#18033=CARTESIAN_POINT ( 'NONE',  ( 803.4237431249931660, -351.1800572038740142, -331.2633955100225194 ) ) ;
#18040=VECTOR ( 'NONE', #4993, 1000.000000000000000 ) ;
#18043=ORIENTED_EDGE ( 'NONE', *, *, #20725, .F. ) ;
#18044=CARTESIAN_POINT ( 'NONE',  ( 768.9521613784389729, -369.8272453906068904, -373.2346286133773106 ) ) ;
#18045=CARTESIAN_POINT ( 'NONE',  ( 792.3570229623691148, 2.819942796124898621, -373.1304606946836770 ) ) ;
#18048=CARTESIAN_POINT ( 'NONE',  ( 755.3201227861273992, -363.7255117493284047, -345.3687786644892981 ) ) ;
#18051=CARTESIAN_POINT ( 'NONE',  ( 804.4086373105744769, -217.6454272087891582, -333.3843516231986541 ) ) ;
#18055=CARTESIAN_POINT ( 'NONE',  ( 777.5031285880264704, -406.8164208402375266, -374.9108240113588408 ) ) ;
#18062=CARTESIAN_POINT ( 'NONE',  ( 796.7737145352015204, -68.63460265842033436, -370.7187646348536987 ) ) ;
#18063=CARTESIAN_POINT ( 'NONE',  ( 754.8072714833581358, -292.8164208402376971, -338.1981804954720587 ) ) ;
#18067=CARTESIAN_POINT ( 'NONE',  ( 791.0478386215596629, -69.82724539060775726, -306.7653713866226326 ) ) ;
#18068=CARTESIAN_POINT ( 'NONE',  ( 773.3843516231979720, -85.44195992623282621, -364.4086373105754433 ) ) ;
#18074=CARTESIAN_POINT ( 'NONE',  ( 802.1676090361156639, -86.63460265842023489, -327.8955696845344505 ) ) ;
#18077=CARTESIAN_POINT ( 'NONE',  ( 794.1144889064781864, -394.1692326535045368, -360.9840315886528401 ) ) ;
#18080=CARTESIAN_POINT ( 'NONE',  ( 745.1769319972822814, -401.8055962898681059, -346.2694204179732083 ) ) ;
#18081=CARTESIAN_POINT ( 'NONE',  ( 779.9999999999992042, -452.9681489794448339, -370.0000000000000568 ) ) ;
#18086=CARTESIAN_POINT ( 'NONE',  ( 745.4481719005789273, -243.7255117493287742, -347.5162901302853129 ) ) ;
#18091=CARTESIAN_POINT ( 'NONE',  ( 775.8780910478218402, -57.28179084515326736, -364.9511171171680530 ) ) ;
#18092=CARTESIAN_POINT ( 'NONE',  ( 803.6646147819162707, -257.9073299311469327, -348.8264449731211130 ) ) ;
#18096=CARTESIAN_POINT ( 'NONE',  ( 764.8639956371174549, -344.0891481129647786, -319.7806653035542013 ) ) ;
#18097=CARTESIAN_POINT ( 'NONE',  ( 756.3353852180819104, -5.907329931147798696, -331.1735550268788302 ) ) ;
#18103=CARTESIAN_POINT ( 'NONE',  ( 781.7834795799800531, -34.81642084023861372, -315.0636971347436202 ) ) ;
#18104=DIRECTION ( 'NONE',  ( 0.000000000000000000, 0.000000000000000000, 1.000000000000000000 ) ) ;
#18107=CARTESIAN_POINT ( 'NONE',  ( 749.5768839229115201, -276.5545181178798657, -358.0661480581553064 ) ) ;
#18112=CARTESIAN_POINT ( 'NONE',  ( 803.4237431249931660, -255.1800572038742700, -331.2633955100225194 ) ) ;
#18114=CARTESIAN_POINT ( 'NONE',  ( 798.5707757039680246, -101.4636090269713264, -356.7845633553585003 ) ) ;
#18118=CARTESIAN_POINT ( 'NONE',  ( 801.9858362298568863, 20.92167643740319605, -312.7379699480935642 ) ) ;
#18119=CARTESIAN_POINT ( 'NONE',  ( 772.4837098697145166, -311.3618753856923149, -374.5518280994205611 ) ) ;
#18123=CARTESIAN_POINT ( 'NONE',  ( 746.7653713866222915, -209.2601417444142839, -351.0478386215610271 ) ) ;
#18125=CARTESIAN_POINT ( 'NONE',  ( 812.7932403749906598, -447.1800572038736732, -327.7687537140311633 ) ) ;
#18131=CARTESIAN_POINT ( 'NONE',  ( 804.9511171171677688, 18.19440371013048008, -335.8780910478229202 ) ) ;
#18132=AXIS2_PLACEMENT_3D ( 'NONE', #17475, #24596, #41728 ) ;
#18134=CARTESIAN_POINT ( 'NONE',  ( 767.9999999999992042, 205.0000000000000568, -329.9999999999999432 ) ) ;
#18138=CARTESIAN_POINT ( 'NONE',  ( 770.0799878456142551, -277.9874144716867477, -362.9823548866085616 ) ) ;
#18140=CARTESIAN_POINT ( 'NONE',  ( 754.0944755984390895, -279.6237781080503737, -364.1009440267246760 ) ) ;
#18146=AXIS2_PLACEMENT_3D ( 'NONE', #3061, #10218, #31236 ) ;
#18147=CARTESIAN_POINT ( 'NONE',  ( 755.5713283507202505, -173.3618753856927128, -334.6858677611754729 ) ) ;
#18148=CARTESIAN_POINT ( 'NONE',  ( 788.8264449731200330, -213.1800572038743553, -363.6646147819171233 ) ) ;
#18152=CARTESIAN_POINT ( 'NONE',  ( 747.2067596250078623, -147.1800572038746395, -352.2312462859687230 ) ) ;
#18156=CARTESIAN_POINT ( 'NONE',  ( 768.0187753319979720, -152.6346026584200786, -318.0580252608186242 ) ) ;
#18158=CARTESIAN_POINT ( 'NONE',  ( 757.4527132478984868, -376.3726999360614514, -329.1273215169538844 ) ) ;
#18162=DIRECTION ( 'NONE',  ( 0.000000000000000000, 0.000000000000000000, -1.000000000000000000 ) ) ;
#18166=CARTESIAN_POINT ( 'NONE',  ( 793.0897708529556667, -390.5545181178794678, -361.3366627262616362 ) ) ;
#18168=CARTESIAN_POINT ( 'NONE',  ( 744.6391490659812007, -158.7363362996984222, -338.7502325331110455 ) ) ;
#18173=CARTESIAN_POINT ( 'NONE',  ( 795.9930595647434757, -315.0783235625957559, -320.7433823573372820 ) ) ;
#18174=CARTESIAN_POINT ( 'NONE',  ( 794.9819416627830151, -444.9982390220554862, -319.9864689768909898 ) ) ;
#18175=CARTESIAN_POINT ( 'NONE',  ( 797.8822607201568644, -174.5545181178801784, -370.1134526219340160 ) ) ;
#18181=CARTESIAN_POINT ( 'NONE',  ( 777.5031285880264704, -190.8164208402381234, -374.9108240113588408 ) ) ;
#18183=CARTESIAN_POINT ( 'NONE',  ( 771.2633955100217236, 0.09267006885218045942, -363.4237431249939618 ) ) ;
#18186=CARTESIAN_POINT ( 'NONE',  ( 754.0944755984390895, -87.62377810805102740, -364.1009440267246760 ) ) ;
#18188=CARTESIAN_POINT ( 'NONE',  ( 763.2262854647970016, -344.6346026584195101, -309.2812353651462445 ) ) ;
#18194=CARTESIAN_POINT ( 'NONE',  ( 783.7566961878529810, -408.8965053807772847, -305.1792804349288417 ) ) ;
#18195=CARTESIAN_POINT ( 'NONE',  ( 759.0252816721024374, -432.9982390220555999, -368.0189434323527280 ) ) ;
#18201=CARTESIAN_POINT ( 'NONE',  ( 800.1688906516307043, -202.1692326535051905, -369.0717654672308186 ) ) ;
#18205=VERTEX_POINT ( 'NONE', #40878 ) ;
#18208=EDGE_CURVE ( 'NONE', #24210, #17589, #4808, .T. ) ;
#18209=CARTESIAN_POINT ( 'NONE',  ( 800.9747183278959710, -36.99823902205679360, -311.9810565676471583 ) ) ;
#18213=CARTESIAN_POINT ( 'NONE',  ( 766.4474001241216001, -451.0999726633339151, -307.3154664389482491 ) ) ;
#18222=CARTESIAN_POINT ( 'NONE',  ( 802.5472867521000353, -292.3726999360616219, -350.8726784830461156 ) ) ;
#18223=CARTESIAN_POINT ( 'NONE',  ( 781.8018195045266339, -286.2709662947833635, -365.1927285166406705 ) ) ;
#18225=CARTESIAN_POINT ( 'NONE',  ( 802.1676090361156639, -134.6346026584201070, -327.8955696845344505 ) ) ;
#18232=CARTESIAN_POINT ( 'NONE',  ( 778.7629533639073998, -80.73633629969864955, -375.0009284576466371 ) ) ;
#18239=CARTESIAN_POINT ( 'NONE',  ( 796.1575198192839480, -54.00906357242601530, -359.4546378042384163 ) ) ;
#18240=CARTESIAN_POINT ( 'NONE',  ( 763.0537975583476964, -120.4527844766019768, -371.0346526505628617 ) ) ;
#18245=CARTESIAN_POINT ( 'NONE',  ( 744.7301800767019131, -220.8164208402379529, -337.4774526936615757 ) ) ;
#18249=CARTESIAN_POINT ( 'NONE',  ( 803.8556311672234642, -321.6237781080502600, -365.6418435158340117 ) ) ;
#18253=CARTESIAN_POINT ( 'NONE',  ( 805.0032342141412300, -301.5436935675105588, -314.9967657858571783 ) ) ;
#18257=CARTESIAN_POINT ( 'NONE',  ( 765.0180583372156207, -408.9982390220556567, -360.0135310231089534 ) ) ;
#18258=VECTOR ( 'NONE', #29901, 1000.000000000000000 ) ;
#18261=CARTESIAN_POINT ( 'NONE',  ( 783.7566961878529810, -72.89650538077830788, -305.1792804349288417 ) ) ;
#18264=ORIENTED_EDGE ( 'NONE', *, *, #1528, .T. ) ;
#18265=CARTESIAN_POINT ( 'NONE',  ( 776.9566956441375396, -204.8965053807779100, -364.8461984189686405 ) ) ;
#18269=CARTESIAN_POINT ( 'NONE',  ( 778.7502325331095108, -24.35105083532392811, -304.6391490659818828 ) ) ;
#18272=CARTESIAN_POINT ( 'NONE',  ( 799.9999999999993179, 205.0000000000000568, -360.0000000000000000 ) ) ;
#18275=CARTESIAN_POINT ( 'NONE',  ( 754.3581564841646241, -329.4636090269706870, -316.1443688327762516 ) ) ;
#18278=CARTESIAN_POINT ( 'NONE',  ( 772.4468031744293057, -201.8272453906073451, -363.8651313633793620 ) ) ;
#18279=CARTESIAN_POINT ( 'NONE',  ( 754.8072714833581358, -196.8164208402380950, -338.1981804954720587 ) ) ;
#18280=CARTESIAN_POINT ( 'NONE',  ( 774.6312213355098493, -359.3618753856921444, -364.6798772138717482 ) ) ;
#18282=CARTESIAN_POINT ( 'NONE',  ( 789.5670355615794733, -453.0432664090020012, -363.0970091259334822 ) ) ;
#18289=CARTESIAN_POINT ( 'NONE',  ( 807.2620300519052989, -408.0090635724249069, -318.0141637701419768 ) ) ;
#18290=CARTESIAN_POINT ( 'NONE',  ( 810.7187646348534145, 5.547215523397618142, -356.7737145352016341 ) ) ;
#18293=CARTESIAN_POINT ( 'NONE',  ( 768.0187753319979720, -368.6346026584193964, -318.0580252608186242 ) ) ;
#18297=CARTESIAN_POINT ( 'NONE',  ( 790.0220218866281812, -271.0999726633344267, -363.2186876482849129 ) ) ;
#18301=CARTESIAN_POINT ( 'NONE',  ( 801.1904061080338124, -452.0891481129646081, -368.3070685750236066 ) ) ;
#18307=CARTESIAN_POINT ( 'NONE',  ( 772.5602148656447525, -105.7255117493293000, -305.7998596910095443 ) ) ;
#18308=CARTESIAN_POINT ( 'NONE',  ( 768.0187753319979720, -272.6346026584196807, -318.0580252608186242 ) ) ;
#18312=CARTESIAN_POINT ( 'NONE',  ( 814.4686193811664907, -75.28179084515321051, -346.2056067578752732 ) ) ;
#18313=CARTESIAN_POINT ( 'NONE',  ( 783.0433043558608688, -96.89650538077825104, -315.1538015810313027 ) ) ;
#18318=CARTESIAN_POINT ( 'NONE',  ( 757.2208543904082489, -112.7146871989600356, -350.9844846989624330 ) ) ;
#18320=CARTESIAN_POINT ( 'NONE',  ( 756.3353852180819104, -101.9073299311474727, -331.1735550268788302 ) ) ;
#18321=CARTESIAN_POINT ( 'NONE',  ( 803.2186876482843445, -415.9874144716862361, -350.0220218866286928 ) ) ;
#18324=CARTESIAN_POINT ( 'NONE',  ( 805.9055244015594326, -387.6237781080499758, -315.8990559732753240 ) ) ;
#18332=CARTESIAN_POINT ( 'NONE',  ( 799.2566176426618085, -72.00906357242594424, -324.0069404352559559 ) ) ;
#18334=CARTESIAN_POINT ( 'NONE',  ( 801.9419747391806368, -258.4527844766016074, -351.9812246680014027 ) ) ;
#18336=CARTESIAN_POINT ( 'NONE',  ( 805.1927285166397041, -400.8164208402373561, -341.8018195045277707 ) ) ;
#18337=CARTESIAN_POINT ( 'NONE',  ( 791.9812246680005501, -44.63460265842040542, -361.9419747391813189 ) ) ;
#18341=CARTESIAN_POINT ( 'NONE',  ( 800.0135310231082713, -14.08914811296595460, -325.0180583372163028 ) ) ;
#18345=CARTESIAN_POINT ( 'NONE',  ( 809.0717654672305343, -316.9181544815160692, -360.1688906516309885 ) ) ;
#18349=CARTESIAN_POINT ( 'NONE',  ( 767.8955696845333705, -264.4527844766016074, -362.1676090361162323 ) ) ;
#18351=CARTESIAN_POINT ( 'NONE',  ( 773.4516893846965786, -115.6454272087894424, -315.8398074228977066 ) ) ;
#18354=CARTESIAN_POINT ( 'NONE',  ( 748.9653473494365699, -338.6346026584195101, -356.9462024416520762 ) ) ;
#18358=CARTESIAN_POINT ( 'NONE',  ( 773.7943932421234194, -191.8055962898689017, -305.5313806188329409 ) ) ;
#18360=CARTESIAN_POINT ( 'NONE',  ( 801.1904061080336987, 3.910851887033985896, -368.3070685750235498 ) ) ;
#18366=CARTESIAN_POINT ( 'NONE',  ( 765.8855110935204493, 25.83076734649409545, -319.0159684113471599 ) ) ;
#18372=CARTESIAN_POINT ( 'NONE',  ( 800.7704444035546203, -292.1692326535048210, -326.0291762391768771 ) ) ;
#18373=CARTESIAN_POINT ( 'NONE',  ( 768.8385539511368734, -311.2601417444139429, -306.4236121716840557 ) ) ;
#18378=CARTESIAN_POINT ( 'NONE',  ( 756.1348686366196716, -65.26014174441471027, -347.5531968255698416 ) ) ;
#18379=CYLINDRICAL_SURFACE ( 'NONE', #33500, 30.00000000000008171 ) ;
#18380=CARTESIAN_POINT ( 'NONE',  ( 744.7301800767019131, -148.8164208402382656, -337.4774526936615757 ) ) ;
#18382=CARTESIAN_POINT ( 'NONE',  ( 774.6858677611749044, -153.7255117493291721, -315.5713283507209894 ) ) ;
#18384=CARTESIAN_POINT ( 'NONE',  ( 772.4468031744293057, -417.8272453906067199, -363.8651313633793620 ) ) ;
#18392=CARTESIAN_POINT ( 'NONE',  ( 760.7433823573367135, -396.0090635724249637, -355.9930595647440441 ) ) ;
#18394=CARTESIAN_POINT ( 'NONE',  ( 799.9636004259356241, -166.9181544815165523, -311.2241431872006956 ) ) ;
#18398=CARTESIAN_POINT ( 'NONE',  ( 796.7845633553578182, -321.6237781080502600, -358.5707757039688204 ) ) ;
#18400=CARTESIAN_POINT ( 'NONE',  ( 788.6739635108323228, -175.6454272087892718, -373.9316612368139090 ) ) ;
#18404=CARTESIAN_POINT ( 'NONE',  ( 805.0032342141413437, -205.5436935675108145, -314.9967657858572352 ) ) ;
#18406=CARTESIAN_POINT ( 'NONE',  ( 801.9419747391806368, -18.45278447660230725, -351.9812246680014027 ) ) ;
#18407=AXIS2_PLACEMENT_3D ( 'NONE', #45508, #21237, #13625 ) ;
#18409=CARTESIAN_POINT ( 'NONE',  ( 761.9338519418445230, -86.53286901714194812, -370.4231160770881957 ) ) ;
#18411=CARTESIAN_POINT ( 'NONE',  ( 811.0346526505616112, -326.6346026584193396, -323.0537975583477532 ) ) ;
#18416=CARTESIAN_POINT ( 'NONE',  ( 786.2056067578752163, -395.8055962898682765, -374.4686193811670023 ) ) ;
#18417=CARTESIAN_POINT ( 'NONE',  ( 782.5225473063381969, -406.2709662947829088, -375.2698199232970637 ) ) ;
#18421=CARTESIAN_POINT ( 'NONE',  ( 799.4546378042377910, -177.0783235625961538, -356.1575198192848006 ) ) ;
#18423=CARTESIAN_POINT ( 'NONE',  ( 813.2346286133761168, -197.2601417444143124, -328.9521613784389160 ) ) ;
#18428=CARTESIAN_POINT ( 'NONE',  ( 800.0135310231082713, -134.0891481129655745, -325.0180583372163028 ) ) ;
#18430=CARTESIAN_POINT ( 'NONE',  ( 808.0189434323515343, -38.08914811296587999, -319.0252816721025511 ) ) ;
#18431=ADVANCED_FACE ( 'NONE', ( #9689 ), #43034, .T. ) ;
#18432=ORIENTED_EDGE ( 'NONE', *, *, #18463, .F. ) ;
#18433=CARTESIAN_POINT ( 'NONE',  ( 805.6418435158337843, -437.4636090269703459, -363.8556311672236916 ) ) ;
#18436=CARTESIAN_POINT ( 'NONE',  ( 801.5560724626406000, -336.5545181178796952, -326.7756240680316182 ) ) ;
#18439=CARTESIAN_POINT ( 'NONE',  ( 774.6312213355099630, -287.3618753856923718, -364.6798772138717482 ) ) ;
#18443=CARTESIAN_POINT ( 'NONE',  ( 783.0745993439762742, -272.1908817542434917, -365.1016975059196739 ) ) ;
#18444=CARTESIAN_POINT ( 'NONE',  ( 765.0180583372156207, -288.9982390220559978, -360.0135310231089534 ) ) ;
#18446=CARTESIAN_POINT ( 'NONE',  ( 792.1044303154645831, -132.4527844766018916, -317.8323909638837677 ) ) ;
#18452=CARTESIAN_POINT ( 'NONE',  ( 813.5763878283155464, -75.82724539060775726, -351.1614460488615350 ) ) ;
#18460=CARTESIAN_POINT ( 'NONE',  ( 790.8050863131179540, -452.8379544210779954, -362.5841948692291226 ) ) ;
#18462=CARTESIAN_POINT ( 'NONE',  ( 772.4837098697144029, -239.3618753856924570, -374.5518280994205611 ) ) ;
#18463=EDGE_CURVE ( 'NONE', #13016, #40052, #45433, .T. ) ;
#18467=CARTESIAN_POINT ( 'NONE',  ( 798.0661480581538854, -314.5328690171411949, -309.5768839229118043 ) ) ;
#18469=CARTESIAN_POINT ( 'NONE',  ( 811.0346526505616112, -326.6346026584193396, -323.0537975583477532 ) ) ;
#18474=CARTESIAN_POINT ( 'NONE',  ( 803.6646147819161570, -425.9073299311463074, -348.8264449731210561 ) ) ;
#18476=CARTESIAN_POINT ( 'NONE',  ( 801.9419747391806368, -210.4527844766016926, -351.9812246680014027 ) ) ;
#18477=CARTESIAN_POINT ( 'NONE',  ( 813.2346286133761168, -77.26014174441466764, -328.9521613784389160 ) ) ;
#18484=CARTESIAN_POINT ( 'NONE',  ( 804.9511171171677688, -221.8055962898687881, -335.8780910478229202 ) ) ;
#18486=CARTESIAN_POINT ( 'NONE',  ( 811.6461892240364477, -52.71468719896020616, -324.1737431748509835 ) ) ;
#18491=CARTESIAN_POINT ( 'NONE',  ( 752.7379699480933368, -348.0090635724251342, -361.9858362298580232 ) ) ;
#18494=CARTESIAN_POINT ( 'NONE',  ( 776.9254006560222479, -188.1908817542437760, -314.8983024940802125 ) ) ;
#18495=CARTESIAN_POINT ( 'NONE',  ( 757.8323909638827445, -170.6346026584199649, -352.1044303154654358 ) ) ;
#18496=CARTESIAN_POINT ( 'NONE',  ( 758.0580252608178853, -390.4527844766011526, -328.0187753319985404 ) ) ;
#18508=CARTESIAN_POINT ( 'NONE',  ( 768.9521613784389729, -417.8272453906067199, -373.2346286133773106 ) ) ;
#18511=CARTESIAN_POINT ( 'NONE',  ( 771.1735550268778070, -345.1800572038739006, -316.3353852180827630 ) ) ;
#18515=CARTESIAN_POINT ( 'NONE',  ( 804.4086373105744769, -241.6454272087890729, -333.3843516231986541 ) ) ;
#18524=CARTESIAN_POINT ( 'NONE',  ( 788.7366044899766848, -323.9073299311468190, -316.5762568750059813 ) ) ;
#18528=CARTESIAN_POINT ( 'NONE',  ( 746.4236121716829757, -63.82724539060779279, -328.8385539511384650 ) ) ;
#18529=CARTESIAN_POINT ( 'NONE',  ( 764.0069404352550464, -135.0783235625962959, -359.2566176426627180 ) ) ;
#18534=CARTESIAN_POINT ( 'NONE',  ( 755.5713283507202505, -5.361875385693257279, -334.6858677611754729 ) ) ;
#18535=CARTESIAN_POINT ( 'NONE',  ( 754.9735926884551418, -138.3510508353236048, -340.5236548041000333 ) ) ;
#18537=CARTESIAN_POINT ( 'NONE',  ( 802.1676090361156639, -110.6346026584201638, -327.8955696845344505 ) ) ;
#18538=CARTESIAN_POINT ( 'NONE',  ( 799.4546378042377910, -393.0783235625954717, -356.1575198192848006 ) ) ;
#18549=CARTESIAN_POINT ( 'NONE',  ( 757.0176451133909268, -85.09997266333499510, -349.9200121543848354 ) ) ;
#18551=CARTESIAN_POINT ( 'NONE',  ( 755.0636971347428243, -244.2709662947834204, -341.7834795799807353 ) ) ;
#18553=CARTESIAN_POINT ( 'NONE',  ( 804.4286716492782716, -401.3618753856920307, -345.3141322388244703 ) ) ;
#18554=CARTESIAN_POINT ( 'NONE',  ( 792.1044303154645831, -60.45278447660215448, -317.8323909638837677 ) ) ;
#18560=CARTESIAN_POINT ( 'NONE',  ( 801.9419747391806368, -18.45278447660230725, -351.9812246680014027 ) ) ;
#18562=ORIENTED_EDGE ( 'NONE', *, *, #44085, .F. ) ;
#18563=CARTESIAN_POINT ( 'NONE',  ( 805.6418435158337843, -293.4636090269707438, -363.8556311672236916 ) ) ;
#18566=CARTESIAN_POINT ( 'NONE',  ( 756.5762568750052424, -267.1800572038742985, -348.7366044899774238 ) ) ;
#18567=CARTESIAN_POINT ( 'NONE',  ( 755.3028492785439312, -135.2817908451530116, -335.9200461376539693 ) ) ;
#18572=CARTESIAN_POINT ( 'NONE',  ( 791.1614460488616487, -11.26014174441488258, -373.5763878283158874 ) ) ;
#18573=CARTESIAN_POINT ( 'NONE',  ( 767.7687537140311633, -359.9073299311467053, -372.7932403749916830 ) ) ;
#18577=CARTESIAN_POINT ( 'NONE',  ( 744.8212110874229666, -234.8965053807777963, -336.2046728542121627 ) ) ;
#18579=CARTESIAN_POINT ( 'NONE',  ( 796.7737145352015204, 3.365397341579444479, -370.7187646348536987 ) ) ;
#18584=CARTESIAN_POINT ( 'NONE',  ( 799.4546378042377910, 14.92167643740321381, -356.1575198192848006 ) ) ;
#18590=CARTESIAN_POINT ( 'NONE',  ( 758.6633372737375112, -308.5328690171412518, -326.9102291470432533 ) ) ;
#18592=CARTESIAN_POINT ( 'NONE',  ( 781.2497674668890113, -324.3510508353229511, -375.3608509340180603 ) ) ;
#18597=CARTESIAN_POINT ( 'NONE',  ( 756.1348686366196716, -89.26014174441463922, -347.5531968255698416 ) ) ;
#18599=CARTESIAN_POINT ( 'NONE',  ( 767.7687537140311633, -143.9073299311473590, -372.7932403749916830 ) ) ;
#18602=CARTESIAN_POINT ( 'NONE',  ( 774.6858677611749044, -129.7255117493292289, -315.5713283507209894 ) ) ;
#18604=CARTESIAN_POINT ( 'NONE',  ( 775.8780910478218402, -417.2817908451522158, -364.9511171171680530 ) ) ;
#18611=CARTESIAN_POINT ( 'NONE',  ( 766.0291762391763086, -394.9181544815158418, -360.7704444035551319 ) ) ;
#18613=CARTESIAN_POINT ( 'NONE',  ( 814.2805881961230625, -217.6454272087891582, -331.2368401574024119 ) ) ;
#18616=FACE_BOUND ( 'NONE', #25798, .T. ) ;
#18617=CARTESIAN_POINT ( 'NONE',  ( 754.8983024940795303, -330.8965053807774552, -336.9254006560228163 ) ) ;
#18619=CARTESIAN_POINT ( 'NONE',  ( 793.5525998758768083, -199.0999726633346825, -372.6845335610516941 ) ) ;
#18624=CARTESIAN_POINT ( 'NONE',  ( 767.7687537140311633, -239.9073299311470748, -372.7932403749916830 ) ) ;
#18626=CARTESIAN_POINT ( 'NONE',  ( 788.8264449731200330, -21.18005720387502677, -363.6646147819171233 ) ) ;
#18628=CARTESIAN_POINT ( 'NONE',  ( 771.2368401574024119, -109.4419599262327836, -374.2805881961240857 ) ) ;
#18630=CARTESIAN_POINT ( 'NONE',  ( 792.2312462859673587, -371.9073299311465917, -307.2067596250082602 ) ) ;
#18636=CARTESIAN_POINT ( 'NONE',  ( 745.1769319972822814, -401.8055962898681059, -346.2694204179732083 ) ) ;
#18637=CARTESIAN_POINT ( 'NONE',  ( 804.1009440267234822, 0.5363909730283709099, -314.0944755984392600 ) ) ;
#18640=CARTESIAN_POINT ( 'NONE',  ( 805.0264073115434940, -198.3510508353234059, -339.4763451958999099 ) ) ;
#18642=CARTESIAN_POINT ( 'NONE',  ( 814.8230680027162407, -221.8055962898687881, -333.7305795820267917 ) ) ;
#18647=CARTESIAN_POINT ( 'NONE',  ( 778.1981804954714335, -154.2709662947836478, -314.8072714833589885 ) ) ;
#18649=CARTESIAN_POINT ( 'NONE',  ( 763.2262854647970016, -56.63460265842036279, -309.2812353651462445 ) ) ;
#18652=CARTESIAN_POINT ( 'NONE',  ( 814.2805881961230625, -457.6454272087884760, -331.2368401574024119 ) ) ;
#18654=CARTESIAN_POINT ( 'NONE',  ( 769.0155153010367712, -322.3726999360615082, -362.7791456095907279 ) ) ;
#18657=CARTESIAN_POINT ( 'NONE',  ( 805.1927285166397041, -304.8164208402376403, -341.8018195045277707 ) ) ;
#18660=CARTESIAN_POINT ( 'NONE',  ( 804.1105419155481968, -291.8272453906071746, -347.6308680596136469 ) ) ;
#18661=CARTESIAN_POINT ( 'NONE',  ( 794.9819416627830151, -276.9982390220559978, -319.9864689768909898 ) ) ;
#18663=CARTESIAN_POINT ( 'NONE',  ( 767.8955696845333705, -168.4527844766018347, -362.1676090361162323 ) ) ;
#18670=CARTESIAN_POINT ( 'NONE',  ( 814.8207195650702488, -98.19088175424404596, -336.2433038121456548 ) ) ;
#18675=ORIENTED_EDGE ( 'NONE', *, *, #7399, .F. ) ;
#18676=CARTESIAN_POINT ( 'NONE',  ( 754.9967657858570647, -121.5436935675110561, -365.0032342141425943 ) ) ;
#18680=CARTESIAN_POINT ( 'NONE',  ( 804.7487373415286811, -259.5436935675106156, -364.7487373415288516 ) ) ;
#18685=CARTESIAN_POINT ( 'NONE',  ( 761.9338519418445230, -302.5328690171411949, -370.4231160770881957 ) ) ;
#18688=CARTESIAN_POINT ( 'NONE',  ( 745.7998596910086917, -341.3618753856922012, -332.5602148656461168 ) ) ;
#18692=CARTESIAN_POINT ( 'NONE',  ( 778.2165204200184689, -430.8164208402374129, -364.9363028652563230 ) ) ;
#18693=CARTESIAN_POINT ( 'NONE',  ( 749.8865473780648472, -92.53286901714190549, -322.1177392798429082 ) ) ;
#18698=CARTESIAN_POINT ( 'NONE',  ( 789.9200121543843807, -241.9874144716869182, -317.0176451133914384 ) ) ;
#18700=CARTESIAN_POINT ( 'NONE',  ( 812.6845335610512393, -79.98741447168740137, -353.5525998758768651 ) ) ;
#18701=CARTESIAN_POINT ( 'NONE',  ( 809.1994704715707485, -452.9681489794448908, -335.3884333643831042 ) ) ;
#18704=CARTESIAN_POINT ( 'NONE',  ( 807.2620300519052989, -336.0090635724251911, -318.0141637701419768 ) ) ;
#18708=CARTESIAN_POINT ( 'NONE',  ( 801.5560724626406000, -168.5545181178802352, -326.7756240680316182 ) ) ;
#18709=CARTESIAN_POINT ( 'NONE',  ( 794.9819416627830151, -180.9982390220563389, -319.9864689768909898 ) ) ;
#18711=CARTESIAN_POINT ( 'NONE',  ( 804.9363028652555840, -376.2709662947829656, -338.2165204200192079 ) ) ;
#18713=ORIENTED_EDGE ( 'NONE', *, *, #25160, .T. ) ;
#18715=CARTESIAN_POINT ( 'NONE',  ( 796.7845633553578182, 14.37622189194867417, -358.5707757039688204 ) ) ;
#18725=CARTESIAN_POINT ( 'NONE',  ( 760.0363995740630116, -418.9181544815157849, -368.7758568127991907 ) ) ;
#18726=CARTESIAN_POINT ( 'NONE',  ( 751.6929314249750860, -6.998239022056886860, -318.8095938919659034 ) ) ;
#18729=CARTESIAN_POINT ( 'NONE',  ( 797.6776695296629214, -403.5436935675101608, -357.6776695296636603 ) ) ;
#18730=CARTESIAN_POINT ( 'NONE',  ( 792.1044303154646968, 11.54721552339759860, -317.8323909638837677 ) ) ;
#18735=CARTESIAN_POINT ( 'NONE',  ( 763.0428371773158460, -251.4636090269709143, -358.7617431975195359 ) ) ;
#18743=CARTESIAN_POINT ( 'NONE',  ( 804.6798772138708955, -303.7255117493287457, -334.6312213355107019 ) ) ;
#18748=CARTESIAN_POINT ( 'NONE',  ( 778.7629533639073998, -80.73633629969864955, -375.0009284576466371 ) ) ;
#18749=CARTESIAN_POINT ( 'NONE',  ( 794.1144889064781864, -130.1692326535054463, -360.9840315886528401 ) ) ;
#18753=CARTESIAN_POINT ( 'NONE',  ( 800.0135310231082713, -38.08914811296587999, -325.0180583372163028 ) ) ;
#18754=CARTESIAN_POINT ( 'NONE',  ( 786.6156483768007774, -145.4419599262326699, -315.5913626894246136 ) ) ;
#18755=CARTESIAN_POINT ( 'NONE',  ( 771.2633955100217236, -119.9073299311474443, -363.4237431249939618 ) ) ;
#18757=CARTESIAN_POINT ( 'NONE',  ( 803.2186876482843445, -439.9874144716862929, -350.0220218866286928 ) ) ;
#18765=ADVANCED_FACE ( 'NONE', ( #21846 ), #1286, .F. ) ;
#18771=CARTESIAN_POINT ( 'NONE',  ( 776.9254006560222479, -92.19088175424406018, -314.8983024940802125 ) ) ;
#18773=CARTESIAN_POINT ( 'NONE',  ( 765.0180583372156207, -264.9982390220561115, -360.0135310231089534 ) ) ;
#18775=CARTESIAN_POINT ( 'NONE',  ( 801.9419747391806368, -378.4527844766011526, -351.9812246680014027 ) ) ;
#18776=CARTESIAN_POINT ( 'NONE',  ( 804.9363028652555840, -64.27096629478397460, -338.2165204200192079 ) ) ;
#18780=CARTESIAN_POINT ( 'NONE',  ( 809.0717654672305343, -4.918154481517067467, -360.1688906516309885 ) ) ;
#18783=CARTESIAN_POINT ( 'NONE',  ( 797.8822607201568644, -318.5545181178796952, -370.1134526219340160 ) ) ;
#18785=EDGE_CURVE ( 'NONE', #37618, #15749, #15148, .T. ) ;
#18787=FACE_OUTER_BOUND ( 'NONE', #6760, .T. ) ;
#18788=CARTESIAN_POINT ( 'NONE',  ( 794.9819416627830151, -252.9982390220560831, -319.9864689768909898 ) ) ;
#18791=CARTESIAN_POINT ( 'NONE',  ( 757.0176451133909268, -157.0999726633347962, -349.9200121543848354 ) ) ;
#18794=CARTESIAN_POINT ( 'NONE',  ( 745.4481719005789273, -339.7255117493285184, -347.5162901302853697 ) ) ;
#18800=CARTESIAN_POINT ( 'NONE',  ( 773.7943932421234194, -239.8055962898687028, -305.5313806188329409 ) ) ;
#18802=CARTESIAN_POINT ( 'NONE',  ( 814.5518280994195948, 8.274488250670337663, -332.4837098697145734 ) ) ;
#18805=ORIENTED_EDGE ( 'NONE', *, *, #1836, .T. ) ;
#18809=CARTESIAN_POINT ( 'NONE',  ( 769.1273215169530886, 1.285312801039623753, -317.4527132478988847 ) ) ;
#18817=CARTESIAN_POINT ( 'NONE',  ( 796.7845633553578182, -321.6237781080502600, -358.5707757039688204 ) ) ;
#18820=CARTESIAN_POINT ( 'NONE',  ( 745.1769319972822814, -329.8055962898683902, -346.2694204179732083 ) ) ;
#18826=CARTESIAN_POINT ( 'NONE',  ( 799.4546378042377910, -81.07832356259649487, -356.1575198192848006 ) ) ;
#18827=ORIENTED_EDGE ( 'NONE', *, *, #36789, .F. ) ;
#18829=CARTESIAN_POINT ( 'NONE',  ( 755.2512626584698410, -175.5436935675108998, -315.2512626584710915 ) ) ;
#18831=CARTESIAN_POINT ( 'NONE',  ( 762.3223304703356007, -175.5436935675108998, -322.3223304703362828 ) ) ;
#18833=CARTESIAN_POINT ( 'NONE',  ( 796.9571628226829034, -431.4636090269702322, -321.2382568024804641 ) ) ;
#18843=CARTESIAN_POINT ( 'NONE',  ( 766.9102291470427417, -426.5545181178794678, -318.6633372737382501 ) ) ;
#18845=CARTESIAN_POINT ( 'NONE',  ( 750.9282345327678740, -208.9181544815164102, -319.8311093483690115 ) ) ;
#18849=CARTESIAN_POINT ( 'NONE',  ( 801.3366627262608972, -320.5328690171411949, -353.0897708529566899 ) ) ;
#18851=CARTESIAN_POINT ( 'NONE',  ( 797.8822607201568644, -198.5545181178800647, -370.1134526219340160 ) ) ;
#18853=DIRECTION ( 'NONE',  ( 0.000000000000000000, 0.000000000000000000, -1.000000000000000000 ) ) ;
#18856=CARTESIAN_POINT ( 'NONE',  ( 751.9810565676468741, -242.0891481129652618, -360.9747183278973921 ) ) ;
#18858=CARTESIAN_POINT ( 'NONE',  ( 774.6858677611749044, -9.725511749329603717, -315.5713283507209894 ) ) ;
#18861=CARTESIAN_POINT ( 'NONE',  ( 795.6651683502461765, -130.7146871989599504, -371.3240766477733814 ) ) ;
#18863=CARTESIAN_POINT ( 'NONE',  ( 754.9967657858570647, -361.5436935675103882, -365.0032342141425374 ) ) ;
#18868=CARTESIAN_POINT ( 'NONE',  ( 800.2193346964447755, -402.9982390220555430, -355.1360043628815788 ) ) ;
#18870=CARTESIAN_POINT ( 'NONE',  ( 781.2370466360911223, 3.263663700301089765, -304.9990715423533629 ) ) ;
#18874=AXIS2_PLACEMENT_3D ( 'NONE', #41433, #34254, #9785 ) ;
#18875=CARTESIAN_POINT ( 'NONE',  ( 789.9200121543843807, -193.9874144716870319, -317.0176451133914384 ) ) ;
#18877=CARTESIAN_POINT ( 'NONE',  ( 747.3154664389472828, -235.9874144716868898, -326.4474001241230781 ) ) ;
#18883=CARTESIAN_POINT ( 'NONE',  ( 777.5031285880264704, -94.81642084023843609, -374.9108240113588408 ) ) ;
#18886=CARTESIAN_POINT ( 'NONE',  ( 796.1575198192839480, -6.009063572426154742, -359.4546378042384163 ) ) ;
#18889=CARTESIAN_POINT ( 'NONE',  ( 779.4763451958990572, -320.7363362996979390, -365.0264073115438919 ) ) ;
#18892=CARTESIAN_POINT ( 'NONE',  ( 774.6312213355099630, -335.3618753856920307, -364.6798772138717482 ) ) ;
#18896=CARTESIAN_POINT ( 'NONE',  ( 755.3028492785439312, -303.2817908451525000, -335.9200461376539693 ) ) ;
#18897=CARTESIAN_POINT ( 'NONE',  ( 801.9419747391806368, -282.4527844766014937, -351.9812246680014027 ) ) ;
#18899=CARTESIAN_POINT ( 'NONE',  ( 759.7806653035534055, -150.9982390220563957, -324.8639956371180801 ) ) ;
#18906=CARTESIAN_POINT ( 'NONE',  ( 786.2694204179717872, -69.28179084515321051, -305.1769319972829067 ) ) ;
#18913=CARTESIAN_POINT ( 'NONE',  ( 748.9653473494365699, -146.6346026584200786, -356.9462024416520762 ) ) ;
#18917=CARTESIAN_POINT ( 'NONE',  ( 755.2512626584698410, -271.5436935675106156, -315.2512626584710915 ) ) ;
#18921=CARTESIAN_POINT ( 'NONE',  ( 813.9316612368132837, -319.4419599262320730, -348.6739635108323228 ) ) ;
#18924=CARTESIAN_POINT ( 'NONE',  ( 754.9967657858570647, -361.5436935675103882, -365.0032342141425374 ) ) ;
#18928=CARTESIAN_POINT ( 'NONE',  ( 801.9419747391806368, -426.4527844766010389, -351.9812246680014027 ) ) ;
#18930=CARTESIAN_POINT ( 'NONE',  ( 778.2165204200184689, -214.8164208402380666, -364.9363028652563230 ) ) ;
#18931=CARTESIAN_POINT ( 'NONE',  ( 800.1688906516307043, -130.1692326535054463, -369.0717654672308186 ) ) ;
#18935=CARTESIAN_POINT ( 'NONE',  ( 756.7813123517142913, -235.9874144716868898, -329.9779781133712504 ) ) ;
#18938=CARTESIAN_POINT ( 'NONE',  ( 751.2241431872005251, -64.16923265350563099, -359.9636004259367610 ) ) ;
#18939=CARTESIAN_POINT ( 'NONE',  ( 808.0106897970731552, -452.9681489794447771, -338.3625385368115985 ) ) ;
#18942=CARTESIAN_POINT ( 'NONE',  ( 749.5768839229115201, -348.5545181178796383, -358.0661480581553064 ) ) ;
#18945=CARTESIAN_POINT ( 'NONE',  ( 793.0897708529556667, -198.5545181178800647, -361.3366627262616362 ) ) ;
#18946=CARTESIAN_POINT ( 'NONE',  ( 771.1735550268778070, -177.1800572038744690, -316.3353852180827630 ) ) ;
#18947=CARTESIAN_POINT ( 'NONE',  ( 785.3687786644885591, -395.3618753856919739, -315.3201227861280813 ) ) ;
#18958=CARTESIAN_POINT ( 'NONE',  ( 776.2046728542105711, -404.1908817542431507, -304.8212110874238761 ) ) ;
#18960=CARTESIAN_POINT ( 'NONE',  ( 745.4481719005789273, -51.72551174932947049, -347.5162901302853697 ) ) ;
#18962=AXIS2_PLACEMENT_3D ( 'NONE', #24487, #29116, #6950 ) ;
#18963=CARTESIAN_POINT ( 'NONE',  ( 804.9363028652555840, -400.2709662947828519, -338.2165204200192079 ) ) ;
#18964=CARTESIAN_POINT ( 'NONE',  ( 767.8955696845334842, -0.4527844766023629286, -362.1676090361161755 ) ) ;
#18967=CARTESIAN_POINT ( 'NONE',  ( 755.3028492785439312, -255.2817908451526705, -335.9200461376539693 ) ) ;
#18968=CARTESIAN_POINT ( 'NONE',  ( 787.5162901302840055, -155.3618753856927128, -305.4481719005792684 ) ) ;
#18974=EDGE_CURVE ( 'NONE', #22826, #31261, #31351, .T. ) ;
#18979=CARTESIAN_POINT ( 'NONE',  ( 755.0636971347428243, -316.2709662947832499, -341.7834795799807353 ) ) ;
#18981=CARTESIAN_POINT ( 'NONE',  ( 814.8207195650702488, -98.19088175424404596, -336.2433038121456548 ) ) ;
#18982=CARTESIAN_POINT ( 'NONE',  ( 790.8726784830453198, -106.7146871989600498, -362.5472867521010585 ) ) ;
#18986=CARTESIAN_POINT ( 'NONE',  ( 792.1044303154645831, -36.45278447660223975, -317.8323909638837677 ) ) ;
#18987=CARTESIAN_POINT ( 'NONE',  ( 790.8726784830453198, -130.7146871989599504, -362.5472867521010585 ) ) ;
#18989=CARTESIAN_POINT ( 'NONE',  ( 803.8651313633788504, -437.2601417444135450, -332.4468031744301015 ) ) ;
#19001=CARTESIAN_POINT ( 'NONE',  ( 755.5913626894240451, -85.64542720878952764, -346.6156483768012890 ) ) ;
#19002=CARTESIAN_POINT ( 'NONE',  ( 802.1676090361155502, -278.6346026584196807, -327.8955696845344505 ) ) ;
#19004=CARTESIAN_POINT ( 'NONE',  ( 778.2165204200184689, -382.8164208402374697, -364.9363028652563230 ) ) ;
#19005=CARTESIAN_POINT ( 'NONE',  ( 785.3687786644884454, -35.36187538569316047, -315.3201227861279676 ) ) ;
#19009=CARTESIAN_POINT ( 'NONE',  ( 793.5525998758768083, -31.09997266333516919, -372.6845335610516941 ) ) ;
#19010=DIRECTION ( 'NONE',  ( 0.000000000000000000, 0.000000000000000000, 1.000000000000000000 ) ) ;
#19012=CARTESIAN_POINT ( 'NONE',  ( 752.7379699480933368, -324.0090635724251911, -361.9858362298580232 ) ) ;
#19015=CARTESIAN_POINT ( 'NONE',  ( 800.0135310231082713, -278.0891481129651197, -325.0180583372163028 ) ) ;
#19017=CARTESIAN_POINT ( 'NONE',  ( 775.8780910478218402, -153.2817908451529831, -364.9511171171680530 ) ) ;
#19021=CARTESIAN_POINT ( 'NONE',  ( 795.6651683502461765, -10.71468719896033761, -371.3240766477733814 ) ) ;
#19022=CARTESIAN_POINT ( 'NONE',  ( 813.1304606946831655, -329.9073299311467622, -352.3570229623691716 ) ) ;
#19026=CARTESIAN_POINT ( 'NONE',  ( 771.2368401574024119, -253.4419599262323572, -374.2805881961240857 ) ) ;
#19028=CARTESIAN_POINT ( 'NONE',  ( 808.7758568127978833, -436.1692326535044231, -320.0363995740631822 ) ) ;
#19030=DIRECTION ( 'NONE',  ( 0.000000000000000000, 0.000000000000000000, -1.000000000000000000 ) ) ;
#19034=CARTESIAN_POINT ( 'NONE',  ( 783.0433043558608688, -0.8965053807785533513, -315.1538015810313027 ) ) ;
#19039=CARTESIAN_POINT ( 'NONE',  ( 805.1016975059191054, -318.8965053807775121, -343.0745993439771837 ) ) ;
#19041=CARTESIAN_POINT ( 'NONE',  ( 815.0009284576459549, -342.3510508353228943, -338.7629533639073429 ) ) ;
#19049=CARTESIAN_POINT ( 'NONE',  ( 745.4481719005789273, -171.7255117493291152, -347.5162901302853129 ) ) ;
#19051=EDGE_LOOP ( 'NONE', ( #19991, #36260, #8028, #41362 ) ) ;
#19052=CARTESIAN_POINT ( 'NONE',  ( 768.0187753319979720, -176.6346026584199933, -318.0580252608186242 ) ) ;
#19055=CARTESIAN_POINT ( 'NONE',  ( 786.5483106153019435, -415.6454272087885897, -364.1601925771022366 ) ) ;
#19063=CARTESIAN_POINT ( 'NONE',  ( 793.9708237608222134, -430.9181544815157849, -319.2295555964448681 ) ) ;
#19065=CARTESIAN_POINT ( 'NONE',  ( 804.1009440267234822, -191.4636090269709996, -314.0944755984392600 ) ) ;
#19067=LINE ( 'NONE', #26439, #18258 ) ;
#19068=CARTESIAN_POINT ( 'NONE',  ( 792.1044303154645831, -204.4527844766016926, -317.8323909638837677 ) ) ;
#19070=CARTESIAN_POINT ( 'NONE',  ( 783.0433043558608688, -336.8965053807774552, -315.1538015810313027 ) ) ;
#19072=CARTESIAN_POINT ( 'NONE',  ( 745.1792804349281596, -206.1908817542437191, -343.7566961878542884 ) ) ;
#19075=CARTESIAN_POINT ( 'NONE',  ( 802.5472867521000353, -52.37269993606237506, -350.8726784830461156 ) ) ;
#19078=CARTESIAN_POINT ( 'NONE',  ( 754.9967657858570647, -241.5436935675106440, -365.0032342141425943 ) ) ;
#19080=CARTESIAN_POINT ( 'NONE',  ( 771.2633955100217236, -23.90732993114773919, -363.4237431249939618 ) ) ;
#19082=CARTESIAN_POINT ( 'NONE',  ( 764.3348316497523456, -142.7146871989599219, -308.6759233522265617 ) ) ;
#19084=CARTESIAN_POINT ( 'NONE',  ( 796.7737145352015204, -380.6346026584192828, -370.7187646348536987 ) ) ;
#19091=CARTESIAN_POINT ( 'NONE',  ( 804.9363028652555840, -400.2709662947828519, -338.2165204200192079 ) ) ;
#19093=CARTESIAN_POINT ( 'NONE',  ( 796.7737145352015204, -452.6346026584191691, -370.7187646348536987 ) ) ;
#19097=CARTESIAN_POINT ( 'NONE',  ( 760.5453621957607311, -237.0783235625960117, -323.8424801807151425 ) ) ;
#19099=CARTESIAN_POINT ( 'NONE',  ( 747.3154664389472828, -211.9874144716869750, -326.4474001241230781 ) ) ;
#19105=CARTESIAN_POINT ( 'NONE',  ( 756.5762568750052424, -147.1800572038746395, -348.7366044899774238 ) ) ;
#19107=CARTESIAN_POINT ( 'NONE',  ( 751.6929314249748586, -78.99823902205662307, -318.8095938919659034 ) ) ;
#19108=CARTESIAN_POINT ( 'NONE',  ( 797.8594530101009923, -85.54369356751118403, -322.1405469898982119 ) ) ;
#19110=CARTESIAN_POINT ( 'NONE',  ( 772.4468031744293057, -9.827245390607961539, -363.8651313633793620 ) ) ;
#19112=CARTESIAN_POINT ( 'NONE',  ( 804.1105419155481968, -315.8272453906070609, -347.6308680596136469 ) ) ;
#19119=CARTESIAN_POINT ( 'NONE',  ( 757.0176451133909268, -325.0999726633342561, -349.9200121543848354 ) ) ;
#19120=CARTESIAN_POINT ( 'NONE',  ( 803.6646147819161570, -281.9073299311468759, -348.8264449731210561 ) ) ;
#19121=CARTESIAN_POINT ( 'NONE',  ( 804.6798772138708955, -159.7255117493291436, -334.6312213355107019 ) ) ;
#19127=CARTESIAN_POINT ( 'NONE',  ( 778.7629533639073998, -128.7363362996984790, -375.0009284576466371 ) ) ;
#19132=CARTESIAN_POINT ( 'NONE',  ( 814.2001403089898304, -137.3618753856928265, -347.4397851343538264 ) ) ;
#19135=CARTESIAN_POINT ( 'NONE',  ( 805.0032342141412300, -277.5436935675105019, -314.9967657858571783 ) ) ;
#19136=CARTESIAN_POINT ( 'NONE',  ( 744.7301800767020268, -436.8164208402372992, -337.4774526936615189 ) ) ;
#19139=CARTESIAN_POINT ( 'NONE',  ( 752.4576283171824116, -333.0783235625956991, -317.7880784355627952 ) ) ;
#19140=CARTESIAN_POINT ( 'NONE',  ( 811.0346526505616112, -86.63460265842023489, -323.0537975583477532 ) ) ;
#19142=CARTESIAN_POINT ( 'NONE',  ( 747.2067596250078623, -363.1800572038739006, -352.2312462859687230 ) ) ;
#19147=CARTESIAN_POINT ( 'NONE',  ( 788.7631598425961101, -121.4419599262327267, -305.7194118038759143 ) ) ;
#19152=CARTESIAN_POINT ( 'NONE',  ( 769.1273215169530886, -238.7146871989596661, -317.4527132478988847 ) ) ;
#19154=CARTESIAN_POINT ( 'NONE',  ( 796.9462024416508257, 11.54721552339760038, -308.9653473494370246 ) ) ;
#19155=CARTESIAN_POINT ( 'NONE',  ( 798.0661480581538854, -74.53286901714196233, -309.5768839229118043 ) ) ;
#19159=CARTESIAN_POINT ( 'NONE',  ( 748.6759233522253680, -376.3726999360614514, -324.3348316497537098 ) ) ;
#19160=CARTESIAN_POINT ( 'NONE',  ( 778.1981804954714335, -226.2709662947834204, -314.8072714833589885 ) ) ;
#19163=CARTESIAN_POINT ( 'NONE',  ( 796.1575198192839480, -222.0090635724254184, -359.4546378042384163 ) ) ;
#19164=CARTESIAN_POINT ( 'NONE',  ( 792.1044303154645831, -180.4527844766017211, -317.8323909638837677 ) ) ;
#19165=CARTESIAN_POINT ( 'NONE',  ( 804.4286716492782716, -401.3618753856920307, -345.3141322388244703 ) ) ;
#19168=CARTESIAN_POINT ( 'NONE',  ( 804.9363028652555840, -112.2709662947838325, -338.2165204200192079 ) ) ;
#19177=CARTESIAN_POINT ( 'NONE',  ( 744.6391490659812007, -398.7363362996976548, -338.7502325331110455 ) ) ;
#19178=CARTESIAN_POINT ( 'NONE',  ( 810.7187646348534145, -42.45278447660223264, -356.7737145352016341 ) ) ;
#19180=CARTESIAN_POINT ( 'NONE',  ( 754.8072714833581358, -412.8164208402372992, -338.1981804954720587 ) ) ;
#19181=CARTESIAN_POINT ( 'NONE',  ( 801.9419747391806368, -18.45278447660230725, -351.9812246680014027 ) ) ;
#19183=CARTESIAN_POINT ( 'NONE',  ( 804.8461984189677878, -266.1908817542435486, -336.9566956441385628 ) ) ;
#19184=CARTESIAN_POINT ( 'NONE',  ( 801.1904061080336987, -164.0891481129655176, -368.3070685750235498 ) ) ;
#19191=CARTESIAN_POINT ( 'NONE',  ( 768.0187753319979720, -320.6346026584195670, -318.0580252608186242 ) ) ;
#19193=CARTESIAN_POINT ( 'NONE',  ( 754.3581564841646241, -89.46360902697134065, -316.1443688327762516 ) ) ;
#19194=CARTESIAN_POINT ( 'NONE',  ( 776.9566956441375396, -108.8965053807782084, -364.8461984189686405 ) ) ;
#19197=CARTESIAN_POINT ( 'NONE',  ( 781.7834795799800531, -34.81642084023861372, -315.0636971347436202 ) ) ;
#19198=CARTESIAN_POINT ( 'NONE',  ( 769.1273215169530886, -142.7146871989599219, -317.4527132478988847 ) ) ;
#19199=CARTESIAN_POINT ( 'NONE',  ( 762.1405469898971887, -121.5436935675110419, -357.8594530101015607 ) ) ;
#19201=CARTESIAN_POINT ( 'NONE',  ( 802.7791456095903868, -436.7146871989589272, -329.0155153010375102 ) ) ;
#19207=CARTESIAN_POINT ( 'NONE',  ( 744.6391490659812007, -278.7363362996980527, -338.7502325331110455 ) ) ;
#19214=CARTESIAN_POINT ( 'NONE',  ( 769.9779781133707957, -67.09997266333506616, -316.7813123517150871 ) ) ;
#19215=CARTESIAN_POINT ( 'NONE',  ( 801.9419747391806368, -282.4527844766014937, -351.9812246680014027 ) ) ;
#19217=CARTESIAN_POINT ( 'NONE',  ( 767.8955696845333705, -408.4527844766009252, -362.1676090361162323 ) ) ;
#19218=CARTESIAN_POINT ( 'NONE',  ( 757.8323909638827445, -98.63460265842024910, -352.1044303154654358 ) ) ;
#19220=CYLINDRICAL_SURFACE ( 'NONE', #41799, 10.00000000000000888 ) ;
#19222=CARTESIAN_POINT ( 'NONE',  ( 745.5313806188320314, -15.28179084515340058, -333.7943932421247268 ) ) ;
#19225=CARTESIAN_POINT ( 'NONE',  ( 760.0363995740630116, -322.9181544815161260, -368.7758568127991907 ) ) ;
#19228=CARTESIAN_POINT ( 'NONE',  ( 794.9819416627830151, -300.9982390220559409, -319.9864689768909898 ) ) ;
#19230=CARTESIAN_POINT ( 'NONE',  ( 799.2566176426618085, -168.0090635724256458, -324.0069404352559559 ) ) ;
#19233=CARTESIAN_POINT ( 'NONE',  ( 772.4837098697145166, -359.3618753856921444, -374.5518280994205611 ) ) ;
#19238=CARTESIAN_POINT ( 'NONE',  ( 813.2346286133761168, -437.2601417444135450, -328.9521613784389160 ) ) ;
#19243=CARTESIAN_POINT ( 'NONE',  ( 754.8983024940795303, -18.89650538077849617, -336.9254006560228163 ) ) ;
#19249=CARTESIAN_POINT ( 'NONE',  ( 799.4546378042377910, -345.0783235625956991, -356.1575198192848006 ) ) ;
#19251=CARTESIAN_POINT ( 'NONE',  ( 808.7758568127978833, -316.1692326535048210, -320.0363995740631822 ) ) ;
#19258=CARTESIAN_POINT ( 'NONE',  ( 751.9810565676468741, -194.0891481129654039, -360.9747183278973921 ) ) ;
#19261=CARTESIAN_POINT ( 'NONE',  ( 797.6776695296629214, -187.5436935675108430, -357.6776695296636603 ) ) ;
#19263=CARTESIAN_POINT ( 'NONE',  ( 775.8780910478218402, -441.2817908451521021, -364.9511171171680530 ) ) ;
#19270=CARTESIAN_POINT ( 'NONE',  ( 804.1105419155481968, -411.8272453906067199, -347.6308680596136469 ) ) ;
#19272=CARTESIAN_POINT ( 'NONE',  ( 795.8262568251477660, -190.3726999360619629, -308.3538107759623585 ) ) ;
#19276=CARTESIAN_POINT ( 'NONE',  ( 762.3223304703356007, -175.5436935675108998, -322.3223304703362828 ) ) ;
#19277=CARTESIAN_POINT ( 'NONE',  ( 766.7756240680305382, -350.5328690171411381, -361.5560724626415663 ) ) ;
#19279=CARTESIAN_POINT ( 'NONE',  ( 747.6481478633932056, -229.0999726633345404, -353.4146539503763620 ) ) ;
#19281=CARTESIAN_POINT ( 'NONE',  ( 779.9999999999992042, 16.45630643248849267, -339.9999999999999432 ) ) ;
#19282=CARTESIAN_POINT ( 'NONE',  ( 755.5913626894240451, -37.64542720878968396, -346.6156483768012890 ) ) ;
#19285=CARTESIAN_POINT ( 'NONE',  ( 782.4968714119720516, -226.8164208402380098, -305.0891759886411023 ) ) ;
#19289=CARTESIAN_POINT ( 'NONE',  ( 800.2193346964447755, -42.99823902205675807, -355.1360043628815788 ) ) ;
#19292=CARTESIAN_POINT ( 'NONE',  ( 813.2346286133761168, -149.2601417444144261, -328.9521613784389160 ) ) ;
#19294=CARTESIAN_POINT ( 'NONE',  ( 796.9462024416508257, -372.4527844766010958, -308.9653473494370246 ) ) ;
#19296=EDGE_CURVE ( 'NONE', #21713, #30422, #13498, .T. ) ;
#19299=CARTESIAN_POINT ( 'NONE',  ( 755.0636971347428243, -388.2709662947829656, -341.7834795799807353 ) ) ;
#19301=CARTESIAN_POINT ( 'NONE',  ( 811.0346526505616112, -446.6346026584189985, -323.0537975583477532 ) ) ;
#19306=CARTESIAN_POINT ( 'NONE',  ( 789.9200121543843807, -217.9874144716870035, -317.0176451133914384 ) ) ;
#19309=CARTESIAN_POINT ( 'NONE',  ( 776.2433038121456548, -228.8965053807778816, -374.8207195650711014 ) ) ;
#19315=CARTESIAN_POINT ( 'NONE',  ( 805.0264073115434940, -30.35105083532391390, -339.4763451958999099 ) ) ;
#19318=CARTESIAN_POINT ( 'NONE',  ( 812.7932403749906598, -87.18005720387481006, -327.7687537140311633 ) ) ;
#19319=CARTESIAN_POINT ( 'NONE',  ( 771.2633955100217236, -71.90732993114760063, -363.4237431249939618 ) ) ;
#19321=CARTESIAN_POINT ( 'NONE',  ( 763.8424801807145741, 5.990936427573807954, -320.5453621957614700 ) ) ;
#19322=CARTESIAN_POINT ( 'NONE',  ( 780.5236548040995785, -332.7363362996979390, -314.9735926884559944 ) ) ;
#19331=CARTESIAN_POINT ( 'NONE',  ( 804.8461984189677878, -338.1908817542433212, -336.9566956441385628 ) ) ;
#19332=CARTESIAN_POINT ( 'NONE',  ( 795.1360043628807261, -332.0891481129649492, -360.2193346964456282 ) ) ;
#19333=CARTESIAN_POINT ( 'NONE',  ( 765.0180583372156207, -144.9982390220564525, -360.0135310231089534 ) ) ;
#19337=CARTESIAN_POINT ( 'NONE',  ( 793.5525998758768083, -127.0999726633348672, -372.6845335610516941 ) ) ;
#19343=CARTESIAN_POINT ( 'NONE',  ( 767.7687537140311633, -143.9073299311473590, -372.7932403749916830 ) ) ;
#19348=CARTESIAN_POINT ( 'NONE',  ( 767.6429770376289525, -273.1800572038742985, -306.8695393053162093 ) ) ;
#19349=CARTESIAN_POINT ( 'NONE',  ( 796.9462024416508257, -444.4527844766009821, -308.9653473494370246 ) ) ;
#19352=CARTESIAN_POINT ( 'NONE',  ( 744.8212110874229666, -330.8965053807774552, -336.2046728542121627 ) ) ;
#19353=CARTESIAN_POINT ( 'NONE',  ( 763.0537975583475827, -72.45278447660213317, -371.0346526505627480 ) ) ;
#19355=CARTESIAN_POINT ( 'NONE',  ( 744.7301800767019131, -340.8164208402376971, -337.4774526936615757 ) ) ;
#19360=CARTESIAN_POINT ( 'NONE',  ( 762.3223304703356007, -223.5436935675107577, -322.3223304703362828 ) ) ;
#19362=CARTESIAN_POINT ( 'NONE',  ( 795.6651683502461765, -130.7146871989599504, -371.3240766477733814 ) ) ;
#19368=CARTESIAN_POINT ( 'NONE',  ( 787.6308680596127942, -227.2601417444141987, -364.1105419155492768 ) ) ;
#19371=CARTESIAN_POINT ( 'NONE',  ( 805.0032342141412300, 10.45630643248850866, -314.9967657858571783 ) ) ;
#19372=CARTESIAN_POINT ( 'NONE',  ( 813.2346286133761168, -77.26014174441466764, -328.9521613784389160 ) ) ;
#19376=CARTESIAN_POINT ( 'NONE',  ( 746.4236121716829757, -375.8272453906069472, -328.8385539511384650 ) ) ;
#19379=CARTESIAN_POINT ( 'NONE',  ( 755.5913626894240451, -205.6454272087891297, -346.6156483768012890 ) ) ;
#19380=CARTESIAN_POINT ( 'NONE',  ( 781.7834795799800531, -202.8164208402380950, -315.0636971347436202 ) ) ;
#19381=CARTESIAN_POINT ( 'NONE',  ( 764.8639956371174549, -392.0891481129647786, -319.7806653035542581 ) ) ;
#19384=CARTESIAN_POINT ( 'NONE',  ( 785.3141322388236176, -93.72551174932934259, -364.4286716492789537 ) ) ;
#19393=CARTESIAN_POINT ( 'NONE',  ( 799.9636004259356241, -454.9181544815156713, -311.2241431872006956 ) ) ;
#19395=CARTESIAN_POINT ( 'NONE',  ( 745.7998596910086917, -29.36187538569318178, -332.5602148656461168 ) ) ;
#19398=CARTESIAN_POINT ( 'NONE',  ( 756.3353852180819104, -389.9073299311465348, -331.1735550268788302 ) ) ;
#19399=CARTESIAN_POINT ( 'NONE',  ( 781.8018195045267476, -22.27096629478410605, -365.1927285166407273 ) ) ;
#19402=CARTESIAN_POINT ( 'NONE',  ( 763.8424801807145741, -282.0090635724253048, -320.5453621957614700 ) ) ;
#19403=CARTESIAN_POINT ( 'NONE',  ( 813.1304606946830518, -161.9073299311472454, -352.3570229623690580 ) ) ;
#19410=CARTESIAN_POINT ( 'NONE',  ( 767.8955696845333705, -360.4527844766010958, -362.1676090361162323 ) ) ;
#19412=CARTESIAN_POINT ( 'NONE',  ( 812.3518521366052028, -97.09997266333496668, -326.5853460496235243 ) ) ;
#19413=CARTESIAN_POINT ( 'NONE',  ( 754.8983024940795303, -114.8965053807782226, -336.9254006560228163 ) ) ;
#19416=CARTESIAN_POINT ( 'NONE',  ( 762.3223304703356007, -31.54369356751135456, -322.3223304703362828 ) ) ;
#19417=CARTESIAN_POINT ( 'NONE',  ( 779.4709603349208464, -120.3510508353236048, -314.7162404726379918 ) ) ;
#19418=CARTESIAN_POINT ( 'NONE',  ( 778.1981804954714335, -130.2709662947837899, -314.8072714833589885 ) ) ;
#19420=CARTESIAN_POINT ( 'NONE',  ( 755.8398074228967971, -427.4419599262317888, -333.4516893846970333 ) ) ;
#19427=CARTESIAN_POINT ( 'NONE',  ( 748.6759233522253680, -256.3726999360617924, -324.3348316497537098 ) ) ;
#19428=ORIENTED_EDGE ( 'NONE', *, *, #19574, .T. ) ;
#19433=CARTESIAN_POINT ( 'NONE',  ( 757.0176451133909268, -109.0999726633349241, -349.9200121543848354 ) ) ;
#19434=CARTESIAN_POINT ( 'NONE',  ( 797.6776695296629214, -283.5436935675105019, -357.6776695296636603 ) ) ;
#19436=CARTESIAN_POINT ( 'NONE',  ( 755.3201227861273992, -435.7255117493282341, -345.3687786644892981 ) ) ;
#19437=CARTESIAN_POINT ( 'NONE',  ( 774.6312213355099630, -95.36187538569294020, -364.6798772138717482 ) ) ;
#19443=CARTESIAN_POINT ( 'NONE',  ( 745.1792804349281596, -326.1908817542433781, -343.7566961878542884 ) ) ;
#19446=CARTESIAN_POINT ( 'NONE',  ( 797.8594530101008786, -301.5436935675105588, -322.1405469898980982 ) ) ;
#19448=CARTESIAN_POINT ( 'NONE',  ( 793.0897708529556667, -150.5545181178802352, -361.3366627262616362 ) ) ;
#19452=CARTESIAN_POINT ( 'NONE',  ( 800.9747183278959710, -396.9982390220556567, -311.9810565676471583 ) ) ;
#19453=AXIS2_PLACEMENT_3D ( 'NONE', #30362, #1958, #16058 ) ;
#19458=CARTESIAN_POINT ( 'NONE',  ( 745.0891759886404770, -28.27096629478409540, -342.4968714119734159 ) ) ;
#19463=CARTESIAN_POINT ( 'NONE',  ( 787.6308680596127942, -11.26014174441488258, -364.1105419155492768 ) ) ;
#19464=LINE ( 'NONE', #12543, #31383 ) ;
#19469=CARTESIAN_POINT ( 'NONE',  ( 802.7791456095903868, -340.7146871989592114, -329.0155153010375102 ) ) ;
#19473=CARTESIAN_POINT ( 'NONE',  ( 814.8230680027162407, -341.8055962898683333, -333.7305795820267917 ) ) ;
#19478=CARTESIAN_POINT ( 'NONE',  ( 782.5225473063381969, -190.2709662947835909, -375.2698199232970637 ) ) ;
#19482=CARTESIAN_POINT ( 'NONE',  ( 762.1405469898973024, -193.5436935675108714, -357.8594530101016176 ) ) ;
#19485=CARTESIAN_POINT ( 'NONE',  ( 766.9102291470427417, -450.5545181178793541, -318.6633372737382501 ) ) ;
#19491=CARTESIAN_POINT ( 'NONE',  ( 783.0745993439762742, -416.1908817542430938, -365.1016975059196739 ) ) ;
#19494=CARTESIAN_POINT ( 'NONE',  ( 771.3260364891663130, -211.6454272087891582, -306.0683387631859773 ) ) ;
#19498=CARTESIAN_POINT ( 'NONE',  ( 758.0580252608178853, -198.4527844766017495, -328.0187753319985404 ) ) ;
#19499=CARTESIAN_POINT ( 'NONE',  ( 789.9200121543843807, -361.9874144716864635, -317.0176451133914384 ) ) ;
#19501=CARTESIAN_POINT ( 'NONE',  ( 793.5525998758768083, -223.0999726633346256, -372.6845335610516941 ) ) ;
#19504=CARTESIAN_POINT ( 'NONE',  ( 754.7162404726377645, -62.73633629969871350, -339.4709603349214717 ) ) ;
#19507=CARTESIAN_POINT ( 'NONE',  ( 747.2067596250078623, -243.1800572038743269, -352.2312462859687230 ) ) ;
#19510=CARTESIAN_POINT ( 'NONE',  ( 768.0187753319979720, -32.63460265842044095, -318.0580252608186242 ) ) ;
#19512=CARTESIAN_POINT ( 'NONE',  ( 803.8556311672234642, -129.6237781080508853, -365.6418435158340117 ) ) ;
#19514=CARTESIAN_POINT ( 'NONE',  ( 759.0252816721024374, -384.9982390220556567, -368.0189434323527280 ) ) ;
#19515=LINE ( 'NONE', #22529, #18040 ) ;
#19520=CARTESIAN_POINT ( 'NONE',  ( 755.5713283507202505, -389.3618753856919739, -334.6858677611754729 ) ) ;
#19522=CARTESIAN_POINT ( 'NONE',  ( 768.9521613784389729, -9.827245390607961539, -373.2346286133773106 ) ) ;
#19525=VERTEX_POINT ( 'NONE', #10102 ) ;
#19526=ADVANCED_FACE ( 'NONE', ( #27416 ), #24396, .T. ) ;
#19527=CARTESIAN_POINT ( 'NONE',  ( 804.9511171171677688, -221.8055962898687881, -335.8780910478229202 ) ) ;
#19529=CARTESIAN_POINT ( 'NONE',  ( 758.0141637701419768, -231.0783235625960401, -367.2620300519063790 ) ) ;
#19532=EDGE_LOOP ( 'NONE', ( #3308, #15478, #25696, #35993, #44471, #32801, #43967, #37037 ) ) ;
#19535=CARTESIAN_POINT ( 'NONE',  ( 758.6633372737375112, -20.53286901714212931, -326.9102291470432533 ) ) ;
#19536=CARTESIAN_POINT ( 'NONE',  ( 762.1405469898971887, -169.5436935675108430, -357.8594530101015607 ) ) ;
#19539=CARTESIAN_POINT ( 'NONE',  ( 805.0032342141412300, -85.54369356751118403, -314.9967657858571783 ) ) ;
#19540=CARTESIAN_POINT ( 'NONE',  ( 758.0580252608178853, -78.45278447660211896, -328.0187753319985404 ) ) ;
#19542=CARTESIAN_POINT ( 'NONE',  ( 793.0897708529556667, -6.554518117880697048, -361.3366627262616362 ) ) ;
#19544=CARTESIAN_POINT ( 'NONE',  ( 786.5483106153019435, -367.6454272087886466, -364.1601925771022366 ) ) ;
#19550=CIRCLE ( 'NONE', #23234, 10.00000000000000888 ) ;
#19552=CARTESIAN_POINT ( 'NONE',  ( 773.4516893846965786, -331.6454272087888171, -315.8398074228977066 ) ) ;
#19553=CARTESIAN_POINT ( 'NONE',  ( 785.3141322388236176, -309.7255117493287457, -364.4286716492789537 ) ) ;
#19554=CARTESIAN_POINT ( 'NONE',  ( 805.1927285166397041, -136.8164208402382371, -341.8018195045277707 ) ) ;
#19560=CARTESIAN_POINT ( 'NONE',  ( 793.2243759319678702, -266.5328690171413655, -318.4439275373583200 ) ) ;
#19561=CARTESIAN_POINT ( 'NONE',  ( 745.5313806188320314, -135.2817908451530116, -333.7943932421247268 ) ) ;
#19568=CARTESIAN_POINT ( 'NONE',  ( 777.4774526936600978, -154.2709662947836762, -304.7301800767028226 ) ) ;
#19569=DIRECTION ( 'NONE',  ( -0.000000000000000000, 1.000000000000000000, -0.000000000000000000 ) ) ;
#19572=CARTESIAN_POINT ( 'NONE',  ( 808.0189434323515343, -254.0891481129652334, -319.0252816721025511 ) ) ;
#19574=EDGE_CURVE ( 'NONE', #33292, #14459, #7067, .T. ) ;
#19578=CARTESIAN_POINT ( 'NONE',  ( 744.9990715423526808, -354.3510508353228943, -341.2370466360926002 ) ) ;
#19579=CARTESIAN_POINT ( 'NONE',  ( 772.4837098697144029, -95.36187538569294020, -374.5518280994205611 ) ) ;
#19581=CARTESIAN_POINT ( 'NONE',  ( 759.0252816721024374, -336.9982390220558273, -368.0189434323527280 ) ) ;
#19586=CARTESIAN_POINT ( 'NONE',  ( 759.8311093483677041, -118.1692326535054463, -310.9282345327691814 ) ) ;
#19591=CARTESIAN_POINT ( 'NONE',  ( 796.7845633553578182, -9.623778108051251223, -358.5707757039688204 ) ) ;
#19594=CARTESIAN_POINT ( 'NONE',  ( 748.3538107759620743, -424.7146871989589840, -355.8262568251490165 ) ) ;
#19599=CARTESIAN_POINT ( 'NONE',  ( 783.7953271457878373, -392.1908817542432075, -375.1787889125761239 ) ) ;
#19602=CARTESIAN_POINT ( 'NONE',  ( 792.1044303154645831, -228.4527844766015789, -317.8323909638837677 ) ) ;
#19606=CARTESIAN_POINT ( 'NONE',  ( 793.9708237608222134, -214.9181544815164386, -319.2295555964448681 ) ) ;
#19607=CARTESIAN_POINT ( 'NONE',  ( 805.1927285166397041, -208.8164208402380666, -341.8018195045277707 ) ) ;
#19608=CARTESIAN_POINT ( 'NONE',  ( 768.0187753319979720, -416.6346026584192259, -318.0580252608186242 ) ) ;
#19609=VERTEX_POINT ( 'NONE', #6851 ) ;
#19611=CARTESIAN_POINT ( 'NONE',  ( 759.7806653035534055, -102.9982390220565520, -324.8639956371180801 ) ) ;
#19616=CYLINDRICAL_SURFACE ( 'NONE', #38521, 10.00000000000000888 ) ;
#19619=ORIENTED_EDGE ( 'NONE', *, *, #15065, .F. ) ;
#19620=CARTESIAN_POINT ( 'NONE',  ( 755.8990559732751535, -443.4636090269702322, -365.9055244015606831 ) ) ;
#19621=CARTESIAN_POINT ( 'NONE',  ( 787.4397851343537695, -21.72551174932956641, -374.2001403089903988 ) ) ;
#19624=CARTESIAN_POINT ( 'NONE',  ( 791.9812246680005501, -380.6346026584192828, -361.9419747391813189 ) ) ;
#19625=CARTESIAN_POINT ( 'NONE',  ( 802.1676090361155502, -14.63460265842049779, -327.8955696845344505 ) ) ;
#19629=CARTESIAN_POINT ( 'NONE',  ( 776.9254006560222479, -284.1908817542434917, -314.8983024940802125 ) ) ;
#19630=CARTESIAN_POINT ( 'NONE',  ( 745.0891759886404770, -148.2709662947837330, -342.4968714119734159 ) ) ;
#19634=CARTESIAN_POINT ( 'NONE',  ( 781.4876528434626834, 16.45630643248849267, -313.8857452882203347 ) ) ;
#19640=CARTESIAN_POINT ( 'NONE',  ( 762.1405469898971887, -361.5436935675103882, -357.8594530101015607 ) ) ;
#19644=CARTESIAN_POINT ( 'NONE',  ( 752.7379699480933368, -108.0090635724258448, -361.9858362298580232 ) ) ;
#19645=CARTESIAN_POINT ( 'NONE',  ( 758.6633372737375112, -164.5328690171416781, -326.9102291470432533 ) ) ;
#19649=CARTESIAN_POINT ( 'NONE',  ( 785.3141322388236176, -21.72551174932956641, -364.4286716492789537 ) ) ;
#19650=CARTESIAN_POINT ( 'NONE',  ( 784.0799538623451781, -179.8055962898688733, -364.6971507214555572 ) ) ;
#19652=CARTESIAN_POINT ( 'NONE',  ( 755.0488828828309806, -425.8055962898680491, -344.1219089521771934 ) ) ;
#19658=CARTESIAN_POINT ( 'NONE',  ( 747.6481478633932056, -277.0999726633344267, -353.4146539503763620 ) ) ;
#19665=CARTESIAN_POINT ( 'NONE',  ( 786.5483106153019435, -103.6454272087894850, -364.1601925771022366 ) ) ;
#19666=CARTESIAN_POINT ( 'NONE',  ( 801.9419747391806368, -114.4527844766020053, -351.9812246680014027 ) ) ;
#19667=CARTESIAN_POINT ( 'NONE',  ( 797.8594530101009923, -277.5436935675105588, -322.1405469898982119 ) ) ;
#19669=CARTESIAN_POINT ( 'NONE',  ( 797.8594530101008786, -421.5436935675101040, -322.1405469898980982 ) ) ;
#19670=CARTESIAN_POINT ( 'NONE',  ( 756.5762568750052424, -75.18005720387485269, -348.7366044899774238 ) ) ;
#19678=CARTESIAN_POINT ( 'NONE',  ( 773.7305795820266212, -345.2817908451523863, -374.8230680027170365 ) ) ;
#19681=CARTESIAN_POINT ( 'NONE',  ( 771.1735550268778070, -297.1800572038740711, -316.3353852180827630 ) ) ;
#19684=CARTESIAN_POINT ( 'NONE',  ( 761.4292242960306112, -185.4636090269710280, -323.2154366446414429 ) ) ;
#19687=CARTESIAN_POINT ( 'NONE',  ( 792.3570229623691148, -381.1800572038739006, -373.1304606946836770 ) ) ;
#19693=CARTESIAN_POINT ( 'NONE',  ( 777.4774526936600978, -10.27096629478414691, -304.7301800767027657 ) ) ;
#19694=AXIS2_PLACEMENT_3D ( 'NONE', #4363, #26029, #36676 ) ;
#19696=CARTESIAN_POINT ( 'NONE',  ( 800.2193346964447755, -234.9982390220561683, -355.1360043628815788 ) ) ;
#19697=LINE ( 'NONE', #30306, #339 ) ;
#19700=CARTESIAN_POINT ( 'NONE',  ( 769.1273215169530886, -22.71468719896029853, -317.4527132478988847 ) ) ;
#19702=AXIS2_PLACEMENT_3D ( 'NONE', #39853, #4283, #24823 ) ;
#19703=CARTESIAN_POINT ( 'NONE',  ( 767.9999999999992042, 205.0000000000000568, -350.0000000000000000 ) ) ;
#19708=CARTESIAN_POINT ( 'NONE',  ( 785.3141322388236176, -45.72551174932949181, -364.4286716492789537 ) ) ;
#19710=CARTESIAN_POINT ( 'NONE',  ( 766.7756240680305382, -326.5328690171411381, -361.5560724626415663 ) ) ;
#19713=CARTESIAN_POINT ( 'NONE',  ( 807.5423716828161105, -369.0783235625956422, -362.2119215644372048 ) ) ;
#19718=CARTESIAN_POINT ( 'NONE',  ( 746.8695393053150156, -197.9073299311472169, -327.6429770376306010 ) ) ;
#19721=CARTESIAN_POINT ( 'NONE',  ( 771.1735550268780344, -177.1800572038744974, -316.3353852180828198 ) ) ;
#19723=CARTESIAN_POINT ( 'NONE',  ( 795.1360043628807261, -332.0891481129649492, -360.2193346964456282 ) ) ;
#19724=CARTESIAN_POINT ( 'NONE',  ( 759.0159684113467620, -448.9181544815156144, -325.8855110935213020 ) ) ;
#19727=CARTESIAN_POINT ( 'NONE',  ( 779.9999999999992042, 16.45630643248849267, -370.0000000000000568 ) ) ;
#19730=EDGE_LOOP ( 'NONE', ( #39388, #29439, #15694, #38516, #22168, #22496 ) ) ;
#19731=CARTESIAN_POINT ( 'NONE',  ( 802.5472867521000353, -412.3726999360612808, -350.8726784830461156 ) ) ;
#19735=CARTESIAN_POINT ( 'NONE',  ( 805.6418435158337843, -221.4636090269709428, -363.8556311672236916 ) ) ;
#19739=CARTESIAN_POINT ( 'NONE',  ( 771.2633955100217236, -191.9073299311471885, -363.4237431249939618 ) ) ;
#19740=CARTESIAN_POINT ( 'NONE',  ( 803.2186876482843445, -367.9874144716865203, -350.0220218866286928 ) ) ;
#19742=CARTESIAN_POINT ( 'NONE',  ( 778.7629533639073998, -224.7363362996982232, -375.0009284576466371 ) ) ;
#19744=LINE ( 'NONE', #6339, #26766 ) ;
#19745=CARTESIAN_POINT ( 'NONE',  ( 805.2837595273609850, -98.73633629969859271, -340.5290396650784714 ) ) ;
#19748=CARTESIAN_POINT ( 'NONE',  ( 805.1016975059191054, -414.8965053807771710, -343.0745993439771837 ) ) ;
#19749=CARTESIAN_POINT ( 'NONE',  ( 808.3070685750232087, -282.9982390220559409, -361.1904061080339829 ) ) ;
#19752=CARTESIAN_POINT ( 'NONE',  ( 794.9819416627830151, -60.99823902205671544, -319.9864689768909898 ) ) ;
#19754=CARTESIAN_POINT ( 'NONE',  ( 788.7631598425961101, -169.4419599262325562, -305.7194118038759143 ) ) ;
#19756=CARTESIAN_POINT ( 'NONE',  ( 808.0189434323515343, -422.0891481129647218, -319.0252816721025511 ) ) ;
#19760=CARTESIAN_POINT ( 'NONE',  ( 803.4237431249931660, -375.1800572038739574, -331.2633955100225194 ) ) ;
#19762=CARTESIAN_POINT ( 'NONE',  ( 795.8262568251477660, -46.37269993606239638, -308.3538107759623585 ) ) ;
#19763=CARTESIAN_POINT ( 'NONE',  ( 759.9999999999992042, -462.9681489794448339, -309.9999999999998863 ) ) ;
#19766=CARTESIAN_POINT ( 'NONE',  ( 784.0799538623451781, -227.8055962898687596, -364.6971507214555572 ) ) ;
#19767=CARTESIAN_POINT ( 'NONE',  ( 755.3201227861273992, -123.7255117493292147, -345.3687786644892981 ) ) ;
#19769=CARTESIAN_POINT ( 'NONE',  ( 781.2497674668890113, -252.3510508353232353, -375.3608509340180603 ) ) ;
#19775=CARTESIAN_POINT ( 'NONE',  ( 779.4709603349208464, -24.35105083532392811, -314.7162404726379918 ) ) ;
#19776=CARTESIAN_POINT ( 'NONE',  ( 781.8018195045266339, -166.2709662947835909, -365.1927285166406705 ) ) ;
#19778=CARTESIAN_POINT ( 'NONE',  ( 777.4774526936600978, -82.27096629478388934, -304.7301800767027657 ) ) ;
#19779=CARTESIAN_POINT ( 'NONE',  ( 771.1735550268780344, -57.18005720387490243, -316.3353852180828198 ) ) ;
#19780=CARTESIAN_POINT ( 'NONE',  ( 793.9708237608222134, 1.081845518482914104, -319.2295555964448681 ) ) ;
#19782=CARTESIAN_POINT ( 'NONE',  ( 804.8461984189677878, -338.1908817542433212, -336.9566956441385628 ) ) ;
#19790=CARTESIAN_POINT ( 'NONE',  ( 802.5472867521000353, -316.3726999360615082, -350.8726784830461156 ) ) ;
#19791=CARTESIAN_POINT ( 'NONE',  ( 759.9864689768902508, -314.0891481129650629, -354.9819416627836404 ) ) ;
#19792=CARTESIAN_POINT ( 'NONE',  ( 813.5763878283155464, -147.8272453906075157, -351.1614460488615350 ) ) ;
#19796=CARTESIAN_POINT ( 'NONE',  ( 781.2370466360911223, -116.7363362996985217, -304.9990715423533629 ) ) ;
#19801=VERTEX_POINT ( 'NONE', #44760 ) ;
#19803=CARTESIAN_POINT ( 'NONE',  ( 782.5225473063383106, -166.2709662947836478, -375.2698199232970637 ) ) ;
#19805=AXIS2_PLACEMENT_3D ( 'NONE', #20370, #8458, #40097 ) ;
#19807=CARTESIAN_POINT ( 'NONE',  ( 767.6429770376289525, -297.1800572038740711, -306.8695393053162093 ) ) ;
#19808=CARTESIAN_POINT ( 'NONE',  ( 804.7487373415286811, -451.5436935675099903, -364.7487373415288516 ) ) ;
#19812=CARTESIAN_POINT ( 'NONE',  ( 788.7631598425961101, -337.4419599262319593, -305.7194118038759143 ) ) ;
#19813=CARTESIAN_POINT ( 'NONE',  ( 814.2001403089898304, -89.36187538569299704, -347.4397851343538264 ) ) ;
#19815=CARTESIAN_POINT ( 'NONE',  ( 792.3570229623688874, -381.1800572038737869, -373.1304606946836202 ) ) ;
#19820=CARTESIAN_POINT ( 'NONE',  ( 764.3348316497523456, -118.7146871989600072, -308.6759233522265617 ) ) ;
#19825=CARTESIAN_POINT ( 'NONE',  ( 763.2154366446407039, 2.376221891948710585, -321.4292242960311228 ) ) ;
#19827=CARTESIAN_POINT ( 'NONE',  ( 747.3154664389472828, -427.9874144716862929, -326.4474001241230781 ) ) ;
#19831=CARTESIAN_POINT ( 'NONE',  ( 752.7379699480933368, -372.0090635724250205, -361.9858362298580232 ) ) ;
#19833=CARTESIAN_POINT ( 'NONE',  ( 804.9363028652555840, -232.2709662947834488, -338.2165204200192079 ) ) ;
#19837=CARTESIAN_POINT ( 'NONE',  ( 755.3028492785439312, -207.2817908451527842, -335.9200461376539693 ) ) ;
#19838=CARTESIAN_POINT ( 'NONE',  ( 797.6776695296629214, -235.5436935675107293, -357.6776695296636603 ) ) ;
#19839=CARTESIAN_POINT ( 'NONE',  ( 794.9819416627830151, -420.9982390220555999, -319.9864689768909898 ) ) ;
#19840=EDGE_LOOP ( 'NONE', ( #38297, #37461, #40719, #34430 ) ) ;
#19842=CARTESIAN_POINT ( 'NONE',  ( 803.4237431249931660, -111.1800572038747532, -331.2633955100225194 ) ) ;
#19853=CARTESIAN_POINT ( 'NONE',  ( 802.2119215644370342, -438.0090635724247932, -367.5423716828165084 ) ) ;
#19854=CARTESIAN_POINT ( 'NONE',  ( 748.9653473494365699, -50.63460265842038410, -356.9462024416520762 ) ) ;
#19856=CARTESIAN_POINT ( 'NONE',  ( 781.8018195045266339, -430.2709662947827383, -365.1927285166406705 ) ) ;
#19857=CARTESIAN_POINT ( 'NONE',  ( 754.8072714833583632, -28.81642084023863504, -338.1981804954721156 ) ) ;
#19860=CARTESIAN_POINT ( 'NONE',  ( 775.8780910478218402, -297.2817908451526137, -364.9511171171680530 ) ) ;
#19861=CARTESIAN_POINT ( 'NONE',  ( 748.9653473494363425, -170.6346026584199649, -356.9462024416521331 ) ) ;
#19864=CARTESIAN_POINT ( 'NONE',  ( 794.1255485493337574, 16.45630643248849978, -314.6638991903497526 ) ) ;
#19867=CARTESIAN_POINT ( 'NONE',  ( 788.7631598425961101, -241.4419599262322720, -305.7194118038759143 ) ) ;
#19874=CARTESIAN_POINT ( 'NONE',  ( 774.6858677611749044, -369.7255117493284615, -315.5713283507209894 ) ) ;
#19877=CARTESIAN_POINT ( 'NONE',  ( 781.2370466360911223, -116.7363362996985217, -304.9990715423533629 ) ) ;
#19878=CARTESIAN_POINT ( 'NONE',  ( 755.0488828828309806, -137.8055962898690154, -344.1219089521771934 ) ) ;
#19881=CARTESIAN_POINT ( 'NONE',  ( 788.7366044899766848, -59.90732993114762905, -316.5762568750059813 ) ) ;
#19882=CARTESIAN_POINT ( 'NONE',  ( 804.1601925771018387, -151.4419599262326415, -346.5483106153029098 ) ) ;
#19884=CARTESIAN_POINT ( 'NONE',  ( 788.7631598425961101, -1.441959926233096656, -305.7194118038759143 ) ) ;
#19890=CARTESIAN_POINT ( 'NONE',  ( 811.3240766477731540, -268.3726999360616787, -355.6651683502462902 ) ) ;
#19891=EDGE_CURVE ( 'NONE', #3536, #30163, #16560, .T. ) ;
#19899=CARTESIAN_POINT ( 'NONE',  ( 775.8780910478218402, -129.2817908451530400, -364.9511171171680530 ) ) ;
#19900=CARTESIAN_POINT ( 'NONE',  ( 788.8264449731200330, -117.1800572038746964, -363.6646147819171233 ) ) ;
#19901=CARTESIAN_POINT ( 'NONE',  ( 804.9363028652555840, -328.2709662947831362, -338.2165204200192079 ) ) ;
#19903=CARTESIAN_POINT ( 'NONE',  ( 757.8323909638827445, -434.6346026584190554, -352.1044303154654358 ) ) ;
#19910=CARTESIAN_POINT ( 'NONE',  ( 781.2370466360911223, -356.7363362996978253, -304.9990715423533629 ) ) ;
#19912=CARTESIAN_POINT ( 'NONE',  ( 797.6776695296629214, -307.5436935675104451, -357.6776695296636603 ) ) ;
#19914=CARTESIAN_POINT ( 'NONE',  ( 772.4468031744293057, -201.8272453906073451, -363.8651313633793620 ) ) ;
#19917=CARTESIAN_POINT ( 'NONE',  ( 808.0189434323515343, -374.0891481129647786, -319.0252816721025511 ) ) ;
#19918=CARTESIAN_POINT ( 'NONE',  ( 799.9999999999993179, -512.9681489794448908, -350.0000000000000000 ) ) ;
#19924=CARTESIAN_POINT ( 'NONE',  ( 745.4481719005789273, -27.72551174932954510, -347.5162901302853129 ) ) ;
#19925=CARTESIAN_POINT ( 'NONE',  ( 785.3687786644884454, -251.3618753856923149, -315.3201227861279676 ) ) ;
#19929=CARTESIAN_POINT ( 'NONE',  ( 787.6308680596127942, -59.26014174441473870, -364.1105419155492768 ) ) ;
#19937=CARTESIAN_POINT ( 'NONE',  ( 804.9511171171677688, -365.8055962898682765, -335.8780910478229202 ) ) ;
#19940=CARTESIAN_POINT ( 'NONE',  ( 773.7943932421234194, -359.8055962898683333, -305.5313806188329409 ) ) ;
#19946=CARTESIAN_POINT ( 'NONE',  ( 815.2698199232961542, -208.8164208402380666, -342.5225473063383106 ) ) ;
#19949=ORIENTED_EDGE ( 'NONE', *, *, #43665, .T. ) ;
#19950=CARTESIAN_POINT ( 'NONE',  ( 803.4237431249931660, -207.1800572038744406, -331.2633955100225194 ) ) ;
#19951=ORIENTED_EDGE ( 'NONE', *, *, #20048, .F. ) ;
#19952=CARTESIAN_POINT ( 'NONE',  ( 785.3687786644884454, -323.3618753856923149, -315.3201227861279676 ) ) ;
#19953=CARTESIAN_POINT ( 'NONE',  ( 797.8594530101008786, 10.45630643248850866, -322.1405469898980982 ) ) ;
#19961=CARTESIAN_POINT ( 'NONE',  ( 785.3687786644884454, 12.63812461430668321, -315.3201227861279676 ) ) ;
#19965=CARTESIAN_POINT ( 'NONE',  ( 746.4236121716829757, -231.8272453906072315, -328.8385539511384650 ) ) ;
#19968=CARTESIAN_POINT ( 'NONE',  ( 755.5713283507202505, -197.3618753856926560, -334.6858677611754729 ) ) ;
#19969=CARTESIAN_POINT ( 'NONE',  ( 793.2243759319678702, -362.5328690171410813, -318.4439275373583200 ) ) ;
#19970=CARTESIAN_POINT ( 'NONE',  ( 804.1009440267234822, -215.4636090269709712, -314.0944755984392600 ) ) ;
#19972=CARTESIAN_POINT ( 'NONE',  ( 775.8780910478218402, -81.28179084515319630, -364.9511171171680530 ) ) ;
#19975=CARTESIAN_POINT ( 'NONE',  ( 756.1348686366196716, -425.2601417444136018, -347.5531968255698416 ) ) ;
#19976=CARTESIAN_POINT ( 'NONE',  ( 808.0189434323515343, -278.0891481129651197, -319.0252816721025511 ) ) ;
#19979=CARTESIAN_POINT ( 'NONE',  ( 781.7834795799800531, -34.81642084023861372, -315.0636971347436202 ) ) ;
#19981=CARTESIAN_POINT ( 'NONE',  ( 810.1134526219336749, -152.5328690171416781, -357.8822607201570349 ) ) ;
#19983=CARTESIAN_POINT ( 'NONE',  ( 745.7998596910086917, -413.3618753856920307, -332.5602148656461168 ) ) ;
#19987=CARTESIAN_POINT ( 'NONE',  ( 785.3687786644884454, -443.3618753856917465, -315.3201227861279676 ) ) ;
#19991=ORIENTED_EDGE ( 'NONE', *, *, #31205, .F. ) ;
#19992=CARTESIAN_POINT ( 'NONE',  ( 765.8855110935204493, -238.1692326535050768, -319.0159684113471599 ) ) ;
#19994=CARTESIAN_POINT ( 'NONE',  ( 744.8212110874229666, -258.8965053807777963, -336.2046728542121627 ) ) ;
#19997=EDGE_LOOP ( 'NONE', ( #37496, #28185, #40735, #21770 ) ) ;
#19999=CARTESIAN_POINT ( 'NONE',  ( 781.8018195045266339, -190.2709662947835909, -365.1927285166406705 ) ) ;
#20001=CARTESIAN_POINT ( 'NONE',  ( 748.9653473494363425, -122.6346026584201354, -356.9462024416521331 ) ) ;
#20002=CARTESIAN_POINT ( 'NONE',  ( 802.1676090361155502, -62.63460265842032726, -327.8955696845344505 ) ) ;
#20004=CARTESIAN_POINT ( 'NONE',  ( 804.1105419155481968, -51.82724539060782121, -347.6308680596136469 ) ) ;
#20006=CARTESIAN_POINT ( 'NONE',  ( 773.4516893846965786, -355.6454272087887603, -315.8398074228977066 ) ) ;
#20012=CARTESIAN_POINT ( 'NONE',  ( 779.4763451958990572, -320.7363362996979390, -365.0264073115438919 ) ) ;
#20013=CARTESIAN_POINT ( 'NONE',  ( 800.2193346964447755, -330.9982390220558273, -355.1360043628815788 ) ) ;
#20014=CARTESIAN_POINT ( 'NONE',  ( 815.3608509340175488, -122.7363362996985074, -341.2497674668889545 ) ) ;
#20018=CARTESIAN_POINT ( 'NONE',  ( 802.7791456095903868, -268.7146871989595525, -329.0155153010375102 ) ) ;
#20019=CARTESIAN_POINT ( 'NONE',  ( 797.8822607201568644, -102.5545181178804057, -370.1134526219340160 ) ) ;
#20023=ORIENTED_EDGE ( 'NONE', *, *, #14855, .T. ) ;
#20025=CARTESIAN_POINT ( 'NONE',  ( 759.0252816721024374, -168.9982390220563673, -368.0189434323527280 ) ) ;
#20028=CARTESIAN_POINT ( 'NONE',  ( 804.7487373415286811, -307.5436935675104451, -364.7487373415288516 ) ) ;
#20034=CARTESIAN_POINT ( 'NONE',  ( 749.8865473780648472, -356.5328690171410813, -322.1177392798429082 ) ) ;
#20035=CARTESIAN_POINT ( 'NONE',  ( 810.7187646348534145, -114.4527844766020053, -356.7737145352016341 ) ) ;
#20037=CARTESIAN_POINT ( 'NONE',  ( 782.4968714119720516, -394.8164208402374697, -305.0891759886411023 ) ) ;
#20041=CARTESIAN_POINT ( 'NONE',  ( 805.9055244015594326, -171.6237781080507432, -315.8990559732753240 ) ) ;
#20047=CARTESIAN_POINT ( 'NONE',  ( 763.2262854647970016, -8.634602658420517329, -309.2812353651462445 ) ) ;
#20048=EDGE_CURVE ( 'NONE', #17925, #16350, #35954, .T. ) ;
#20052=CARTESIAN_POINT ( 'NONE',  ( 795.8262568251477660, -406.3726999360612808, -308.3538107759623585 ) ) ;
#20055=CARTESIAN_POINT ( 'NONE',  ( 772.4468031744293057, -225.8272453906072599, -363.8651313633793620 ) ) ;
#20056=CARTESIAN_POINT ( 'NONE',  ( 754.8072714833581358, -220.8164208402379529, -338.1981804954720587 ) ) ;
#20057=CIRCLE ( 'NONE', #32646, 10.00000000000000888 ) ;
#20058=CARTESIAN_POINT ( 'NONE',  ( 774.6312213355098493, -431.3618753856918602, -364.6798772138717482 ) ) ;
#20060=CARTESIAN_POINT ( 'NONE',  ( 804.6798772138708955, -111.7255117493293000, -334.6312213355107019 ) ) ;
#20064=CARTESIAN_POINT ( 'NONE',  ( 815.3608509340175488, -2.736336299698892027, -341.2497674668889545 ) ) ;
#20071=CARTESIAN_POINT ( 'NONE',  ( 781.2370466360911223, -452.7363362996975411, -304.9990715423533629 ) ) ;
#20072=CARTESIAN_POINT ( 'NONE',  ( 758.8095938919644823, -56.08914811296581604, -311.6929314249762797 ) ) ;
#20074=CARTESIAN_POINT ( 'NONE',  ( 794.9819416627830151, -420.9982390220555999, -319.9864689768909898 ) ) ;
#20075=CARTESIAN_POINT ( 'NONE',  ( 794.9819416627830151, -36.99823902205679360, -319.9864689768909898 ) ) ;
#20078=CARTESIAN_POINT ( 'NONE',  ( 802.9823548866075953, -289.0999726633343698, -330.0799878456151077 ) ) ;
#20079=CARTESIAN_POINT ( 'NONE',  ( 814.5518280994195948, -207.7255117493289447, -332.4837098697145734 ) ) ;
#20085=CARTESIAN_POINT ( 'NONE',  ( 815.1787889125755555, -222.8965053807778531, -343.7953271457877804 ) ) ;
#20087=CARTESIAN_POINT ( 'NONE',  ( 745.4481719005789273, -267.7255117493286320, -347.5162901302853129 ) ) ;
#20091=CARTESIAN_POINT ( 'NONE',  ( 794.9819416627830151, -348.9982390220558273, -319.9864689768909898 ) ) ;
#20093=CARTESIAN_POINT ( 'NONE',  ( 756.1443688327750579, -45.62377810805114109, -314.3581564841659315 ) ) ;
#20094=CARTESIAN_POINT ( 'NONE',  ( 799.4546378042377910, -153.0783235625962675, -356.1575198192848006 ) ) ;
#20099=CARTESIAN_POINT ( 'NONE',  ( 754.8072714833581358, -52.81642084023856398, -338.1981804954720587 ) ) ;
#20100=CARTESIAN_POINT ( 'NONE',  ( 773.3843516231979720, -157.4419599262326130, -364.4086373105754433 ) ) ;
#20103=CARTESIAN_POINT ( 'NONE',  ( 766.5853460496234675, -13.98741447168760033, -372.3518521366060554 ) ) ;
#20108=CARTESIAN_POINT ( 'NONE',  ( 804.1009440267234822, -287.4636090269708575, -314.0944755984392600 ) ) ;
#20115=ORIENTED_EDGE ( 'NONE', *, *, #30652, .T. ) ;
#20116=CARTESIAN_POINT ( 'NONE',  ( 802.9823548866075953, -121.0999726633348956, -330.0799878456151077 ) ) ;
#20117=CARTESIAN_POINT ( 'NONE',  ( 756.3353852180819104, -125.9073299311474159, -331.1735550268788302 ) ) ;
#20119=CARTESIAN_POINT ( 'NONE',  ( 774.6858677611749044, -321.7255117493286320, -315.5713283507209894 ) ) ;
#20121=CARTESIAN_POINT ( 'NONE',  ( 788.7366044899766848, -443.9073299311464780, -316.5762568750059813 ) ) ;
#20124=CARTESIAN_POINT ( 'NONE',  ( 779.9999999999992042, 16.45630643248849267, -309.9999999999998863 ) ) ;
#20128=CARTESIAN_POINT ( 'NONE',  ( 745.7194118038753459, -349.6454272087887603, -348.7631598425976449 ) ) ;
#20130=CARTESIAN_POINT ( 'NONE',  ( 765.0180583372156207, -312.9982390220559409, -360.0135310231089534 ) ) ;
#20132=CARTESIAN_POINT ( 'NONE',  ( 796.9571628226829034, -191.4636090269709996, -321.2382568024804641 ) ) ;
#20135=CARTESIAN_POINT ( 'NONE',  ( 782.4968714119720516, -394.8164208402374697, -305.0891759886411023 ) ) ;
#20140=CARTESIAN_POINT ( 'NONE',  ( 755.2512626584698410, -7.543693567511430942, -315.2512626584710915 ) ) ;
#20141=CARTESIAN_POINT ( 'NONE',  ( 762.1405469898971887, -241.5436935675106156, -357.8594530101015607 ) ) ;
#20147=CARTESIAN_POINT ( 'NONE',  ( 764.0069404352550464, -39.07832356259662276, -359.2566176426627180 ) ) ;
#20153=CARTESIAN_POINT ( 'NONE',  ( 762.1405469898971887, -49.54369356751129061, -357.8594530101015607 ) ) ;
#20156=CARTESIAN_POINT ( 'NONE',  ( 773.3843516231979720, -349.4419599262320162, -364.4086373105754433 ) ) ;
#20159=CARTESIAN_POINT ( 'NONE',  ( 761.9338519418445230, -374.5328690171410813, -370.4231160770881957 ) ) ;
#20165=CARTESIAN_POINT ( 'NONE',  ( 763.2262854647970016, -224.6346026584198228, -309.2812353651462445 ) ) ;
#20167=VERTEX_POINT ( 'NONE', #30148 ) ;
#20168=CARTESIAN_POINT ( 'NONE',  ( 778.1981804954715471, -226.2709662947834488, -314.8072714833591021 ) ) ;
#20171=CARTESIAN_POINT ( 'NONE',  ( 804.1105419155481968, -459.8272453906066062, -347.6308680596136469 ) ) ;
#20179=CARTESIAN_POINT ( 'NONE',  ( 804.9363028652555840, 7.729033705215793582, -338.2165204200192079 ) ) ;
#20184=CARTESIAN_POINT ( 'NONE',  ( 788.6739635108323228, -247.6454272087890160, -373.9316612368139090 ) ) ;
#20187=CARTESIAN_POINT ( 'NONE',  ( 788.7366044899766848, -227.9073299311471033, -316.5762568750059813 ) ) ;
#20188=CARTESIAN_POINT ( 'NONE',  ( 764.0069404352550464, -351.0783235625955854, -359.2566176426627180 ) ) ;
#20189=CARTESIAN_POINT ( 'NONE',  ( 749.5768839229115201, -252.5545181178799226, -358.0661480581553064 ) ) ;
#20192=CARTESIAN_POINT ( 'NONE',  ( 800.9840315886518738, -76.91815448151683654, -354.1144889064786412 ) ) ;
#20196=CARTESIAN_POINT ( 'NONE',  ( 792.3570229623691148, -261.1800572038742416, -373.1304606946836770 ) ) ;
#20199=CARTESIAN_POINT ( 'NONE',  ( 797.8594530101008786, -37.54369356751132614, -322.1405469898980982 ) ) ;
#20202=CARTESIAN_POINT ( 'NONE',  ( 807.5423716828161105, -177.0783235625961538, -362.2119215644372048 ) ) ;
#20204=CARTESIAN_POINT ( 'NONE',  ( 767.6429770376289525, -417.1800572038736163, -306.8695393053162093 ) ) ;
#20209=CARTESIAN_POINT ( 'NONE',  ( 756.3353852180819104, -437.9073299311463074, -331.1735550268788302 ) ) ;
#20215=CARTESIAN_POINT ( 'NONE',  ( 803.8651313633788504, -269.2601417444139997, -332.4468031744301015 ) ) ;
#20217=AXIS2_PLACEMENT_3D ( 'NONE', #28255, #17435, #45618 ) ;
#20218=CARTESIAN_POINT ( 'NONE',  ( 808.7758568127978833, -268.1692326535049347, -320.0363995740631822 ) ) ;
#20221=ORIENTED_EDGE ( 'NONE', *, *, #20442, .F. ) ;
#20224=CARTESIAN_POINT ( 'NONE',  ( 792.1044303154645831, -156.4527844766018916, -317.8323909638837677 ) ) ;
#20226=CARTESIAN_POINT ( 'NONE',  ( 751.6929314249748586, -102.9982390220565520, -318.8095938919659034 ) ) ;
#20227=CARTESIAN_POINT ( 'NONE',  ( 805.1927285166399315, -112.8164208402383650, -341.8018195045277707 ) ) ;
#20229=CARTESIAN_POINT ( 'NONE',  ( 796.1575198192839480, -30.00906357242607925, -359.4546378042384163 ) ) ;
#20230=CARTESIAN_POINT ( 'NONE',  ( 804.8461984189677878, -362.1908817542432644, -336.9566956441385628 ) ) ;
#20238=CARTESIAN_POINT ( 'NONE',  ( 757.0176451133909268, -373.0999726633340856, -349.9200121543848354 ) ) ;
#20239=CARTESIAN_POINT ( 'NONE',  ( 778.2165204200184689, -310.8164208402377540, -364.9363028652563230 ) ) ;
#20240=CARTESIAN_POINT ( 'NONE',  ( 773.7305795820266212, -129.2817908451530400, -374.8230680027170365 ) ) ;
#20243=CARTESIAN_POINT ( 'NONE',  ( 761.2382568024794409, -255.6237781080504874, -356.9571628226838129 ) ) ;
#20244=CARTESIAN_POINT ( 'NONE',  ( 748.6759233522253680, -136.3726999360621051, -324.3348316497537098 ) ) ;
#20251=CARTESIAN_POINT ( 'NONE',  ( 810.7187646348534145, -186.4527844766017779, -356.7737145352016341 ) ) ;
#20255=CARTESIAN_POINT ( 'NONE',  ( 751.9810565676468741, -290.0891481129650629, -360.9747183278973921 ) ) ;
#20261=CARTESIAN_POINT ( 'NONE',  ( 744.8212110874229666, -378.8965053807772847, -336.2046728542121627 ) ) ;
#20262=CARTESIAN_POINT ( 'NONE',  ( 805.0032342141412300, -109.5436935675110988, -314.9967657858571783 ) ) ;
#20265=CARTESIAN_POINT ( 'NONE',  ( 746.8695393053150156, -389.9073299311465348, -327.6429770376306010 ) ) ;
#20270=CARTESIAN_POINT ( 'NONE',  ( 795.6651683502461765, -154.7146871989598935, -371.3240766477733814 ) ) ;
#20275=CARTESIAN_POINT ( 'NONE',  ( 799.4546378042377910, -9.078323562596708030, -356.1575198192848006 ) ) ;
#20277=CARTESIAN_POINT ( 'NONE',  ( 767.7687537140311633, 0.09267006885218045942, -372.7932403749916830 ) ) ;
#20280=CARTESIAN_POINT ( 'NONE',  ( 802.1676090361156639, -182.6346026584199649, -327.8955696845344505 ) ) ;
#20281=CARTESIAN_POINT ( 'NONE',  ( 760.0363995740630116, -394.9181544815158418, -368.7758568127991907 ) ) ;
#20283=CARTESIAN_POINT ( 'NONE',  ( 792.1044303154645831, -252.4527844766015789, -317.8323909638837677 ) ) ;
#20286=CARTESIAN_POINT ( 'NONE',  ( 796.1575198192839480, -270.0090635724253048, -359.4546378042384163 ) ) ;
#20287=CARTESIAN_POINT ( 'NONE',  ( 781.8018195045266339, -214.2709662947834488, -365.1927285166406705 ) ) ;
#20288=CARTESIAN_POINT ( 'NONE',  ( 800.0135310231082713, -422.0891481129647218, -325.0180583372163028 ) ) ;
#20294=CARTESIAN_POINT ( 'NONE',  ( 788.6739635108323228, -7.645427208789786100, -373.9316612368139090 ) ) ;
#20301=CARTESIAN_POINT ( 'NONE',  ( 762.1177392798416577, -450.5545181178793541, -309.8865473780659272 ) ) ;
#20302=CARTESIAN_POINT ( 'NONE',  ( 805.0032342141413437, -61.54369356751124798, -314.9967657858572352 ) ) ;
#20304=CARTESIAN_POINT ( 'NONE',  ( 804.4286716492782716, -425.3618753856919170, -345.3141322388244703 ) ) ;
#20305=CARTESIAN_POINT ( 'NONE',  ( 767.8955696845334842, -48.45278447660221133, -362.1676090361161755 ) ) ;
#20308=CARTESIAN_POINT ( 'NONE',  ( 782.5225473063381969, -214.2709662947834488, -375.2698199232970637 ) ) ;
#20312=CARTESIAN_POINT ( 'NONE',  ( 799.9999999999993179, 205.0000000000000568, -360.0000000000000000 ) ) ;
#20313=CARTESIAN_POINT ( 'NONE',  ( 748.3538107759620743, -280.7146871989594956, -355.8262568251490165 ) ) ;
#20316=CARTESIAN_POINT ( 'NONE',  ( 759.0252816721024374, -288.9982390220559978, -368.0189434323527280 ) ) ;
#20320=CARTESIAN_POINT ( 'NONE',  ( 754.8072714833581358, -340.8164208402376971, -338.1981804954720587 ) ) ;
#20322=CARTESIAN_POINT ( 'NONE',  ( 815.0009284576459549, -54.35105083532383219, -338.7629533639073429 ) ) ;
#20323=CARTESIAN_POINT ( 'NONE',  ( 775.9200461376533440, -167.8055962898689586, -315.3028492785443291 ) ) ;
#20328=CARTESIAN_POINT ( 'NONE',  ( 755.0636971347428243, -76.27096629478394618, -341.7834795799807353 ) ) ;
#20329=CARTESIAN_POINT ( 'NONE',  ( 755.0488828828309806, -161.8055962898689870, -344.1219089521771934 ) ) ;
#20331=VECTOR ( 'NONE', #43527, 1000.000000000000000 ) ;
#20333=CARTESIAN_POINT ( 'NONE',  ( 795.6651683502461765, 13.28531280103958423, -371.3240766477733814 ) ) ;
#20339=CARTESIAN_POINT ( 'NONE',  ( 793.5525998758768083, -295.0999726633343698, -372.6845335610516941 ) ) ;
#20344=CARTESIAN_POINT ( 'NONE',  ( 793.0897708529556667, -102.5545181178804057, -361.3366627262616362 ) ) ;
#20345=CARTESIAN_POINT ( 'NONE',  ( 804.4286716492782716, -113.3618753856929260, -345.3141322388244703 ) ) ;
#20346=CARTESIAN_POINT ( 'NONE',  ( 797.8594530101009923, -325.5436935675104451, -322.1405469898982119 ) ) ;
#20348=CARTESIAN_POINT ( 'NONE',  ( 771.1735550268778070, -417.1800572038736163, -316.3353852180827630 ) ) ;
#20351=DIRECTION ( 'NONE',  ( 1.000000000000000000, 0.000000000000000000, -0.000000000000000000 ) ) ;
#20352=CARTESIAN_POINT ( 'NONE',  ( 791.4716058693660443, -452.9681489794448339, -367.7200696026887954 ) ) ;
#20356=CARTESIAN_POINT ( 'NONE',  ( 804.1009440267234822, -335.4636090269705733, -314.0944755984392600 ) ) ;
#20359=CARTESIAN_POINT ( 'NONE',  ( 792.1044303154645831, -324.4527844766013231, -317.8323909638837677 ) ) ;
#20362=CARTESIAN_POINT ( 'NONE',  ( 793.0897708529556667, -198.5545181178800647, -361.3366627262616362 ) ) ;
#20367=CARTESIAN_POINT ( 'NONE',  ( 814.9108240113580450, -376.2709662947829656, -337.5031285880265273 ) ) ;
#20370=CARTESIAN_POINT ( 'NONE',  ( 759.9999999999992042, -512.9681489794448908, -339.9999999999999432 ) ) ;
#20372=CARTESIAN_POINT ( 'NONE',  ( 763.2262854647970016, -8.634602658420517329, -309.2812353651462445 ) ) ;
#20373=CARTESIAN_POINT ( 'NONE',  ( 781.8018195045266339, -238.2709662947833920, -365.1927285166406705 ) ) ;
#20377=CARTESIAN_POINT ( 'NONE',  ( 755.8398074228967971, -43.44195992623296831, -333.4516893846970333 ) ) ;
#20383=CARTESIAN_POINT ( 'NONE',  ( 755.5713283507202505, -77.36187538569302546, -334.6858677611754729 ) ) ;
#20385=CARTESIAN_POINT ( 'NONE',  ( 763.2154366446407039, -357.6237781080501463, -321.4292242960311228 ) ) ;
#20389=CARTESIAN_POINT ( 'NONE',  ( 745.1769319972822814, -377.8055962898682765, -346.2694204179732083 ) ) ;
#20395=VECTOR ( 'NONE', #11057, 1000.000000000000000 ) ;
#20396=CARTESIAN_POINT ( 'NONE',  ( 814.9108240113580450, -232.2709662947834488, -337.5031285880265273 ) ) ;
#20399=CARTESIAN_POINT ( 'NONE',  ( 792.1044303154646968, -228.4527844766016074, -317.8323909638837677 ) ) ;
#20401=CARTESIAN_POINT ( 'NONE',  ( 756.3353852180819104, -341.9073299311465917, -331.1735550268788302 ) ) ;
#20402=CARTESIAN_POINT ( 'NONE',  ( 800.2193346964447755, 5.001760977943074948, -355.1360043628815788 ) ) ;
#20409=CARTESIAN_POINT ( 'NONE',  ( 804.8461984189677878, -458.1908817542429802, -336.9566956441385628 ) ) ;
#20412=ORIENTED_EDGE ( 'NONE', *, *, #38242, .T. ) ;
#20413=CARTESIAN_POINT ( 'NONE',  ( 764.1737431748507561, -250.3726999360618208, -371.6461892240376415 ) ) ;
#20417=CARTESIAN_POINT ( 'NONE',  ( 803.6646147819161570, -209.9073299311470748, -348.8264449731210561 ) ) ;
#20418=CARTESIAN_POINT ( 'NONE',  ( 800.7704444035546203, -412.1692326535045936, -326.0291762391768771 ) ) ;
#20419=CARTESIAN_POINT ( 'NONE',  ( 815.3608509340175488, -242.7363362996980811, -341.2497674668889545 ) ) ;
#20422=CARTESIAN_POINT ( 'NONE',  ( 804.8461984189677878, -74.19088175424410281, -336.9566956441385628 ) ) ;
#20428=CARTESIAN_POINT ( 'NONE',  ( 775.9200461376533440, -431.8055962898681059, -315.3028492785443291 ) ) ;
#20429=CARTESIAN_POINT ( 'NONE',  ( 751.9810565676468741, -290.0891481129650629, -360.9747183278973921 ) ) ;
#20430=FACE_OUTER_BOUND ( 'NONE', #11550, .T. ) ;
#20432=CARTESIAN_POINT ( 'NONE',  ( 792.1044303154645831, -84.45278447660206211, -317.8323909638837677 ) ) ;
#20435=CARTESIAN_POINT ( 'NONE',  ( 761.9338519418445230, -158.5328690171417065, -370.4231160770881957 ) ) ;
#20437=CARTESIAN_POINT ( 'NONE',  ( 815.2698199232961542, -400.8164208402373561, -342.5225473063383106 ) ) ;
#20439=DIRECTION ( 'NONE',  ( 0.000000000000000000, 0.000000000000000000, -1.000000000000000000 ) ) ;
#20442=EDGE_CURVE ( 'NONE', #24791, #39264, #19515, .T. ) ;
#20443=CARTESIAN_POINT ( 'NONE',  ( 759.7806653035534055, -438.9982390220553157, -324.8639956371180801 ) ) ;
#20450=CARTESIAN_POINT ( 'NONE',  ( 787.6308680596127942, -275.2601417444140566, -364.1105419155492768 ) ) ;
#20451=CARTESIAN_POINT ( 'NONE',  ( 788.7366044899766848, -131.9073299311473875, -316.5762568750059813 ) ) ;
#20453=CARTESIAN_POINT ( 'NONE',  ( 745.1769319972822814, -257.8055962898686744, -346.2694204179732083 ) ) ;
#20459=CARTESIAN_POINT ( 'NONE',  ( 773.3843516231979720, -61.44195992623291147, -364.4086373105754433 ) ) ;
#20460=CARTESIAN_POINT ( 'NONE',  ( 788.7366044899766848, -155.9073299311473306, -316.5762568750059813 ) ) ;
#20462=CARTESIAN_POINT ( 'NONE',  ( 777.4774526936600978, -106.2709662947838467, -304.7301800767027657 ) ) ;
#20463=CARTESIAN_POINT ( 'NONE',  ( 778.2165204200184689, -118.8164208402383508, -364.9363028652563230 ) ) ;
#20465=CARTESIAN_POINT ( 'NONE',  ( 799.2566176426618085, -48.00906357242602951, -324.0069404352559559 ) ) ;
#20467=CARTESIAN_POINT ( 'NONE',  ( 790.0220218866281812, -367.0999726633342561, -363.2186876482849129 ) ) ;
#20477=CARTESIAN_POINT ( 'NONE',  ( 755.1538015810308480, -374.1908817542432075, -343.0433043558613804 ) ) ;
#20478=CARTESIAN_POINT ( 'NONE',  ( 759.9864689768902508, -362.0891481129648923, -354.9819416627836404 ) ) ;
#20479=CARTESIAN_POINT ( 'NONE',  ( 766.4474001241216001, -139.0999726633348530, -307.3154664389482491 ) ) ;
#20483=CARTESIAN_POINT ( 'NONE',  ( 775.9200461376533440, -263.8055962898686175, -315.3028492785443291 ) ) ;
#20484=CARTESIAN_POINT ( 'NONE',  ( 815.3608509340175488, -170.7363362996983938, -341.2497674668889545 ) ) ;
#20490=CARTESIAN_POINT ( 'NONE',  ( 751.6929314249750860, -174.9982390220563673, -318.8095938919659034 ) ) ;
#20493=CARTESIAN_POINT ( 'NONE',  ( 751.6929314249748586, -318.9982390220557704, -318.8095938919659034 ) ) ;
#20499=CARTESIAN_POINT ( 'NONE',  ( 748.3538107759620743, -376.7146871989592682, -355.8262568251490165 ) ) ;
#20501=CARTESIAN_POINT ( 'NONE',  ( 808.3070685750230950, -114.9982390220565236, -361.1904061080339261 ) ) ;
#20503=CARTESIAN_POINT ( 'NONE',  ( 814.9108240113580450, -400.2709662947828519, -337.5031285880265273 ) ) ;
#20508=CARTESIAN_POINT ( 'NONE',  ( 764.3348316497523456, -166.7146871989598367, -308.6759233522265617 ) ) ;
#20514=CARTESIAN_POINT ( 'NONE',  ( 748.9653473494363425, -2.634602658420536869, -356.9462024416521331 ) ) ;
#20517=CARTESIAN_POINT ( 'NONE',  ( 788.6739635108323228, -415.6454272087885897, -373.9316612368139090 ) ) ;
#20519=CARTESIAN_POINT ( 'NONE',  ( 781.7834795799800531, -250.8164208402379245, -315.0636971347436202 ) ) ;
#20522=CARTESIAN_POINT ( 'NONE',  ( 805.2837595273609850, -266.7363362996981095, -340.5290396650784714 ) ) ;
#20523=CARTESIAN_POINT ( 'NONE',  ( 765.0180583372156207, -264.9982390220561115, -360.0135310231089534 ) ) ;
#20524=CARTESIAN_POINT ( 'NONE',  ( 755.3201227861273992, -435.7255117493282341, -345.3687786644892981 ) ) ;
#20525=CARTESIAN_POINT ( 'NONE',  ( 767.8955696845333705, -72.45278447660213317, -362.1676090361162323 ) ) ;
#20530=CARTESIAN_POINT ( 'NONE',  ( 754.3581564841646241, -41.46360902697149697, -316.1443688327762516 ) ) ;
#20532=CARTESIAN_POINT ( 'NONE',  ( 795.2725662613897839, 16.45630643248849267, -314.1785221222716586 ) ) ;
#20536=CARTESIAN_POINT ( 'NONE',  ( 800.9840315886518738, -28.91815448151699286, -354.1144889064786412 ) ) ;
#20537=CARTESIAN_POINT ( 'NONE',  ( 796.9462024416508257, -84.45278447660207632, -308.9653473494370246 ) ) ;
#20539=CARTESIAN_POINT ( 'NONE',  ( 797.8594530101008786, -445.5436935675098766, -322.1405469898980982 ) ) ;
#20540=CARTESIAN_POINT ( 'NONE',  ( 805.1927285166399315, -40.81642084023859951, -341.8018195045277707 ) ) ;
#20542=CARTESIAN_POINT ( 'NONE',  ( 796.7737145352015204, -188.6346026584199365, -370.7187646348536987 ) ) ;
#20544=CARTESIAN_POINT ( 'NONE',  ( 787.4999999999992042, -512.9681489794448908, -339.9999999999999432 ) ) ;
#20545=CARTESIAN_POINT ( 'NONE',  ( 744.8212110874229666, -258.8965053807777963, -336.2046728542121627 ) ) ;
#20547=CARTESIAN_POINT ( 'NONE',  ( 796.9462024416508257, -276.4527844766013800, -308.9653473494370246 ) ) ;
#20548=DIRECTION ( 'NONE',  ( -0.000000000000000000, -1.000000000000000000, -0.000000000000000000 ) ) ;
#20551=CARTESIAN_POINT ( 'NONE',  ( 808.7758568127978833, -28.16923265350574468, -320.0363995740631822 ) ) ;
#20552=CARTESIAN_POINT ( 'NONE',  ( 794.9819416627830151, -372.9982390220557704, -319.9864689768909898 ) ) ;
#20554=CARTESIAN_POINT ( 'NONE',  ( 773.7943932421234194, -47.80559628986931386, -305.5313806188329409 ) ) ;
#20555=CARTESIAN_POINT ( 'NONE',  ( 761.2382568024794409, -159.6237781080508285, -356.9571628226838129 ) ) ;
#20561=CARTESIAN_POINT ( 'NONE',  ( 788.8264449731200330, -69.18005720387488111, -363.6646147819171233 ) ) ;
#20562=CARTESIAN_POINT ( 'NONE',  ( 787.6308680596127942, -179.2601417444143692, -364.1105419155492768 ) ) ;
#20565=CARTESIAN_POINT ( 'NONE',  ( 751.2241431872005251, 7.830767346494148740, -359.9636004259367610 ) ) ;
#20569=CARTESIAN_POINT ( 'NONE',  ( 768.9521613784389729, -297.8272453906070041, -373.2346286133773106 ) ) ;
#20573=CARTESIAN_POINT ( 'NONE',  ( 773.4516893846965786, -163.6454272087893003, -315.8398074228977066 ) ) ;
#20574=CARTESIAN_POINT ( 'NONE',  ( 755.5713283507202505, -149.3618753856928265, -334.6858677611754729 ) ) ;
#20575=CARTESIAN_POINT ( 'NONE',  ( 778.2165204200184689, -310.8164208402377540, -364.9363028652563230 ) ) ;
#20583=CARTESIAN_POINT ( 'NONE',  ( 815.3608509340175488, -386.7363362996977116, -341.2497674668889545 ) ) ;
#20588=CARTESIAN_POINT ( 'NONE',  ( 755.5713283507202505, -341.3618753856922012, -334.6858677611754729 ) ) ;
#20589=CARTESIAN_POINT ( 'NONE',  ( 769.9779781133707957, -187.0999726633346825, -316.7813123517150871 ) ) ;
#20592=CARTESIAN_POINT ( 'NONE',  ( 767.7687537140311633, -407.9073299311465348, -372.7932403749916830 ) ) ;
#20597=CARTESIAN_POINT ( 'NONE',  ( 745.7998596910086917, -53.36187538569310362, -332.5602148656461168 ) ) ;
#20598=CARTESIAN_POINT ( 'NONE',  ( 804.4286716492782716, -257.3618753856924286, -345.3141322388244703 ) ) ;
#20602=CARTESIAN_POINT ( 'NONE',  ( 791.0478386215596629, -21.82724539060792424, -306.7653713866226326 ) ) ;
#20603=CARTESIAN_POINT ( 'NONE',  ( 780.5290396650775619, -60.35105083532383219, -365.2837595273619513 ) ) ;
#20610=CARTESIAN_POINT ( 'NONE',  ( 800.2193346964447755, -66.99823902205672255, -355.1360043628815788 ) ) ;
#20611=CARTESIAN_POINT ( 'NONE',  ( 799.4546378042377910, -369.0783235625956422, -356.1575198192848006 ) ) ;
#20614=CARTESIAN_POINT ( 'NONE',  ( 771.2368401574024119, -349.4419599262320162, -374.2805881961240857 ) ) ;
#20618=AXIS2_PLACEMENT_3D ( 'NONE', #20630, #13031, #34256 ) ;
#20620=CARTESIAN_POINT ( 'NONE',  ( 804.7487373415286811, -211.5436935675107861, -364.7487373415288516 ) ) ;
#20623=CARTESIAN_POINT ( 'NONE',  ( 794.9819416627830151, -204.9982390220562820, -319.9864689768909898 ) ) ;
#20624=EDGE_CURVE ( 'NONE', #38644, #38597, #8907, .T. ) ;
#20626=CARTESIAN_POINT ( 'NONE',  ( 771.1735550268778070, -369.1800572038739574, -316.3353852180827630 ) ) ;
#20627=CARTESIAN_POINT ( 'NONE',  ( 754.8072714833581358, -28.81642084023863148, -338.1981804954720587 ) ) ;
#20630=CARTESIAN_POINT ( 'NONE',  ( 779.9999999999992042, -462.9681489794448339, -339.9999999999999432 ) ) ;
#20632=CARTESIAN_POINT ( 'NONE',  ( 804.6971507214547046, -459.2817908451519884, -344.0799538623459739 ) ) ;
#20635=CARTESIAN_POINT ( 'NONE',  ( 807.2620300519052989, -288.0090635724252479, -318.0141637701419768 ) ) ;
#20638=CARTESIAN_POINT ( 'NONE',  ( 755.5713283507202505, -221.3618753856925707, -334.6858677611754729 ) ) ;
#20639=CARTESIAN_POINT ( 'NONE',  ( 765.8855110935204493, -406.1692326535045368, -319.0159684113471599 ) ) ;
#20642=CARTESIAN_POINT ( 'NONE',  ( 760.7433823573367135, -84.00906357242590161, -355.9930595647440441 ) ) ;
#20646=CARTESIAN_POINT ( 'NONE',  ( 756.1443688327750579, 2.376221891948710585, -314.3581564841659315 ) ) ;
#20647=CARTESIAN_POINT ( 'NONE',  ( 745.7998596910086917, -293.3618753856923718, -332.5602148656461168 ) ) ;
#20650=CARTESIAN_POINT ( 'NONE',  ( 797.6776695296629214, -91.54369356751116982, -357.6776695296636603 ) ) ;
#20652=CARTESIAN_POINT ( 'NONE',  ( 761.9338519418445230, -182.5328690171416497, -370.4231160770881957 ) ) ;
#20654=CARTESIAN_POINT ( 'NONE',  ( 767.7687537140311633, -407.9073299311465348, -372.7932403749916830 ) ) ;
#20658=CARTESIAN_POINT ( 'NONE',  ( 785.3141322388236176, -429.7255117493282910, -364.4286716492789537 ) ) ;
#20664=ADVANCED_FACE ( 'NONE', ( #27149 ), #9368, .F. ) ;
#20665=CARTESIAN_POINT ( 'NONE',  ( 776.9566956441375396, -252.8965053807777394, -364.8461984189686405 ) ) ;
#20667=CARTESIAN_POINT ( 'NONE',  ( 810.1134526219336749, -272.5328690171413086, -357.8822607201570349 ) ) ;
#20672=CARTESIAN_POINT ( 'NONE',  ( 799.4546378042377910, -33.07832356259662987, -356.1575198192848006 ) ) ;
#20673=CARTESIAN_POINT ( 'NONE',  ( 756.5762568750052424, -171.1800572038745543, -348.7366044899774238 ) ) ;
#20674=CARTESIAN_POINT ( 'NONE',  ( 755.0636971347428243, -196.2709662947835909, -341.7834795799807353 ) ) ;
#20677=CARTESIAN_POINT ( 'NONE',  ( 751.6929314249748586, -126.9982390220565094, -318.8095938919659034 ) ) ;
#20678=CARTESIAN_POINT ( 'NONE',  ( 795.1360043628808398, -116.0891481129656313, -360.2193346964456282 ) ) ;
#20680=CARTESIAN_POINT ( 'NONE',  ( 800.9840315886518738, -28.91815448151699286, -354.1144889064786412 ) ) ;
#20681=CARTESIAN_POINT ( 'NONE',  ( 775.8780910478218402, -393.2817908451522726, -364.9511171171680530 ) ) ;
#20688=CARTESIAN_POINT ( 'NONE',  ( 757.0176451133909268, -349.0999726633342561, -349.9200121543848354 ) ) ;
#20689=CARTESIAN_POINT ( 'NONE',  ( 756.3353852180819104, -341.9073299311465917, -331.1735550268788302 ) ) ;
#20690=CARTESIAN_POINT ( 'NONE',  ( 746.4236121716829757, -135.8272453906076009, -328.8385539511384650 ) ) ;
#20694=CARTESIAN_POINT ( 'NONE',  ( 769.1273215169530886, -286.7146871989594388, -317.4527132478988847 ) ) ;
#20696=CARTESIAN_POINT ( 'NONE',  ( 807.2620300519052989, -144.0090635724257027, -318.0141637701419768 ) ) ;
#20697=CARTESIAN_POINT ( 'NONE',  ( 799.9999999999993179, -512.9681489794448908, -339.9999999999999432 ) ) ;
#20701=CARTESIAN_POINT ( 'NONE',  ( 782.4968714119720516, -178.8164208402381519, -305.0891759886411023 ) ) ;
#20704=CARTESIAN_POINT ( 'NONE',  ( 772.5602148656447525, -297.7255117493286889, -305.7998596910095443 ) ) ;
#20710=CARTESIAN_POINT ( 'NONE',  ( 752.4576283171824116, -381.0783235625954717, -317.7880784355627952 ) ) ;
#20711=CARTESIAN_POINT ( 'NONE',  ( 801.1904061080336987, -140.0891481129654892, -368.3070685750235498 ) ) ;
#20713=CARTESIAN_POINT ( 'NONE',  ( 800.9747183278959710, -372.9982390220557704, -311.9810565676471583 ) ) ;
#20718=CARTESIAN_POINT ( 'NONE',  ( 813.2346286133761168, -149.2601417444144261, -328.9521613784389160 ) ) ;
#20725=EDGE_CURVE ( 'NONE', #3824, #17451, #5895, .T. ) ;
#20726=CARTESIAN_POINT ( 'NONE',  ( 810.7187646348534145, -18.45278447660230725, -356.7737145352016341 ) ) ;
#20729=CARTESIAN_POINT ( 'NONE',  ( 745.5313806188320314, -399.2817908451522726, -333.7943932421247268 ) ) ;
#20731=CARTESIAN_POINT ( 'NONE',  ( 764.8639956371174549, -272.0891481129651197, -319.7806653035542013 ) ) ;
#20735=CARTESIAN_POINT ( 'NONE',  ( 779.4763451958990572, -248.7363362996981380, -365.0264073115438919 ) ) ;
#20736=CARTESIAN_POINT ( 'NONE',  ( 778.2165204200184689, -262.8164208402379245, -364.9363028652563230 ) ) ;
#20738=CARTESIAN_POINT ( 'NONE',  ( 785.3141322388236176, -93.72551174932934259, -364.4286716492789537 ) ) ;
#20744=CARTESIAN_POINT ( 'NONE',  ( 815.3608509340175488, -50.73633629969874193, -341.2497674668889545 ) ) ;
#20751=CARTESIAN_POINT ( 'NONE',  ( 804.6971507214547046, -27.28179084515336328, -344.0799538623459739 ) ) ;
#20753=CARTESIAN_POINT ( 'NONE',  ( 804.7487373415286811, -67.54369356751125508, -364.7487373415288516 ) ) ;
#20755=CARTESIAN_POINT ( 'NONE',  ( 771.1735550268778070, -441.1800572038735027, -316.3353852180827630 ) ) ;
#20757=CARTESIAN_POINT ( 'NONE',  ( 812.7932403749906598, -207.1800572038744406, -327.7687537140311633 ) ) ;
#20760=DIRECTION ( 'NONE',  ( -0.000000000000000000, 1.000000000000000000, -1.056348263647623421E-15 ) ) ;
#20763=CARTESIAN_POINT ( 'NONE',  ( 776.2433038121456548, -276.8965053807776258, -374.8207195650711014 ) ) ;
#20766=CARTESIAN_POINT ( 'NONE',  ( 759.0252816721024374, -264.9982390220561115, -368.0189434323527280 ) ) ;
#20767=CARTESIAN_POINT ( 'NONE',  ( 758.7867965644026071, 16.45630643248849267, -318.7867965644036303 ) ) ;
#20770=CARTESIAN_POINT ( 'NONE',  ( 771.2633955100217236, -383.9073299311466485, -363.4237431249939618 ) ) ;
#20773=CARTESIAN_POINT ( 'NONE',  ( 744.8212110874229666, -66.89650538077835051, -336.2046728542121627 ) ) ;
#20774=CARTESIAN_POINT ( 'NONE',  ( 804.1601925771018387, -175.4419599262325562, -346.5483106153029098 ) ) ;
#20778=CARTESIAN_POINT ( 'NONE',  ( 800.2193346964447755, -66.99823902205672255, -355.1360043628815788 ) ) ;
#20779=CARTESIAN_POINT ( 'NONE',  ( 775.9200461376533440, -215.8055962898687881, -315.3028492785443291 ) ) ;
#20781=CARTESIAN_POINT ( 'NONE',  ( 801.9858362298568863, -3.078323562596726681, -312.7379699480935642 ) ) ;
#20786=CARTESIAN_POINT ( 'NONE',  ( 760.0363995740630116, -298.9181544815161828, -368.7758568127991907 ) ) ;
#20790=CARTESIAN_POINT ( 'NONE',  ( 755.3028492785439312, -135.2817908451530116, -335.9200461376539693 ) ) ;
#20791=CARTESIAN_POINT ( 'NONE',  ( 804.9363028652555840, -136.2709662947837330, -338.2165204200192079 ) ) ;
#20792=CARTESIAN_POINT ( 'NONE',  ( 788.7366044899766848, -323.9073299311468190, -316.5762568750059813 ) ) ;
#20798=ORIENTED_EDGE ( 'NONE', *, *, #13176, .F. ) ;
#20799=CARTESIAN_POINT ( 'NONE',  ( 778.7629533639073998, -368.7363362996977685, -375.0009284576466371 ) ) ;
#20803=CARTESIAN_POINT ( 'NONE',  ( 771.2633955100217236, -311.9073299311468759, -363.4237431249939618 ) ) ;
#20805=CARTESIAN_POINT ( 'NONE',  ( 790.9844846989617508, -214.3726999360618493, -317.2208543904092721 ) ) ;
#20810=CARTESIAN_POINT ( 'NONE',  ( 796.7737145352015204, -428.6346026584192259, -370.7187646348536987 ) ) ;
#20813=CARTESIAN_POINT ( 'NONE',  ( 794.9285562942586694, -457.5945560043289788, -366.0218793896430043 ) ) ;
#20815=CARTESIAN_POINT ( 'NONE',  ( 782.5225473063381969, -70.27096629478397460, -375.2698199232970637 ) ) ;
#20816=CARTESIAN_POINT ( 'NONE',  ( 781.8018195045266339, -286.2709662947833635, -365.1927285166406705 ) ) ;
#20820=CARTESIAN_POINT ( 'NONE',  ( 814.2805881961230625, -25.64542720878973014, -331.2368401574024119 ) ) ;
#20821=CARTESIAN_POINT ( 'NONE',  ( 759.2295555964440155, -40.16923265350570915, -353.9708237608231229 ) ) ;
#20827=CARTESIAN_POINT ( 'NONE',  ( 805.1016975059191054, -102.8965053807782368, -343.0745993439771837 ) ) ;
#20829=CARTESIAN_POINT ( 'NONE',  ( 785.3687786644884454, -59.36187538569306810, -315.3201227861279676 ) ) ;
#20830=CARTESIAN_POINT ( 'NONE',  ( 793.2243759319678702, -362.5328690171410813, -318.4439275373583200 ) ) ;
#20835=CARTESIAN_POINT ( 'NONE',  ( 803.8556311672234642, -393.6237781080500326, -365.6418435158340117 ) ) ;
#20841=CARTESIAN_POINT ( 'NONE',  ( 787.5162901302840055, -251.3618753856923149, -305.4481719005792684 ) ) ;
#20845=CARTESIAN_POINT ( 'NONE',  ( 788.7366044899766848, -227.9073299311471033, -316.5762568750059813 ) ) ;
#20847=CARTESIAN_POINT ( 'NONE',  ( 755.5713283507202505, -365.3618753856920875, -334.6858677611754729 ) ) ;
#20848=CARTESIAN_POINT ( 'NONE',  ( 774.6858677611749044, -9.725511749329603717, -315.5713283507209894 ) ) ;
#20853=CARTESIAN_POINT ( 'NONE',  ( 762.3223304703356007, 16.45630643248849267, -322.3223304703362828 ) ) ;
#20857=CARTESIAN_POINT ( 'NONE',  ( 771.3260364891663130, -283.6454272087889308, -306.0683387631859773 ) ) ;
#20860=CARTESIAN_POINT ( 'NONE',  ( 801.9419747391806368, -234.4527844766016358, -351.9812246680014027 ) ) ;
#20861=CARTESIAN_POINT ( 'NONE',  ( 801.3366627262608972, -392.5328690171409107, -353.0897708529566899 ) ) ;
#20862=DIRECTION ( 'NONE',  ( 0.000000000000000000, 0.000000000000000000, 1.000000000000000000 ) ) ;
#20864=CARTESIAN_POINT ( 'NONE',  ( 800.9840315886518738, -124.9181544815167086, -354.1144889064786412 ) ) ;
#20866=AXIS2_PLACEMENT_3D ( 'NONE', #19281, #29467, #18853 ) ;
#20868=CARTESIAN_POINT ( 'NONE',  ( 756.1443688327750579, 26.37622189194863509, -314.3581564841659315 ) ) ;
#20869=CARTESIAN_POINT ( 'NONE',  ( 815.2698199232962679, -328.8164208402375834, -342.5225473063383674 ) ) ;
#20872=CARTESIAN_POINT ( 'NONE',  ( 757.8323909638827445, -74.63460265842032015, -352.1044303154654358 ) ) ;
#20875=CARTESIAN_POINT ( 'NONE',  ( 815.0009284576459549, -198.3510508353234059, -338.7629533639073429 ) ) ;
#20877=CARTESIAN_POINT ( 'NONE',  ( 745.4481719005789273, -435.7255117493282341, -347.5162901302853129 ) ) ;
#20881=CARTESIAN_POINT ( 'NONE',  ( 759.9864689768902508, -410.0891481129647218, -354.9819416627836404 ) ) ;
#20888=CARTESIAN_POINT ( 'NONE',  ( 801.3366627262608972, -248.5328690171414223, -353.0897708529566899 ) ) ;
#20890=CARTESIAN_POINT ( 'NONE',  ( 773.7943932421234194, -287.8055962898685038, -305.5313806188329409 ) ) ;
#20895=CARTESIAN_POINT ( 'NONE',  ( 764.0069404352550464, -39.07832356259662276, -359.2566176426627180 ) ) ;
#20896=CARTESIAN_POINT ( 'NONE',  ( 755.3201227861273992, -147.7255117493291152, -345.3687786644892981 ) ) ;
#20897=CARTESIAN_POINT ( 'NONE',  ( 755.3201227861273992, -219.7255117493289447, -345.3687786644892981 ) ) ;
#20899=CARTESIAN_POINT ( 'NONE',  ( 763.2262854647970016, -104.6346026584202207, -309.2812353651462445 ) ) ;
#20901=CARTESIAN_POINT ( 'NONE',  ( 800.2193346964446619, -114.9982390220565378, -355.1360043628816925 ) ) ;
#20904=CARTESIAN_POINT ( 'NONE',  ( 755.8894580844503253, -399.8272453906067767, -332.3691319403863531 ) ) ;
#20912=CARTESIAN_POINT ( 'NONE',  ( 760.7433823573367135, -348.0090635724251342, -355.9930595647440441 ) ) ;
#20913=CARTESIAN_POINT ( 'NONE',  ( 801.9419747391806368, -354.4527844766012095, -351.9812246680014027 ) ) ;
#20914=CARTESIAN_POINT ( 'NONE',  ( 745.7194118038753459, -157.6454272087893287, -348.7631598425976449 ) ) ;
#20919=CARTESIAN_POINT ( 'NONE',  ( 773.3843516231979720, -301.4419599262320730, -364.4086373105754433 ) ) ;
#20920=CARTESIAN_POINT ( 'NONE',  ( 801.9419747391806368, -450.4527844766009821, -351.9812246680014027 ) ) ;
#20921=CARTESIAN_POINT ( 'NONE',  ( 771.3260364891663130, -139.6454272087893571, -306.0683387631859773 ) ) ;
#20926=CARTESIAN_POINT ( 'NONE',  ( 745.4481719005789273, -219.7255117493289447, -347.5162901302853697 ) ) ;
#20929=CARTESIAN_POINT ( 'NONE',  ( 745.7998596910086917, -341.3618753856922012, -332.5602148656461168 ) ) ;
#20938=CARTESIAN_POINT ( 'NONE',  ( 801.9858362298568863, -387.0783235625955285, -312.7379699480935642 ) ) ;
#20939=CARTESIAN_POINT ( 'NONE',  ( 813.1304606946830518, -113.9073299311474301, -352.3570229623690580 ) ) ;
#20940=CARTESIAN_POINT ( 'NONE',  ( 747.2067596250078623, -435.1800572038737869, -352.2312462859687230 ) ) ;
#20944=CARTESIAN_POINT ( 'NONE',  ( 766.5853460496234675, -157.9874144716871456, -372.3518521366060554 ) ) ;
#20952=CARTESIAN_POINT ( 'NONE',  ( 759.0252816721024374, -24.99823902205683268, -368.0189434323527280 ) ) ;
#20954=CARTESIAN_POINT ( 'NONE',  ( 779.9999999999992042, -462.9681489794448339, -339.9999999999999432 ) ) ;
#20955=CARTESIAN_POINT ( 'NONE',  ( 771.3260364891663130, -427.6454272087885897, -306.0683387631859773 ) ) ;
#20957=CARTESIAN_POINT ( 'NONE',  ( 758.0580252608178853, -270.4527844766014937, -328.0187753319985404 ) ) ;
#20962=CARTESIAN_POINT ( 'NONE',  ( 784.1219089521767955, -261.2817908451526705, -315.0488828828318333 ) ) ;
#20963=CARTESIAN_POINT ( 'NONE',  ( 774.6312213355099630, -239.3618753856924570, -364.6798772138717482 ) ) ;
#20966=CARTESIAN_POINT ( 'NONE',  ( 774.6312213355099630, -119.3618753856928691, -364.6798772138717482 ) ) ;
#20972=CARTESIAN_POINT ( 'NONE',  ( 783.7953271457878373, -32.19088175424425913, -375.1787889125761239 ) ) ;
#20979=CARTESIAN_POINT ( 'NONE',  ( 766.0291762391763086, -10.91815448151704793, -360.7704444035551319 ) ) ;
#20981=CARTESIAN_POINT ( 'NONE',  ( 812.7932403749906598, -63.18005720387488822, -327.7687537140311633 ) ) ;
#20984=AXIS2_PLACEMENT_3D ( 'NONE', #9426, #44769, #40835 ) ;
#20987=CARTESIAN_POINT ( 'NONE',  ( 812.7932403749906598, -183.1800572038744974, -327.7687537140311633 ) ) ;
#20993=CARTESIAN_POINT ( 'NONE',  ( 745.1769319972822814, -257.8055962898686744, -346.2694204179732083 ) ) ;
#20995=CARTESIAN_POINT ( 'NONE',  ( 755.2512626584698410, -295.5436935675105588, -315.2512626584710915 ) ) ;
#20999=CARTESIAN_POINT ( 'NONE',  ( 774.6312213355099630, -383.3618753856921444, -364.6798772138717482 ) ) ;
#21001=CARTESIAN_POINT ( 'NONE',  ( 771.2633955100217236, -191.9073299311471885, -363.4237431249939618 ) ) ;
#21003=CARTESIAN_POINT ( 'NONE',  ( 747.3154664389472828, -43.98741447168752217, -326.4474001241230781 ) ) ;
#21004=CARTESIAN_POINT ( 'NONE',  ( 805.1016975059191054, -174.8965053807779952, -343.0745993439771837 ) ) ;
#21011=CARTESIAN_POINT ( 'NONE',  ( 804.4286716492782716, -89.36187538569299704, -345.3141322388244703 ) ) ;
#21012=CARTESIAN_POINT ( 'NONE',  ( 805.1016975059191054, -198.8965053807779384, -343.0745993439771837 ) ) ;
#21014=CARTESIAN_POINT ( 'NONE',  ( 801.9858362298568863, -27.07832356259665474, -312.7379699480935642 ) ) ;
#21016=CARTESIAN_POINT ( 'NONE',  ( 767.9999999999992042, 178.9475563372491251, -320.0000000000000000 ) ) ;
#21019=CARTESIAN_POINT ( 'NONE',  ( 805.6418435158337843, -317.4636090269706301, -363.8556311672236916 ) ) ;
#21020=VECTOR ( 'NONE', #25994, 1000.000000000000000 ) ;
#21026=CARTESIAN_POINT ( 'NONE',  ( 783.0745993439762742, -152.1908817542438612, -365.1016975059196739 ) ) ;
#21027=CARTESIAN_POINT ( 'NONE',  ( 802.1676090361156639, -158.6346026584199933, -327.8955696845344505 ) ) ;
#21028=CARTESIAN_POINT ( 'NONE',  ( 791.9812246680005501, -356.6346026584193964, -361.9419747391813189 ) ) ;
#21029=ORIENTED_EDGE ( 'NONE', *, *, #28357, .F. ) ;
#21039=CARTESIAN_POINT ( 'NONE',  ( 809.0717654672305343, -364.9181544815158986, -360.1688906516309885 ) ) ;
#21045=CARTESIAN_POINT ( 'NONE',  ( 756.5762568750052424, -315.1800572038740711, -348.7366044899774238 ) ) ;
#21047=CARTESIAN_POINT ( 'NONE',  ( 804.8461984189677878, -218.1908817542437191, -336.9566956441385628 ) ) ;
#21054=CARTESIAN_POINT ( 'NONE',  ( 751.6929314249750860, -414.9982390220555430, -318.8095938919659034 ) ) ;
#21058=CARTESIAN_POINT ( 'NONE',  ( 798.6699377194444196, -457.0491014588743042, -363.8754770338464368 ) ) ;
#21060=CARTESIAN_POINT ( 'NONE',  ( 744.7301800767019131, -52.81642084023856398, -337.4774526936615757 ) ) ;
#21061=CARTESIAN_POINT ( 'NONE',  ( 797.6776695296629214, -283.5436935675105019, -357.6776695296636603 ) ) ;
#21066=CARTESIAN_POINT ( 'NONE',  ( 755.8990559732751535, -35.46360902697151829, -365.9055244015606831 ) ) ;
#21067=CARTESIAN_POINT ( 'NONE',  ( 756.7813123517142913, -91.98741447168737295, -329.9779781133712504 ) ) ;
#21073=CARTESIAN_POINT ( 'NONE',  ( 781.7834795799800531, -10.81642084023869543, -315.0636971347436202 ) ) ;
#21075=CARTESIAN_POINT ( 'NONE',  ( 765.0180583372156207, -48.99823902205675807, -360.0135310231089534 ) ) ;
#21076=CARTESIAN_POINT ( 'NONE',  ( 800.7704444035546203, -412.1692326535045936, -326.0291762391768771 ) ) ;
#21081=CARTESIAN_POINT ( 'NONE',  ( 815.1787889125755555, -390.8965053807772279, -343.7953271457877804 ) ) ;
#21087=ORIENTED_EDGE ( 'NONE', *, *, #9203, .F. ) ;
#21090=CARTESIAN_POINT ( 'NONE',  ( 767.7687537140311633, -239.9073299311470748, -372.7932403749916830 ) ) ;
#21092=ORIENTED_EDGE ( 'NONE', *, *, #33961, .T. ) ;
#21093=CARTESIAN_POINT ( 'NONE',  ( 795.1360043628808398, -236.0891481129652334, -360.2193346964456282 ) ) ;
#21095=CARTESIAN_POINT ( 'NONE',  ( 781.7834795799800531, -346.8164208402376971, -315.0636971347436202 ) ) ;
#21096=CARTESIAN_POINT ( 'NONE',  ( 802.1676090361156639, -14.63460265842049424, -327.8955696845344505 ) ) ;
#21097=VECTOR ( 'NONE', #22595, 1000.000000000000000 ) ;
#21101=PLANE ( 'NONE',  #20618 ) ;
#21104=VERTEX_POINT ( 'NONE', #13975 ) ;
#21105=CARTESIAN_POINT ( 'NONE',  ( 756.3353852180819104, -5.907329931147798696, -331.1735550268788302 ) ) ;
#21108=CARTESIAN_POINT ( 'NONE',  ( 804.1009440267234822, -263.4636090269708006, -314.0944755984392600 ) ) ;
#21111=CARTESIAN_POINT ( 'NONE',  ( 803.6646147819161570, -233.9073299311470180, -348.8264449731210561 ) ) ;
#21112=CARTESIAN_POINT ( 'NONE',  ( 770.0799878456142551, -397.9874144716864066, -362.9823548866085616 ) ) ;
#21114=CARTESIAN_POINT ( 'NONE',  ( 796.1575198192839480, -126.0090635724257737, -359.4546378042384163 ) ) ;
#21117=CARTESIAN_POINT ( 'NONE',  ( 796.7845633553578182, -441.6237781080499190, -358.5707757039688204 ) ) ;
#21118=CARTESIAN_POINT ( 'NONE',  ( 755.2512626584698410, -295.5436935675105588, -315.2512626584710915 ) ) ;
#21121=CARTESIAN_POINT ( 'NONE',  ( 778.2165204200184689, -70.81642084023850714, -364.9363028652563230 ) ) ;
#21123=CARTESIAN_POINT ( 'NONE',  ( 783.7566961878529810, -192.8965053807779668, -305.1792804349288417 ) ) ;
#21125=CARTESIAN_POINT ( 'NONE',  ( 787.4397851343537695, -429.7255117493282910, -374.2001403089903988 ) ) ;
#21130=CARTESIAN_POINT ( 'NONE',  ( 802.1676090361156639, -446.6346026584189985, -327.8955696845344505 ) ) ;
#21137=CARTESIAN_POINT ( 'NONE',  ( 798.7617431975189675, -243.6237781080504590, -323.0428371773161871 ) ) ;
#21139=CARTESIAN_POINT ( 'NONE',  ( 781.2497674668890113, -300.3510508353230080, -375.3608509340180603 ) ) ;
#21144=CARTESIAN_POINT ( 'NONE',  ( 755.8398074228967971, -43.44195992623296831, -333.4516893846970333 ) ) ;
#21145=CARTESIAN_POINT ( 'NONE',  ( 788.8264449731200330, -165.1800572038745258, -363.6646147819171233 ) ) ;
#21146=CARTESIAN_POINT ( 'NONE',  ( 774.6312213355099630, -191.3618753856925991, -364.6798772138717482 ) ) ;
#21148=CARTESIAN_POINT ( 'NONE',  ( 814.2001403089898304, -137.3618753856928265, -347.4397851343538264 ) ) ;
#21149=CARTESIAN_POINT ( 'NONE',  ( 754.8072714833583632, -100.8164208402383935, -338.1981804954721156 ) ) ;
#21151=CARTESIAN_POINT ( 'NONE',  ( 769.9779781133707957, -379.0999726633341993, -316.7813123517150871 ) ) ;
#21156=DIRECTION ( 'NONE',  ( -0.000000000000000000, 0.000000000000000000, -1.000000000000000000 ) ) ;
#21159=CARTESIAN_POINT ( 'NONE',  ( 786.5483106153019435, -367.6454272087886466, -364.1601925771022366 ) ) ;
#21160=CARTESIAN_POINT ( 'NONE',  ( 778.2165204200184689, -358.8164208402375834, -364.9363028652563230 ) ) ;
#21161=CARTESIAN_POINT ( 'NONE',  ( 804.1009440267234822, -167.4636090269711133, -314.0944755984392600 ) ) ;
#21167=CARTESIAN_POINT ( 'NONE',  ( 804.1601925771018387, -295.4419599262320730, -346.5483106153029098 ) ) ;
#21169=CARTESIAN_POINT ( 'NONE',  ( 757.7880784355613741, -162.0090635724256742, -312.4576283171834916 ) ) ;
#21175=CARTESIAN_POINT ( 'NONE',  ( 815.2698199232962679, -208.8164208402380666, -342.5225473063383674 ) ) ;
#21179=CARTESIAN_POINT ( 'NONE',  ( 808.7758568127978833, -100.1692326535055315, -320.0363995740631822 ) ) ;
#21181=CARTESIAN_POINT ( 'NONE',  ( 782.5225473063381969, -334.2709662947829656, -375.2698199232970637 ) ) ;
#21187=CARTESIAN_POINT ( 'NONE',  ( 811.6461892240364477, -412.7146871989590409, -324.1737431748509835 ) ) ;
#21188=CARTESIAN_POINT ( 'NONE',  ( 763.0537975583475827, -144.4527844766018632, -371.0346526505627480 ) ) ;
#21189=CARTESIAN_POINT ( 'NONE',  ( 777.4774526936600978, -418.2709662947827383, -304.7301800767027657 ) ) ;
#21194=CARTESIAN_POINT ( 'NONE',  ( 800.1688906516307043, -178.1692326535052473, -369.0717654672308186 ) ) ;
#21199=CARTESIAN_POINT ( 'NONE',  ( 787.5162901302840055, -35.36187538569316047, -305.4481719005792684 ) ) ;
#21202=CARTESIAN_POINT ( 'NONE',  ( 795.8262568251477660, -454.3726999360611103, -308.3538107759623585 ) ) ;
#21206=CARTESIAN_POINT ( 'NONE',  ( 758.0580252608178853, -246.4527844766016074, -328.0187753319985404 ) ) ;
#21210=CARTESIAN_POINT ( 'NONE',  ( 759.0159684113467620, -256.9181544815163534, -325.8855110935213020 ) ) ;
#21211=CARTESIAN_POINT ( 'NONE',  ( 762.1405469898971887, -241.5436935675106156, -357.8594530101015607 ) ) ;
#21213=CARTESIAN_POINT ( 'NONE',  ( 781.8018195045266339, -118.2709662947837899, -365.1927285166406705 ) ) ;
#21219=CARTESIAN_POINT ( 'NONE',  ( 745.7194118038753459, -37.64542720878968396, -348.7631598425976449 ) ) ;
#21225=CARTESIAN_POINT ( 'NONE',  ( 755.1538015810308480, -14.19088175424431242, -343.0433043558613804 ) ) ;
#21226=CARTESIAN_POINT ( 'NONE',  ( 772.4837098697145166, -95.36187538569296862, -374.5518280994205611 ) ) ;
#21231=CARTESIAN_POINT ( 'NONE',  ( 751.9810565676468741, -242.0891481129652618, -360.9747183278973921 ) ) ;
#21234=CARTESIAN_POINT ( 'NONE',  ( 745.1769319972822814, -281.8055962898686175, -346.2694204179732083 ) ) ;
#21236=CARTESIAN_POINT ( 'NONE',  ( 745.0891759886404770, -316.2709662947832499, -342.4968714119734159 ) ) ;
#21237=DIRECTION ( 'NONE',  ( 0.000000000000000000, -1.000000000000000000, 0.000000000000000000 ) ) ;
#21240=CARTESIAN_POINT ( 'NONE',  ( 768.0187753319979720, -392.6346026584193396, -318.0580252608186242 ) ) ;
#21242=CARTESIAN_POINT ( 'NONE',  ( 785.3687786644884454, -203.3618753856925991, -315.3201227861279676 ) ) ;
#21243=CARTESIAN_POINT ( 'NONE',  ( 793.4146539503750546, -73.98741447168741558, -307.6481478633938877 ) ) ;
#21248=CARTESIAN_POINT ( 'NONE',  ( 758.6633372737375112, -212.5328690171415076, -326.9102291470432533 ) ) ;
#21251=CARTESIAN_POINT ( 'NONE',  ( 808.7758568127978833, -28.16923265350574468, -320.0363995740631822 ) ) ;
#21256=CARTESIAN_POINT ( 'NONE',  ( 815.3608509340175488, -314.7363362996979959, -341.2497674668889545 ) ) ;
#21257=VECTOR ( 'NONE', #21477, 1000.000000000000000 ) ;
#21261=CARTESIAN_POINT ( 'NONE',  ( 757.4527132478984868, -160.3726999360620482, -329.1273215169538844 ) ) ;
#21262=CARTESIAN_POINT ( 'NONE',  ( 803.4237431249931660, -135.1800572038746679, -331.2633955100225194 ) ) ;
#21263=CARTESIAN_POINT ( 'NONE',  ( 778.2165204200184689, -334.8164208402376403, -364.9363028652563230 ) ) ;
#21272=CARTESIAN_POINT ( 'NONE',  ( 773.7305795820266212, -393.2817908451522726, -374.8230680027170365 ) ) ;
#21273=CARTESIAN_POINT ( 'NONE',  ( 814.2001403089898304, -17.36187538569322086, -347.4397851343538264 ) ) ;
#21277=CARTESIAN_POINT ( 'NONE',  ( 757.8323909638827445, -362.6346026584194533, -352.1044303154654358 ) ) ;
#21281=CARTESIAN_POINT ( 'NONE',  ( 773.4516893846965786, -235.6454272087890729, -315.8398074228977066 ) ) ;
#21285=CARTESIAN_POINT ( 'NONE',  ( 748.9653473494365699, -410.6346026584191691, -356.9462024416520762 ) ) ;
#21291=CARTESIAN_POINT ( 'NONE',  ( 751.6929314249748586, -54.99823902205672255, -318.8095938919659034 ) ) ;
#21292=CARTESIAN_POINT ( 'NONE',  ( 755.3201227861273992, -267.7255117493286320, -345.3687786644892981 ) ) ;
#21296=CARTESIAN_POINT ( 'NONE',  ( 809.0717654672305343, -28.91815448151699286, -360.1688906516309885 ) ) ;
#21297=CARTESIAN_POINT ( 'NONE',  ( 772.3691319403857278, -71.26014174441469606, -315.8894580844506663 ) ) ;
#21300=EDGE_CURVE ( 'NONE', #10014, #9510, #13649, .T. ) ;
#21302=CARTESIAN_POINT ( 'NONE',  ( 804.6798772138708955, 8.274488250670337663, -334.6312213355107019 ) ) ;
#21304=CARTESIAN_POINT ( 'NONE',  ( 797.6776695296629214, -91.54369356751116982, -357.6776695296636603 ) ) ;
#21306=CARTESIAN_POINT ( 'NONE',  ( 786.6156483768007774, -409.4419599262317320, -315.5913626894246136 ) ) ;
#21310=CARTESIAN_POINT ( 'NONE',  ( 815.0009284576459549, -390.3510508353227237, -338.7629533639073429 ) ) ;
#21317=CARTESIAN_POINT ( 'NONE',  ( 810.7187646348534145, -258.4527844766016074, -356.7737145352016341 ) ) ;
#21320=CARTESIAN_POINT ( 'NONE',  ( 788.8264449731201466, -237.1800572038742985, -363.6646147819170665 ) ) ;
#21323=CARTESIAN_POINT ( 'NONE',  ( 785.3687786644884454, -371.3618753856919739, -315.3201227861279676 ) ) ;
#21324=CARTESIAN_POINT ( 'NONE',  ( 788.7366044899766848, -11.90732993114778182, -316.5762568750059813 ) ) ;
#21329=CARTESIAN_POINT ( 'NONE',  ( 781.7834795799800531, -10.81642084023869543, -315.0636971347436202 ) ) ;
#21333=CARTESIAN_POINT ( 'NONE',  ( 781.2370466360911223, -260.7363362996981095, -304.9990715423533629 ) ) ;
#21336=CARTESIAN_POINT ( 'NONE',  ( 804.6798772138708955, -255.7255117493287742, -334.6312213355107019 ) ) ;
#21337=CARTESIAN_POINT ( 'NONE',  ( 793.2243759319678702, -410.5328690171408539, -318.4439275373583200 ) ) ;
#21340=CARTESIAN_POINT ( 'NONE',  ( 758.4439275373578084, -132.5545181178802920, -353.2243759319684386 ) ) ;
#21342=DIRECTION ( 'NONE',  ( -1.000000000000000000, -0.000000000000000000, -0.000000000000000000 ) ) ;
#21343=CARTESIAN_POINT ( 'NONE',  ( 766.5853460496234675, 10.01258552831232329, -372.3518521366060554 ) ) ;
#21344=CARTESIAN_POINT ( 'NONE',  ( 748.9653473494365699, -314.6346026584195101, -356.9462024416520762 ) ) ;
#21348=CARTESIAN_POINT ( 'NONE',  ( 813.9316612368132837, -199.4419599262324709, -348.6739635108323228 ) ) ;
#21350=CARTESIAN_POINT ( 'NONE',  ( 758.8095938919642549, -440.0891481129644944, -311.6929314249763365 ) ) ;
#21355=CARTESIAN_POINT ( 'NONE',  ( 770.0799878456142551, 10.01258552831232329, -362.9823548866085616 ) ) ;
#21356=AXIS2_PLACEMENT_3D ( 'NONE', #2861, #45599, #30570 ) ;
#21357=DIRECTION ( 'NONE',  ( -0.000000000000000000, 1.000000000000000000, -0.000000000000000000 ) ) ;
#21363=CARTESIAN_POINT ( 'NONE',  ( 797.8594530101008786, -37.54369356751132614, -322.1405469898980982 ) ) ;
#21365=CARTESIAN_POINT ( 'NONE',  ( 755.8398074228967971, -283.4419599262321867, -333.4516893846970333 ) ) ;
#21367=CARTESIAN_POINT ( 'NONE',  ( 815.1787889125755555, -294.8965053807775689, -343.7953271457877804 ) ) ;
#21368=DIRECTION ( 'NONE',  ( 0.000000000000000000, 0.000000000000000000, -1.000000000000000000 ) ) ;
#21372=CARTESIAN_POINT ( 'NONE',  ( 790.8726784830453198, -58.71468719896019905, -362.5472867521010585 ) ) ;
#21373=CARTESIAN_POINT ( 'NONE',  ( 788.7366044899766848, -155.9073299311473306, -316.5762568750059813 ) ) ;
#21374=CARTESIAN_POINT ( 'NONE',  ( 762.3223304703356007, -223.5436935675107577, -322.3223304703362828 ) ) ;
#21376=CARTESIAN_POINT ( 'NONE',  ( 763.0537975583475827, -144.4527844766018632, -371.0346526505627480 ) ) ;
#21380=CARTESIAN_POINT ( 'NONE',  ( 781.8018195045267476, -142.2709662947837330, -365.1927285166407273 ) ) ;
#21382=CARTESIAN_POINT ( 'NONE',  ( 755.5913626894240451, -397.6454272087885329, -346.6156483768012890 ) ) ;
#21389=EDGE_LOOP ( 'NONE', ( #3988, #41546, #26319, #22892, #9664, #36305 ) ) ;
#21390=CARTESIAN_POINT ( 'NONE',  ( 801.5560724626406000, -408.5545181178794110, -326.7756240680316182 ) ) ;
#21392=CARTESIAN_POINT ( 'NONE',  ( 773.7305795820266212, -177.2817908451528695, -374.8230680027170365 ) ) ;
#21397=CARTESIAN_POINT ( 'NONE',  ( 749.5768839229115201, -204.5545181178800931, -358.0661480581553064 ) ) ;
#21402=CARTESIAN_POINT ( 'NONE',  ( 755.2512626584698410, -199.5436935675108430, -315.2512626584710915 ) ) ;
#21406=CARTESIAN_POINT ( 'NONE',  ( 752.4576283171824116, -93.07832356259645223, -317.7880784355627952 ) ) ;
#21408=CARTESIAN_POINT ( 'NONE',  ( 808.0189434323515343, -326.0891481129649492, -319.0252816721025511 ) ) ;
#21409=CARTESIAN_POINT ( 'NONE',  ( 799.9999999999993179, -462.9681489794448339, -309.9999999999998863 ) ) ;
#21413=CARTESIAN_POINT ( 'NONE',  ( 747.3154664389472828, -427.9874144716862929, -326.4474001241230781 ) ) ;
#21414=CARTESIAN_POINT ( 'NONE',  ( 812.7932403749906598, -423.1800572038737300, -327.7687537140311633 ) ) ;
#21419=CARTESIAN_POINT ( 'NONE',  ( 812.6845335610512393, -199.9874144716870603, -353.5525998758768651 ) ) ;
#21423=ORIENTED_EDGE ( 'NONE', *, *, #24044, .T. ) ;
#21425=CARTESIAN_POINT ( 'NONE',  ( 804.7487373415286811, -43.54369356751131903, -364.7487373415288516 ) ) ;
#21428=CARTESIAN_POINT ( 'NONE',  ( 814.8207195650702488, -434.1908817542430370, -336.2433038121456548 ) ) ;
#21432=CARTESIAN_POINT ( 'NONE',  ( 805.1927285166397041, -280.8164208402378677, -341.8018195045277707 ) ) ;
#21436=CARTESIAN_POINT ( 'NONE',  ( 805.2837595273609850, -290.7363362996980527, -340.5290396650784714 ) ) ;
#21437=CARTESIAN_POINT ( 'NONE',  ( 785.3687786644884454, -251.3618753856923149, -315.3201227861279676 ) ) ;
#21439=CARTESIAN_POINT ( 'NONE',  ( 794.9819416627830151, -108.9982390220565804, -319.9864689768909898 ) ) ;
#21444=CARTESIAN_POINT ( 'NONE',  ( 750.9282345327678740, -64.91815448151686496, -319.8311093483690115 ) ) ;
#21449=ORIENTED_EDGE ( 'NONE', *, *, #17059, .F. ) ;
#21450=CARTESIAN_POINT ( 'NONE',  ( 773.4516893846965786, -43.64542720878966975, -315.8398074228977066 ) ) ;
#21451=CARTESIAN_POINT ( 'NONE',  ( 787.4397851343537695, -117.7255117493292715, -374.2001403089903988 ) ) ;
#21455=CARTESIAN_POINT ( 'NONE',  ( 747.2067596250078623, -243.1800572038743269, -352.2312462859687230 ) ) ;
#21459=CARTESIAN_POINT ( 'NONE',  ( 768.8385539511368734, -311.2601417444139429, -306.4236121716840557 ) ) ;
#21461=CARTESIAN_POINT ( 'NONE',  ( 810.7187646348534145, -330.4527844766013231, -356.7737145352016341 ) ) ;
#21465=CARTESIAN_POINT ( 'NONE',  ( 804.4286716492782716, -401.3618753856920307, -345.3141322388244703 ) ) ;
#21467=CARTESIAN_POINT ( 'NONE',  ( 759.8311093483677041, -70.16923265350563099, -310.9282345327691814 ) ) ;
#21471=CARTESIAN_POINT ( 'NONE',  ( 798.7617431975189675, -195.6237781080506863, -323.0428371773161871 ) ) ;
#21474=CARTESIAN_POINT ( 'NONE',  ( 812.6845335610512393, -31.98741447168754348, -353.5525998758768651 ) ) ;
#21476=CARTESIAN_POINT ( 'NONE',  ( 808.4681505782122031, -452.9681489794450613, -336.7690310503822388 ) ) ;
#21477=DIRECTION ( 'NONE',  ( -1.000000000000000000, -0.000000000000000000, -0.000000000000000000 ) ) ;
#21480=CARTESIAN_POINT ( 'NONE',  ( 797.8822607201568644, -342.5545181178796952, -370.1134526219340160 ) ) ;
#21484=CARTESIAN_POINT ( 'NONE',  ( 755.1538015810308480, -182.1908817542437760, -343.0433043558613804 ) ) ;
#21485=CARTESIAN_POINT ( 'NONE',  ( 785.3687786644884454, -155.3618753856927128, -315.3201227861279676 ) ) ;
#21486=CARTESIAN_POINT ( 'NONE',  ( 762.1405469898973024, -361.5436935675103882, -357.8594530101016176 ) ) ;
#21494=ORIENTED_EDGE ( 'NONE', *, *, #39098, .F. ) ;
#21495=CARTESIAN_POINT ( 'NONE',  ( 757.7880784355613741, -378.0090635724250774, -312.4576283171834916 ) ) ;
#21496=CARTESIAN_POINT ( 'NONE',  ( 767.7687537140311633, 0.09267006885218045942, -372.7932403749916830 ) ) ;
#21499=CARTESIAN_POINT ( 'NONE',  ( 804.4286716492782716, -353.3618753856922012, -345.3141322388244703 ) ) ;
#21501=DIRECTION ( 'NONE',  ( -0.000000000000000000, -0.000000000000000000, 1.000000000000000000 ) ) ;
#21502=CARTESIAN_POINT ( 'NONE',  ( 784.1219089521767955, -213.2817908451527842, -315.0488828828318333 ) ) ;
#21506=CARTESIAN_POINT ( 'NONE',  ( 805.0032342141413437, -421.5436935675101040, -314.9967657858572352 ) ) ;
#21511=CARTESIAN_POINT ( 'NONE',  ( 814.9108240113580450, -64.27096629478397460, -337.5031285880265273 ) ) ;
#21513=CARTESIAN_POINT ( 'NONE',  ( 762.1405469898971887, -289.5436935675103882, -357.8594530101015607 ) ) ;
#21519=CARTESIAN_POINT ( 'NONE',  ( 812.3518521366052028, -49.09997266333511590, -326.5853460496235243 ) ) ;
#21520=CARTESIAN_POINT ( 'NONE',  ( 784.0799538623451781, -83.80559628986920018, -364.6971507214555572 ) ) ;
#21524=CARTESIAN_POINT ( 'NONE',  ( 762.1405469898971887, -1.543693567511449150, -357.8594530101015607 ) ) ;
#21526=CARTESIAN_POINT ( 'NONE',  ( 755.3201227861273992, -99.72551174932928575, -345.3687786644892981 ) ) ;
#21527=CARTESIAN_POINT ( 'NONE',  ( 773.3843516231979720, -397.4419599262317320, -364.4086373105754433 ) ) ;
#21530=CARTESIAN_POINT ( 'NONE',  ( 768.8385539511368734, -407.2601417444137155, -306.4236121716840557 ) ) ;
#21535=CARTESIAN_POINT ( 'NONE',  ( 745.7998596910086917, -245.3618753856925139, -332.5602148656461168 ) ) ;
#21539=CARTESIAN_POINT ( 'NONE',  ( 798.5707757039680246, -53.46360902697146855, -356.7845633553585003 ) ) ;
#21540=CARTESIAN_POINT ( 'NONE',  ( 774.6312213355098493, -263.3618753856924286, -364.6798772138717482 ) ) ;
#21542=CARTESIAN_POINT ( 'NONE',  ( 774.6858677611749044, -345.7255117493285184, -315.5713283507209894 ) ) ;
#21543=CARTESIAN_POINT ( 'NONE',  ( 803.4237431249931660, -15.18005720387504631, -331.2633955100225194 ) ) ;
#21547=ORIENTED_EDGE ( 'NONE', *, *, #29090, .F. ) ;
#21548=CARTESIAN_POINT ( 'NONE',  ( 778.1981804954714335, -34.27096629478407408, -314.8072714833589885 ) ) ;
#21552=CARTESIAN_POINT ( 'NONE',  ( 776.2046728542105711, -284.1908817542434917, -304.8212110874238761 ) ) ;
#21556=CARTESIAN_POINT ( 'NONE',  ( 765.0180583372156207, -240.9982390220561683, -360.0135310231089534 ) ) ;
#21558=CARTESIAN_POINT ( 'NONE',  ( 796.1575198192839480, -102.0090635724258448, -359.4546378042384163 ) ) ;
#21559=EDGE_CURVE ( 'NONE', #25862, #5020, #22470, .T. ) ;
#21562=CARTESIAN_POINT ( 'NONE',  ( 758.0141637701419768, 8.921676437403235127, -367.2620300519063790 ) ) ;
#21563=CARTESIAN_POINT ( 'NONE',  ( 796.9462024416508257, -300.4527844766013231, -308.9653473494370246 ) ) ;
#21567=CARTESIAN_POINT ( 'NONE',  ( 803.8556311672234642, -201.6237781080506863, -365.6418435158340117 ) ) ;
#21569=CARTESIAN_POINT ( 'NONE',  ( 777.4774526936600978, -442.2709662947826814, -304.7301800767027657 ) ) ;
#21576=CARTESIAN_POINT ( 'NONE',  ( 803.4237431249931660, -447.1800572038736732, -331.2633955100225194 ) ) ;
#21582=CARTESIAN_POINT ( 'NONE',  ( 766.7756240680305382, -278.5328690171412518, -361.5560724626415663 ) ) ;
#21585=CARTESIAN_POINT ( 'NONE',  ( 756.1443688327750579, -309.6237781080502600, -314.3581564841659315 ) ) ;
#21588=ADVANCED_FACE ( 'NONE', ( #2425 ), #7857, .F. ) ;
#21592=CARTESIAN_POINT ( 'NONE',  ( 787.6308680596127942, -83.26014174441466764, -364.1105419155492768 ) ) ;
#21593=CARTESIAN_POINT ( 'NONE',  ( 800.0135310231082713, -158.0891481129655176, -325.0180583372163028 ) ) ;
#21594=CARTESIAN_POINT ( 'NONE',  ( 803.4237431249931660, -207.1800572038744406, -331.2633955100225194 ) ) ;
#21596=CARTESIAN_POINT ( 'NONE',  ( 777.5031285880264704, -142.8164208402382656, -374.9108240113588408 ) ) ;
#21599=CARTESIAN_POINT ( 'NONE',  ( 762.3223304703356007, -151.5436935675109851, -322.3223304703362828 ) ) ;
#21601=CARTESIAN_POINT ( 'NONE',  ( 763.8424801807145741, -378.0090635724250774, -320.5453621957614700 ) ) ;
#21608=CARTESIAN_POINT ( 'NONE',  ( 801.5560724626406000, -384.5545181178795247, -326.7756240680316182 ) ) ;
#21611=CARTESIAN_POINT ( 'NONE',  ( 748.6759233522253680, -184.3726999360619629, -324.3348316497537098 ) ) ;
#21616=CARTESIAN_POINT ( 'NONE',  ( 754.8983024940795303, -306.8965053807775689, -336.9254006560228163 ) ) ;
#21618=CARTESIAN_POINT ( 'NONE',  ( 750.9282345327678740, -184.9181544815165239, -319.8311093483690115 ) ) ;
#21624=CARTESIAN_POINT ( 'NONE',  ( 808.3070685750232087, -210.9982390220562252, -361.1904061080339829 ) ) ;
#21625=CARTESIAN_POINT ( 'NONE',  ( 799.9999999999993179, -462.9681489794448339, -309.9999999999998863 ) ) ;
#21626=CARTESIAN_POINT ( 'NONE',  ( 803.6646147819161570, 6.092670068852159559, -348.8264449731210561 ) ) ;
#21628=CARTESIAN_POINT ( 'NONE',  ( 795.6651683502461765, -82.71468719896012090, -371.3240766477733814 ) ) ;
#21630=CARTESIAN_POINT ( 'NONE',  ( 751.9810565676468741, -338.0891481129649492, -360.9747183278973921 ) ) ;
#21636=CARTESIAN_POINT ( 'NONE',  ( 763.2262854647970016, -416.6346026584192259, -309.2812353651462445 ) ) ;
#21642=CARTESIAN_POINT ( 'NONE',  ( 815.0009284576459549, -174.3510508353234627, -338.7629533639073429 ) ) ;
#21649=CARTESIAN_POINT ( 'NONE',  ( 808.3070685750230950, -42.99823902205675807, -361.1904061080339261 ) ) ;
#21652=CARTESIAN_POINT ( 'NONE',  ( 809.0717654672305343, -460.9181544815156713, -360.1688906516309885 ) ) ;
#21657=CARTESIAN_POINT ( 'NONE',  ( 781.7834795799800531, -298.8164208402377540, -315.0636971347436202 ) ) ;
#21661=CARTESIAN_POINT ( 'NONE',  ( 779.4763451958990572, -272.7363362996981095, -365.0264073115438919 ) ) ;
#21662=CARTESIAN_POINT ( 'NONE',  ( 778.1981804954714335, -274.2709662947833067, -314.8072714833589885 ) ) ;
#21664=CARTESIAN_POINT ( 'NONE',  ( 759.7806653035534055, -102.9982390220565520, -324.8639956371180801 ) ) ;
#21668=CARTESIAN_POINT ( 'NONE',  ( 764.1737431748507561, -82.37269993606227558, -371.6461892240376415 ) ) ;
#21674=CARTESIAN_POINT ( 'NONE',  ( 755.8894580844503253, -39.82724539060786384, -332.3691319403863531 ) ) ;
#21677=CARTESIAN_POINT ( 'NONE',  ( 792.3570229623691148, -93.18005720387479585, -373.1304606946836770 ) ) ;
#21681=CARTESIAN_POINT ( 'NONE',  ( 748.9653473494363425, -218.6346026584197944, -356.9462024416521331 ) ) ;
#21684=CARTESIAN_POINT ( 'NONE',  ( 746.0683387631852383, -307.4419599262320730, -331.3260364891676204 ) ) ;
#21687=CARTESIAN_POINT ( 'NONE',  ( 782.4968714119720516, -322.8164208402377540, -305.0891759886411023 ) ) ;
#21691=CARTESIAN_POINT ( 'NONE',  ( 778.1981804954714335, -418.2709662947827383, -314.8072714833589885 ) ) ;
#21693=CARTESIAN_POINT ( 'NONE',  ( 752.4576283171824116, -69.07832356259653750, -317.7880784355627952 ) ) ;
#21697=CARTESIAN_POINT ( 'NONE',  ( 800.7704444035546203, -196.1692326535052473, -326.0291762391768771 ) ) ;
#21699=CARTESIAN_POINT ( 'NONE',  ( 800.1688906516307043, -34.16923265350572336, -369.0717654672308186 ) ) ;
#21702=CARTESIAN_POINT ( 'NONE',  ( 798.5757817331792694, -452.9681489794448339, -357.1584183591081683 ) ) ;
#21707=CARTESIAN_POINT ( 'NONE',  ( 747.6481478633932056, -349.0999726633342561, -353.4146539503763620 ) ) ;
#21710=CARTESIAN_POINT ( 'NONE',  ( 798.5707757039680246, -197.4636090269709996, -356.7845633553585003 ) ) ;
#21711=CARTESIAN_POINT ( 'NONE',  ( 804.9363028652555840, -184.2709662947835909, -338.2165204200192079 ) ) ;
#21712=CARTESIAN_POINT ( 'NONE',  ( 759.7806653035535192, -342.9982390220557704, -324.8639956371181370 ) ) ;
#21713=VERTEX_POINT ( 'NONE', #43772 ) ;
#21714=CARTESIAN_POINT ( 'NONE',  ( 757.2208543904082489, 7.285312801039605546, -350.9844846989624330 ) ) ;
#21724=CARTESIAN_POINT ( 'NONE',  ( 752.7379699480933368, -396.0090635724249637, -361.9858362298580232 ) ) ;
#21725=CARTESIAN_POINT ( 'NONE',  ( 755.2512626584698410, -7.543693567511430942, -315.2512626584710915 ) ) ;
#21728=CARTESIAN_POINT ( 'NONE',  ( 788.7366044899766848, -371.9073299311465917, -316.5762568750059813 ) ) ;
#21731=CARTESIAN_POINT ( 'NONE',  ( 801.5560724626406000, -216.5545181178800931, -326.7756240680316182 ) ) ;
#21734=LINE ( 'NONE', #264, #26904 ) ;
#21741=CARTESIAN_POINT ( 'NONE',  ( 747.2067596250078623, -99.18005720387478164, -352.2312462859687230 ) ) ;
#21742=CARTESIAN_POINT ( 'NONE',  ( 791.9812246680005501, -284.6346026584196807, -361.9419747391813189 ) ) ;
#21747=CARTESIAN_POINT ( 'NONE',  ( 814.8207195650702488, -50.19088175424420939, -336.2433038121456548 ) ) ;
#21748=CARTESIAN_POINT ( 'NONE',  ( 769.1273215169530886, -94.71468719896007826, -317.4527132478988847 ) ) ;
#21753=CARTESIAN_POINT ( 'NONE',  ( 756.3353852180819104, -5.907329931147798696, -331.1735550268788302 ) ) ;
#21755=CARTESIAN_POINT ( 'NONE',  ( 788.8264449731200330, -93.18005720387481006, -363.6646147819171233 ) ) ;
#21758=CARTESIAN_POINT ( 'NONE',  ( 766.7756240680305382, -398.5328690171409107, -361.5560724626415663 ) ) ;
#21761=CARTESIAN_POINT ( 'NONE',  ( 798.0661480581538854, -410.5328690171408539, -309.5768839229118043 ) ) ;
#21763=ORIENTED_EDGE ( 'NONE', *, *, #33741, .F. ) ;
#21766=CARTESIAN_POINT ( 'NONE',  ( 808.0189434323515343, -254.0891481129652334, -319.0252816721025511 ) ) ;
#21770=ORIENTED_EDGE ( 'NONE', *, *, #17335, .T. ) ;
#21771=CARTESIAN_POINT ( 'NONE',  ( 776.9254006560222479, -68.19088175424413123, -314.8983024940802125 ) ) ;
#21772=CARTESIAN_POINT ( 'NONE',  ( 803.6646147819162707, -233.9073299311470464, -348.8264449731211130 ) ) ;
#21775=CARTESIAN_POINT ( 'NONE',  ( 797.6776695296629214, -379.5436935675102745, -357.6776695296636603 ) ) ;
#21776=CARTESIAN_POINT ( 'NONE',  ( 774.6858677611749044, -57.72551174932945628, -315.5713283507209894 ) ) ;
#21781=CARTESIAN_POINT ( 'NONE',  ( 771.2633955100217236, -23.90732993114773919, -363.4237431249939618 ) ) ;
#21785=CARTESIAN_POINT ( 'NONE',  ( 766.4474001241216001, -307.0999726633343130, -307.3154664389482491 ) ) ;
#21789=CARTESIAN_POINT ( 'NONE',  ( 755.0636971347428243, -244.2709662947834204, -341.7834795799807353 ) ) ;
#21791=CARTESIAN_POINT ( 'NONE',  ( 776.9254006560222479, -116.1908817542440033, -314.8983024940802125 ) ) ;
#21794=CARTESIAN_POINT ( 'NONE',  ( 746.0683387631852383, -19.44195992623303937, -331.3260364891676204 ) ) ;
#21795=CARTESIAN_POINT ( 'NONE',  ( 767.6429770376291799, -297.1800572038741279, -306.8695393053162093 ) ) ;
#21799=CARTESIAN_POINT ( 'NONE',  ( 768.8385539511368734, -215.2601417444141987, -306.4236121716840557 ) ) ;
#21801=CARTESIAN_POINT ( 'NONE',  ( 804.7487373415286811, -451.5436935675099903, -364.7487373415288516 ) ) ;
#21805=CARTESIAN_POINT ( 'NONE',  ( 795.9930595647434757, 20.92167643740319605, -320.7433823573372820 ) ) ;
#21807=PLANE ( 'NONE',  #401 ) ;
#21813=CARTESIAN_POINT ( 'NONE',  ( 759.2295555964440155, -280.1692326535049347, -353.9708237608231229 ) ) ;
#21816=CARTESIAN_POINT ( 'NONE',  ( 778.7502325331095108, -288.3510508353231216, -304.6391490659818828 ) ) ;
#21821=CARTESIAN_POINT ( 'NONE',  ( 761.2382568024794409, -87.62377810805102740, -356.9571628226838129 ) ) ;
#21825=CARTESIAN_POINT ( 'NONE',  ( 814.9108240113580450, -160.2709662947836762, -337.5031285880265273 ) ) ;
#21826=ORIENTED_EDGE ( 'NONE', *, *, #14121, .T. ) ;
#21827=CARTESIAN_POINT ( 'NONE',  ( 788.7366044899766848, -131.9073299311473875, -316.5762568750059813 ) ) ;
#21829=CARTESIAN_POINT ( 'NONE',  ( 800.9840315886518738, -412.9181544815157281, -354.1144889064786412 ) ) ;
#21838=CARTESIAN_POINT ( 'NONE',  ( 790.9844846989617508, -382.3726999360613945, -317.2208543904092721 ) ) ;
#21839=DIRECTION ( 'NONE',  ( -1.000000000000000000, 0.000000000000000000, 0.000000000000000000 ) ) ;
#21840=CARTESIAN_POINT ( 'NONE',  ( 760.0363995740630116, -178.9181544815165239, -368.7758568127991907 ) ) ;
#21845=CARTESIAN_POINT ( 'NONE',  ( 803.8651313633788504, -317.2601417444139429, -332.4468031744301015 ) ) ;
#21846=FACE_OUTER_BOUND ( 'NONE', #34442, .T. ) ;
#21847=CARTESIAN_POINT ( 'NONE',  ( 793.5525998758768083, -175.0999726633346825, -372.6845335610516941 ) ) ;
#21854=CARTESIAN_POINT ( 'NONE',  ( 746.8695393053151292, -221.9073299311471033, -327.6429770376306578 ) ) ;
#21857=CARTESIAN_POINT ( 'NONE',  ( 759.9864689768902508, -2.089148112965993231, -354.9819416627836404 ) ) ;
#21861=CARTESIAN_POINT ( 'NONE',  ( 744.9990715423526808, -90.35105083532373271, -341.2370466360926002 ) ) ;
#21863=CARTESIAN_POINT ( 'NONE',  ( 777.4774526936600978, -346.2709662947830793, -304.7301800767027657 ) ) ;
#21870=CARTESIAN_POINT ( 'NONE',  ( 788.7631598425961101, -409.4419599262317320, -305.7194118038759143 ) ) ;
#21871=CARTESIAN_POINT ( 'NONE',  ( 767.6429770376289525, -417.1800572038736163, -306.8695393053162093 ) ) ;
#21875=CARTESIAN_POINT ( 'NONE',  ( 786.6156483768007774, -193.4419599262325278, -315.5913626894246136 ) ) ;
#21877=CARTESIAN_POINT ( 'NONE',  ( 813.9316612368132837, -175.4419599262325562, -348.6739635108323228 ) ) ;
#21887=CARTESIAN_POINT ( 'NONE',  ( 814.5518280994195948, -39.72551174932951312, -332.4837098697145734 ) ) ;
#21891=CARTESIAN_POINT ( 'NONE',  ( 745.1792804349281596, -446.1908817542429802, -343.7566961878542884 ) ) ;
#21903=CARTESIAN_POINT ( 'NONE',  ( 755.8894580844503253, -279.8272453906071746, -332.3691319403863531 ) ) ;
#21904=CARTESIAN_POINT ( 'NONE',  ( 785.3141322388236176, -285.7255117493286889, -364.4286716492789537 ) ) ;
#21905=CARTESIAN_POINT ( 'NONE',  ( 797.6776695296629214, -115.5436935675110988, -357.6776695296636603 ) ) ;
#21911=CARTESIAN_POINT ( 'NONE',  ( 745.7194118038753459, -85.64542720878952764, -348.7631598425976449 ) ) ;
#21917=CARTESIAN_POINT ( 'NONE',  ( 796.9462024416508257, -108.4527844766020053, -308.9653473494370246 ) ) ;
#21923=CARTESIAN_POINT ( 'NONE',  ( 745.7998596910086917, -245.3618753856925139, -332.5602148656461168 ) ) ;
#21928=CARTESIAN_POINT ( 'NONE',  ( 791.1614460488616487, -299.2601417444139997, -373.5763878283158874 ) ) ;
#21931=CARTESIAN_POINT ( 'NONE',  ( 772.5602148656447525, -321.7255117493286320, -305.7998596910095443 ) ) ;
#21936=CARTESIAN_POINT ( 'NONE',  ( 800.2193346964447755, -426.9982390220554862, -355.1360043628815788 ) ) ;
#21939=CARTESIAN_POINT ( 'NONE',  ( 764.3348316497523456, -70.71468719896014932, -308.6759233522265617 ) ) ;
#21944=CARTESIAN_POINT ( 'NONE',  ( 799.4546378042377910, -249.0783235625959549, -356.1575198192848006 ) ) ;
#21947=CARTESIAN_POINT ( 'NONE',  ( 766.5853460496234675, -37.98741447168752927, -372.3518521366060554 ) ) ;
#21949=CARTESIAN_POINT ( 'NONE',  ( 807.9206849184947714, -452.9681489794447202, -338.7201299304387021 ) ) ;
#21952=CARTESIAN_POINT ( 'NONE',  ( 745.1792804349281596, -326.1908817542433781, -343.7566961878542884 ) ) ;
#21955=CARTESIAN_POINT ( 'NONE',  ( 796.9571628226829034, -191.4636090269709996, -321.2382568024804641 ) ) ;
#21956=CARTESIAN_POINT ( 'NONE',  ( 774.6312213355099630, -191.3618753856925991, -364.6798772138717482 ) ) ;
#21957=CARTESIAN_POINT ( 'NONE',  ( 788.7366044899766848, -347.9073299311467053, -316.5762568750059813 ) ) ;
#21959=CARTESIAN_POINT ( 'NONE',  ( 793.2243759319678702, 21.46713098285774279, -318.4439275373583200 ) ) ;
#21968=CARTESIAN_POINT ( 'NONE',  ( 799.9636004259356241, -406.9181544815157849, -311.2241431872006956 ) ) ;
#21969=CARTESIAN_POINT ( 'NONE',  ( 763.2262854647970016, -8.634602658420517329, -309.2812353651462445 ) ) ;
#21972=CARTESIAN_POINT ( 'NONE',  ( 781.7834795799800531, -370.8164208402375834, -315.0636971347436202 ) ) ;
#21975=CARTESIAN_POINT ( 'NONE',  ( 773.4516893846965786, -259.6454272087890445, -315.8398074228977066 ) ) ;
#21982=CARTESIAN_POINT ( 'NONE',  ( 781.8018195045266339, -334.2709662947829656, -365.1927285166406705 ) ) ;
#21986=CARTESIAN_POINT ( 'NONE',  ( 750.9282345327678740, -64.91815448151686496, -319.8311093483690115 ) ) ;
#21987=CARTESIAN_POINT ( 'NONE',  ( 804.9511171171677688, -125.8055962898690581, -335.8780910478229202 ) ) ;
#21992=CARTESIAN_POINT ( 'NONE',  ( 756.7813123517142913, -139.9874144716872024, -329.9779781133712504 ) ) ;
#21993=ORIENTED_EDGE ( 'NONE', *, *, #26982, .T. ) ;
#21994=CARTESIAN_POINT ( 'NONE',  ( 797.8594530101008786, -109.5436935675110988, -322.1405469898980982 ) ) ;
#21995=CARTESIAN_POINT ( 'NONE',  ( 779.4709603349208464, -384.3510508353227806, -314.7162404726379918 ) ) ;
#22005=CARTESIAN_POINT ( 'NONE',  ( 784.1219089521767955, -69.28179084515321051, -315.0488828828318333 ) ) ;
#22007=CARTESIAN_POINT ( 'NONE',  ( 781.8018195045267476, -238.2709662947833920, -365.1927285166407273 ) ) ;
#22009=CARTESIAN_POINT ( 'NONE',  ( 755.0636971347428243, -388.2709662947829656, -341.7834795799807353 ) ) ;
#22010=CARTESIAN_POINT ( 'NONE',  ( 764.8639956371174549, -56.08914811296580893, -319.7806653035542013 ) ) ;
#22014=CARTESIAN_POINT ( 'NONE',  ( 765.0180583372156207, -0.9982390220569063999, -360.0135310231089534 ) ) ;
#22017=CARTESIAN_POINT ( 'NONE',  ( 757.7880784355613741, -306.0090635724252479, -312.4576283171834916 ) ) ;
#22021=CARTESIAN_POINT ( 'NONE',  ( 797.8594530101008786, -253.5436935675104735, -322.1405469898980982 ) ) ;
#22023=CARTESIAN_POINT ( 'NONE',  ( 780.5236548040995785, -164.7363362996983938, -314.9735926884559944 ) ) ;
#22026=CARTESIAN_POINT ( 'NONE',  ( 749.8865473780648472, -20.53286901714212931, -322.1177392798429082 ) ) ;
#22027=CARTESIAN_POINT ( 'NONE',  ( 814.5518280994195948, -351.7255117493284615, -332.4837098697145166 ) ) ;
#22031=CARTESIAN_POINT ( 'NONE',  ( 778.7502325331095108, -240.3510508353232069, -304.6391490659818828 ) ) ;
#22033=CARTESIAN_POINT ( 'NONE',  ( 764.3348316497523456, -430.7146871989590409, -308.6759233522265617 ) ) ;
#22034=CARTESIAN_POINT ( 'NONE',  ( 779.9999999999992042, 16.45630643248849267, -339.9999999999999432 ) ) ;
#22038=CARTESIAN_POINT ( 'NONE',  ( 786.6156483768007774, 22.55804007376682918, -315.5913626894246136 ) ) ;
#22044=CARTESIAN_POINT ( 'NONE',  ( 793.2243759319678702, -290.5328690171412518, -318.4439275373583200 ) ) ;
#22046=EDGE_CURVE ( 'NONE', #22721, #2036, #37987, .T. ) ;
#22047=CARTESIAN_POINT ( 'NONE',  ( 801.9858362298568863, -339.0783235625956422, -312.7379699480935642 ) ) ;
#22053=CARTESIAN_POINT ( 'NONE',  ( 757.2208543904082489, -88.71468719896009247, -350.9844846989624330 ) ) ;
#22055=CARTESIAN_POINT ( 'NONE',  ( 754.9967657858570647, -145.5436935675109851, -365.0032342141425374 ) ) ;
#22057=CARTESIAN_POINT ( 'NONE',  ( 762.3223304703356007, -127.5436935675110561, -322.3223304703362828 ) ) ;
#22059=CARTESIAN_POINT ( 'NONE',  ( 776.9254006560222479, -428.1908817542430938, -314.8983024940802125 ) ) ;
#22067=CARTESIAN_POINT ( 'NONE',  ( 790.9844846989617508, -406.3726999360612808, -317.2208543904092721 ) ) ;
#22069=CARTESIAN_POINT ( 'NONE',  ( 810.4231160770870019, -216.5545181178800931, -321.9338519418446936 ) ) ;
#22073=CARTESIAN_POINT ( 'NONE',  ( 760.5453621957607311, -333.0783235625956991, -323.8424801807151425 ) ) ;
#22075=CARTESIAN_POINT ( 'NONE',  ( 815.3608509340175488, -194.7363362996982517, -341.2497674668889545 ) ) ;
#22080=CARTESIAN_POINT ( 'NONE',  ( 804.7487373415286811, -235.5436935675107293, -364.7487373415288516 ) ) ;
#22082=CARTESIAN_POINT ( 'NONE',  ( 805.1927285166397041, -16.81642084023866701, -341.8018195045277707 ) ) ;
#22085=CARTESIAN_POINT ( 'NONE',  ( 758.0141637701419768, -87.07832356259646645, -367.2620300519063790 ) ) ;
#22087=CARTESIAN_POINT ( 'NONE',  ( 746.8695393053150156, -389.9073299311465348, -327.6429770376306010 ) ) ;
#22089=DIRECTION ( 'NONE',  ( 0.7071067811865753283, 0.000000000000000000, -0.7071067811865198172 ) ) ;
#22092=CARTESIAN_POINT ( 'NONE',  ( 754.0944755984390895, -423.6237781080499190, -364.1009440267246760 ) ) ;
#22093=CARTESIAN_POINT ( 'NONE',  ( 813.5763878283155464, -3.827245390607979303, -351.1614460488615350 ) ) ;
#22097=CARTESIAN_POINT ( 'NONE',  ( 758.6633372737375112, -188.5328690171416497, -326.9102291470432533 ) ) ;
#22099=CARTESIAN_POINT ( 'NONE',  ( 814.8230680027162407, -173.8055962898689302, -333.7305795820267917 ) ) ;
#22104=CARTESIAN_POINT ( 'NONE',  ( 764.8639956371174549, -152.0891481129655460, -319.7806653035542013 ) ) ;
#22106=CARTESIAN_POINT ( 'NONE',  ( 751.9810565676468741, -26.08914811296592262, -360.9747183278973921 ) ) ;
#22108=CARTESIAN_POINT ( 'NONE',  ( 750.9282345327678740, -448.9181544815156144, -319.8311093483690115 ) ) ;
#22110=CARTESIAN_POINT ( 'NONE',  ( 784.1219089521767955, -309.2817908451525568, -315.0488828828318333 ) ) ;
#22113=CARTESIAN_POINT ( 'NONE',  ( 801.9419747391806368, -306.4527844766013800, -351.9812246680014027 ) ) ;
#22117=CARTESIAN_POINT ( 'NONE',  ( 776.9254006560222479, -284.1908817542434917, -314.8983024940802125 ) ) ;
#22118=CARTESIAN_POINT ( 'NONE',  ( 755.3201227861273992, -291.7255117493285752, -345.3687786644892981 ) ) ;
#22120=CARTESIAN_POINT ( 'NONE',  ( 804.4286716492782716, -161.3618753856927697, -345.3141322388244703 ) ) ;
#22126=CARTESIAN_POINT ( 'NONE',  ( 748.6759233522253680, -88.37269993606226137, -324.3348316497537098 ) ) ;
#22132=CARTESIAN_POINT ( 'NONE',  ( 808.0189434323515343, -110.0891481129656597, -319.0252816721025511 ) ) ;
#22137=CARTESIAN_POINT ( 'NONE',  ( 767.6429770376289525, -249.1800572038742416, -306.8695393053162093 ) ) ;
#22138=EDGE_CURVE ( 'NONE', #18205, #38597, #41242, .T. ) ;
#22141=CARTESIAN_POINT ( 'NONE',  ( 813.2346286133761168, -317.2601417444139429, -328.9521613784389160 ) ) ;
#22143=CARTESIAN_POINT ( 'NONE',  ( 814.2001403089898304, -329.3618753856922581, -347.4397851343538264 ) ) ;
#22147=CARTESIAN_POINT ( 'NONE',  ( 762.1405469898971887, -409.5436935675101040, -357.8594530101015607 ) ) ;
#22149=CARTESIAN_POINT ( 'NONE',  ( 797.6776695296629214, -211.5436935675107861, -357.6776695296636603 ) ) ;
#22150=CARTESIAN_POINT ( 'NONE',  ( 815.1787889125755555, -78.89650538077832209, -343.7953271457877804 ) ) ;
#22154=ORIENTED_EDGE ( 'NONE', *, *, #18208, .F. ) ;
#22155=CARTESIAN_POINT ( 'NONE',  ( 764.0069404352550464, -231.0783235625960401, -359.2566176426627180 ) ) ;
#22157=CARTESIAN_POINT ( 'NONE',  ( 813.9316612368132837, -79.44195992623286884, -348.6739635108323228 ) ) ;
#22158=CARTESIAN_POINT ( 'NONE',  ( 796.3364271039121149, -452.9681489794448339, -359.1033184105688747 ) ) ;
#22161=CARTESIAN_POINT ( 'NONE',  ( 781.2370466360911223, -332.7363362996979390, -304.9990715423533629 ) ) ;
#22165=CARTESIAN_POINT ( 'NONE',  ( 805.2837595273609850, -170.7363362996983938, -340.5290396650784714 ) ) ;
#22166=CARTESIAN_POINT ( 'NONE',  ( 767.8955696845333705, -168.4527844766018347, -362.1676090361162323 ) ) ;
#22167=CARTESIAN_POINT ( 'NONE',  ( 788.7366044899766848, -371.9073299311465917, -316.5762568750059813 ) ) ;
#22168=ORIENTED_EDGE ( 'NONE', *, *, #11776, .F. ) ;
#22177=CARTESIAN_POINT ( 'NONE',  ( 811.3240766477731540, -412.3726999360612808, -355.6651683502462902 ) ) ;
#22179=CARTESIAN_POINT ( 'NONE',  ( 796.7737145352015204, 3.365397341579444479, -370.7187646348536987 ) ) ;
#22182=CARTESIAN_POINT ( 'NONE',  ( 785.3141322388236176, -405.7255117493283478, -364.4286716492789537 ) ) ;
#22187=CARTESIAN_POINT ( 'NONE',  ( 799.2566176426618085, -240.0090635724253900, -324.0069404352559559 ) ) ;
#22197=CARTESIAN_POINT ( 'NONE',  ( 791.9812246680005501, -308.6346026584195670, -361.9419747391813189 ) ) ;
#22201=CARTESIAN_POINT ( 'NONE',  ( 762.1177392798416577, -66.55451811788050520, -309.8865473780659272 ) ) ;
#22202=CARTESIAN_POINT ( 'NONE',  ( 757.2208543904082489, -136.7146871989600072, -350.9844846989624330 ) ) ;
#22205=CARTESIAN_POINT ( 'NONE',  ( 803.6646147819161570, -41.90732993114767169, -348.8264449731210561 ) ) ;
#22206=CARTESIAN_POINT ( 'NONE',  ( 773.3843516231979720, -133.4419599262326699, -364.4086373105754433 ) ) ;
#22207=CARTESIAN_POINT ( 'NONE',  ( 797.8594530101008786, -85.54369356751118403, -322.1405469898980982 ) ) ;
#22208=CARTESIAN_POINT ( 'NONE',  ( 805.1016975059191054, -438.8965053807771710, -343.0745993439771837 ) ) ;
#22218=CARTESIAN_POINT ( 'NONE',  ( 805.2837595273609850, -74.73633629969866377, -340.5290396650784714 ) ) ;
#22220=CARTESIAN_POINT ( 'NONE',  ( 788.8264449731201466, -285.1800572038741279, -363.6646147819170665 ) ) ;
#22222=CARTESIAN_POINT ( 'NONE',  ( 771.2633955100217236, -383.9073299311466485, -363.4237431249939618 ) ) ;
#22223=CARTESIAN_POINT ( 'NONE',  ( 803.4237431249931660, -63.18005720387488822, -331.2633955100225194 ) ) ;
#22227=CARTESIAN_POINT ( 'NONE',  ( 786.2694204179717872, -21.28179084515337749, -305.1769319972829067 ) ) ;
#22230=CARTESIAN_POINT ( 'NONE',  ( 773.7305795820266212, -297.2817908451526137, -374.8230680027170365 ) ) ;
#22233=CARTESIAN_POINT ( 'NONE',  ( 759.7806653035534055, -246.9982390220560546, -324.8639956371180801 ) ) ;
#22235=CARTESIAN_POINT ( 'NONE',  ( 759.0159684113467620, -136.9181544815166376, -325.8855110935213020 ) ) ;
#22238=CARTESIAN_POINT ( 'NONE',  ( 783.7566961878529810, -24.89650538077847486, -305.1792804349288417 ) ) ;
#22239=CARTESIAN_POINT ( 'NONE',  ( 746.8695393053151292, -341.9073299311466485, -327.6429770376306578 ) ) ;
#22243=CARTESIAN_POINT ( 'NONE',  ( 761.9338519418445230, -230.5328690171415076, -370.4231160770881957 ) ) ;
#22245=CARTESIAN_POINT ( 'NONE',  ( 773.7943932421234194, -431.8055962898681059, -305.5313806188329409 ) ) ;
#22250=CARTESIAN_POINT ( 'NONE',  ( 805.0264073115434940, -6.351050835323991173, -339.4763451958999099 ) ) ;
#22257=CARTESIAN_POINT ( 'NONE',  ( 792.1044303154645831, -36.45278447660223975, -317.8323909638837677 ) ) ;
#22258=CARTESIAN_POINT ( 'NONE',  ( 760.5453621957607311, -309.0783235625957559, -323.8424801807151425 ) ) ;
#22260=CARTESIAN_POINT ( 'NONE',  ( 761.9338519418445230, -326.5328690171411381, -370.4231160770881957 ) ) ;
#22265=CARTESIAN_POINT ( 'NONE',  ( 784.0799538623451781, -83.80559628986920018, -364.6971507214555572 ) ) ;
#22268=CARTESIAN_POINT ( 'NONE',  ( 745.4481719005789273, -195.7255117493289731, -347.5162901302853129 ) ) ;
#22271=CARTESIAN_POINT ( 'NONE',  ( 805.1927285166399315, -184.8164208402381234, -341.8018195045277707 ) ) ;
#22273=CARTESIAN_POINT ( 'NONE',  ( 766.9102291470427417, -426.5545181178794678, -318.6633372737382501 ) ) ;
#22281=CARTESIAN_POINT ( 'NONE',  ( 800.9840315886518738, -436.9181544815157281, -354.1144889064786412 ) ) ;
#22283=CARTESIAN_POINT ( 'NONE',  ( 814.4686193811664907, -219.2817908451527558, -346.2056067578752732 ) ) ;
#22287=CARTESIAN_POINT ( 'NONE',  ( 793.2243759319678702, -338.5328690171411381, -318.4439275373583200 ) ) ;
#22289=CARTESIAN_POINT ( 'NONE',  ( 773.7305795820266212, -201.2817908451528126, -374.8230680027170365 ) ) ;
#22290=DIRECTION ( 'NONE',  ( -1.000000000000000000, 0.000000000000000000, 0.000000000000000000 ) ) ;
#22293=CARTESIAN_POINT ( 'NONE',  ( 814.5518280994195948, -255.7255117493287742, -332.4837098697145166 ) ) ;
#22296=CARTESIAN_POINT ( 'NONE',  ( 774.6312213355099630, -23.36187538569318889, -364.6798772138717482 ) ) ;
#22298=CARTESIAN_POINT ( 'NONE',  ( 801.9858362298568863, -147.0783235625962959, -312.7379699480935642 ) ) ;
#22300=CARTESIAN_POINT ( 'NONE',  ( 767.6429770376289525, -369.1800572038739574, -306.8695393053162093 ) ) ;
#22305=CARTESIAN_POINT ( 'NONE',  ( 757.8323909638827445, -386.6346026584191691, -352.1044303154654358 ) ) ;
#22306=CARTESIAN_POINT ( 'NONE',  ( 795.1271208383656131, -452.8379544210779954, -371.6178728169206238 ) ) ;
#22310=CARTESIAN_POINT ( 'NONE',  ( 802.7791456095903868, -172.7146871989598083, -329.0155153010375102 ) ) ;
#22312=CARTESIAN_POINT ( 'NONE',  ( 812.6845335610512393, -223.9874144716869182, -353.5525998758768651 ) ) ;
#22315=CARTESIAN_POINT ( 'NONE',  ( 801.9419747391806368, -138.4527844766019200, -351.9812246680014027 ) ) ;
#22317=CARTESIAN_POINT ( 'NONE',  ( 814.5518280994195948, -63.72551174932939233, -332.4837098697145734 ) ) ;
#22320=CARTESIAN_POINT ( 'NONE',  ( 763.0428371773158460, -11.46360902697159290, -358.7617431975195359 ) ) ;
#22322=CARTESIAN_POINT ( 'NONE',  ( 757.4527132478984868, -328.3726999360615650, -329.1273215169538844 ) ) ;
#22325=CARTESIAN_POINT ( 'NONE',  ( 788.7366044899766848, -299.9073299311468759, -316.5762568750059813 ) ) ;
#22328=CARTESIAN_POINT ( 'NONE',  ( 773.4516893846965786, -283.6454272087889308, -315.8398074228977066 ) ) ;
#22329=CARTESIAN_POINT ( 'NONE',  ( 774.6858677611749044, -297.7255117493286889, -315.5713283507209894 ) ) ;
#22331=CARTESIAN_POINT ( 'NONE',  ( 797.6776695296629214, -139.5436935675110135, -357.6776695296636603 ) ) ;
#22336=CARTESIAN_POINT ( 'NONE',  ( 762.1177392798416577, -90.55451811788041994, -309.8865473780659272 ) ) ;
#22337=DIRECTION ( 'NONE',  ( 1.000000000000000000, 0.000000000000000000, 0.000000000000000000 ) ) ;
#22343=CARTESIAN_POINT ( 'NONE',  ( 813.1304606946831655, -137.9073299311473875, -352.3570229623691716 ) ) ;
#22346=CARTESIAN_POINT ( 'NONE',  ( 772.3691319403857278, -431.2601417444136018, -315.8894580844506663 ) ) ;
#22348=CARTESIAN_POINT ( 'NONE',  ( 767.7687537140311633, -263.9073299311469327, -372.7932403749916830 ) ) ;
#22353=CARTESIAN_POINT ( 'NONE',  ( 801.9858362298568863, -291.0783235625957559, -312.7379699480935642 ) ) ;
#22355=CARTESIAN_POINT ( 'NONE',  ( 808.0189434323515343, -350.0891481129648923, -319.0252816721025511 ) ) ;
#22359=CARTESIAN_POINT ( 'NONE',  ( 755.3201227861273992, -411.7255117493282910, -345.3687786644892981 ) ) ;
#22361=CARTESIAN_POINT ( 'NONE',  ( 815.0009284576459549, -126.3510508353236048, -338.7629533639073429 ) ) ;
#22366=CARTESIAN_POINT ( 'NONE',  ( 755.0488828828309806, -233.8055962898687028, -344.1219089521771934 ) ) ;
#22368=CARTESIAN_POINT ( 'NONE',  ( 791.1614460488616487, -59.26014174441473870, -373.5763878283158874 ) ) ;
#22372=CARTESIAN_POINT ( 'NONE',  ( 802.2119215644370342, -342.0090635724251342, -367.5423716828165084 ) ) ;
#22376=CARTESIAN_POINT ( 'NONE',  ( 804.1105419155481968, -171.8272453906074304, -347.6308680596136469 ) ) ;
#22377=CARTESIAN_POINT ( 'NONE',  ( 759.7806653035534055, -198.9982390220562252, -324.8639956371180801 ) ) ;
#22379=CARTESIAN_POINT ( 'NONE',  ( 755.5713283507202505, -389.3618753856919739, -334.6858677611754729 ) ) ;
#22391=CARTESIAN_POINT ( 'NONE',  ( 771.3260364891663130, -427.6454272087885897, -306.0683387631859773 ) ) ;
#22392=CARTESIAN_POINT ( 'NONE',  ( 777.5031285880264704, -46.81642084023858530, -374.9108240113588408 ) ) ;
#22394=CARTESIAN_POINT ( 'NONE',  ( 765.0180583372156207, -384.9982390220556567, -360.0135310231089534 ) ) ;
#22395=CARTESIAN_POINT ( 'NONE',  ( 771.1735550268780344, -9.180057203875058747, -316.3353852180828198 ) ) ;
#22396=AXIS2_PLACEMENT_3D ( 'NONE', #1659, #22906, #22688 ) ;
#22399=CARTESIAN_POINT ( 'NONE',  ( 796.9571628226829034, -263.4636090269708006, -321.2382568024804641 ) ) ;
#22400=CARTESIAN_POINT ( 'NONE',  ( 800.9747183278959710, -180.9982390220563389, -311.9810565676471583 ) ) ;
#22411=CARTESIAN_POINT ( 'NONE',  ( 767.8955696845333705, -312.4527844766012663, -362.1676090361162323 ) ) ;
#22415=CARTESIAN_POINT ( 'NONE',  ( 745.7194118038753459, -61.64542720878961291, -348.7631598425976449 ) ) ;
#22416=CARTESIAN_POINT ( 'NONE',  ( 794.1144889064781864, -106.1692326535054889, -360.9840315886528401 ) ) ;
#22419=CARTESIAN_POINT ( 'NONE',  ( 797.8594530101008786, -13.54369356751140785, -322.1405469898980982 ) ) ;
#22420=CARTESIAN_POINT ( 'NONE',  ( 754.9735926884551418, -114.3510508353236617, -340.5236548041000333 ) ) ;
#22421=CARTESIAN_POINT ( 'NONE',  ( 755.0636971347428243, -124.2709662947837899, -341.7834795799807353 ) ) ;
#22422=CARTESIAN_POINT ( 'NONE',  ( 799.4546378042377910, -441.0783235625953580, -356.1575198192848006 ) ) ;
#22438=CARTESIAN_POINT ( 'NONE',  ( 801.5560724626406000, -96.55451811788039151, -326.7756240680316182 ) ) ;
#22440=CARTESIAN_POINT ( 'NONE',  ( 785.3141322388236176, -285.7255117493286889, -364.4286716492789537 ) ) ;
#22442=CARTESIAN_POINT ( 'NONE',  ( 788.8264449731200330, -381.1800572038737869, -363.6646147819171233 ) ) ;
#22443=CARTESIAN_POINT ( 'NONE',  ( 778.1981804954714335, -34.27096629478407408, -314.8072714833589885 ) ) ;
#22445=ADVANCED_FACE ( 'NONE', ( #36349, #8186 ), #21807, .F. ) ;
#22448=EDGE_CURVE ( 'NONE', #9510, #34870, #7972, .T. ) ;
#22450=CARTESIAN_POINT ( 'NONE',  ( 797.8822607201568644, -30.55451811788062244, -370.1134526219340160 ) ) ;
#22453=CARTESIAN_POINT ( 'NONE',  ( 814.4686193811664907, -291.2817908451525000, -346.2056067578752732 ) ) ;
#22457=CARTESIAN_POINT ( 'NONE',  ( 767.8955696845333705, -288.4527844766014937, -362.1676090361162323 ) ) ;
#22459=CARTESIAN_POINT ( 'NONE',  ( 804.4086373105744769, -145.6454272087893287, -333.3843516231986541 ) ) ;
#22462=CARTESIAN_POINT ( 'NONE',  ( 808.0189434323515343, -350.0891481129648923, -319.0252816721025511 ) ) ;
#22466=CARTESIAN_POINT ( 'NONE',  ( 776.2433038121456548, -252.8965053807777394, -374.8207195650711014 ) ) ;
#22468=CARTESIAN_POINT ( 'NONE',  ( 805.9055244015594326, -435.6237781080499190, -315.8990559732753240 ) ) ;
#22470=CIRCLE ( 'NONE', #9230, 10.00000000000000888 ) ;
#22474=CARTESIAN_POINT ( 'NONE',  ( 805.1016975059191054, -30.89650538077846065, -343.0745993439771837 ) ) ;
#22480=CARTESIAN_POINT ( 'NONE',  ( 784.0799538623451781, -323.8055962898684470, -364.6971507214555572 ) ) ;
#22483=CARTESIAN_POINT ( 'NONE',  ( 778.7502325331095108, -336.3510508353228943, -304.6391490659818828 ) ) ;
#22490=CARTESIAN_POINT ( 'NONE',  ( 796.7845633553578182, -81.62377810805104161, -358.5707757039688204 ) ) ;
#22493=CARTESIAN_POINT ( 'NONE',  ( 801.1904061080336987, -188.0891481129653187, -368.3070685750235498 ) ) ;
#22495=CARTESIAN_POINT ( 'NONE',  ( 800.2193346964446619, -186.9982390220563104, -355.1360043628816925 ) ) ;
#22496=ORIENTED_EDGE ( 'NONE', *, *, #17335, .F. ) ;
#22497=CARTESIAN_POINT ( 'NONE',  ( 799.2566176426618085, -432.0090635724247932, -324.0069404352559559 ) ) ;
#22506=CARTESIAN_POINT ( 'NONE',  ( 755.8894580844503253, -423.8272453906067199, -332.3691319403863531 ) ) ;
#22508=CARTESIAN_POINT ( 'NONE',  ( 771.3260364891663130, -187.6454272087892434, -306.0683387631859773 ) ) ;
#22510=CARTESIAN_POINT ( 'NONE',  ( 799.9999999999993179, -512.9681489794448908, -309.9999999999998863 ) ) ;
#22511=CARTESIAN_POINT ( 'NONE',  ( 785.3687786644884454, -203.3618753856925991, -315.3201227861279676 ) ) ;
#22512=CARTESIAN_POINT ( 'NONE',  ( 756.1348686366196716, -329.2601417444138860, -347.5531968255698416 ) ) ;
#22513=DIRECTION ( 'NONE',  ( 0.000000000000000000, -0.000000000000000000, -1.000000000000000000 ) ) ;
#22514=CARTESIAN_POINT ( 'NONE',  ( 748.6759233522253680, -232.3726999360617924, -324.3348316497537098 ) ) ;
#22517=CARTESIAN_POINT ( 'NONE',  ( 790.9844846989617508, -46.37269993606239638, -317.2208543904092721 ) ) ;
#22520=CARTESIAN_POINT ( 'NONE',  ( 748.9653473494365699, -242.6346026584197659, -356.9462024416520762 ) ) ;
#22521=LINE ( 'NONE', #36849, #27566 ) ;
#22522=CARTESIAN_POINT ( 'NONE',  ( 771.1735550268778070, -9.180057203875058747, -316.3353852180827630 ) ) ;
#22525=CARTESIAN_POINT ( 'NONE',  ( 808.7758568127978833, -124.1692326535054463, -320.0363995740631822 ) ) ;
#22527=CARTESIAN_POINT ( 'NONE',  ( 804.7487373415286811, -379.5436935675102745, -364.7487373415288516 ) ) ;
#22528=VECTOR ( 'NONE', #6619, 1000.000000000000000 ) ;
#22529=CARTESIAN_POINT ( 'NONE',  ( 767.9999999999992042, 240.0000000000000853, -360.0000000000000000 ) ) ;
#22533=CARTESIAN_POINT ( 'NONE',  ( 759.9864689768902508, -386.0891481129647786, -354.9819416627836404 ) ) ;
#22535=CARTESIAN_POINT ( 'NONE',  ( 778.7629533639073998, -8.736336299698871599, -375.0009284576466371 ) ) ;
#22540=CARTESIAN_POINT ( 'NONE',  ( 789.9200121543843807, -241.9874144716869182, -317.0176451133914384 ) ) ;
#22543=CARTESIAN_POINT ( 'NONE',  ( 811.6461892240364477, -220.7146871989596661, -324.1737431748509835 ) ) ;
#22546=CARTESIAN_POINT ( 'NONE',  ( 794.9819416627830151, -84.99823902205663728, -319.9864689768909898 ) ) ;
#22549=CARTESIAN_POINT ( 'NONE',  ( 765.0180583372156207, -144.9982390220564525, -360.0135310231089534 ) ) ;
#22551=CARTESIAN_POINT ( 'NONE',  ( 814.9108240113580450, -64.27096629478397460, -337.5031285880265273 ) ) ;
#22552=CARTESIAN_POINT ( 'NONE',  ( 803.4237431249931660, -63.18005720387488822, -331.2633955100225194 ) ) ;
#22554=CARTESIAN_POINT ( 'NONE',  ( 804.4086373105744769, -1.645427208789804308, -333.3843516231986541 ) ) ;
#22557=CARTESIAN_POINT ( 'NONE',  ( 759.0159684113467620, -328.9181544815160692, -325.8855110935213020 ) ) ;
#22565=CARTESIAN_POINT ( 'NONE',  ( 796.9571628226829034, -311.4636090269706870, -321.2382568024804641 ) ) ;
#22566=CARTESIAN_POINT ( 'NONE',  ( 797.8594530101008786, -301.5436935675105588, -322.1405469898980982 ) ) ;
#22567=CARTESIAN_POINT ( 'NONE',  ( 755.5713283507202505, -149.3618753856928265, -334.6858677611754729 ) ) ;
#22572=CARTESIAN_POINT ( 'NONE',  ( 805.6418435158337843, -101.4636090269713264, -363.8556311672236916 ) ) ;
#22579=CARTESIAN_POINT ( 'NONE',  ( 777.4774526936600978, -130.2709662947837614, -304.7301800767028226 ) ) ;
#22582=CARTESIAN_POINT ( 'NONE',  ( 810.7187646348534145, -258.4527844766016074, -356.7737145352016341 ) ) ;
#22585=CARTESIAN_POINT ( 'NONE',  ( 751.2241431872005251, -328.1692326535048210, -359.9636004259367610 ) ) ;
#22586=CARTESIAN_POINT ( 'NONE',  ( 787.4397851343537695, -93.72551174932934259, -374.2001403089903988 ) ) ;
#22588=CARTESIAN_POINT ( 'NONE',  ( 796.9462024416508257, -348.4527844766012663, -308.9653473494370246 ) ) ;
#22593=CARTESIAN_POINT ( 'NONE',  ( 762.1405469898971887, -217.5436935675107293, -357.8594530101015607 ) ) ;
#22594=CARTESIAN_POINT ( 'NONE',  ( 815.1787889125755555, -102.8965053807782368, -343.7953271457877804 ) ) ;
#22595=DIRECTION ( 'NONE',  ( -1.000000000000000000, -0.000000000000000000, -0.000000000000000000 ) ) ;
#22599=CARTESIAN_POINT ( 'NONE',  ( 756.1348686366196716, -233.2601417444141987, -347.5531968255698416 ) ) ;
#22602=CARTESIAN_POINT ( 'NONE',  ( 792.2312462859673587, 12.09267006885214180, -307.2067596250082602 ) ) ;
#22603=CARTESIAN_POINT ( 'NONE',  ( 764.3348316497523456, -70.71468719896014932, -308.6759233522265617 ) ) ;
#22608=CARTESIAN_POINT ( 'NONE',  ( 793.5525998758768083, -391.0999726633340288, -372.6845335610516941 ) ) ;
#22609=CARTESIAN_POINT ( 'NONE',  ( 778.2165204200184689, -238.8164208402379813, -364.9363028652563230 ) ) ;
#22612=CARTESIAN_POINT ( 'NONE',  ( 799.2566176426618085, -216.0090635724255037, -324.0069404352559559 ) ) ;
#22613=CARTESIAN_POINT ( 'NONE',  ( 762.3223304703356007, -175.5436935675108998, -322.3223304703362828 ) ) ;
#22614=CARTESIAN_POINT ( 'NONE',  ( 778.2165204200184689, -382.8164208402374697, -364.9363028652563230 ) ) ;
#22616=CARTESIAN_POINT ( 'NONE',  ( 791.9812246680005501, -452.6346026584191691, -361.9419747391813189 ) ) ;
#22628=CARTESIAN_POINT ( 'NONE',  ( 815.3608509340175488, -410.7363362996976548, -341.2497674668889545 ) ) ;
#22630=CARTESIAN_POINT ( 'NONE',  ( 792.2312462859673587, -35.90732993114770011, -307.2067596250082602 ) ) ;
#22633=CARTESIAN_POINT ( 'NONE',  ( 757.8323909638827445, -410.6346026584191122, -352.1044303154654358 ) ) ;
#22634=CARTESIAN_POINT ( 'NONE',  ( 800.2193346964446619, 5.001760977943074948, -355.1360043628816925 ) ) ;
#22636=LINE ( 'NONE', #40208, #30347 ) ;
#22637=CARTESIAN_POINT ( 'NONE',  ( 799.2566176426618085, -264.0090635724253616, -324.0069404352559559 ) ) ;
#22638=CARTESIAN_POINT ( 'NONE',  ( 747.2067596250078623, -171.1800572038745543, -352.2312462859687230 ) ) ;
#22646=CARTESIAN_POINT ( 'NONE',  ( 778.1981804954714335, -322.2709662947830225, -314.8072714833589885 ) ) ;
#22649=CARTESIAN_POINT ( 'NONE',  ( 793.5525998758768083, -103.0999726633349525, -372.6845335610516941 ) ) ;
#22650=CARTESIAN_POINT ( 'NONE',  ( 793.2243759319678702, -122.5328690171417918, -318.4439275373583200 ) ) ;
#22655=CARTESIAN_POINT ( 'NONE',  ( 797.6776695296629214, -19.54369356751139364, -357.6776695296636603 ) ) ;
#22656=CARTESIAN_POINT ( 'NONE',  ( 758.6633372737375112, -140.5328690171417634, -326.9102291470432533 ) ) ;
#22657=CARTESIAN_POINT ( 'NONE',  ( 802.1676090361156639, -134.6346026584201070, -327.8955696845344505 ) ) ;
#22660=CARTESIAN_POINT ( 'NONE',  ( 804.9511171171677688, -437.8055962898679923, -335.8780910478229202 ) ) ;
#22666=CARTESIAN_POINT ( 'NONE',  ( 771.3260364891663130, -259.6454272087890445, -306.0683387631859773 ) ) ;
#22667=AXIS2_PLACEMENT_3D ( 'NONE', #43296, #32454, #39627 ) ;
#22674=CARTESIAN_POINT ( 'NONE',  ( 804.4086373105744769, -73.64542720878957027, -333.3843516231986541 ) ) ;
#22675=CARTESIAN_POINT ( 'NONE',  ( 755.5713283507202505, -293.3618753856923718, -334.6858677611754729 ) ) ;
#22677=CARTESIAN_POINT ( 'NONE',  ( 767.8955696845333705, -384.4527844766011526, -362.1676090361162323 ) ) ;
#22678=CARTESIAN_POINT ( 'NONE',  ( 755.3201227861273992, -51.72551174932946338, -345.3687786644892981 ) ) ;
#22683=CARTESIAN_POINT ( 'NONE',  ( 814.4686193811664907, -27.28179084515336328, -346.2056067578752732 ) ) ;
#22684=CYLINDRICAL_SURFACE ( 'NONE', #25501, 20.00000000000001776 ) ;
#22685=EDGE_LOOP ( 'NONE', ( #26536, #25700, #3546, #43018 ) ) ;
#22686=CARTESIAN_POINT ( 'NONE',  ( 745.5313806188320314, -303.2817908451525000, -333.7943932421247268 ) ) ;
#22688=DIRECTION ( 'NONE',  ( 0.000000000000000000, -0.000000000000000000, -1.000000000000000000 ) ) ;
#22689=CARTESIAN_POINT ( 'NONE',  ( 778.2165204200184689, -286.8164208402378677, -364.9363028652563230 ) ) ;
#22691=CARTESIAN_POINT ( 'NONE',  ( 793.9708237608222134, -166.9181544815165523, -319.2295555964448681 ) ) ;
#22692=CARTESIAN_POINT ( 'NONE',  ( 799.9999999999993179, -512.9681489794448908, -309.9999999999998863 ) ) ;
#22693=CARTESIAN_POINT ( 'NONE',  ( 755.2512626584698410, -343.5436935675103314, -315.2512626584710915 ) ) ;
#22699=CARTESIAN_POINT ( 'NONE',  ( 815.2698199232961542, 7.183579159761247723, -342.5225473063383106 ) ) ;
#22705=CARTESIAN_POINT ( 'NONE',  ( 764.0069404352550464, -15.07832356259669560, -359.2566176426627180 ) ) ;
#22711=CARTESIAN_POINT ( 'NONE',  ( 803.4237431249931660, -39.18005720387496638, -331.2633955100225194 ) ) ;
#22714=CARTESIAN_POINT ( 'NONE',  ( 800.7704444035546203, -340.1692326535047641, -326.0291762391768771 ) ) ;
#22717=CARTESIAN_POINT ( 'NONE',  ( 786.2056067578752163, -323.8055962898684470, -374.4686193811670023 ) ) ;
#22721=VERTEX_POINT ( 'NONE', #29429 ) ;
#22723=CARTESIAN_POINT ( 'NONE',  ( 812.7932403749906598, -183.1800572038744974, -327.7687537140311633 ) ) ;
#22725=ORIENTED_EDGE ( 'NONE', *, *, #11087, .T. ) ;
#22726=CARTESIAN_POINT ( 'NONE',  ( 781.8018195045267476, -190.2709662947835625, -365.1927285166407273 ) ) ;
#22730=CARTESIAN_POINT ( 'NONE',  ( 754.7162404726377645, -422.7363362996975980, -339.4709603349214717 ) ) ;
#22735=DIRECTION ( 'NONE',  ( 0.000000000000000000, 0.000000000000000000, -1.000000000000000000 ) ) ;
#22739=CARTESIAN_POINT ( 'NONE',  ( 801.5560724626406000, -432.5545181178793541, -326.7756240680316182 ) ) ;
#22741=CARTESIAN_POINT ( 'NONE',  ( 749.5768839229115201, -204.5545181178800931, -358.0661480581553064 ) ) ;
#22744=CARTESIAN_POINT ( 'NONE',  ( 755.3201227861273992, -195.7255117493289731, -345.3687786644892981 ) ) ;
#22745=CARTESIAN_POINT ( 'NONE',  ( 775.9200461376533440, -335.8055962898683902, -315.3028492785443291 ) ) ;
#22747=CARTESIAN_POINT ( 'NONE',  ( 776.2046728542105711, -236.1908817542436338, -304.8212110874238761 ) ) ;
#22750=CARTESIAN_POINT ( 'NONE',  ( 772.4468031744293057, -33.82724539060788516, -363.8651313633793620 ) ) ;
#22752=CARTESIAN_POINT ( 'NONE',  ( 763.2262854647970016, -248.6346026584197659, -309.2812353651462445 ) ) ;
#22754=DIRECTION ( 'NONE',  ( 0.7071067811865697772, 0.000000000000000000, -0.7071067811865252573 ) ) ;
#22755=CARTESIAN_POINT ( 'NONE',  ( 765.0180583372156207, -24.99823902205683268, -360.0135310231089534 ) ) ;
#22758=CARTESIAN_POINT ( 'NONE',  ( 813.9316612368132837, -127.4419599262326983, -348.6739635108323228 ) ) ;
#22760=CARTESIAN_POINT ( 'NONE',  ( 814.5518280994195948, -375.7255117493283478, -332.4837098697145734 ) ) ;
#22765=CARTESIAN_POINT ( 'NONE',  ( 788.8264449731200330, -381.1800572038737869, -363.6646147819171233 ) ) ;
#22768=CARTESIAN_POINT ( 'NONE',  ( 797.8822607201568644, -6.554518117880697048, -370.1134526219340160 ) ) ;
#22773=CARTESIAN_POINT ( 'NONE',  ( 803.2186876482843445, -223.9874144716869182, -350.0220218866286928 ) ) ;
#22775=CARTESIAN_POINT ( 'NONE',  ( 748.3538107759620743, -232.7146871989596377, -355.8262568251490165 ) ) ;
#22780=CARTESIAN_POINT ( 'NONE',  ( 803.8651313633788504, -29.26014174441482751, -332.4468031744301015 ) ) ;
#22782=CARTESIAN_POINT ( 'NONE',  ( 811.0346526505616112, -62.63460265842031305, -323.0537975583477532 ) ) ;
#22783=CARTESIAN_POINT ( 'NONE',  ( 785.3141322388236176, -69.72551174932942786, -364.4286716492789537 ) ) ;
#22785=CARTESIAN_POINT ( 'NONE',  ( 804.1105419155481968, -27.82724539060790292, -347.6308680596136469 ) ) ;
#22787=CARTESIAN_POINT ( 'NONE',  ( 790.0220218866281812, -319.0999726633342561, -363.2186876482849129 ) ) ;
#22794=CARTESIAN_POINT ( 'NONE',  ( 775.8780910478218402, -321.2817908451525000, -364.9511171171680530 ) ) ;
#22795=CARTESIAN_POINT ( 'NONE',  ( 804.4286716492782716, -329.3618753856922581, -345.3141322388244703 ) ) ;
#22796=CARTESIAN_POINT ( 'NONE',  ( 771.1735550268778070, -153.1800572038746395, -316.3353852180827630 ) ) ;
#22801=CARTESIAN_POINT ( 'NONE',  ( 812.3518521366052028, -121.0999726633348956, -326.5853460496235243 ) ) ;
#22807=CARTESIAN_POINT ( 'NONE',  ( 772.4837098697145166, -143.3618753856927697, -374.5518280994205611 ) ) ;
#22811=CARTESIAN_POINT ( 'NONE',  ( 777.5031285880264704, -286.8164208402378677, -374.9108240113588408 ) ) ;
#22812=CARTESIAN_POINT ( 'NONE',  ( 795.1271208383658404, -452.8379544210779954, -371.6178728169206238 ) ) ;
#22814=CARTESIAN_POINT ( 'NONE',  ( 761.9338519418445230, -350.5328690171411381, -370.4231160770881957 ) ) ;
#22815=CARTESIAN_POINT ( 'NONE',  ( 800.9747183278959710, -84.99823902205663728, -311.9810565676471583 ) ) ;
#22817=CARTESIAN_POINT ( 'NONE',  ( 754.9967657858570647, -337.5436935675102177, -365.0032342141425374 ) ) ;
#22821=CARTESIAN_POINT ( 'NONE',  ( 812.6845335610512393, -127.9874144716872308, -353.5525998758768651 ) ) ;
#22826=VERTEX_POINT ( 'NONE', #19703 ) ;
#22827=CARTESIAN_POINT ( 'NONE',  ( 754.9735926884551418, -234.3510508353232638, -340.5236548041000333 ) ) ;
#22829=CARTESIAN_POINT ( 'NONE',  ( 795.6651683502461765, -442.7146871989589840, -371.3240766477733814 ) ) ;
#22830=CARTESIAN_POINT ( 'NONE',  ( 812.6845335610512393, -55.98741447168748664, -353.5525998758768651 ) ) ;
#22834=CARTESIAN_POINT ( 'NONE',  ( 797.8822607201568644, -366.5545181178795815, -370.1134526219340160 ) ) ;
#22835=CARTESIAN_POINT ( 'NONE',  ( 804.6798772138708955, -231.7255117493288310, -334.6312213355107019 ) ) ;
#22839=CARTESIAN_POINT ( 'NONE',  ( 766.0291762391763086, -226.9181544815163534, -360.7704444035551319 ) ) ;
#22840=CARTESIAN_POINT ( 'NONE',  ( 804.9363028652555840, -208.2709662947835341, -338.2165204200192079 ) ) ;
#22841=CARTESIAN_POINT ( 'NONE',  ( 774.6312213355098493, -383.3618753856920875, -364.6798772138717482 ) ) ;
#22844=CARTESIAN_POINT ( 'NONE',  ( 800.2193346964447755, -114.9982390220565236, -355.1360043628815788 ) ) ;
#22853=CARTESIAN_POINT ( 'NONE',  ( 814.4686193811664907, -459.2817908451519884, -346.2056067578752732 ) ) ;
#22854=CARTESIAN_POINT ( 'NONE',  ( 796.7737145352015204, -20.63460265842048003, -370.7187646348536987 ) ) ;
#22856=CARTESIAN_POINT ( 'NONE',  ( 774.6858677611749044, -393.7255117493283478, -315.5713283507209894 ) ) ;
#22857=CARTESIAN_POINT ( 'NONE',  ( 800.0135310231082713, -14.08914811296595460, -325.0180583372163028 ) ) ;
#22860=CARTESIAN_POINT ( 'NONE',  ( 755.1538015810308480, -278.1908817542434917, -343.0433043558613804 ) ) ;
#22861=CARTESIAN_POINT ( 'NONE',  ( 808.0189434323515343, -182.0891481129654323, -319.0252816721025511 ) ) ;
#22865=EDGE_CURVE ( 'NONE', #811, #8509, #19464, .T. ) ;
#22869=CARTESIAN_POINT ( 'NONE',  ( 801.9419747391806368, -330.4527844766013231, -351.9812246680014027 ) ) ;
#22871=CARTESIAN_POINT ( 'NONE',  ( 802.2119215644370342, -102.0090635724258448, -367.5423716828165084 ) ) ;
#22872=CARTESIAN_POINT ( 'NONE',  ( 773.3843516231979720, -133.4419599262326699, -364.4086373105754433 ) ) ;
#22873=B_SPLINE_CURVE_WITH_KNOTS ( 'NONE', 3,
 ( #1402, #39992, #26777, #5778, #1619, #36739, #15718, #2076, #43442, #40444, #15506, #8796, #29586, #9009, #19634, #23317, #12479, #29804, #36957, #40656, #26102, #37421, #43883, #8340, #40883, #15949, #23079, #33729, #19864, #9247, #30031, #4870, #37178, #33273, #43662, #12260 ),
 .UNSPECIFIED., .F., .F.,
 ( 4, 2, 2, 2, 2, 2, 2, 2, 2, 2, 2, 2, 2, 2, 2, 2, 2, 4 ),
 ( 0.000000000000000000, 0.004405609005296106002, 0.008811218010592212005, 0.01101402251324022814, 0.01321682701588824428, 0.01762243602118459054, 0.01982524052383277668, 0.02202804502648095936, 0.02643365403177701245, 0.02863645853442487593, 0.03083926303707274288, 0.03194066528839652197, 0.03304206753972029759, 0.03359276866538235540, 0.03414346979104441321, 0.03469417091670646408, 0.03496952147953734380, 0.03524487204236821658 ),
 .UNSPECIFIED. ) ;
#22876=CARTESIAN_POINT ( 'NONE',  ( 771.2633955100217236, -23.90732993114773919, -363.4237431249939618 ) ) ;
#22877=CARTESIAN_POINT ( 'NONE',  ( 803.2186876482843445, -127.9874144716872308, -350.0220218866286928 ) ) ;
#22878=CARTESIAN_POINT ( 'NONE',  ( 764.8639956371174549, -128.0891481129655176, -319.7806653035542013 ) ) ;
#22880=CARTESIAN_POINT ( 'NONE',  ( 764.3348316497523456, 25.28531280103955226, -308.6759233522265617 ) ) ;
#22887=CARTESIAN_POINT ( 'NONE',  ( 814.8207195650702488, -290.1908817542434349, -336.2433038121456548 ) ) ;
#22892=ORIENTED_EDGE ( 'NONE', *, *, #38314, .F. ) ;
#22893=CARTESIAN_POINT ( 'NONE',  ( 769.9779781133707957, -115.0999726633348956, -316.7813123517150871 ) ) ;
#22894=CARTESIAN_POINT ( 'NONE',  ( 756.5762568750052424, -267.1800572038742985, -348.7366044899774238 ) ) ;
#22896=CARTESIAN_POINT ( 'NONE',  ( 791.9812246680005501, -428.6346026584192259, -361.9419747391813189 ) ) ;
#22897=CARTESIAN_POINT ( 'NONE',  ( 754.8072714833581358, -76.81642084023845030, -338.1981804954720587 ) ) ;
#22901=CARTESIAN_POINT ( 'NONE',  ( 771.3260364891663130, -19.64542720878974791, -306.0683387631859773 ) ) ;
#22904=CARTESIAN_POINT ( 'NONE',  ( 783.7953271457878373, -344.1908817542433212, -375.1787889125761239 ) ) ;
#22906=DIRECTION ( 'NONE',  ( 0.000000000000000000, -1.000000000000000000, 0.000000000000000000 ) ) ;
#22907=CARTESIAN_POINT ( 'NONE',  ( 755.3201227861273992, -291.7255117493285752, -345.3687786644892981 ) ) ;
#22909=CARTESIAN_POINT ( 'NONE',  ( 754.7162404726377645, -158.7363362996984222, -339.4709603349214717 ) ) ;
#22913=CARTESIAN_POINT ( 'NONE',  ( 759.0252816721024374, -336.9982390220558273, -368.0189434323527280 ) ) ;
#22918=CARTESIAN_POINT ( 'NONE',  ( 772.4837098697144029, 0.6381246143067236254, -374.5518280994205611 ) ) ;
#22923=CARTESIAN_POINT ( 'NONE',  ( 805.1016975059191054, -6.896505380778533478, -343.0745993439771837 ) ) ;
#22928=CARTESIAN_POINT ( 'NONE',  ( 798.7617431975189675, -339.6237781080502600, -323.0428371773161871 ) ) ;
#22931=CARTESIAN_POINT ( 'NONE',  ( 798.0661480581538854, -314.5328690171411949, -309.5768839229118043 ) ) ;
#22936=CARTESIAN_POINT ( 'NONE',  ( 758.8095938919642549, -176.0891481129653755, -311.6929314249763365 ) ) ;
#22939=CARTESIAN_POINT ( 'NONE',  ( 771.2633955100217236, -191.9073299311471885, -363.4237431249939618 ) ) ;
#22941=CARTESIAN_POINT ( 'NONE',  ( 802.1676090361156639, 9.365397341579420498, -327.8955696845344505 ) ) ;
#22947=EDGE_LOOP ( 'NONE', ( #37721, #18805 ) ) ;
#22948=CARTESIAN_POINT ( 'NONE',  ( 754.7162404726377645, -422.7363362996975980, -339.4709603349214717 ) ) ;
#22951=CARTESIAN_POINT ( 'NONE',  ( 799.9636004259356241, -190.9181544815164955, -311.2241431872006956 ) ) ;
#22954=CARTESIAN_POINT ( 'NONE',  ( 785.3687786644884454, -179.3618753856927128, -315.3201227861279676 ) ) ;
#22955=CARTESIAN_POINT ( 'NONE',  ( 779.4709603349208464, -360.3510508353228374, -314.7162404726379918 ) ) ;
#22957=CARTESIAN_POINT ( 'NONE',  ( 811.3240766477731540, -220.3726999360618208, -355.6651683502462902 ) ) ;
#22961=CARTESIAN_POINT ( 'NONE',  ( 757.0176451133909268, -61.09997266333506616, -349.9200121543848354 ) ) ;
#22964=CARTESIAN_POINT ( 'NONE',  ( 808.0189434323515343, -230.0891481129652618, -319.0252816721025511 ) ) ;
#22968=CARTESIAN_POINT ( 'NONE',  ( 771.1735550268778070, -33.18005720387498769, -316.3353852180827630 ) ) ;
#22970=CARTESIAN_POINT ( 'NONE',  ( 761.9338519418445230, -134.5328690171417350, -370.4231160770881957 ) ) ;
#22972=CARTESIAN_POINT ( 'NONE',  ( 813.1304606946830518, -377.9073299311466485, -352.3570229623690580 ) ) ;
#22977=CARTESIAN_POINT ( 'NONE',  ( 791.9812246680005501, -404.6346026584193396, -361.9419747391813189 ) ) ;
#22979=CARTESIAN_POINT ( 'NONE',  ( 814.4686193811664907, -3.281790845153435221, -346.2056067578752732 ) ) ;
#22980=CARTESIAN_POINT ( 'NONE',  ( 759.2380499001254748, 21.41625977839825978, -318.3449445151863415 ) ) ;
#22984=CARTESIAN_POINT ( 'NONE',  ( 755.0488828828309806, -209.8055962898687881, -344.1219089521771934 ) ) ;
#22985=EDGE_CURVE ( 'NONE', #16350, #31813, #6295, .T. ) ;
#22987=CARTESIAN_POINT ( 'NONE',  ( 751.2241431872005251, -208.1692326535051905, -359.9636004259367610 ) ) ;
#22990=ORIENTED_EDGE ( 'NONE', *, *, #43102, .T. ) ;
#22992=CARTESIAN_POINT ( 'NONE',  ( 792.1044303154645831, -180.4527844766017211, -317.8323909638837677 ) ) ;
#22994=CARTESIAN_POINT ( 'NONE',  ( 745.4481719005789273, -75.72551174932937101, -347.5162901302853129 ) ) ;
#22995=CARTESIAN_POINT ( 'NONE',  ( 804.9363028652555840, -88.27096629478390355, -338.2165204200192079 ) ) ;
#22997=CARTESIAN_POINT ( 'NONE',  ( 804.8461984189677878, -26.19088175424427334, -336.9566956441385628 ) ) ;
#22999=CARTESIAN_POINT ( 'NONE',  ( 796.9571628226829034, -335.4636090269705733, -321.2382568024804641 ) ) ;
#23007=CARTESIAN_POINT ( 'NONE',  ( 783.0745993439762742, -320.1908817542434349, -365.1016975059196739 ) ) ;
#23008=CARTESIAN_POINT ( 'NONE',  ( 774.6858677611749044, -321.7255117493286320, -315.5713283507209894 ) ) ;
#23009=CARTESIAN_POINT ( 'NONE',  ( 778.1981804954714335, -154.2709662947836478, -314.8072714833589885 ) ) ;
#23013=CARTESIAN_POINT ( 'NONE',  ( 745.7194118038753459, -133.6454272087893571, -348.7631598425976449 ) ) ;
#23022=CARTESIAN_POINT ( 'NONE',  ( 763.2262854647970016, -152.6346026584200786, -309.2812353651462445 ) ) ;
#23023=LINE ( 'NONE', #15883, #44520 ) ;
#23025=CARTESIAN_POINT ( 'NONE',  ( 792.2312462859673587, -275.9073299311469896, -307.2067596250082602 ) ) ;
#23029=CARTESIAN_POINT ( 'NONE',  ( 764.3348316497523456, -334.7146871989593251, -308.6759233522265617 ) ) ;
#23030=CARTESIAN_POINT ( 'NONE',  ( 808.0189434323515343, -86.08914811296573077, -319.0252816721025511 ) ) ;
#23032=CARTESIAN_POINT ( 'NONE',  ( 746.8695393053150156, -365.9073299311465917, -327.6429770376306010 ) ) ;
#23037=CARTESIAN_POINT ( 'NONE',  ( 776.2433038121456548, -132.8965053807781374, -374.8207195650711014 ) ) ;
#23041=CARTESIAN_POINT ( 'NONE',  ( 766.7756240680305382, -14.53286901714214707, -361.5560724626415663 ) ) ;
#23043=CARTESIAN_POINT ( 'NONE',  ( 786.2056067578752163, -419.8055962898681059, -374.4686193811670023 ) ) ;
#23046=ORIENTED_EDGE ( 'NONE', *, *, #39154, .F. ) ;
#23047=CARTESIAN_POINT ( 'NONE',  ( 768.9521613784389729, -369.8272453906068904, -373.2346286133773106 ) ) ;
#23049=CARTESIAN_POINT ( 'NONE',  ( 757.8323909638827445, -242.6346026584197659, -352.1044303154654358 ) ) ;
#23052=CARTESIAN_POINT ( 'NONE',  ( 773.4516893846965786, -211.6454272087891582, -315.8398074228977066 ) ) ;
#23053=CARTESIAN_POINT ( 'NONE',  ( 803.6646147819161570, -209.9073299311470748, -348.8264449731210561 ) ) ;
#23054=CARTESIAN_POINT ( 'NONE',  ( 758.0580252608178853, -414.4527844766010389, -328.0187753319985404 ) ) ;
#23057=CARTESIAN_POINT ( 'NONE',  ( 791.9812246680005501, -92.63460265842026331, -361.9419747391813189 ) ) ;
#23060=CARTESIAN_POINT ( 'NONE',  ( 767.9999999999992042, 178.9475563372491251, -360.0000000000000000 ) ) ;
#23066=CARTESIAN_POINT ( 'NONE',  ( 797.8822607201568644, -462.5545181178792973, -370.1134526219340160 ) ) ;
#23067=CIRCLE ( 'NONE', #14231, 4.999999999999982236 ) ;
#23068=CARTESIAN_POINT ( 'NONE',  ( 777.5031285880264704, -22.81642084023865280, -374.9108240113588408 ) ) ;
#23071=CARTESIAN_POINT ( 'NONE',  ( 802.1676090361156639, -398.6346026584193396, -327.8955696845344505 ) ) ;
#23072=CARTESIAN_POINT ( 'NONE',  ( 803.6646147819162707, 6.092670068852160448, -348.8264449731211130 ) ) ;
#23075=CARTESIAN_POINT ( 'NONE',  ( 754.7162404726377645, -302.7363362996979959, -339.4709603349214717 ) ) ;
#23076=CARTESIAN_POINT ( 'NONE',  ( 755.2512626584698410, -175.5436935675108998, -315.2512626584710915 ) ) ;
#23079=CARTESIAN_POINT ( 'NONE',  ( 793.5727445751998630, 16.45630643248830793, -314.6726781324130684 ) ) ;
#23082=CARTESIAN_POINT ( 'NONE',  ( 769.9999999999992042, 178.9475563372491251, -320.0000000000000000 ) ) ;
#23084=CARTESIAN_POINT ( 'NONE',  ( 762.3223304703356007, -343.5436935675103314, -322.3223304703362828 ) ) ;
#23086=CARTESIAN_POINT ( 'NONE',  ( 778.7629533639073998, -104.7363362996985785, -375.0009284576466371 ) ) ;
#23087=CARTESIAN_POINT ( 'NONE',  ( 754.9735926884551418, -162.3510508353235196, -340.5236548041000333 ) ) ;
#23090=CARTESIAN_POINT ( 'NONE',  ( 804.4286716492782716, -41.36187538569314626, -345.3141322388244703 ) ) ;
#23091=CARTESIAN_POINT ( 'NONE',  ( 766.7756240680305382, -158.5328690171417065, -361.5560724626415663 ) ) ;
#23092=CARTESIAN_POINT ( 'NONE',  ( 767.8955696845333705, -120.4527844766019484, -362.1676090361162323 ) ) ;
#23094=CARTESIAN_POINT ( 'NONE',  ( 794.1144889064781864, -418.1692326535044799, -360.9840315886528401 ) ) ;
#23101=CARTESIAN_POINT ( 'NONE',  ( 814.4686193811664907, -267.2817908451526137, -346.2056067578752732 ) ) ;
#23107=CARTESIAN_POINT ( 'NONE',  ( 804.1105419155481968, -123.8272453906076009, -347.6308680596136469 ) ) ;
#23108=CARTESIAN_POINT ( 'NONE',  ( 771.1735550268778070, -129.1800572038746111, -316.3353852180827630 ) ) ;
#23109=CARTESIAN_POINT ( 'NONE',  ( 785.3687786644885591, -275.3618753856924286, -315.3201227861280813 ) ) ;
#23111=CARTESIAN_POINT ( 'NONE',  ( 774.6312213355099630, -431.3618753856918033, -364.6798772138717482 ) ) ;
#23112=CARTESIAN_POINT ( 'NONE',  ( 797.6776695296629214, -91.54369356751116982, -357.6776695296636603 ) ) ;
#23118=CARTESIAN_POINT ( 'NONE',  ( 786.2694204179717872, -357.2817908451523294, -305.1769319972829067 ) ) ;
#23120=CARTESIAN_POINT ( 'NONE',  ( 794.9819416627830151, -276.9982390220559978, -319.9864689768909898 ) ) ;
#23122=CARTESIAN_POINT ( 'NONE',  ( 787.5531968255692163, -189.8272453906073736, -316.1348686366205811 ) ) ;
#23126=CARTESIAN_POINT ( 'NONE',  ( 814.2001403089898304, -377.3618753856920875, -347.4397851343538264 ) ) ;
#23132=CARTESIAN_POINT ( 'NONE',  ( 755.2512626584698410, -31.54369356751135456, -315.2512626584710915 ) ) ;
#23133=CARTESIAN_POINT ( 'NONE',  ( 804.9363028652555840, -232.2709662947834488, -338.2165204200192079 ) ) ;
#23137=CARTESIAN_POINT ( 'NONE',  ( 756.7813123517142913, -19.98741447168758256, -329.9779781133712504 ) ) ;
#23144=CARTESIAN_POINT ( 'NONE',  ( 804.1601925771018387, -319.4419599262320730, -346.5483106153029098 ) ) ;
#23147=CARTESIAN_POINT ( 'NONE',  ( 781.2497674668890113, -372.3510508353228374, -375.3608509340180603 ) ) ;
#23152=ORIENTED_EDGE ( 'NONE', *, *, #16294, .F. ) ;
#23153=CARTESIAN_POINT ( 'NONE',  ( 0.000000000000000000, 0.000000000000000000, 0.000000000000000000 ) ) ;
#23154=CARTESIAN_POINT ( 'NONE',  ( 744.7301800767019131, -196.8164208402380950, -337.4774526936615757 ) ) ;
#23158=CARTESIAN_POINT ( 'NONE',  ( 759.9864689768902508, -194.0891481129654039, -354.9819416627836404 ) ) ;
#23161=CARTESIAN_POINT ( 'NONE',  ( 804.4286716492782716, -329.3618753856922581, -345.3141322388244703 ) ) ;
#23162=CARTESIAN_POINT ( 'NONE',  ( 796.9571628226829034, -455.4636090269701754, -321.2382568024804641 ) ) ;
#23169=CARTESIAN_POINT ( 'NONE',  ( 798.5707757039680246, -437.4636090269703459, -356.7845633553585003 ) ) ;
#23173=CARTESIAN_POINT ( 'NONE',  ( 760.0363995740630116, -250.9181544815163534, -368.7758568127991907 ) ) ;
#23177=CARTESIAN_POINT ( 'NONE',  ( 755.5713283507202505, -173.3618753856927128, -334.6858677611754729 ) ) ;
#23178=CARTESIAN_POINT ( 'NONE',  ( 760.5453621957607311, -357.0783235625956422, -323.8424801807151425 ) ) ;
#23180=CARTESIAN_POINT ( 'NONE',  ( 783.7953271457878373, -224.1908817542436623, -375.1787889125761239 ) ) ;
#23182=DIRECTION ( 'NONE',  ( -0.000000000000000000, -0.000000000000000000, 1.000000000000000000 ) ) ;
#23183=CARTESIAN_POINT ( 'NONE',  ( 769.0155153010367712, -82.37269993606227558, -362.7791456095907279 ) ) ;
#23187=CARTESIAN_POINT ( 'NONE',  ( 814.5518280994195948, -279.7255117493288026, -332.4837098697145166 ) ) ;
#23190=CARTESIAN_POINT ( 'NONE',  ( 803.6646147819161570, -41.90732993114767169, -348.8264449731210561 ) ) ;
#23192=CARTESIAN_POINT ( 'NONE',  ( 744.8212110874229666, -138.8965053807781374, -336.2046728542121627 ) ) ;
#23194=CARTESIAN_POINT ( 'NONE',  ( 763.0537975583475827, -408.4527844766009252, -371.0346526505627480 ) ) ;
#23198=CARTESIAN_POINT ( 'NONE',  ( 802.1676090361156639, -374.6346026584192828, -327.8955696845344505 ) ) ;
#23200=CARTESIAN_POINT ( 'NONE',  ( 776.2046728542105711, -44.19088175424421649, -304.8212110874238761 ) ) ;
#23206=CARTESIAN_POINT ( 'NONE',  ( 757.2208543904082489, -208.7146871989596946, -350.9844846989624330 ) ) ;
#23209=CARTESIAN_POINT ( 'NONE',  ( 751.2241431872005251, -232.1692326535051620, -359.9636004259367610 ) ) ;
#23215=CARTESIAN_POINT ( 'NONE',  ( 763.2154366446407039, -21.62377810805121570, -321.4292242960311228 ) ) ;
#23216=CARTESIAN_POINT ( 'NONE',  ( 797.6776695296629214, -187.5436935675108430, -357.6776695296636603 ) ) ;
#23220=CARTESIAN_POINT ( 'NONE',  ( 813.1304606946830518, -89.90732993114750116, -352.3570229623690580 ) ) ;
#23223=CARTESIAN_POINT ( 'NONE',  ( 785.3687786644885591, -59.36187538569307520, -315.3201227861280813 ) ) ;
#23225=CARTESIAN_POINT ( 'NONE',  ( 757.4527132478984868, -16.37269993606248519, -329.1273215169538844 ) ) ;
#23227=CARTESIAN_POINT ( 'NONE',  ( 804.4086373105744769, -361.6454272087887603, -333.3843516231986541 ) ) ;
#23234=AXIS2_PLACEMENT_3D ( 'NONE', #7441, #32388, #14617 ) ;
#23235=CARTESIAN_POINT ( 'NONE',  ( 799.2566176426618085, -312.0090635724251911, -324.0069404352559559 ) ) ;
#23236=CARTESIAN_POINT ( 'NONE',  ( 781.8018195045266339, -310.2709662947832499, -365.1927285166406705 ) ) ;
#23237=CARTESIAN_POINT ( 'NONE',  ( 745.5313806188320314, -135.2817908451530116, -333.7943932421247268 ) ) ;
#23243=DIRECTION ( 'NONE',  ( 0.000000000000000000, 1.000000000000000000, 0.000000000000000000 ) ) ;
#23245=CARTESIAN_POINT ( 'NONE',  ( 771.3260364891663130, -115.6454272087894424, -306.0683387631859773 ) ) ;
#23253=CARTESIAN_POINT ( 'NONE',  ( 814.5518280994195948, -159.7255117493291436, -332.4837098697145166 ) ) ;
#23257=CARTESIAN_POINT ( 'NONE',  ( 814.2001403089898304, -257.3618753856924286, -347.4397851343538264 ) ) ;
#23259=CARTESIAN_POINT ( 'NONE',  ( 748.9653473494365699, -434.6346026584190554, -356.9462024416520762 ) ) ;
#23263=CARTESIAN_POINT ( 'NONE',  ( 759.8311093483677041, -334.1692326535047073, -310.9282345327691814 ) ) ;
#23264=CARTESIAN_POINT ( 'NONE',  ( 805.0032342141412300, -85.54369356751118403, -314.9967657858571783 ) ) ;
#23267=CARTESIAN_POINT ( 'NONE',  ( 745.7998596910086917, -389.3618753856919739, -332.5602148656461168 ) ) ;
#23272=CARTESIAN_POINT ( 'NONE',  ( 771.2368401574024119, -133.4419599262326699, -374.2805881961240857 ) ) ;
#23278=CARTESIAN_POINT ( 'NONE',  ( 780.5290396650775619, -12.35105083532396897, -365.2837595273619513 ) ) ;
#23282=CARTESIAN_POINT ( 'NONE',  ( 756.1443688327750579, -429.6237781080499190, -314.3581564841659315 ) ) ;
#23284=ORIENTED_EDGE ( 'NONE', *, *, #7500, .T. ) ;
#23286=CARTESIAN_POINT ( 'NONE',  ( 750.9282345327678740, -376.9181544815159555, -319.8311093483690115 ) ) ;
#23288=CARTESIAN_POINT ( 'NONE',  ( 785.3141322388236176, -237.7255117493289163, -364.4286716492789537 ) ) ;
#23293=CARTESIAN_POINT ( 'NONE',  ( 804.1105419155481968, -219.8272453906073167, -347.6308680596136469 ) ) ;
#23294=CARTESIAN_POINT ( 'NONE',  ( 803.6646147819161570, -233.9073299311470180, -348.8264449731210561 ) ) ;
#23295=CARTESIAN_POINT ( 'NONE',  ( 791.9812246680005501, -428.6346026584192259, -361.9419747391813189 ) ) ;
#23297=CARTESIAN_POINT ( 'NONE',  ( 755.3201227861273992, -99.72551174932928575, -345.3687786644892981 ) ) ;
#23306=CARTESIAN_POINT ( 'NONE',  ( 747.6481478633932056, -445.0999726633338582, -353.4146539503763620 ) ) ;
#23307=CARTESIAN_POINT ( 'NONE',  ( 811.0346526505617248, -38.63460265842041963, -323.0537975583478101 ) ) ;
#23309=CARTESIAN_POINT ( 'NONE',  ( 797.6776695296629214, -427.5436935675101040, -357.6776695296636603 ) ) ;
#23310=CARTESIAN_POINT ( 'NONE',  ( 759.7806653035535192, -6.998239022056886860, -324.8639956371181370 ) ) ;
#23313=CARTESIAN_POINT ( 'NONE',  ( 790.9844846989617508, -286.3726999360617356, -317.2208543904092721 ) ) ;
#23314=CARTESIAN_POINT ( 'NONE',  ( 804.7487373415286811, -163.5436935675109567, -364.7487373415288516 ) ) ;
#23317=CARTESIAN_POINT ( 'NONE',  ( 783.6926022324497580, 16.45630643248849267, -313.7971720364932935 ) ) ;
#23319=CARTESIAN_POINT ( 'NONE',  ( 745.1769319972822814, -233.8055962898687028, -346.2694204179732083 ) ) ;
#23324=CARTESIAN_POINT ( 'NONE',  ( 768.0187753319979720, -344.6346026584195101, -318.0580252608186242 ) ) ;
#23328=CARTESIAN_POINT ( 'NONE',  ( 815.3608509340175488, -98.73633629969859271, -341.2497674668889545 ) ) ;
#23329=CARTESIAN_POINT ( 'NONE',  ( 756.7813123517142913, -139.9874144716872024, -329.9779781133712504 ) ) ;
#23331=CARTESIAN_POINT ( 'NONE',  ( 787.4999999999992042, -462.9681489794448339, -370.0000000000000568 ) ) ;
#23332=CARTESIAN_POINT ( 'NONE',  ( 790.8726784830453198, -154.7146871989598935, -362.5472867521010585 ) ) ;
#23334=CARTESIAN_POINT ( 'NONE',  ( 800.1688906516307043, -10.16923265350579442, -369.0717654672308186 ) ) ;
#23335=PRODUCT_DEFINITION ( 'UNKNOWN', '', #45220, #41365 ) ;
#23341=CARTESIAN_POINT ( 'NONE',  ( 799.9636004259356241, -262.9181544815162965, -311.2241431872006956 ) ) ;
#23349=CARTESIAN_POINT ( 'NONE',  ( 804.4086373105744769, -121.6454272087894282, -333.3843516231986541 ) ) ;
#23351=CARTESIAN_POINT ( 'NONE',  ( 788.7366044899766848, -107.9073299311474727, -316.5762568750059813 ) ) ;
#23352=CARTESIAN_POINT ( 'NONE',  ( 800.0135310231082713, -302.0891481129650629, -325.0180583372163028 ) ) ;
#23354=CARTESIAN_POINT ( 'NONE',  ( 762.1405469898971887, -433.5436935675099903, -357.8594530101015607 ) ) ;
#23361=CARTESIAN_POINT ( 'NONE',  ( 807.2620300519052989, -360.0090635724250774, -318.0141637701419768 ) ) ;
#23363=CARTESIAN_POINT ( 'NONE',  ( 801.9419747391806368, -306.4527844766013800, -351.9812246680014027 ) ) ;
#23365=CARTESIAN_POINT ( 'NONE',  ( 776.9254006560222479, -188.1908817542437760, -314.8983024940802125 ) ) ;
#23367=DIRECTION ( 'NONE',  ( 0.000000000000000000, -1.000000000000000000, 0.000000000000000000 ) ) ;
#23368=CARTESIAN_POINT ( 'NONE',  ( 745.7998596910086917, -365.3618753856920875, -332.5602148656461168 ) ) ;
#23373=CARTESIAN_POINT ( 'NONE',  ( 746.8695393053150156, -29.90732993114771787, -327.6429770376306010 ) ) ;
#23375=CARTESIAN_POINT ( 'NONE',  ( 800.2193346964447755, -258.9982390220561115, -355.1360043628815788 ) ) ;
#23379=CARTESIAN_POINT ( 'NONE',  ( 804.9511171171677688, -53.80559628986930676, -335.8780910478229202 ) ) ;
#23384=CARTESIAN_POINT ( 'NONE',  ( 787.4999999999992042, -462.9681489794447771, -309.9999999999998863 ) ) ;
#23388=CARTESIAN_POINT ( 'NONE',  ( 755.8398074228967971, -355.4419599262319593, -333.4516893846970333 ) ) ;
#23391=CARTESIAN_POINT ( 'NONE',  ( 752.4576283171824116, -381.0783235625954717, -317.7880784355627952 ) ) ;
#23396=CARTESIAN_POINT ( 'NONE',  ( 746.8695393053150156, -221.9073299311470464, -327.6429770376306010 ) ) ;
#23399=CARTESIAN_POINT ( 'NONE',  ( 767.8955696845334842, -216.4527844766016926, -362.1676090361161755 ) ) ;
#23401=CARTESIAN_POINT ( 'NONE',  ( 756.3353852180819104, -317.9073299311468190, -331.1735550268788302 ) ) ;
#23402=CARTESIAN_POINT ( 'NONE',  ( 780.5236548040995785, -452.7363362996975411, -314.9735926884559944 ) ) ;
#23410=CARTESIAN_POINT ( 'NONE',  ( 801.5560724626406000, -456.5545181178792404, -326.7756240680316182 ) ) ;
#23411=CARTESIAN_POINT ( 'NONE',  ( 777.0937506421101943, 18.86692508245304367, -309.9999999999999432 ) ) ;
#23413=ORIENTED_EDGE ( 'NONE', *, *, #39098, .T. ) ;
#23414=CARTESIAN_POINT ( 'NONE',  ( 814.8207195650702488, -242.1908817542435770, -336.2433038121456548 ) ) ;
#23418=CARTESIAN_POINT ( 'NONE',  ( 759.9864689768902508, -194.0891481129654039, -354.9819416627836404 ) ) ;
#23419=CARTESIAN_POINT ( 'NONE',  ( 758.6633372737375112, -356.5328690171410813, -326.9102291470432533 ) ) ;
#23420=CARTESIAN_POINT ( 'NONE',  ( 773.7305795820266212, -225.2817908451527273, -374.8230680027170365 ) ) ;
#23422=DIRECTION ( 'NONE',  ( 0.000000000000000000, 0.000000000000000000, -1.000000000000000000 ) ) ;
#23423=CARTESIAN_POINT ( 'NONE',  ( 787.5531968255692163, -69.82724539060775726, -316.1348686366205811 ) ) ;
#23426=CARTESIAN_POINT ( 'NONE',  ( 799.4546378042377910, -417.0783235625954148, -356.1575198192848006 ) ) ;
#23427=CARTESIAN_POINT ( 'NONE',  ( 751.9810565676468741, -266.0891481129651197, -360.9747183278973921 ) ) ;
#23429=DIRECTION ( 'NONE',  ( 1.000000000000000000, 0.000000000000000000, 0.000000000000000000 ) ) ;
#23430=CARTESIAN_POINT ( 'NONE',  ( 801.9419747391806368, -66.45278447660216159, -351.9812246680014027 ) ) ;
#23432=CARTESIAN_POINT ( 'NONE',  ( 807.5423716828161105, -153.0783235625962675, -362.2119215644372048 ) ) ;
#23434=CARTESIAN_POINT ( 'NONE',  ( 745.0891759886404770, -412.2709662947829088, -342.4968714119734159 ) ) ;
#23438=CARTESIAN_POINT ( 'NONE',  ( 771.1735550268778070, -441.1800572038735027, -316.3353852180827630 ) ) ;
#23443=CARTESIAN_POINT ( 'NONE',  ( 761.2382568024794409, -231.6237781080504874, -356.9571628226838129 ) ) ;
#23444=CARTESIAN_POINT ( 'NONE',  ( 781.7834795799800531, -130.8164208402383224, -315.0636971347436202 ) ) ;
#23446=CARTESIAN_POINT ( 'NONE',  ( 761.9338519418445230, -254.5328690171413655, -370.4231160770881957 ) ) ;
#23451=CARTESIAN_POINT ( 'NONE',  ( 791.9812246680005501, -188.6346026584199365, -361.9419747391813189 ) ) ;
#23453=CARTESIAN_POINT ( 'NONE',  ( 772.4837098697144029, -119.3618753856928691, -374.5518280994205611 ) ) ;
#23455=CARTESIAN_POINT ( 'NONE',  ( 788.7366044899766848, -59.90732993114762905, -316.5762568750059813 ) ) ;
#23457=CARTESIAN_POINT ( 'NONE',  ( 766.0291762391763086, -34.91815448151697154, -360.7704444035551319 ) ) ;
#23459=CARTESIAN_POINT ( 'NONE',  ( 755.1538015810308480, -350.1908817542433212, -343.0433043558613804 ) ) ;
#23466=CARTESIAN_POINT ( 'NONE',  ( 755.3028492785439312, -327.2817908451525000, -335.9200461376539693 ) ) ;
#23467=CARTESIAN_POINT ( 'NONE',  ( 804.6798772138708955, -327.7255117493285184, -334.6312213355107019 ) ) ;
#23468=CARTESIAN_POINT ( 'NONE',  ( 752.7379699480933368, -132.0090635724257595, -361.9858362298580232 ) ) ;
#23472=CARTESIAN_POINT ( 'NONE',  ( 766.7756240680305382, -254.5328690171413655, -361.5560724626415663 ) ) ;
#23473=CARTESIAN_POINT ( 'NONE',  ( 809.0717654672305343, -124.9181544815167086, -360.1688906516309885 ) ) ;
#23479=CARTESIAN_POINT ( 'NONE',  ( 758.8095938919644823, -176.0891481129654039, -311.6929314249762797 ) ) ;
#23483=CARTESIAN_POINT ( 'NONE',  ( 812.7932403749906598, -303.1800572038740711, -327.7687537140311633 ) ) ;
#23489=CARTESIAN_POINT ( 'NONE',  ( 813.9316612368132837, -343.4419599262320162, -348.6739635108323228 ) ) ;
#23490=CARTESIAN_POINT ( 'NONE',  ( 800.9747183278959710, -132.9982390220564810, -311.9810565676471583 ) ) ;
#23492=CARTESIAN_POINT ( 'NONE',  ( 767.7687537140311633, -383.9073299311466485, -372.7932403749916830 ) ) ;
#23497=CARTESIAN_POINT ( 'NONE',  ( 798.0661480581538854, -170.5328690171416781, -309.5768839229118043 ) ) ;
#23503=CARTESIAN_POINT ( 'NONE',  ( 798.0661480581538854, -434.5328690171407970, -309.5768839229118043 ) ) ;
#23507=CARTESIAN_POINT ( 'NONE',  ( 786.2694204179717872, -381.2817908451523294, -305.1769319972829067 ) ) ;
#23509=CARTESIAN_POINT ( 'NONE',  ( 801.9419747391806368, -234.4527844766016358, -351.9812246680014027 ) ) ;
#23512=CARTESIAN_POINT ( 'NONE',  ( 763.8424801807145741, -234.0090635724255037, -320.5453621957614700 ) ) ;
#23513=CARTESIAN_POINT ( 'NONE',  ( 785.3687786644884454, -227.3618753856925707, -315.3201227861279676 ) ) ;
#23514=CARTESIAN_POINT ( 'NONE',  ( 804.6798772138710092, -423.7255117493282341, -334.6312213355106451 ) ) ;
#23516=CARTESIAN_POINT ( 'NONE',  ( 781.7834795799800531, -106.8164208402383935, -315.0636971347436202 ) ) ;
#23526=CARTESIAN_POINT ( 'NONE',  ( 793.5525998758768083, -439.0999726633339719, -372.6845335610516941 ) ) ;
#23527=CARTESIAN_POINT ( 'NONE',  ( 747.2067596250078623, -75.18005720387485269, -352.2312462859687230 ) ) ;
#23529=CARTESIAN_POINT ( 'NONE',  ( 804.9363028652555840, -424.2709662947829088, -338.2165204200192079 ) ) ;
#23530=CARTESIAN_POINT ( 'NONE',  ( 778.1981804954715471, -34.27096629478407408, -314.8072714833591021 ) ) ;
#23532=CARTESIAN_POINT ( 'NONE',  ( 781.7834795799800531, 13.18357915976123174, -315.0636971347436202 ) ) ;
#23533=CARTESIAN_POINT ( 'NONE',  ( 804.8461984189677878, -290.1908817542434349, -336.9566956441385628 ) ) ;
#23534=CARTESIAN_POINT ( 'NONE',  ( 777.4774526936600978, -202.2709662947834772, -304.7301800767027657 ) ) ;
#23539=CARTESIAN_POINT ( 'NONE',  ( 810.1134526219336749, -224.5328690171415076, -357.8822607201570349 ) ) ;
#23540=VECTOR ( 'NONE', #13264, 1000.000000000000000 ) ;
#23542=CARTESIAN_POINT ( 'NONE',  ( 751.9810565676468741, -290.0891481129650629, -360.9747183278973921 ) ) ;
#23543=LINE ( 'NONE', #23082, #33876 ) ;
#23546=CARTESIAN_POINT ( 'NONE',  ( 792.1044303154645831, -348.4527844766012663, -317.8323909638837677 ) ) ;
#23548=CARTESIAN_POINT ( 'NONE',  ( 745.5313806188320314, -87.28179084515316788, -333.7943932421247268 ) ) ;
#23549=CARTESIAN_POINT ( 'NONE',  ( 795.9930595647434757, -171.0783235625962106, -320.7433823573372820 ) ) ;
#23555=CARTESIAN_POINT ( 'NONE',  ( 794.9819416627830151, -60.99823902205671544, -319.9864689768909898 ) ) ;
#23556=CARTESIAN_POINT ( 'NONE',  ( 796.7845633553578182, -153.6237781080508000, -358.5707757039688204 ) ) ;
#23558=CARTESIAN_POINT ( 'NONE',  ( 810.1134526219336749, 15.46713098285775878, -357.8822607201570349 ) ) ;
#23564=CARTESIAN_POINT ( 'NONE',  ( 757.7880784355613741, -258.0090635724253616, -312.4576283171834916 ) ) ;
#23571=CARTESIAN_POINT ( 'NONE',  ( 760.7433823573367135, -108.0090635724258448, -355.9930595647440441 ) ) ;
#23572=CARTESIAN_POINT ( 'NONE',  ( 803.4237431249931660, -111.1800572038747532, -331.2633955100225194 ) ) ;
#23573=CARTESIAN_POINT ( 'NONE',  ( 804.4286716492782716, -305.3618753856922581, -345.3141322388244703 ) ) ;
#23575=CARTESIAN_POINT ( 'NONE',  ( 794.9819416627830151, -444.9982390220554862, -319.9864689768909898 ) ) ;
#23584=CARTESIAN_POINT ( 'NONE',  ( 788.6739635108323228, -343.6454272087887603, -373.9316612368139090 ) ) ;
#23586=CARTESIAN_POINT ( 'NONE',  ( 756.5762568750052424, -339.1800572038740142, -348.7366044899774238 ) ) ;
#23588=CARTESIAN_POINT ( 'NONE',  ( 804.8461984189677878, -170.1908817542438328, -336.9566956441385628 ) ) ;
#23591=CARTESIAN_POINT ( 'NONE',  ( 747.2067596250078623, -387.1800572038738437, -352.2312462859687230 ) ) ;
#23596=CARTESIAN_POINT ( 'NONE',  ( 744.7301800767019131, -4.816420840238714085, -337.4774526936615757 ) ) ;
#23597=CARTESIAN_POINT ( 'NONE',  ( 788.8264449731200330, -237.1800572038742985, -363.6646147819171233 ) ) ;
#23601=CARTESIAN_POINT ( 'NONE',  ( 795.9930595647434757, -51.07832356259657303, -320.7433823573372820 ) ) ;
#23608=CARTESIAN_POINT ( 'NONE',  ( 803.6646147819161570, -65.90732993114758642, -348.8264449731210561 ) ) ;
#23609=CARTESIAN_POINT ( 'NONE',  ( 764.0069404352550464, -375.0783235625955285, -359.2566176426627180 ) ) ;
#23612=CARTESIAN_POINT ( 'NONE',  ( 745.1769319972822814, -353.8055962898683333, -346.2694204179732083 ) ) ;
#23617=CARTESIAN_POINT ( 'NONE',  ( 745.0891759886404770, -220.2709662947834772, -342.4968714119734159 ) ) ;
#23620=CARTESIAN_POINT ( 'NONE',  ( 781.8018195045267476, -214.2709662947834772, -365.1927285166407273 ) ) ;
#23622=CARTESIAN_POINT ( 'NONE',  ( 767.8955696845333705, -312.4527844766012663, -362.1676090361162323 ) ) ;
#23623=CARTESIAN_POINT ( 'NONE',  ( 757.4527132478984868, -448.3726999360611103, -329.1273215169538844 ) ) ;
#23630=CARTESIAN_POINT ( 'NONE',  ( 799.2566176426618085, -456.0090635724247932, -324.0069404352559559 ) ) ;
#23634=CARTESIAN_POINT ( 'NONE',  ( 795.8262568251477660, -238.3726999360617640, -308.3538107759623585 ) ) ;
#23637=CARTESIAN_POINT ( 'NONE',  ( 805.1927285166397041, -208.8164208402380666, -341.8018195045277707 ) ) ;
#23638=CARTESIAN_POINT ( 'NONE',  ( 794.1144889064781864, -370.1692326535045936, -360.9840315886528401 ) ) ;
#23639=CARTESIAN_POINT ( 'NONE',  ( 764.1737431748507561, -250.3726999360618208, -371.6461892240376415 ) ) ;
#23642=CARTESIAN_POINT ( 'NONE',  ( 786.5483106153019435, -79.64542720878957027, -364.1601925771022366 ) ) ;
#23646=CARTESIAN_POINT ( 'NONE',  ( 805.0264073115434940, -438.3510508353226669, -339.4763451958999099 ) ) ;
#23647=CARTESIAN_POINT ( 'NONE',  ( 746.8695393053151292, -269.9073299311469327, -327.6429770376306578 ) ) ;
#23650=CARTESIAN_POINT ( 'NONE',  ( 767.8955696845333705, -48.45278447660219712, -362.1676090361162323 ) ) ;
#23652=CARTESIAN_POINT ( 'NONE',  ( 795.6651683502461765, -154.7146871989598935, -371.3240766477733814 ) ) ;
#23654=CARTESIAN_POINT ( 'NONE',  ( 796.9462024416508257, -396.4527844766010389, -308.9653473494370246 ) ) ;
#23658=CARTESIAN_POINT ( 'NONE',  ( 755.3201227861273992, -435.7255117493282341, -345.3687786644892981 ) ) ;
#23664=CARTESIAN_POINT ( 'NONE',  ( 763.2154366446407039, -261.6237781080504305, -321.4292242960311228 ) ) ;
#23666=CARTESIAN_POINT ( 'NONE',  ( 805.9055244015594326, -267.6237781080504305, -315.8990559732753240 ) ) ;
#23672=CARTESIAN_POINT ( 'NONE',  ( 789.9200121543843807, -25.98741447168755769, -317.0176451133914384 ) ) ;
#23673=CARTESIAN_POINT ( 'NONE',  ( 757.8323909638827445, -170.6346026584199649, -352.1044303154654358 ) ) ;
#23675=CARTESIAN_POINT ( 'NONE',  ( 755.2512626584698410, -127.5436935675110561, -315.2512626584710915 ) ) ;
#23677=CARTESIAN_POINT ( 'NONE',  ( 802.1676090361155502, -110.6346026584201923, -327.8955696845344505 ) ) ;
#23679=CARTESIAN_POINT ( 'NONE',  ( 755.3028492785439312, -39.28179084515331709, -335.9200461376539693 ) ) ;
#23680=CARTESIAN_POINT ( 'NONE',  ( 779.4763451958990572, -344.7363362996978253, -365.0264073115438919 ) ) ;
#23688=CARTESIAN_POINT ( 'NONE',  ( 784.1219089521767955, -357.2817908451523294, -315.0488828828318333 ) ) ;
#23689=CARTESIAN_POINT ( 'NONE',  ( 781.7834795799800531, -322.8164208402377540, -315.0636971347436202 ) ) ;
#23690=CARTESIAN_POINT ( 'NONE',  ( 814.4686193811664907, -147.2817908451529547, -346.2056067578752732 ) ) ;
#23694=CARTESIAN_POINT ( 'NONE',  ( 786.6156483768007774, -265.4419599262323004, -315.5913626894246136 ) ) ;
#23695=CARTESIAN_POINT ( 'NONE',  ( 781.2370466360911223, -140.7363362996984506, -304.9990715423533629 ) ) ;
#23701=CARTESIAN_POINT ( 'NONE',  ( 755.2512626584698410, -175.5436935675108998, -315.2512626584710915 ) ) ;
#23704=CARTESIAN_POINT ( 'NONE',  ( 754.9967657858570647, -313.5436935675102745, -365.0032342141425374 ) ) ;
#23711=CARTESIAN_POINT ( 'NONE',  ( 815.1787889125755555, -390.8965053807772279, -343.7953271457877804 ) ) ;
#23712=CARTESIAN_POINT ( 'NONE',  ( 777.4774526936600978, -130.2709662947837899, -304.7301800767027657 ) ) ;
#23714=CARTESIAN_POINT ( 'NONE',  ( 754.9967657858570647, -385.5436935675102745, -365.0032342141425374 ) ) ;
#23718=CARTESIAN_POINT ( 'NONE',  ( 810.1134526219336749, -152.5328690171416781, -357.8822607201570349 ) ) ;
#23723=CARTESIAN_POINT ( 'NONE',  ( 786.6156483768007774, -1.441959926233096656, -315.5913626894246136 ) ) ;
#23725=CARTESIAN_POINT ( 'NONE',  ( 800.9747183278959710, -12.99823902205686821, -311.9810565676471583 ) ) ;
#23729=CARTESIAN_POINT ( 'NONE',  ( 785.3687786644884454, -179.3618753856927128, -315.3201227861279676 ) ) ;
#23730=CARTESIAN_POINT ( 'NONE',  ( 755.8990559732751535, -395.4636090269705164, -365.9055244015606831 ) ) ;
#23731=CARTESIAN_POINT ( 'NONE',  ( 771.1735550268778070, -249.1800572038742416, -316.3353852180827630 ) ) ;
#23735=CARTESIAN_POINT ( 'NONE',  ( 804.6971507214547046, -267.2817908451526137, -344.0799538623459739 ) ) ;
#23736=CARTESIAN_POINT ( 'NONE',  ( 788.8264449731200330, -213.1800572038743553, -363.6646147819171233 ) ) ;
#23738=CARTESIAN_POINT ( 'NONE',  ( 755.3201227861273992, -411.7255117493282910, -345.3687786644892981 ) ) ;
#23747=CARTESIAN_POINT ( 'NONE',  ( 815.3608509340175488, -434.7363362996975980, -341.2497674668889545 ) ) ;
#23748=CARTESIAN_POINT ( 'NONE',  ( 758.8095938919644823, -80.08914811296574499, -311.6929314249762797 ) ) ;
#23750=CARTESIAN_POINT ( 'NONE',  ( 762.3223304703356007, -415.5436935675102177, -322.3223304703362828 ) ) ;
#23751=CARTESIAN_POINT ( 'NONE',  ( 774.6312213355098493, -47.36187538569312494, -364.6798772138717482 ) ) ;
#23753=CARTESIAN_POINT ( 'NONE',  ( 803.4237431249931660, 8.819942796124882634, -331.2633955100225194 ) ) ;
#23754=CARTESIAN_POINT ( 'NONE',  ( 769.9779781133707957, -283.0999726633344267, -316.7813123517150871 ) ) ;
#23755=CARTESIAN_POINT ( 'NONE',  ( 787.4397851343537695, -213.7255117493289731, -374.2001403089903988 ) ) ;
#23761=CARTESIAN_POINT ( 'NONE',  ( 773.7943932421234194, -263.8055962898686175, -305.5313806188329409 ) ) ;
#23763=CARTESIAN_POINT ( 'NONE',  ( 767.6429770376289525, -273.1800572038742985, -306.8695393053162093 ) ) ;
#23767=CARTESIAN_POINT ( 'NONE',  ( 802.1676090361156639, -350.6346026584192828, -327.8955696845344505 ) ) ;
#23769=CARTESIAN_POINT ( 'NONE',  ( 761.9338519418445230, -38.53286901714206891, -370.4231160770881957 ) ) ;
#23770=CARTESIAN_POINT ( 'NONE',  ( 800.7704444035546203, -148.1692326535053610, -326.0291762391768771 ) ) ;
#23774=CARTESIAN_POINT ( 'NONE',  ( 771.2633955100217236, -71.90732993114760063, -363.4237431249939618 ) ) ;
#23775=CARTESIAN_POINT ( 'NONE',  ( 787.6308680596127942, -155.2601417444144261, -364.1105419155492768 ) ) ;
#23778=EDGE_CURVE ( 'NONE', #38196, #9202, #31415, .T. ) ;
#23779=CARTESIAN_POINT ( 'NONE',  ( 758.0141637701419768, 8.921676437403235127, -367.2620300519063790 ) ) ;
#23785=CARTESIAN_POINT ( 'NONE',  ( 764.1737431748507561, -322.3726999360615082, -371.6461892240376415 ) ) ;
#23791=CARTESIAN_POINT ( 'NONE',  ( 769.0155153010367712, -106.3726999360621903, -362.7791456095907279 ) ) ;
#23792=CARTESIAN_POINT ( 'NONE',  ( 781.8018195045266339, -118.2709662947837899, -365.1927285166406705 ) ) ;
#23794=CARTESIAN_POINT ( 'NONE',  ( 791.9812246680005501, -308.6346026584195670, -361.9419747391813189 ) ) ;
#23796=CARTESIAN_POINT ( 'NONE',  ( 800.0135310231082713, -446.0891481129646081, -325.0180583372163028 ) ) ;
#23799=CARTESIAN_POINT ( 'NONE',  ( 791.8656671112827325, -456.3250812000245560, -367.5545208264068719 ) ) ;
#23803=CARTESIAN_POINT ( 'NONE',  ( 746.4236121716829757, -327.8272453906069472, -328.8385539511384650 ) ) ;
#23806=CARTESIAN_POINT ( 'NONE',  ( 803.4237431249931660, -327.1800572038741279, -331.2633955100225194 ) ) ;
#23807=ADVANCED_FACE ( 'NONE', ( #39403 ), #4061, .T. ) ;
#23808=CARTESIAN_POINT ( 'NONE',  ( 759.9999999999992042, -462.9681489794448339, -370.0000000000000568 ) ) ;
#23809=CARTESIAN_POINT ( 'NONE',  ( 790.0220218866281812, -199.0999726633346825, -363.2186876482849129 ) ) ;
#23812=CARTESIAN_POINT ( 'NONE',  ( 767.6429770376291799, -369.1800572038739006, -306.8695393053162093 ) ) ;
#23813=FACE_OUTER_BOUND ( 'NONE', #41053, .T. ) ;
#23815=DIRECTION ( 'NONE',  ( 0.000000000000000000, 0.000000000000000000, -1.000000000000000000 ) ) ;
#23817=CARTESIAN_POINT ( 'NONE',  ( 745.4481719005789273, -3.725511749329622813, -347.5162901302853129 ) ) ;
#23818=CARTESIAN_POINT ( 'NONE',  ( 774.6312213355099630, -239.3618753856924570, -364.6798772138717482 ) ) ;
#23823=CARTESIAN_POINT ( 'NONE',  ( 787.6308680596127942, -35.26014174441480264, -364.1105419155492768 ) ) ;
#23832=CARTESIAN_POINT ( 'NONE',  ( 784.0799538623451781, -371.8055962898682765, -364.6971507214555572 ) ) ;
#23835=CARTESIAN_POINT ( 'NONE',  ( 744.8212110874229666, -354.8965053807774552, -336.2046728542121627 ) ) ;
#23842=EDGE_CURVE ( 'NONE', #17589, #20167, #42468, .T. ) ;
#23843=CARTESIAN_POINT ( 'NONE',  ( 796.9462024416508257, -228.4527844766015789, -308.9653473494370246 ) ) ;
#23846=CARTESIAN_POINT ( 'NONE',  ( 758.0580252608178853, -222.4527844766016642, -328.0187753319985404 ) ) ;
#23848=CARTESIAN_POINT ( 'NONE',  ( 778.2165204200184689, -334.8164208402376403, -364.9363028652563230 ) ) ;
#23849=CARTESIAN_POINT ( 'NONE',  ( 804.8461984189677878, -458.1908817542429802, -336.9566956441385628 ) ) ;
#23855=CARTESIAN_POINT ( 'NONE',  ( 768.0187753319979720, 15.36539734157940629, -318.0580252608186242 ) ) ;
#23856=CARTESIAN_POINT ( 'NONE',  ( 799.9999999999993179, -462.9681489794448339, -370.0000000000000568 ) ) ;
#23858=VERTEX_POINT ( 'NONE', #36829 ) ;
#23859=CARTESIAN_POINT ( 'NONE',  ( 745.1792804349281596, -254.1908817542435770, -343.7566961878542884 ) ) ;
#23863=CARTESIAN_POINT ( 'NONE',  ( 794.9819416627830151, -228.9982390220561683, -319.9864689768909898 ) ) ;
#23864=CARTESIAN_POINT ( 'NONE',  ( 779.4709603349208464, -384.3510508353227806, -314.7162404726379918 ) ) ;
#23865=CARTESIAN_POINT ( 'NONE',  ( 805.6418435158337843, -245.4636090269709143, -363.8556311672236916 ) ) ;
#23868=CARTESIAN_POINT ( 'NONE',  ( 799.2566176426618085, -72.00906357242594424, -324.0069404352559559 ) ) ;
#23872=CARTESIAN_POINT ( 'NONE',  ( 744.7301800767020268, -268.8164208402378677, -337.4774526936615189 ) ) ;
#23875=CARTESIAN_POINT ( 'NONE',  ( 805.1927285166397041, -40.81642084023859951, -341.8018195045277707 ) ) ;
#23878=CARTESIAN_POINT ( 'NONE',  ( 783.7566961878529810, -168.8965053807780237, -305.1792804349288417 ) ) ;
#23880=CARTESIAN_POINT ( 'NONE',  ( 759.0252816721024374, -408.9982390220556567, -368.0189434323527280 ) ) ;
#23884=CARTESIAN_POINT ( 'NONE',  ( 764.8639956371174549, -440.0891481129644944, -319.7806653035542013 ) ) ;
#23890=ORIENTED_EDGE ( 'NONE', *, *, #24119, .T. ) ;
#23891=CARTESIAN_POINT ( 'NONE',  ( 800.7704444035546203, -244.1692326535050768, -326.0291762391768771 ) ) ;
#23893=CARTESIAN_POINT ( 'NONE',  ( 797.8594530101008786, -133.5436935675110135, -322.1405469898980982 ) ) ;
#23896=CARTESIAN_POINT ( 'NONE',  ( 803.8556311672234642, -273.6237781080504305, -365.6418435158340117 ) ) ;
#23901=CARTESIAN_POINT ( 'NONE',  ( 759.2295555964440155, -40.16923265350570915, -353.9708237608231229 ) ) ;
#23902=CARTESIAN_POINT ( 'NONE',  ( 788.8264449731200330, -165.1800572038745258, -363.6646147819171233 ) ) ;
#23905=CARTESIAN_POINT ( 'NONE',  ( 759.0252816721024374, -96.99823902205660886, -368.0189434323527280 ) ) ;
#23906=CARTESIAN_POINT ( 'NONE',  ( 785.3141322388236176, -93.72551174932934259, -364.4286716492789537 ) ) ;
#23908=CARTESIAN_POINT ( 'NONE',  ( 796.9571628226829034, -47.46360902697148987, -321.2382568024804641 ) ) ;
#23909=CARTESIAN_POINT ( 'NONE',  ( 796.9571628226829034, -359.4636090269705164, -321.2382568024804641 ) ) ;
#23910=VECTOR ( 'NONE', #27903, 1000.000000000000000 ) ;
#23916=CARTESIAN_POINT ( 'NONE',  ( 763.0428371773158460, -371.4636090269705164, -358.7617431975195359 ) ) ;
#23917=CARTESIAN_POINT ( 'NONE',  ( 785.3687786644884454, -371.3618753856919739, -315.3201227861279676 ) ) ;
#23918=CARTESIAN_POINT ( 'NONE',  ( 814.8207195650702488, -122.1908817542439749, -336.2433038121456548 ) ) ;
#23922=CARTESIAN_POINT ( 'NONE',  ( 772.3691319403857278, -263.2601417444141134, -315.8894580844506663 ) ) ;
#23923=CARTESIAN_POINT ( 'NONE',  ( 814.2805881961230625, -169.6454272087892718, -331.2368401574024119 ) ) ;
#23930=CARTESIAN_POINT ( 'NONE',  ( 814.9108240113580450, -184.2709662947835909, -337.5031285880265273 ) ) ;
#23934=CARTESIAN_POINT ( 'NONE',  ( 746.8695393053150156, -317.9073299311468190, -327.6429770376306010 ) ) ;
#23940=CARTESIAN_POINT ( 'NONE',  ( 812.6845335610512393, -367.9874144716865203, -353.5525998758768651 ) ) ;
#23941=CARTESIAN_POINT ( 'NONE',  ( 782.5225473063381969, -118.2709662947837899, -375.2698199232970637 ) ) ;
#23944=CARTESIAN_POINT ( 'NONE',  ( 808.0189434323515343, -398.0891481129647218, -319.0252816721025511 ) ) ;
#23950=CARTESIAN_POINT ( 'NONE',  ( 756.1443688327750579, -165.6237781080507716, -314.3581564841659315 ) ) ;
#23956=CARTESIAN_POINT ( 'NONE',  ( 796.9462024416508257, -12.45278447660232146, -308.9653473494370246 ) ) ;
#23961=CARTESIAN_POINT ( 'NONE',  ( 747.6481478633932056, -397.0999726633340288, -353.4146539503763620 ) ) ;
#23963=CARTESIAN_POINT ( 'NONE',  ( 768.0187753319979720, -248.6346026584197659, -318.0580252608186242 ) ) ;
#23966=CARTESIAN_POINT ( 'NONE',  ( 805.2837595273609850, -242.7363362996980811, -340.5290396650784714 ) ) ;
#23967=CARTESIAN_POINT ( 'NONE',  ( 755.5713283507202505, -245.3618753856925139, -334.6858677611754729 ) ) ;
#23968=CARTESIAN_POINT ( 'NONE',  ( 764.8639956371174549, -416.0891481129646650, -319.7806653035542581 ) ) ;
#23969=CARTESIAN_POINT ( 'NONE',  ( 762.1405469898971887, -73.54369356751118403, -357.8594530101015607 ) ) ;
#23974=CARTESIAN_POINT ( 'NONE',  ( 814.2805881961230625, -49.64542720878965554, -331.2368401574024119 ) ) ;
#23981=CARTESIAN_POINT ( 'NONE',  ( 805.2837595273609850, -26.73633629969882008, -340.5290396650784714 ) ) ;
#23982=CARTESIAN_POINT ( 'NONE',  ( 749.2812353651451076, -78.45278447660211896, -323.2262854647983090 ) ) ;
#23984=CARTESIAN_POINT ( 'NONE',  ( 778.2165204200184689, -430.8164208402374129, -364.9363028652563230 ) ) ;
#23985=CARTESIAN_POINT ( 'NONE',  ( 802.1676090361155502, -38.63460265842041963, -327.8955696845344505 ) ) ;
#23987=CARTESIAN_POINT ( 'NONE',  ( 796.9462024416508257, -204.4527844766016926, -308.9653473494370246 ) ) ;
#23993=CARTESIAN_POINT ( 'NONE',  ( 808.7758568127978833, -268.1692326535049347, -320.0363995740631822 ) ) ;
#23996=CARTESIAN_POINT ( 'NONE',  ( 792.3570229623688874, -285.1800572038740711, -373.1304606946836202 ) ) ;
#24000=CARTESIAN_POINT ( 'NONE',  ( 801.9419747391806368, -354.4527844766012095, -351.9812246680014027 ) ) ;
#24003=CARTESIAN_POINT ( 'NONE',  ( 788.8264449731200330, -189.1800572038744122, -363.6646147819171233 ) ) ;
#24004=CARTESIAN_POINT ( 'NONE',  ( 808.7758568127978833, -52.16923265350567362, -320.0363995740631822 ) ) ;
#24005=CARTESIAN_POINT ( 'NONE',  ( 754.9735926884551418, -138.3510508353236048, -340.5236548041000333 ) ) ;
#24009=CARTESIAN_POINT ( 'NONE',  ( 774.6858677611749044, -57.72551174932945628, -315.5713283507209894 ) ) ;
#24010=CARTESIAN_POINT ( 'NONE',  ( 755.8398074228967971, -163.4419599262325846, -333.4516893846970333 ) ) ;
#24012=AXIS2_PLACEMENT_3D ( 'NONE', #32238, #11446, #7754 ) ;
#24014=CARTESIAN_POINT ( 'NONE',  ( 746.7653713866222915, 6.739858255585061464, -351.0478386215610271 ) ) ;
#24021=CARTESIAN_POINT ( 'NONE',  ( 776.2046728542105711, -308.1908817542434349, -304.8212110874238761 ) ) ;
#24025=CARTESIAN_POINT ( 'NONE',  ( 796.9571628226829034, -167.4636090269711133, -321.2382568024804641 ) ) ;
#24026=CARTESIAN_POINT ( 'NONE',  ( 762.1405469898971887, -121.5436935675110419, -357.8594530101015607 ) ) ;
#24027=CARTESIAN_POINT ( 'NONE',  ( 767.8955696845334842, -312.4527844766013800, -362.1676090361161755 ) ) ;
#24035=CARTESIAN_POINT ( 'NONE',  ( 814.4686193811664907, -363.2817908451523294, -346.2056067578752732 ) ) ;
#24040=CARTESIAN_POINT ( 'NONE',  ( 788.7366044899766848, -323.9073299311468190, -316.5762568750059813 ) ) ;
#24042=CARTESIAN_POINT ( 'NONE',  ( 798.5707757039680246, -197.4636090269709996, -356.7845633553585003 ) ) ;
#24044=EDGE_CURVE ( 'NONE', #17589, #10014, #5180, .T. ) ;
#24046=CARTESIAN_POINT ( 'NONE',  ( 754.9967657858570647, -433.5436935675100472, -365.0032342141425943 ) ) ;
#24051=CARTESIAN_POINT ( 'NONE',  ( 759.0252816721024374, -24.99823902205683268, -368.0189434323527280 ) ) ;
#24053=CARTESIAN_POINT ( 'NONE',  ( 759.7806653035534055, -246.9982390220560546, -324.8639956371180801 ) ) ;
#24057=CARTESIAN_POINT ( 'NONE',  ( 766.4474001241216001, -19.09997266333520116, -307.3154664389482491 ) ) ;
#24058=CARTESIAN_POINT ( 'NONE',  ( 799.4546378042377910, -57.07832356259658013, -356.1575198192848006 ) ) ;
#24066=CARTESIAN_POINT ( 'NONE',  ( 758.0580252608178853, -78.45278447660211896, -328.0187753319985404 ) ) ;
#24068=CARTESIAN_POINT ( 'NONE',  ( 780.5290396650775619, -348.3510508353228943, -365.2837595273619513 ) ) ;
#24072=CARTESIAN_POINT ( 'NONE',  ( 812.6845335610512393, -367.9874144716865203, -353.5525998758768651 ) ) ;
#24080=CARTESIAN_POINT ( 'NONE',  ( 811.0346526505616112, -206.6346026584198512, -323.0537975583477532 ) ) ;
#24083=CARTESIAN_POINT ( 'NONE',  ( 804.4286716492782716, -209.3618753856926276, -345.3141322388244703 ) ) ;
#24085=CARTESIAN_POINT ( 'NONE',  ( 794.9819416627830151, -324.9982390220559409, -319.9864689768909898 ) ) ;
#24086=CARTESIAN_POINT ( 'NONE',  ( 755.0636971347428243, -4.270966294784170003, -341.7834795799807353 ) ) ;
#24091=CARTESIAN_POINT ( 'NONE',  ( 801.9419747391806368, 5.547215523397618142, -351.9812246680014027 ) ) ;
#24093=PLANE ( 'NONE',  #36628 ) ;
#24095=CARTESIAN_POINT ( 'NONE',  ( 771.3260364891663130, -235.6454272087890729, -306.0683387631859773 ) ) ;
#24099=CARTESIAN_POINT ( 'NONE',  ( 802.1676090361156639, -230.6346026584197659, -327.8955696845344505 ) ) ;
#24101=CARTESIAN_POINT ( 'NONE',  ( 794.1144889064781864, -394.1692326535045368, -360.9840315886528401 ) ) ;
#24104=CARTESIAN_POINT ( 'NONE',  ( 790.9844846989617508, -94.37269993606224716, -317.2208543904092721 ) ) ;
#24109=CARTESIAN_POINT ( 'NONE',  ( 815.0009284576459549, 17.64894916467593688, -338.7629533639073429 ) ) ;
#24110=CARTESIAN_POINT ( 'NONE',  ( 787.5162901302840055, -275.3618753856924286, -305.4481719005793252 ) ) ;
#24111=PLANE ( 'NONE',  #20217 ) ;
#24113=CARTESIAN_POINT ( 'NONE',  ( 802.1676090361156639, -86.63460265842023489, -327.8955696845344505 ) ) ;
#24116=CARTESIAN_POINT ( 'NONE',  ( 793.4146539503750546, -169.9874144716871172, -307.6481478633938877 ) ) ;
#24118=CARTESIAN_POINT ( 'NONE',  ( 814.2001403089898304, -401.3618753856920307, -347.4397851343538264 ) ) ;
#24119=EDGE_CURVE ( 'NONE', #11372, #38196, #29453, .T. ) ;
#24125=CARTESIAN_POINT ( 'NONE',  ( 800.0135310231082713, -422.0891481129647218, -325.0180583372163028 ) ) ;
#24131=CARTESIAN_POINT ( 'NONE',  ( 793.2243759319678702, -242.5328690171414507, -318.4439275373583200 ) ) ;
#24133=CARTESIAN_POINT ( 'NONE',  ( 798.0661480581538854, -266.5328690171413655, -309.5768839229118043 ) ) ;
#24141=CARTESIAN_POINT ( 'NONE',  ( 780.5290396650775619, -36.35105083532390324, -365.2837595273619513 ) ) ;
#24142=CARTESIAN_POINT ( 'NONE',  ( 762.1405469898971887, -193.5436935675108714, -357.8594530101015607 ) ) ;
#24144=CARTESIAN_POINT ( 'NONE',  ( 767.7687537140311633, -119.9073299311474443, -372.7932403749916830 ) ) ;
#24145=CARTESIAN_POINT ( 'NONE',  ( 765.0180583372156207, -120.9982390220565378, -360.0135310231089534 ) ) ;
#24147=CARTESIAN_POINT ( 'NONE',  ( 755.1538015810308480, -38.19088175424422360, -343.0433043558613804 ) ) ;
#24149=CARTESIAN_POINT ( 'NONE',  ( 784.1219089521767955, -357.2817908451523294, -315.0488828828318333 ) ) ;
#24157=CARTESIAN_POINT ( 'NONE',  ( 783.0745993439762742, -344.1908817542433212, -365.1016975059196739 ) ) ;
#24158=CARTESIAN_POINT ( 'NONE',  ( 781.7834795799800531, -346.8164208402376971, -315.0636971347436202 ) ) ;
#24159=CARTESIAN_POINT ( 'NONE',  ( 814.2805881961230625, -121.6454272087894282, -331.2368401574024119 ) ) ;
#24160=ADVANCED_FACE ( 'NONE', ( #14589 ), #16487, .T. ) ;
#24164=CARTESIAN_POINT ( 'NONE',  ( 787.4999999999992042, -462.9681489794447202, -270.0000000000000568 ) ) ;
#24166=CARTESIAN_POINT ( 'NONE',  ( 754.8983024940795303, -282.8965053807776258, -336.9254006560228163 ) ) ;
#24167=CARTESIAN_POINT ( 'NONE',  ( 814.4686193811664907, -147.2817908451529547, -346.2056067578752732 ) ) ;
#24173=CARTESIAN_POINT ( 'NONE',  ( 813.1304606946831655, -161.9073299311472738, -352.3570229623691716 ) ) ;
#24176=CARTESIAN_POINT ( 'NONE',  ( 751.9810565676468741, -314.0891481129650629, -360.9747183278973921 ) ) ;
#24178=DIRECTION ( 'NONE',  ( 0.000000000000000000, 0.000000000000000000, -1.000000000000000000 ) ) ;
#24183=CARTESIAN_POINT ( 'NONE',  ( 746.7653713866222915, -377.2601417444137724, -351.0478386215610271 ) ) ;
#24185=CARTESIAN_POINT ( 'NONE',  ( 772.4837098697144029, -119.3618753856928691, -374.5518280994205611 ) ) ;
#24187=CARTESIAN_POINT ( 'NONE',  ( 804.7487373415286811, -403.5436935675101608, -364.7487373415288516 ) ) ;
#24188=DIRECTION ( 'NONE',  ( 0.000000000000000000, 0.000000000000000000, 1.000000000000000000 ) ) ;
#24191=CARTESIAN_POINT ( 'NONE',  ( 759.8311093483677041, -142.1692326535054178, -310.9282345327691814 ) ) ;
#24197=CARTESIAN_POINT ( 'NONE',  ( 814.9108240113580450, -16.27096629478413092, -337.5031285880265273 ) ) ;
#24200=CARTESIAN_POINT ( 'NONE',  ( 747.6481478633932056, -421.0999726633340288, -353.4146539503763620 ) ) ;
#24202=CARTESIAN_POINT ( 'NONE',  ( 778.2165204200184689, -262.8164208402379245, -364.9363028652563230 ) ) ;
#24205=CARTESIAN_POINT ( 'NONE',  ( 804.4086373105744769, -241.6454272087890729, -333.3843516231986541 ) ) ;
#24206=CARTESIAN_POINT ( 'NONE',  ( 755.3201227861273992, -267.7255117493286320, -345.3687786644892981 ) ) ;
#24207=CARTESIAN_POINT ( 'NONE',  ( 774.6858677611749044, -441.7255117493282910, -315.5713283507209894 ) ) ;
#24208=CARTESIAN_POINT ( 'NONE',  ( 771.2633955100217236, -71.90732993114760063, -363.4237431249939618 ) ) ;
#24210=VERTEX_POINT ( 'NONE', #30568 ) ;
#24215=CARTESIAN_POINT ( 'NONE',  ( 750.9282345327678740, -40.91815448151695023, -319.8311093483690115 ) ) ;
#24221=CARTESIAN_POINT ( 'NONE',  ( 783.0745993439762742, -8.190881754244330182, -365.1016975059196739 ) ) ;
#24222=CARTESIAN_POINT ( 'NONE',  ( 751.6929314249750860, -54.99823902205672965, -318.8095938919659034 ) ) ;
#24224=CARTESIAN_POINT ( 'NONE',  ( 804.4286716492782716, -449.3618753856918602, -345.3141322388244703 ) ) ;
#24225=CARTESIAN_POINT ( 'NONE',  ( 803.4237431249931660, -39.18005720387496638, -331.2633955100225194 ) ) ;
#24227=CARTESIAN_POINT ( 'NONE',  ( 800.9747183278959710, -204.9982390220562820, -311.9810565676471583 ) ) ;
#24232=CARTESIAN_POINT ( 'NONE',  ( 781.2497674668890113, -276.3510508353231785, -375.3608509340180603 ) ) ;
#24234=CARTESIAN_POINT ( 'NONE',  ( 811.0346526505616112, -278.6346026584196807, -323.0537975583477532 ) ) ;
#24235=DIRECTION ( 'NONE',  ( 0.000000000000000000, 0.000000000000000000, 1.000000000000000000 ) ) ;
#24238=CARTESIAN_POINT ( 'NONE',  ( 788.7366044899766848, -395.9073299311465348, -316.5762568750059813 ) ) ;
#24240=CARTESIAN_POINT ( 'NONE',  ( 745.1769319972822814, -65.80559628986925702, -346.2694204179732083 ) ) ;
#24241=CARTESIAN_POINT ( 'NONE',  ( 803.8651313633788504, -173.2601417444143692, -332.4468031744301015 ) ) ;
#24246=CARTESIAN_POINT ( 'NONE',  ( 778.1981804954714335, -58.27096629478398171, -314.8072714833589885 ) ) ;
#24247=CARTESIAN_POINT ( 'NONE',  ( 784.0799538623451781, -203.8055962898688449, -364.6971507214555572 ) ) ;
#24250=CARTESIAN_POINT ( 'NONE',  ( 791.1614460488616487, 12.73985825558503926, -373.5763878283158874 ) ) ;
#24255=CARTESIAN_POINT ( 'NONE',  ( 764.1737431748507561, -298.3726999360616787, -371.6461892240376415 ) ) ;
#24259=CARTESIAN_POINT ( 'NONE',  ( 802.9823548866075953, -145.0999726633347677, -330.0799878456151077 ) ) ;
#24260=CARTESIAN_POINT ( 'NONE',  ( 805.1927285166397041, -136.8164208402382371, -341.8018195045277707 ) ) ;
#24261=CARTESIAN_POINT ( 'NONE',  ( 759.9864689768902508, -314.0891481129650629, -354.9819416627836404 ) ) ;
#24267=VERTEX_POINT ( 'NONE', #28420 ) ;
#24268=CARTESIAN_POINT ( 'NONE',  ( 809.0717654672305343, -388.9181544815158986, -360.1688906516309885 ) ) ;
#24275=CARTESIAN_POINT ( 'NONE',  ( 762.1405469898971887, -313.5436935675102745, -357.8594530101015607 ) ) ;
#24276=LINE ( 'NONE', #23808, #36256 ) ;
#24277=CARTESIAN_POINT ( 'NONE',  ( 769.9779781133707957, -235.0999726633344835, -316.7813123517150871 ) ) ;
#24280=CARTESIAN_POINT ( 'NONE',  ( 808.0189434323515343, -422.0891481129647218, -319.0252816721025511 ) ) ;
#24284=CARTESIAN_POINT ( 'NONE',  ( 787.4397851343537695, -45.72551174932949181, -374.2001403089903988 ) ) ;
#24285=CARTESIAN_POINT ( 'NONE',  ( 759.9864689768902508, -266.0891481129651197, -354.9819416627836404 ) ) ;
#24290=CARTESIAN_POINT ( 'NONE',  ( 745.7194118038753459, -13.64542720878976390, -348.7631598425976449 ) ) ;
#24291=CARTESIAN_POINT ( 'NONE',  ( 800.7704444035546203, -52.16923265350567362, -326.0291762391768771 ) ) ;
#24299=CARTESIAN_POINT ( 'NONE',  ( 755.3201227861273992, -75.72551174932937101, -345.3687786644892981 ) ) ;
#24300=CARTESIAN_POINT ( 'NONE',  ( 790.8726784830453198, -370.7146871989592114, -362.5472867521010585 ) ) ;
#24303=CARTESIAN_POINT ( 'NONE',  ( 754.0944755984390895, -399.6237781080500326, -364.1009440267246760 ) ) ;
#24310=CARTESIAN_POINT ( 'NONE',  ( 767.7687537140311633, -215.9073299311471317, -372.7932403749916830 ) ) ;
#24313=CARTESIAN_POINT ( 'NONE',  ( 803.6646147819162707, -209.9073299311471317, -348.8264449731211130 ) ) ;
#24316=CARTESIAN_POINT ( 'NONE',  ( 804.4286716492782716, -353.3618753856922012, -345.3141322388244703 ) ) ;
#24317=CARTESIAN_POINT ( 'NONE',  ( 774.6312213355099630, 0.6381246143067236254, -364.6798772138717482 ) ) ;
#24323=CARTESIAN_POINT ( 'NONE',  ( 767.8955696845333705, -0.4527844766023628176, -362.1676090361162323 ) ) ;
#24324=DIRECTION ( 'NONE',  ( -1.000000000000000000, -0.000000000000000000, -0.000000000000000000 ) ) ;
#24326=CARTESIAN_POINT ( 'NONE',  ( 812.3518521366052028, -265.0999726633344267, -326.5853460496235243 ) ) ;
#24329=CARTESIAN_POINT ( 'NONE',  ( 804.9363028652555840, -208.2709662947835341, -338.2165204200192079 ) ) ;
#24330=CARTESIAN_POINT ( 'NONE',  ( 793.2243759319678702, -386.5328690171409676, -318.4439275373583200 ) ) ;
#24332=CARTESIAN_POINT ( 'NONE',  ( 785.3687786644885591, 12.63812461430668677, -315.3201227861280813 ) ) ;
#24333=CARTESIAN_POINT ( 'NONE',  ( 763.8424801807145741, -114.0090635724258163, -320.5453621957614700 ) ) ;
#24336=CARTESIAN_POINT ( 'NONE',  ( 788.7631598425961101, 22.55804007376682918, -305.7194118038759143 ) ) ;
#24337=CARTESIAN_POINT ( 'NONE',  ( 745.0891759886404770, -316.2709662947832499, -342.4968714119734159 ) ) ;
#24340=CARTESIAN_POINT ( 'NONE',  ( 762.1405469898971887, -73.54369356751118403, -357.8594530101015607 ) ) ;
#24342=CARTESIAN_POINT ( 'NONE',  ( 746.0683387631852383, -163.4419599262325846, -331.3260364891676204 ) ) ;
#24344=CARTESIAN_POINT ( 'NONE',  ( 801.1904061080336987, -428.0891481129644944, -368.3070685750235498 ) ) ;
#24348=CARTESIAN_POINT ( 'NONE',  ( 755.5713283507202505, -437.3618753856919170, -334.6858677611754729 ) ) ;
#24349=DIRECTION ( 'NONE',  ( 0.000000000000000000, -1.000000000000000000, 0.000000000000000000 ) ) ;
#24354=CARTESIAN_POINT ( 'NONE',  ( 779.4709603349208464, -264.3510508353232353, -314.7162404726379918 ) ) ;
#24356=CARTESIAN_POINT ( 'NONE',  ( 807.5423716828161105, -273.0783235625958696, -362.2119215644372048 ) ) ;
#24361=CARTESIAN_POINT ( 'NONE',  ( 787.6308680596127942, -35.26014174441480264, -364.1105419155492768 ) ) ;
#24362=CARTESIAN_POINT ( 'NONE',  ( 762.3223304703356007, -151.5436935675109851, -322.3223304703362828 ) ) ;
#24363=CARTESIAN_POINT ( 'NONE',  ( 804.9363028652555840, -208.2709662947835341, -338.2165204200192079 ) ) ;
#24366=CARTESIAN_POINT ( 'NONE',  ( 749.2812353651451076, -102.4527844766020337, -323.2262854647983090 ) ) ;
#24367=CARTESIAN_POINT ( 'NONE',  ( 756.3353852180820240, -101.9073299311474869, -331.1735550268787733 ) ) ;
#24369=CARTESIAN_POINT ( 'NONE',  ( 804.4086373105744769, -385.6454272087888171, -333.3843516231986541 ) ) ;
#24377=CARTESIAN_POINT ( 'NONE',  ( 804.8461984189677878, -362.1908817542432644, -336.9566956441385628 ) ) ;
#24378=CARTESIAN_POINT ( 'NONE',  ( 802.1676090361156639, -350.6346026584192828, -327.8955696845344505 ) ) ;
#24379=CARTESIAN_POINT ( 'NONE',  ( 757.7880784355613741, -162.0090635724256742, -312.4576283171834916 ) ) ;
#24383=CARTESIAN_POINT ( 'NONE',  ( 800.7704444035546203, -292.1692326535048210, -326.0291762391768771 ) ) ;
#24384=CARTESIAN_POINT ( 'NONE',  ( 785.3687786644884454, -443.3618753856917465, -315.3201227861279676 ) ) ;
#24385=CARTESIAN_POINT ( 'NONE',  ( 795.8262568251477660, -142.3726999360620766, -308.3538107759623585 ) ) ;
#24390=CARTESIAN_POINT ( 'NONE',  ( 772.4837098697145166, -191.3618753856926276, -374.5518280994205611 ) ) ;
#24395=CARTESIAN_POINT ( 'NONE',  ( 805.0032342141412300, -325.5436935675105019, -314.9967657858571783 ) ) ;
#24396=CYLINDRICAL_SURFACE ( 'NONE', #32883, 30.00000000000008171 ) ;
#24402=CARTESIAN_POINT ( 'NONE',  ( 783.7566961878529810, -384.8965053807772847, -305.1792804349288417 ) ) ;
#24403=CARTESIAN_POINT ( 'NONE',  ( 792.3570229623688874, -141.1800572038746395, -373.1304606946836202 ) ) ;
#24404=CARTESIAN_POINT ( 'NONE',  ( 792.3570229623688874, -429.1800572038737869, -373.1304606946836202 ) ) ;
#24408=CARTESIAN_POINT ( 'NONE',  ( 758.0141637701419768, -159.0783235625962391, -367.2620300519063790 ) ) ;
#24416=CARTESIAN_POINT ( 'NONE',  ( 804.7487373415286811, 4.456306432488530866, -364.7487373415288516 ) ) ;
#24419=CARTESIAN_POINT ( 'NONE',  ( 811.3240766477731540, -412.3726999360612808, -355.6651683502462902 ) ) ;
#24422=CARTESIAN_POINT ( 'NONE',  ( 759.7806653035534055, -246.9982390220560546, -324.8639956371180801 ) ) ;
#24428=CARTESIAN_POINT ( 'NONE',  ( 780.5236548040995785, -260.7363362996981095, -314.9735926884559944 ) ) ;
#24429=CARTESIAN_POINT ( 'NONE',  ( 757.8323909638827445, -266.6346026584197375, -352.1044303154654358 ) ) ;
#24431=CARTESIAN_POINT ( 'NONE',  ( 762.1405469898971887, -97.54369356751112718, -357.8594530101015607 ) ) ;
#24436=CARTESIAN_POINT ( 'NONE',  ( 768.9521613784389729, -57.82724539060780700, -373.2346286133773106 ) ) ;
#24442=CARTESIAN_POINT ( 'NONE',  ( 796.1575198192839480, -6.009063572426154742, -359.4546378042384163 ) ) ;
#24444=CARTESIAN_POINT ( 'NONE',  ( 800.9747183278959710, -60.99823902205671544, -311.9810565676471583 ) ) ;
#24448=CARTESIAN_POINT ( 'NONE',  ( 810.7187646348534145, -186.4527844766017779, -356.7737145352016341 ) ) ;
#24452=CARTESIAN_POINT ( 'NONE',  ( 801.9858362298568863, -267.0783235625958696, -312.7379699480935642 ) ) ;
#24454=CARTESIAN_POINT ( 'NONE',  ( 792.2312462859673587, -275.9073299311469896, -307.2067596250082602 ) ) ;
#24458=CARTESIAN_POINT ( 'NONE',  ( 813.2346286133761168, -29.26014174441482751, -328.9521613784389160 ) ) ;
#24459=CARTESIAN_POINT ( 'NONE',  ( 759.7806653035534055, -390.9982390220557136, -324.8639956371180801 ) ) ;
#24461=CARTESIAN_POINT ( 'NONE',  ( 810.1134526219336749, -56.53286901714201917, -357.8822607201570349 ) ) ;
#24462=CARTESIAN_POINT ( 'NONE',  ( 787.6308680596127942, -203.2601417444143124, -364.1105419155492768 ) ) ;
#24468=CARTESIAN_POINT ( 'NONE',  ( 754.9735926884551418, -186.3510508353234343, -340.5236548041000333 ) ) ;
#24470=CARTESIAN_POINT ( 'NONE',  ( 756.1443688327750579, -45.62377810805114109, -314.3581564841659315 ) ) ;
#24476=CARTESIAN_POINT ( 'NONE',  ( 771.3260364891663130, -307.6454272087888171, -306.0683387631859773 ) ) ;
#24481=CARTESIAN_POINT ( 'NONE',  ( 757.0176451133909268, -133.0999726633348246, -349.9200121543848354 ) ) ;
#24482=CARTESIAN_POINT ( 'NONE',  ( 801.9419747391806368, -138.4527844766019200, -351.9812246680014027 ) ) ;
#24483=CARTESIAN_POINT ( 'NONE',  ( 804.9363028652555840, -352.2709662947830225, -338.2165204200192079 ) ) ;
#24487=CARTESIAN_POINT ( 'NONE',  ( 799.9999999999993179, -512.9681489794448908, -339.9999999999999432 ) ) ;
#24491=CARTESIAN_POINT ( 'NONE',  ( 764.1737431748507561, -370.3726999360613377, -371.6461892240376415 ) ) ;
#24496=CARTESIAN_POINT ( 'NONE',  ( 774.6858677611749044, -321.7255117493286320, -315.5713283507209894 ) ) ;
#24498=CARTESIAN_POINT ( 'NONE',  ( 769.0155153010367712, -226.3726999360617924, -362.7791456095907279 ) ) ;
#24502=CARTESIAN_POINT ( 'NONE',  ( 777.4774526936600978, -418.2709662947828519, -304.7301800767028226 ) ) ;
#24507=CARTESIAN_POINT ( 'NONE',  ( 745.0891759886404770, -52.27096629478401724, -342.4968714119734159 ) ) ;
#24508=CARTESIAN_POINT ( 'NONE',  ( 762.1405469898971887, -265.5436935675106156, -357.8594530101015607 ) ) ;
#24512=CARTESIAN_POINT ( 'NONE',  ( 750.9282345327678740, -40.91815448151695023, -319.8311093483690115 ) ) ;
#24513=CARTESIAN_POINT ( 'NONE',  ( 800.7704444035546203, -100.1692326535055315, -326.0291762391768771 ) ) ;
#24519=CARTESIAN_POINT ( 'NONE',  ( 802.1676090361156639, 9.365397341579420498, -327.8955696845344505 ) ) ;
#24520=CARTESIAN_POINT ( 'NONE',  ( 796.7845633553578182, -105.6237781080509421, -358.5707757039688204 ) ) ;
#24522=CARTESIAN_POINT ( 'NONE',  ( 764.8639956371174549, -56.08914811296580893, -319.7806653035542013 ) ) ;
#24523=CARTESIAN_POINT ( 'NONE',  ( 784.0799538623451781, -395.8055962898682765, -364.6971507214555572 ) ) ;
#24527=CARTESIAN_POINT ( 'NONE',  ( 795.6651683502461765, -394.7146871989591546, -371.3240766477733814 ) ) ;
#24532=CARTESIAN_POINT ( 'NONE',  ( 744.7301800767019131, -244.8164208402378961, -337.4774526936615757 ) ) ;
#24535=CARTESIAN_POINT ( 'NONE',  ( 767.8955696845334842, -240.4527844766015789, -362.1676090361161755 ) ) ;
#24537=CARTESIAN_POINT ( 'NONE',  ( 797.8594530101008786, -349.5436935675102745, -322.1405469898980982 ) ) ;
#24538=CARTESIAN_POINT ( 'NONE',  ( 800.0135310231082713, -14.08914811296595460, -325.0180583372163028 ) ) ;
#24543=CARTESIAN_POINT ( 'NONE',  ( 785.3687786644884454, -11.36187538569323863, -315.3201227861279676 ) ) ;
#24547=CARTESIAN_POINT ( 'NONE',  ( 746.4236121716829757, -279.8272453906071746, -328.8385539511384650 ) ) ;
#24550=CARTESIAN_POINT ( 'NONE',  ( 797.6776695296629214, -235.5436935675107293, -357.6776695296636603 ) ) ;
#24551=CARTESIAN_POINT ( 'NONE',  ( 755.0488828828309806, -401.8055962898681059, -344.1219089521771934 ) ) ;
#24554=CARTESIAN_POINT ( 'NONE',  ( 772.4468031744293057, -129.8272453906075725, -363.8651313633793620 ) ) ;
#24556=CARTESIAN_POINT ( 'NONE',  ( 754.0944755984390895, 8.376221891948691933, -364.1009440267246760 ) ) ;
#24557=CARTESIAN_POINT ( 'NONE',  ( 759.0252816721024374, -312.9982390220559409, -368.0189434323527280 ) ) ;
#24559=CARTESIAN_POINT ( 'NONE',  ( 799.9999999999993179, 205.0000000000000568, -339.9999999999999432 ) ) ;
#24560=CARTESIAN_POINT ( 'NONE',  ( 781.8018195045266339, -94.27096629478386092, -365.1927285166406705 ) ) ;
#24561=CARTESIAN_POINT ( 'NONE',  ( 812.6845335610512393, -271.9874144716868045, -353.5525998758768651 ) ) ;
#24563=CARTESIAN_POINT ( 'NONE',  ( 776.2433038121456548, -204.8965053807779100, -374.8207195650711014 ) ) ;
#24565=CARTESIAN_POINT ( 'NONE',  ( 763.0537975583475827, -432.4527844766008684, -371.0346526505627480 ) ) ;
#24569=CARTESIAN_POINT ( 'NONE',  ( 775.9200461376533440, 24.19440371013046231, -315.3028492785443291 ) ) ;
#24571=MECHANICAL_DESIGN_GEOMETRIC_PRESENTATION_REPRESENTATION('',(#40809),#12772);
#24576=CARTESIAN_POINT ( 'NONE',  ( 790.8726784830453198, -274.7146871989594388, -362.5472867521010585 ) ) ;
#24579=CARTESIAN_POINT ( 'NONE',  ( 810.1134526219336749, -296.5328690171411949, -357.8822607201570349 ) ) ;
#24582=EDGE_LOOP ( 'NONE', ( #7069, #31118, #37248, #39719 ) ) ;
#24584=CARTESIAN_POINT ( 'NONE',  ( 776.9566956441375396, -36.89650538077844288, -364.8461984189686405 ) ) ;
#24585=CARTESIAN_POINT ( 'NONE',  ( 774.6312213355099630, -167.3618753856927412, -364.6798772138717482 ) ) ;
#24586=CARTESIAN_POINT ( 'NONE',  ( 804.6798772138708955, -207.7255117493289447, -334.6312213355107019 ) ) ;
#24588=CARTESIAN_POINT ( 'NONE',  ( 777.4774526936600978, -154.2709662947836478, -304.7301800767027657 ) ) ;
#24589=CARTESIAN_POINT ( 'NONE',  ( 778.1981804954715471, -106.2709662947838467, -314.8072714833591021 ) ) ;
#24591=CARTESIAN_POINT ( 'NONE',  ( 757.0176451133909268, -373.0999726633340856, -349.9200121543848354 ) ) ;
#24596=DIRECTION ( 'NONE',  ( -1.000000000000000000, -0.000000000000000000, -0.000000000000000000 ) ) ;
#24600=CARTESIAN_POINT ( 'NONE',  ( 758.4439275373578084, -348.5545181178796383, -353.2243759319684386 ) ) ;
#24601=CARTESIAN_POINT ( 'NONE',  ( 767.8955696845333705, -360.4527844766010958, -362.1676090361162323 ) ) ;
#24602=CARTESIAN_POINT ( 'NONE',  ( 778.7629533639073998, -152.7363362996983938, -375.0009284576466371 ) ) ;
#24607=CARTESIAN_POINT ( 'NONE',  ( 789.9200121543843807, -289.9874144716866908, -317.0176451133914384 ) ) ;
#24608=CARTESIAN_POINT ( 'NONE',  ( 774.6858677611749044, -441.7255117493282910, -315.5713283507209894 ) ) ;
#24609=CARTESIAN_POINT ( 'NONE',  ( 804.1009440267234822, -167.4636090269711133, -314.0944755984392600 ) ) ;
#24610=CYLINDRICAL_SURFACE ( 'NONE', #35963, 30.00000000000002842 ) ;
#24614=CARTESIAN_POINT ( 'NONE',  ( 744.7301800767020268, -196.8164208402380950, -337.4774526936615189 ) ) ;
#24618=CARTESIAN_POINT ( 'NONE',  ( 748.3538107759620743, -112.7146871989600356, -355.8262568251490165 ) ) ;
#24619=CARTESIAN_POINT ( 'NONE',  ( 814.2001403089898304, -353.3618753856922012, -347.4397851343538264 ) ) ;
#24628=CARTESIAN_POINT ( 'NONE',  ( 803.8556311672234642, -369.6237781080500895, -365.6418435158340117 ) ) ;
#24629=CARTESIAN_POINT ( 'NONE',  ( 787.4397851343537695, -141.7255117493291721, -374.2001403089903988 ) ) ;
#24630=CARTESIAN_POINT ( 'NONE',  ( 796.9462024416508257, -420.4527844766009252, -308.9653473494370246 ) ) ;
#24634=ADVANCED_FACE ( 'NONE', ( #35812, #4619 ), #36488, .F. ) ;
#24635=CARTESIAN_POINT ( 'NONE',  ( 811.6461892240364477, -196.7146871989598083, -324.1737431748509835 ) ) ;
#24644=CARTESIAN_POINT ( 'NONE',  ( 745.4481719005789273, -3.725511749329622813, -347.5162901302853129 ) ) ;
#24648=CARTESIAN_POINT ( 'NONE',  ( 778.7629533639073998, -416.7363362996975980, -375.0009284576466371 ) ) ;
#24653=CARTESIAN_POINT ( 'NONE',  ( 788.7366044899766848, -275.9073299311469896, -316.5762568750059813 ) ) ;
#24658=CARTESIAN_POINT ( 'NONE',  ( 755.8894580844503253, -255.8272453906072315, -332.3691319403863531 ) ) ;
#24659=CARTESIAN_POINT ( 'NONE',  ( 759.7806653035534055, -246.9982390220560546, -324.8639956371180801 ) ) ;
#24661=CARTESIAN_POINT ( 'NONE',  ( 804.9363028652555840, -112.2709662947838325, -338.2165204200192079 ) ) ;
#24667=CARTESIAN_POINT ( 'NONE',  ( 760.0363995740630116, -58.91815448151690759, -368.7758568127991907 ) ) ;
#24668=CARTESIAN_POINT ( 'NONE',  ( 779.9999999999992042, -452.9681489794448339, -350.0000000000000000 ) ) ;
#24673=CARTESIAN_POINT ( 'NONE',  ( 755.8894580844503253, -15.82724539060794200, -332.3691319403863531 ) ) ;
#24674=CARTESIAN_POINT ( 'NONE',  ( 804.7487373415286811, -91.54369356751116982, -364.7487373415288516 ) ) ;
#24676=DIRECTION ( 'NONE',  ( -1.000000000000000000, -0.000000000000000000, -0.000000000000000000 ) ) ;
#24680=CARTESIAN_POINT ( 'NONE',  ( 751.6929314249748586, -222.9982390220561399, -318.8095938919659034 ) ) ;
#24685=CARTESIAN_POINT ( 'NONE',  ( 749.8865473780648472, -260.5328690171413086, -322.1177392798429082 ) ) ;
#24687=CARTESIAN_POINT ( 'NONE',  ( 814.9108240113580450, -304.2709662947832499, -337.5031285880265273 ) ) ;
#24692=CARTESIAN_POINT ( 'NONE',  ( 804.4286716492782716, -377.3618753856920875, -345.3141322388244703 ) ) ;
#24696=CARTESIAN_POINT ( 'NONE',  ( 813.2346286133761168, -101.2601417444146250, -328.9521613784389160 ) ) ;
#24701=CARTESIAN_POINT ( 'NONE',  ( 766.7756240680305382, -206.5328690171415360, -361.5560724626415663 ) ) ;
#24703=CARTESIAN_POINT ( 'NONE',  ( 751.2241431872005251, -40.16923265350570915, -359.9636004259367610 ) ) ;
#24709=CARTESIAN_POINT ( 'NONE',  ( 811.3240766477731540, -316.3726999360615082, -355.6651683502462902 ) ) ;
#24716=CARTESIAN_POINT ( 'NONE',  ( 759.0159684113467620, -160.9181544815165807, -325.8855110935213020 ) ) ;
#24717=CARTESIAN_POINT ( 'NONE',  ( 805.1927285166397041, -160.8164208402382371, -341.8018195045277707 ) ) ;
#24718=CARTESIAN_POINT ( 'NONE',  ( 774.6858677611749044, -345.7255117493285184, -315.5713283507209894 ) ) ;
#24726=ORIENTED_EDGE ( 'NONE', *, *, #3181, .T. ) ;
#24727=CARTESIAN_POINT ( 'NONE',  ( 805.6418435158337843, -389.4636090269704027, -363.8556311672236916 ) ) ;
#24729=CARTESIAN_POINT ( 'NONE',  ( 811.0346526505617248, -14.63460265842049779, -323.0537975583478101 ) ) ;
#24734=CARTESIAN_POINT ( 'NONE',  ( 797.6776695296629214, -379.5436935675102745, -357.6776695296636603 ) ) ;
#24738=CARTESIAN_POINT ( 'NONE',  ( 766.9102291470427417, -210.5545181178800647, -318.6633372737382501 ) ) ;
#24743=CARTESIAN_POINT ( 'NONE',  ( 772.4837098697145166, -407.3618753856920307, -374.5518280994205611 ) ) ;
#24749=CARTESIAN_POINT ( 'NONE',  ( 745.4481719005789273, -51.72551174932946338, -347.5162901302853129 ) ) ;
#24750=CARTESIAN_POINT ( 'NONE',  ( 778.2165204200184689, -286.8164208402378677, -364.9363028652563230 ) ) ;
#24755=CARTESIAN_POINT ( 'NONE',  ( 788.6739635108323228, -31.64542720878970883, -373.9316612368139090 ) ) ;
#24756=CARTESIAN_POINT ( 'NONE',  ( 800.7704444035546203, -76.16923265350557415, -326.0291762391768771 ) ) ;
#24760=CARTESIAN_POINT ( 'NONE',  ( 803.4237431249931660, 8.819942796124882634, -331.2633955100225194 ) ) ;
#24762=CARTESIAN_POINT ( 'NONE',  ( 755.5713283507202505, -101.3618753856929544, -334.6858677611754729 ) ) ;
#24763=CARTESIAN_POINT ( 'NONE',  ( 787.6308680596127942, -395.2601417444136587, -364.1105419155492768 ) ) ;
#24767=CARTESIAN_POINT ( 'NONE',  ( 783.7566961878529810, -384.8965053807772847, -305.1792804349288417 ) ) ;
#24775=CARTESIAN_POINT ( 'NONE',  ( 751.9810565676468741, -242.0891481129652618, -360.9747183278973921 ) ) ;
#24778=CARTESIAN_POINT ( 'NONE',  ( 778.1981804954715471, -250.2709662947833351, -314.8072714833591021 ) ) ;
#24780=CARTESIAN_POINT ( 'NONE',  ( 774.6858677611749044, -369.7255117493284615, -315.5713283507209894 ) ) ;
#24781=CARTESIAN_POINT ( 'NONE',  ( 757.8323909638827445, -26.63460265842045871, -352.1044303154654358 ) ) ;
#24788=CARTESIAN_POINT ( 'NONE',  ( 762.1405469898971887, -1.543693567511449150, -357.8594530101015607 ) ) ;
#24791=VERTEX_POINT ( 'NONE', #23060 ) ;
#24792=CARTESIAN_POINT ( 'NONE',  ( 791.0478386215596629, -261.8272453906071746, -306.7653713866226326 ) ) ;
#24795=CARTESIAN_POINT ( 'NONE',  ( 781.7834795799800531, -250.8164208402379245, -315.0636971347436202 ) ) ;
#24796=CARTESIAN_POINT ( 'NONE',  ( 789.9200121543843807, -409.9874144716863498, -317.0176451133914384 ) ) ;
#24798=CARTESIAN_POINT ( 'NONE',  ( 804.1105419155481968, -123.8272453906076009, -347.6308680596136469 ) ) ;
#24800=CARTESIAN_POINT ( 'NONE',  ( 799.9999999999993179, -512.9681489794448908, -329.9999999999999432 ) ) ;
#24801=CARTESIAN_POINT ( 'NONE',  ( 778.7502325331095108, -0.3510508353240099355, -304.6391490659818828 ) ) ;
#24802=CARTESIAN_POINT ( 'NONE',  ( 814.5518280994195948, -327.7255117493285752, -332.4837098697145166 ) ) ;
#24804=CARTESIAN_POINT ( 'NONE',  ( 791.9812246680005501, -68.63460265842033436, -361.9419747391813189 ) ) ;
#24806=CARTESIAN_POINT ( 'NONE',  ( 812.6845335610512393, -199.9874144716870603, -353.5525998758768651 ) ) ;
#24808=CARTESIAN_POINT ( 'NONE',  ( 810.7187646348534145, -450.4527844766009821, -356.7737145352016341 ) ) ;
#24813=CARTESIAN_POINT ( 'NONE',  ( 759.2295555964440155, 7.830767346494148740, -353.9708237608231229 ) ) ;
#24820=CARTESIAN_POINT ( 'NONE',  ( 764.0069404352550464, -303.0783235625957559, -359.2566176426627180 ) ) ;
#24822=CARTESIAN_POINT ( 'NONE',  ( 812.6845335610512393, -295.9874144716866908, -353.5525998758768651 ) ) ;
#24823=DIRECTION ( 'NONE',  ( 0.000000000000000000, 0.000000000000000000, -1.000000000000000000 ) ) ;
#24827=CARTESIAN_POINT ( 'NONE',  ( 760.5453621957607311, -45.07832356259660145, -323.8424801807151425 ) ) ;
#24828=CARTESIAN_POINT ( 'NONE',  ( 778.1981804954714335, -154.2709662947836478, -314.8072714833589885 ) ) ;
#24829=CARTESIAN_POINT ( 'NONE',  ( 754.8072714833581358, -196.8164208402380950, -338.1981804954720587 ) ) ;
#24831=CARTESIAN_POINT ( 'NONE',  ( 749.2812353651451076, -150.4527844766018916, -323.2262854647983090 ) ) ;
#24833=CARTESIAN_POINT ( 'NONE',  ( 805.1927285166399315, -136.8164208402382656, -341.8018195045277707 ) ) ;
#24836=CARTESIAN_POINT ( 'NONE',  ( 761.4292242960306112, -401.4636090269704027, -323.2154366446414429 ) ) ;
#24844=CARTESIAN_POINT ( 'NONE',  ( 769.0155153010367712, -394.3726999360613377, -362.7791456095907279 ) ) ;
#24845=CARTESIAN_POINT ( 'NONE',  ( 768.0187753319979720, -368.6346026584193964, -318.0580252608186242 ) ) ;
#24846=CARTESIAN_POINT ( 'NONE',  ( 747.6481478633932056, -157.0999726633347962, -353.4146539503763620 ) ) ;
#24850=LINE ( 'NONE', #45664, #22528 ) ;
#24851=CARTESIAN_POINT ( 'NONE',  ( 796.7845633553578182, -297.6237781080502600, -358.5707757039688204 ) ) ;
#24853=CARTESIAN_POINT ( 'NONE',  ( 768.9521613784389729, -201.8272453906073451, -373.2346286133773106 ) ) ;
#24854=DIRECTION ( 'NONE',  ( -1.000000000000000000, -0.000000000000000000, -0.000000000000000000 ) ) ;
#24859=CARTESIAN_POINT ( 'NONE',  ( 763.0537975583476964, -192.4527844766017211, -371.0346526505628617 ) ) ;
#24861=CARTESIAN_POINT ( 'NONE',  ( 800.0135310231082713, 9.910851887033969021, -325.0180583372163028 ) ) ;
#24863=CARTESIAN_POINT ( 'NONE',  ( 744.8212110874229666, -114.8965053807782226, -336.2046728542121627 ) ) ;
#24865=CARTESIAN_POINT ( 'NONE',  ( 815.2698199232961542, -352.8164208402374129, -342.5225473063383106 ) ) ;
#24870=CARTESIAN_POINT ( 'NONE',  ( 746.0683387631852383, -403.4419599262317888, -331.3260364891676204 ) ) ;
#24872=CARTESIAN_POINT ( 'NONE',  ( 745.4481719005789273, -411.7255117493282910, -347.5162901302853129 ) ) ;
#24877=CARTESIAN_POINT ( 'NONE',  ( 786.2056067578752163, -179.8055962898688733, -374.4686193811670023 ) ) ;
#24884=CARTESIAN_POINT ( 'NONE',  ( 796.9462024416508257, -36.45278447660223975, -308.9653473494370246 ) ) ;
#24887=CARTESIAN_POINT ( 'NONE',  ( 773.7305795820266212, -441.2817908451521021, -374.8230680027170365 ) ) ;
#24891=CARTESIAN_POINT ( 'NONE',  ( 803.6646147819161570, -281.9073299311468759, -348.8264449731210561 ) ) ;
#24895=CARTESIAN_POINT ( 'NONE',  ( 759.0159684113467620, -280.9181544815162965, -325.8855110935213020 ) ) ;
#24896=CARTESIAN_POINT ( 'NONE',  ( 778.1981804954714335, -250.2709662947832783, -314.8072714833589885 ) ) ;
#24897=CARTESIAN_POINT ( 'NONE',  ( 781.7834795799800531, -442.8164208402372992, -315.0636971347436202 ) ) ;
#24898=CARTESIAN_POINT ( 'NONE',  ( 795.1360043628807261, -116.0891481129656029, -360.2193346964456282 ) ) ;
#24903=CARTESIAN_POINT ( 'NONE',  ( 764.1737431748507561, -58.37269993606236085, -371.6461892240376415 ) ) ;
#24910=CARTESIAN_POINT ( 'NONE',  ( 775.8780910478218402, -9.281790845153418346, -364.9511171171680530 ) ) ;
#24911=CARTESIAN_POINT ( 'NONE',  ( 745.7998596910086917, -101.3618753856929544, -332.5602148656461168 ) ) ;
#24916=CARTESIAN_POINT ( 'NONE',  ( 772.5602148656447525, -225.7255117493289163, -305.7998596910095443 ) ) ;
#24920=CARTESIAN_POINT ( 'NONE',  ( 759.8311093483677041, -310.1692326535048778, -310.9282345327691814 ) ) ;
#24922=CARTESIAN_POINT ( 'NONE',  ( 748.9653473494363425, -314.6346026584194533, -356.9462024416521331 ) ) ;
#24926=CARTESIAN_POINT ( 'NONE',  ( 801.9419747391806368, -402.4527844766010389, -351.9812246680014027 ) ) ;
#24928=CARTESIAN_POINT ( 'NONE',  ( 762.3223304703356007, -199.5436935675108430, -322.3223304703362828 ) ) ;
#24929=CARTESIAN_POINT ( 'NONE',  ( 752.4576283171824116, -93.07832356259645223, -317.7880784355627952 ) ) ;
#24933=CARTESIAN_POINT ( 'NONE',  ( 754.9735926884551418, -210.3510508353233490, -340.5236548041000333 ) ) ;
#24935=CARTESIAN_POINT ( 'NONE',  ( 761.9338519418445230, -38.53286901714206891, -370.4231160770881957 ) ) ;
#24941=CARTESIAN_POINT ( 'NONE',  ( 807.2620300519052989, -360.0090635724250774, -318.0141637701419768 ) ) ;
#24946=CARTESIAN_POINT ( 'NONE',  ( 755.5913626894240451, -133.6454272087893571, -346.6156483768012890 ) ) ;
#24947=CARTESIAN_POINT ( 'NONE',  ( 792.1044303154645831, -132.4527844766018916, -317.8323909638837677 ) ) ;
#24948=CARTESIAN_POINT ( 'NONE',  ( 756.5762568750052424, -339.1800572038740142, -348.7366044899774238 ) ) ;
#24950=CARTESIAN_POINT ( 'NONE',  ( 804.9363028652555840, -448.2709662947827951, -338.2165204200192079 ) ) ;
#24959=CARTESIAN_POINT ( 'NONE',  ( 746.4236121716829757, -375.8272453906069472, -328.8385539511384650 ) ) ;
#24960=CARTESIAN_POINT ( 'NONE',  ( 801.1904061080338124, 3.910851887033986785, -368.3070685750236066 ) ) ;
#24964=CARTESIAN_POINT ( 'NONE',  ( 788.8264449731200330, -357.1800572038739006, -363.6646147819171233 ) ) ;
#24967=CARTESIAN_POINT ( 'NONE',  ( 763.8424801807145741, -210.0090635724255321, -320.5453621957614700 ) ) ;
#24971=CARTESIAN_POINT ( 'NONE',  ( 787.4397851343537695, -429.7255117493282910, -374.2001403089903988 ) ) ;
#24972=EDGE_CURVE ( 'NONE', #35503, #41096, #813, .T. ) ;
#24978=CARTESIAN_POINT ( 'NONE',  ( 815.2698199232961542, -64.81642084023852135, -342.5225473063383106 ) ) ;
#24979=CARTESIAN_POINT ( 'NONE',  ( 803.4237431249931660, -279.1800572038741848, -331.2633955100225194 ) ) ;
#24982=EDGE_CURVE ( 'NONE', #19525, #8509, #29268, .T. ) ;
#24984=CARTESIAN_POINT ( 'NONE',  ( 793.5525998758768083, -55.09997266333508747, -372.6845335610516941 ) ) ;
#24985=CARTESIAN_POINT ( 'NONE',  ( 803.2186876482843445, -79.98741447168740137, -350.0220218866286928 ) ) ;
#24989=CARTESIAN_POINT ( 'NONE',  ( 797.8594530101008786, 10.45630643248850866, -322.1405469898980982 ) ) ;
#24991=CARTESIAN_POINT ( 'NONE',  ( 765.0180583372156207, -96.99823902205660886, -360.0135310231089534 ) ) ;
#24992=CARTESIAN_POINT ( 'NONE',  ( 805.0264073115434940, -390.3510508353227237, -339.4763451958999099 ) ) ;
#24996=CARTESIAN_POINT ( 'NONE',  ( 814.8230680027162407, -413.8055962898681059, -333.7305795820267917 ) ) ;
#25002=CARTESIAN_POINT ( 'NONE',  ( 777.5031285880264704, -262.8164208402379245, -374.9108240113588408 ) ) ;
#25007=CARTESIAN_POINT ( 'NONE',  ( 786.5483106153019435, -31.64542720878970883, -364.1601925771022366 ) ) ;
#25009=CARTESIAN_POINT ( 'NONE',  ( 797.6776695296629214, -259.5436935675106156, -357.6776695296636603 ) ) ;
#25011=VECTOR ( 'NONE', #20548, 1000.000000000000000 ) ;
#25012=CARTESIAN_POINT ( 'NONE',  ( 764.8639956371174549, -368.0891481129647786, -319.7806653035542013 ) ) ;
#25013=CARTESIAN_POINT ( 'NONE',  ( 759.9864689768902508, -2.089148112965993231, -354.9819416627836404 ) ) ;
#25019=CARTESIAN_POINT ( 'NONE',  ( 774.6858677611749044, -33.72551174932952733, -315.5713283507209894 ) ) ;
#25023=CARTESIAN_POINT ( 'NONE',  ( 776.2046728542105711, -260.1908817542435486, -304.8212110874238761 ) ) ;
#25026=CARTESIAN_POINT ( 'NONE',  ( 759.9864689768902508, -266.0891481129651197, -354.9819416627836404 ) ) ;
#25027=CARTESIAN_POINT ( 'NONE',  ( 802.5472867521000353, -124.3726999360621619, -350.8726784830461156 ) ) ;
#25030=CARTESIAN_POINT ( 'NONE',  ( 808.7758568127978833, 19.83076734649410966, -320.0363995740631822 ) ) ;
#25031=CARTESIAN_POINT ( 'NONE',  ( 782.4968714119720516, -322.8164208402377540, -305.0891759886411023 ) ) ;
#25035=CARTESIAN_POINT ( 'NONE',  ( 744.9990715423526808, -186.3510508353234343, -341.2370466360926002 ) ) ;
#25037=CARTESIAN_POINT ( 'NONE',  ( 772.4837098697144029, -431.3618753856918033, -374.5518280994205611 ) ) ;
#25042=CARTESIAN_POINT ( 'NONE',  ( 804.4286716492782716, -449.3618753856918602, -345.3141322388244703 ) ) ;
#25049=CARTESIAN_POINT ( 'NONE',  ( 757.2208543904082489, -280.7146871989594956, -350.9844846989624330 ) ) ;
#25051=CARTESIAN_POINT ( 'NONE',  ( 752.4576283171824116, -309.0783235625957559, -317.7880784355627952 ) ) ;
#25056=CARTESIAN_POINT ( 'NONE',  ( 755.0488828828309806, -89.80559628986918597, -344.1219089521771934 ) ) ;
#25057=CARTESIAN_POINT ( 'NONE',  ( 757.8323909638827445, -146.6346026584200217, -352.1044303154654358 ) ) ;
#25058=CARTESIAN_POINT ( 'NONE',  ( 771.1735550268778070, -225.1800572038743269, -316.3353852180827630 ) ) ;
#25060=CARTESIAN_POINT ( 'NONE',  ( 782.4968714119720516, -154.8164208402382371, -305.0891759886411023 ) ) ;
#25062=CARTESIAN_POINT ( 'NONE',  ( 759.9864689768902508, -146.0891481129655176, -354.9819416627836404 ) ) ;
#25064=CARTESIAN_POINT ( 'NONE',  ( 776.9254006560222479, -404.1908817542431507, -314.8983024940802125 ) ) ;
#25070=CARTESIAN_POINT ( 'NONE',  ( 766.9102291470427417, -402.5545181178795247, -318.6633372737382501 ) ) ;
#25072=CARTESIAN_POINT ( 'NONE',  ( 744.6391490659812007, -182.7363362996983369, -338.7502325331110455 ) ) ;
#25076=CARTESIAN_POINT ( 'NONE',  ( 805.1016975059191054, -294.8965053807775689, -343.0745993439771837 ) ) ;
#25078=CARTESIAN_POINT ( 'NONE',  ( 811.3240766477731540, -172.3726999360619914, -355.6651683502462902 ) ) ;
#25083=CARTESIAN_POINT ( 'NONE',  ( 747.2067596250078623, -219.1800572038744122, -352.2312462859687230 ) ) ;
#25085=CARTESIAN_POINT ( 'NONE',  ( 797.6776695296629214, 4.456306432488530866, -357.6776695296636603 ) ) ;
#25087=CARTESIAN_POINT ( 'NONE',  ( 746.7653713866222915, -89.26014174441463922, -351.0478386215610271 ) ) ;
#25089=CARTESIAN_POINT ( 'NONE',  ( 810.7187646348534145, -330.4527844766013231, -356.7737145352016341 ) ) ;
#25094=CARTESIAN_POINT ( 'NONE',  ( 814.8230680027162407, -413.8055962898681059, -333.7305795820267917 ) ) ;
#25095=CARTESIAN_POINT ( 'NONE',  ( 772.5602148656447525, -417.7255117493283478, -305.7998596910095443 ) ) ;
#25099=CARTESIAN_POINT ( 'NONE',  ( 749.8865473780648472, -188.5328690171416497, -322.1177392798429082 ) ) ;
#25105=CARTESIAN_POINT ( 'NONE',  ( 777.4774526936600978, -34.27096629478407408, -304.7301800767027657 ) ) ;
#25109=CARTESIAN_POINT ( 'NONE',  ( 795.8262568251477660, -430.3726999360611671, -308.3538107759623585 ) ) ;
#25113=CARTESIAN_POINT ( 'NONE',  ( 804.9363028652555840, -280.2709662947833067, -338.2165204200192079 ) ) ;
#25117=CARTESIAN_POINT ( 'NONE',  ( 760.7433823573367135, -276.0090635724253048, -355.9930595647440441 ) ) ;
#25118=CARTESIAN_POINT ( 'NONE',  ( 803.4237431249931660, -279.1800572038741848, -331.2633955100225194 ) ) ;
#25119=CARTESIAN_POINT ( 'NONE',  ( 800.0135310231082713, -446.0891481129646081, -325.0180583372163028 ) ) ;
#25120=CARTESIAN_POINT ( 'NONE',  ( 788.7366044899766848, -131.9073299311473875, -316.5762568750059813 ) ) ;
#25126=CARTESIAN_POINT ( 'NONE',  ( 793.5525998758768083, -79.09997266333503774, -372.6845335610516941 ) ) ;
#25132=CARTESIAN_POINT ( 'NONE',  ( 793.9708237608222134, -46.91815448151694312, -319.2295555964448681 ) ) ;
#25133=CARTESIAN_POINT ( 'NONE',  ( 804.7487373415286811, -115.5436935675110988, -364.7487373415288516 ) ) ;
#25137=CARTESIAN_POINT ( 'NONE',  ( 782.4968714119720516, -226.8164208402380098, -305.0891759886411023 ) ) ;
#25141=CARTESIAN_POINT ( 'NONE',  ( 751.2241431872005251, -304.1692326535048210, -359.9636004259367610 ) ) ;
#25143=CARTESIAN_POINT ( 'NONE',  ( 746.8695393053150156, -317.9073299311468190, -327.6429770376306010 ) ) ;
#25147=CARTESIAN_POINT ( 'NONE',  ( 805.1927285166397041, -400.8164208402373561, -341.8018195045277707 ) ) ;
#25149=CARTESIAN_POINT ( 'NONE',  ( 767.8955696845333705, -192.4527844766016926, -362.1676090361162323 ) ) ;
#25150=CARTESIAN_POINT ( 'NONE',  ( 756.1443688327750579, -69.62377810805107003, -314.3581564841659315 ) ) ;
#25155=CARTESIAN_POINT ( 'NONE',  ( 793.2243759319678702, -218.5328690171414792, -318.4439275373583200 ) ) ;
#25158=CARTESIAN_POINT ( 'NONE',  ( 810.1134526219336749, -32.53286901714208312, -357.8822607201570349 ) ) ;
#25160=EDGE_CURVE ( 'NONE', #15183, #35055, #25557, .T. ) ;
#25165=CARTESIAN_POINT ( 'NONE',  ( 799.9636004259356241, -358.9181544815160123, -311.2241431872006956 ) ) ;
#25168=CARTESIAN_POINT ( 'NONE',  ( 804.6971507214547046, -195.2817908451528410, -344.0799538623459739 ) ) ;
#25169=CARTESIAN_POINT ( 'NONE',  ( 804.6798772138708955, -159.7255117493291436, -334.6312213355107019 ) ) ;
#25170=CARTESIAN_POINT ( 'NONE',  ( 756.3353852180820240, -365.9073299311466485, -331.1735550268787733 ) ) ;
#25179=CARTESIAN_POINT ( 'NONE',  ( 745.5313806188320314, -423.2817908451521589, -333.7943932421247268 ) ) ;
#25180=CARTESIAN_POINT ( 'NONE',  ( 747.2067596250078623, -3.180057203875080063, -352.2312462859687230 ) ) ;
#25183=CARTESIAN_POINT ( 'NONE',  ( 785.3687786644884454, -371.3618753856919739, -315.3201227861279676 ) ) ;
#25186=CARTESIAN_POINT ( 'NONE',  ( 757.4527132478984868, -208.3726999360619061, -329.1273215169538844 ) ) ;
#25190=CARTESIAN_POINT ( 'NONE',  ( 745.7998596910086917, -437.3618753856919170, -332.5602148656461168 ) ) ;
#25195=CARTESIAN_POINT ( 'NONE',  ( 755.2512626584698410, -79.54369356751119824, -315.2512626584710915 ) ) ;
#25196=CARTESIAN_POINT ( 'NONE',  ( 781.7834795799800531, -298.8164208402377540, -315.0636971347436202 ) ) ;
#25198=CARTESIAN_POINT ( 'NONE',  ( 791.7608162188021197, 205.0000000000000568, -319.9999999999999432 ) ) ;
#25203=CARTESIAN_POINT ( 'NONE',  ( 745.1792804349281596, -62.19088175424416676, -343.7566961878542884 ) ) ;
#25204=CARTESIAN_POINT ( 'NONE',  ( 765.8855110935204493, -94.16923265350555994, -319.0159684113471599 ) ) ;
#25207=CARTESIAN_POINT ( 'NONE',  ( 757.8323909638827445, -2.634602658420536869, -352.1044303154654358 ) ) ;
#25209=CARTESIAN_POINT ( 'NONE',  ( 755.0636971347428243, -100.2709662947838609, -341.7834795799807353 ) ) ;
#25211=CARTESIAN_POINT ( 'NONE',  ( 804.9511171171677688, -413.8055962898681059, -335.8780910478229202 ) ) ;
#25214=CARTESIAN_POINT ( 'NONE',  ( 771.2368401574024119, -397.4419599262317320, -374.2805881961240857 ) ) ;
#25219=SHAPE_REPRESENTATION_RELATIONSHIP ( 'NONE' , 'NONE' ,  #28408, #10570 ) ;
#25220=CARTESIAN_POINT ( 'NONE',  ( 814.9108240113580450, -256.2709662947834204, -337.5031285880265273 ) ) ;
#25225=CARTESIAN_POINT ( 'NONE',  ( 780.5236548040995785, -92.73633629969860692, -314.9735926884559944 ) ) ;
#25227=CARTESIAN_POINT ( 'NONE',  ( 804.6798772138710092, -255.7255117493287742, -334.6312213355106451 ) ) ;
#25230=CARTESIAN_POINT ( 'NONE',  ( 757.8323909638827445, -410.6346026584191122, -352.1044303154654358 ) ) ;
#25231=CARTESIAN_POINT ( 'NONE',  ( 758.0580252608178853, -54.45278447660219001, -328.0187753319985404 ) ) ;
#25237=CARTESIAN_POINT ( 'NONE',  ( 758.0580252608178853, -30.45278447660226817, -328.0187753319985404 ) ) ;
#25241=CARTESIAN_POINT ( 'NONE',  ( 799.9636004259356241, -286.9181544815161828, -311.2241431872006956 ) ) ;
#25245=CARTESIAN_POINT ( 'NONE',  ( 755.5713283507202505, -245.3618753856925139, -334.6858677611754729 ) ) ;
#25246=CARTESIAN_POINT ( 'NONE',  ( 757.4527132478984868, -112.3726999360621761, -329.1273215169538844 ) ) ;
#25249=CARTESIAN_POINT ( 'NONE',  ( 815.1787889125755555, -6.896505380778533478, -343.7953271457877804 ) ) ;
#25250=CARTESIAN_POINT ( 'NONE',  ( 777.5031285880264704, -310.8164208402377540, -374.9108240113588408 ) ) ;
#25255=CARTESIAN_POINT ( 'NONE',  ( 747.3154664389472828, -211.9874144716869750, -326.4474001241230781 ) ) ;
#25257=CARTESIAN_POINT ( 'NONE',  ( 757.7880784355613741, 5.990936427573807954, -312.4576283171834916 ) ) ;
#25261=AXIS2_PLACEMENT_3D ( 'NONE', #16568, #17020, #27631 ) ;
#25264=CARTESIAN_POINT ( 'NONE',  ( 801.3366627262608972, 15.46713098285775878, -353.0897708529566899 ) ) ;
#25272=CARTESIAN_POINT ( 'NONE',  ( 769.1273215169530886, -286.7146871989594388, -317.4527132478988847 ) ) ;
#25274=CARTESIAN_POINT ( 'NONE',  ( 759.8311093483677041, -310.1692326535048778, -310.9282345327691814 ) ) ;
#25279=CARTESIAN_POINT ( 'NONE',  ( 756.7813123517142913, -67.98741447168742980, -329.9779781133712504 ) ) ;
#25280=CARTESIAN_POINT ( 'NONE',  ( 795.1360043628807261, -164.0891481129655176, -360.2193346964456282 ) ) ;
#25282=CARTESIAN_POINT ( 'NONE',  ( 746.8695393053150156, -149.9073299311473875, -327.6429770376306010 ) ) ;
#25284=CARTESIAN_POINT ( 'NONE',  ( 758.0580252608178853, -126.4527844766019626, -328.0187753319985404 ) ) ;
#25286=CARTESIAN_POINT ( 'NONE',  ( 769.0155153010367712, -418.3726999360612808, -362.7791456095907279 ) ) ;
#25295=CARTESIAN_POINT ( 'NONE',  ( 776.9254006560222479, -380.1908817542431507, -314.8983024940802125 ) ) ;
#25298=CARTESIAN_POINT ( 'NONE',  ( 809.0717654672305343, -172.9181544815165239, -360.1688906516309885 ) ) ;
#25303=CARTESIAN_POINT ( 'NONE',  ( 787.6308680596127942, -323.2601417444138860, -364.1105419155492768 ) ) ;
#25305=CARTESIAN_POINT ( 'NONE',  ( 764.1737431748507561, -178.3726999360619629, -371.6461892240376415 ) ) ;
#25310=CARTESIAN_POINT ( 'NONE',  ( 759.0252816721024374, -216.9982390220562252, -368.0189434323527280 ) ) ;
#25312=CARTESIAN_POINT ( 'NONE',  ( 762.1405469898971887, -25.54369356751136877, -357.8594530101015607 ) ) ;
#25315=CARTESIAN_POINT ( 'NONE',  ( 810.1134526219336749, -104.5328690171418913, -357.8822607201570349 ) ) ;
#25317=CARTESIAN_POINT ( 'NONE',  ( 805.0032342141412300, -349.5436935675102745, -314.9967657858571783 ) ) ;
#25320=EDGE_CURVE ( 'NONE', #17032, #34365, #38322, .T. ) ;
#25323=CARTESIAN_POINT ( 'NONE',  ( 768.8385539511368734, -407.2601417444137155, -306.4236121716840557 ) ) ;
#25324=CARTESIAN_POINT ( 'NONE',  ( 782.4968714119720516, -418.8164208402374129, -305.0891759886411023 ) ) ;
#25328=CARTESIAN_POINT ( 'NONE',  ( 765.8855110935204493, -190.1692326535052189, -319.0159684113471599 ) ) ;
#25331=CARTESIAN_POINT ( 'NONE',  ( 771.2368401574024119, -205.4419599262324425, -374.2805881961240857 ) ) ;
#25332=( LENGTH_UNIT ( ) NAMED_UNIT ( * ) SI_UNIT ( .MILLI., .METRE. ) );
#25335=ORIENTED_EDGE ( 'NONE', *, *, #17898, .F. ) ;
#25337=CARTESIAN_POINT ( 'NONE',  ( 810.7187646348534145, -42.45278447660223264, -356.7737145352016341 ) ) ;
#25340=CARTESIAN_POINT ( 'NONE',  ( 812.3518521366052028, -433.0999726633339151, -326.5853460496235243 ) ) ;
#25346=CARTESIAN_POINT ( 'NONE',  ( 758.0580252608178853, -294.4527844766013800, -328.0187753319985404 ) ) ;
#25350=CARTESIAN_POINT ( 'NONE',  ( 784.1219089521767955, -285.2817908451526137, -315.0488828828318333 ) ) ;
#25351=CARTESIAN_POINT ( 'NONE',  ( 804.4286716492782716, -305.3618753856922581, -345.3141322388244703 ) ) ;
#25353=CARTESIAN_POINT ( 'NONE',  ( 802.1676090361156639, -110.6346026584201638, -327.8955696845344505 ) ) ;
#25357=DIRECTION ( 'NONE',  ( -0.000000000000000000, -0.000000000000000000, 1.000000000000000000 ) ) ;
#25358=CARTESIAN_POINT ( 'NONE',  ( 759.9999999999992042, 205.0000000000000568, -360.0000000000000000 ) ) ;
#25359=CARTESIAN_POINT ( 'NONE',  ( 750.9282345327678740, -88.91815448151682233, -319.8311093483690115 ) ) ;
#25365=CARTESIAN_POINT ( 'NONE',  ( 804.4086373105744769, -49.64542720878965554, -333.3843516231986541 ) ) ;
#25368=CARTESIAN_POINT ( 'NONE',  ( 772.4837098697145166, -119.3618753856928834, -374.5518280994205611 ) ) ;
#25370=CARTESIAN_POINT ( 'NONE',  ( 791.9812246680005501, -452.6346026584191691, -361.9419747391813189 ) ) ;
#25372=CARTESIAN_POINT ( 'NONE',  ( 751.6929314249748586, -246.9982390220560546, -318.8095938919659034 ) ) ;
#25376=CARTESIAN_POINT ( 'NONE',  ( 813.9316612368132837, -295.4419599262320730, -348.6739635108323228 ) ) ;
#25379=CARTESIAN_POINT ( 'NONE',  ( 810.7187646348534145, -306.4527844766013800, -356.7737145352016341 ) ) ;
#25383=CARTESIAN_POINT ( 'NONE',  ( 781.7834795799800531, -418.8164208402374129, -315.0636971347436202 ) ) ;
#25385=CARTESIAN_POINT ( 'NONE',  ( 803.4237431249931660, -207.1800572038744406, -331.2633955100225194 ) ) ;
#25386=CARTESIAN_POINT ( 'NONE',  ( 744.9990715423526808, -90.35105083532373271, -341.2370466360926002 ) ) ;
#25390=CARTESIAN_POINT ( 'NONE',  ( 796.7845633553578182, -225.6237781080506011, -358.5707757039688204 ) ) ;
#25392=CARTESIAN_POINT ( 'NONE',  ( 746.7653713866222915, -41.26014174441479554, -351.0478386215610271 ) ) ;
#25399=CARTESIAN_POINT ( 'NONE',  ( 760.0363995740630116, -346.9181544815160123, -368.7758568127991907 ) ) ;
#25402=CARTESIAN_POINT ( 'NONE',  ( 769.0155153010367712, -202.3726999360618777, -362.7791456095907279 ) ) ;
#25403=CARTESIAN_POINT ( 'NONE',  ( 756.5762568750052424, -171.1800572038745543, -348.7366044899774238 ) ) ;
#25404=CARTESIAN_POINT ( 'NONE',  ( 762.1405469898973024, -337.5436935675102745, -357.8594530101016176 ) ) ;
#25406=CARTESIAN_POINT ( 'NONE',  ( 804.1601925771018387, 16.55804007376685050, -346.5483106153029098 ) ) ;
#25416=CARTESIAN_POINT ( 'NONE',  ( 786.2694204179717872, -429.2817908451521021, -305.1769319972829067 ) ) ;
#25417=CARTESIAN_POINT ( 'NONE',  ( 763.2262854647970016, 15.36539734157940629, -309.2812353651462445 ) ) ;
#25420=CARTESIAN_POINT ( 'NONE',  ( 762.3223304703356007, -367.5436935675102745, -322.3223304703362828 ) ) ;
#25424=CARTESIAN_POINT ( 'NONE',  ( 755.8894580844503253, -255.8272453906072315, -332.3691319403863531 ) ) ;
#25435=CARTESIAN_POINT ( 'NONE',  ( 785.3141322388236176, -333.7255117493286320, -364.4286716492789537 ) ) ;
#25440=CARTESIAN_POINT ( 'NONE',  ( 749.5768839229115201, -60.55451811788051941, -358.0661480581553064 ) ) ;
#25441=CARTESIAN_POINT ( 'NONE',  ( 789.9200121543843807, -97.98741447168734453, -317.0176451133914384 ) ) ;
#25445=CARTESIAN_POINT ( 'NONE',  ( 762.3223304703356007, 16.45630643248849267, -322.3223304703362828 ) ) ;
#25446=CARTESIAN_POINT ( 'NONE',  ( 804.9511171171677688, -101.8055962898691718, -335.8780910478229202 ) ) ;
#25448=CARTESIAN_POINT ( 'NONE',  ( 756.5762568750052424, -99.18005720387478164, -348.7366044899774238 ) ) ;
#25451=CARTESIAN_POINT ( 'NONE',  ( 775.9200461376533440, -383.8055962898682765, -315.3028492785443291 ) ) ;
#25462=CARTESIAN_POINT ( 'NONE',  ( 763.8424801807145741, -90.00906357242590161, -320.5453621957614700 ) ) ;
#25464=CARTESIAN_POINT ( 'NONE',  ( 778.2165204200184689, -238.8164208402379813, -364.9363028652563230 ) ) ;
#25467=CARTESIAN_POINT ( 'NONE',  ( 785.3687786644884454, -395.3618753856918602, -315.3201227861279676 ) ) ;
#25468=CARTESIAN_POINT ( 'NONE',  ( 756.3353852180819104, -53.90732993114765037, -331.1735550268788302 ) ) ;
#25474=CARTESIAN_POINT ( 'NONE',  ( 804.9363028652555840, -16.27096629478413092, -338.2165204200192079 ) ) ;
#25477=CARTESIAN_POINT ( 'NONE',  ( 752.7379699480933368, -300.0090635724252479, -361.9858362298580232 ) ) ;
#25482=CARTESIAN_POINT ( 'NONE',  ( 756.3353852180819104, -269.9073299311468190, -331.1735550268788302 ) ) ;
#25484=CARTESIAN_POINT ( 'NONE',  ( 790.9844846989617508, -142.3726999360620766, -317.2208543904092721 ) ) ;
#25490=CARTESIAN_POINT ( 'NONE',  ( 776.2433038121456548, -12.89650538077851216, -374.8207195650711014 ) ) ;
#25491=CARTESIAN_POINT ( 'NONE',  ( 787.5162901302840055, -347.3618753856922012, -305.4481719005793252 ) ) ;
#25495=CARTESIAN_POINT ( 'NONE',  ( 773.7943932421234194, -215.8055962898687881, -305.5313806188329409 ) ) ;
#25497=CARTESIAN_POINT ( 'NONE',  ( 808.3070685750230950, 5.001760977943074948, -361.1904061080339261 ) ) ;
#25501=AXIS2_PLACEMENT_3D ( 'NONE', #43028, #29621, #19010 ) ;
#25503=CARTESIAN_POINT ( 'NONE',  ( 779.4709603349208464, 23.64894916467591912, -314.7162404726379918 ) ) ;
#25510=CARTESIAN_POINT ( 'NONE',  ( 761.2382568024794409, -303.6237781080503169, -356.9571628226838129 ) ) ;
#25512=CARTESIAN_POINT ( 'NONE',  ( 793.4146539503750546, -337.9874144716865771, -307.6481478633938877 ) ) ;
#25518=CARTESIAN_POINT ( 'NONE',  ( 800.7704444035546203, -76.16923265350557415, -326.0291762391768771 ) ) ;
#25521=CARTESIAN_POINT ( 'NONE',  ( 792.3570229623688874, -165.1800572038745258, -373.1304606946836202 ) ) ;
#25523=CARTESIAN_POINT ( 'NONE',  ( 802.1676090361155502, -134.6346026584201070, -327.8955696845344505 ) ) ;
#25525=CARTESIAN_POINT ( 'NONE',  ( 804.8461984189677878, -410.1908817542430370, -336.9566956441385628 ) ) ;
#25531=CARTESIAN_POINT ( 'NONE',  ( 779.9999999999992042, -462.9681489794448339, -370.0000000000000568 ) ) ;
#25535=CARTESIAN_POINT ( 'NONE',  ( 776.9254006560222479, -404.1908817542431507, -314.8983024940802125 ) ) ;
#25537=CARTESIAN_POINT ( 'NONE',  ( 807.2620300519052989, -192.0090635724255606, -318.0141637701419768 ) ) ;
#25542=CARTESIAN_POINT ( 'NONE',  ( 784.0799538623451781, -323.8055962898684470, -364.6971507214555572 ) ) ;
#25544=CARTESIAN_POINT ( 'NONE',  ( 748.6759233522253680, -184.3726999360619629, -324.3348316497537098 ) ) ;
#25546=CARTESIAN_POINT ( 'NONE',  ( 758.7867965644027208, 16.45630643248849267, -318.7867965644036872 ) ) ;
#25549=CARTESIAN_POINT ( 'NONE',  ( 813.1304606946831655, -233.9073299311470464, -352.3570229623691716 ) ) ;
#25551=CARTESIAN_POINT ( 'NONE',  ( 762.3223304703356007, -7.543693567511430942, -322.3223304703362828 ) ) ;
#25554=CARTESIAN_POINT ( 'NONE',  ( 749.8865473780648472, -92.53286901714190549, -322.1177392798429082 ) ) ;
#25556=CARTESIAN_POINT ( 'NONE',  ( 777.5031285880264704, -382.8164208402374697, -374.9108240113588408 ) ) ;
#25557=CIRCLE ( 'NONE', #27033, 10.00000000000000888 ) ;
#25563=CARTESIAN_POINT ( 'NONE',  ( 754.0944755984390895, -399.6237781080500326, -364.1009440267246760 ) ) ;
#25564=CARTESIAN_POINT ( 'NONE',  ( 801.1904061080336987, -452.0891481129646650, -368.3070685750235498 ) ) ;
#25566=EDGE_CURVE ( 'NONE', #14504, #5020, #17986, .T. ) ;
#25569=CARTESIAN_POINT ( 'NONE',  ( 779.4709603349208464, -192.3510508353233774, -314.7162404726379918 ) ) ;
#25571=CARTESIAN_POINT ( 'NONE',  ( 811.6461892240364477, -172.7146871989598083, -324.1737431748509835 ) ) ;
#25576=CARTESIAN_POINT ( 'NONE',  ( 758.0580252608178853, -150.4527844766018916, -328.0187753319985404 ) ) ;
#25579=CARTESIAN_POINT ( 'NONE',  ( 796.7737145352015204, -44.63460265842040542, -370.7187646348536987 ) ) ;
#25580=EDGE_CURVE ( 'NONE', #20167, #26190, #4576, .T. ) ;
#25582=CARTESIAN_POINT ( 'NONE',  ( 793.5525998758768083, -439.0999726633339719, -372.6845335610516941 ) ) ;
#25585=CARTESIAN_POINT ( 'NONE',  ( 790.9844846989617508, -310.3726999360616219, -317.2208543904092721 ) ) ;
#25590=CARTESIAN_POINT ( 'NONE',  ( 803.4237431249931660, -303.1800572038740711, -331.2633955100225194 ) ) ;
#25595=CARTESIAN_POINT ( 'NONE',  ( 755.5913626894240451, -277.6454272087889308, -346.6156483768012890 ) ) ;
#25596=CARTESIAN_POINT ( 'NONE',  ( 764.8639956371174549, -272.0891481129651197, -319.7806653035542013 ) ) ;
#25598=CARTESIAN_POINT ( 'NONE',  ( 801.9419747391806368, -114.4527844766020053, -351.9812246680014027 ) ) ;
#25604=CARTESIAN_POINT ( 'NONE',  ( 760.0363995740630116, -82.91815448151682233, -368.7758568127991907 ) ) ;
#25610=CARTESIAN_POINT ( 'NONE',  ( 777.4774526936600978, -106.2709662947838467, -304.7301800767028226 ) ) ;
#25614=CARTESIAN_POINT ( 'NONE',  ( 748.9653473494363425, -242.6346026584197659, -356.9462024416521331 ) ) ;
#25618=CARTESIAN_POINT ( 'NONE',  ( 810.1134526219336749, -296.5328690171411949, -357.8822607201570349 ) ) ;
#25621=CARTESIAN_POINT ( 'NONE',  ( 754.9967657858570647, -313.5436935675102745, -365.0032342141425374 ) ) ;
#25625=CARTESIAN_POINT ( 'NONE',  ( 788.8264449731200330, -405.1800572038737300, -363.6646147819171233 ) ) ;
#25627=CARTESIAN_POINT ( 'NONE',  ( 785.3687786644884454, -227.3618753856925707, -315.3201227861279676 ) ) ;
#25628=CARTESIAN_POINT ( 'NONE',  ( 778.7502325331095108, -96.35105083532370429, -304.6391490659818828 ) ) ;
#25633=CARTESIAN_POINT ( 'NONE',  ( 802.7791456095903868, -220.7146871989596661, -329.0155153010375102 ) ) ;
#25635=CARTESIAN_POINT ( 'NONE',  ( 756.1443688327750579, -69.62377810805107003, -314.3581564841659315 ) ) ;
#25636=CARTESIAN_POINT ( 'NONE',  ( 808.7373736539768743, -452.9681489794446065, -336.0792598452978268 ) ) ;
#25638=CARTESIAN_POINT ( 'NONE',  ( 781.2370466360911223, -356.7363362996978253, -304.9990715423533629 ) ) ;
#25642=CARTESIAN_POINT ( 'NONE',  ( 804.8461984189677878, -170.1908817542438328, -336.9566956441385628 ) ) ;
#25643=CARTESIAN_POINT ( 'NONE',  ( 755.0636971347428243, -196.2709662947835909, -341.7834795799807353 ) ) ;
#25644=CARTESIAN_POINT ( 'NONE',  ( 757.8323909638828582, -386.6346026584192828, -352.1044303154654358 ) ) ;
#25646=CARTESIAN_POINT ( 'NONE',  ( 772.3691319403857278, 24.73985825558500551, -315.8894580844506663 ) ) ;
#25652=CARTESIAN_POINT ( 'NONE',  ( 772.4999999999993179, -462.9681489794447202, -270.0000000000000568 ) ) ;
#25656=CARTESIAN_POINT ( 'NONE',  ( 814.4686193811664907, -411.2817908451521589, -346.2056067578752732 ) ) ;
#25657=CARTESIAN_POINT ( 'NONE',  ( 812.7932403749906598, -15.18005720387504631, -327.7687537140311633 ) ) ;
#25660=CARTESIAN_POINT ( 'NONE',  ( 778.1981804954714335, -370.2709662947831362, -314.8072714833589885 ) ) ;
#25663=LINE ( 'NONE', #7428, #32574 ) ;
#25664=CARTESIAN_POINT ( 'NONE',  ( 804.1105419155481968, -243.8272453906072030, -347.6308680596136469 ) ) ;
#25672=CARTESIAN_POINT ( 'NONE',  ( 757.8323909638827445, -314.6346026584194533, -352.1044303154654358 ) ) ;
#25676=CARTESIAN_POINT ( 'NONE',  ( 802.2119215644370342, -78.00906357242591582, -367.5423716828165084 ) ) ;
#25677=CARTESIAN_POINT ( 'NONE',  ( 758.6633372737375112, -116.5328690171418202, -326.9102291470432533 ) ) ;
#25682=CARTESIAN_POINT ( 'NONE',  ( 791.9812246680005501, -20.63460265842048003, -361.9419747391813189 ) ) ;
#25683=CARTESIAN_POINT ( 'NONE',  ( 783.0433043558608688, -120.8965053807781800, -315.1538015810313027 ) ) ;
#25684=CARTESIAN_POINT ( 'NONE',  ( 774.6858677611749044, -105.7255117493293000, -315.5713283507209894 ) ) ;
#25685=CARTESIAN_POINT ( 'NONE',  ( 795.9930595647434757, -435.0783235625953580, -320.7433823573372820 ) ) ;
#25696=ORIENTED_EDGE ( 'NONE', *, *, #4683, .T. ) ;
#25697=CARTESIAN_POINT ( 'NONE',  ( 796.1575198192839480, -78.00906357242591582, -359.4546378042384163 ) ) ;
#25699=CARTESIAN_POINT ( 'NONE',  ( 755.5713283507202505, -269.3618753856924286, -334.6858677611754729 ) ) ;
#25700=ORIENTED_EDGE ( 'NONE', *, *, #26355, .T. ) ;
#25701=CARTESIAN_POINT ( 'NONE',  ( 774.6858677611749044, -393.7255117493283478, -315.5713283507209894 ) ) ;
#25702=CARTESIAN_POINT ( 'NONE',  ( 771.1735550268778070, -33.18005720387498769, -316.3353852180827630 ) ) ;
#25706=CARTESIAN_POINT ( 'NONE',  ( 745.1792804349281596, -14.19088175424431242, -343.7566961878542884 ) ) ;
#25709=CARTESIAN_POINT ( 'NONE',  ( 746.4236121716829757, -303.8272453906071178, -328.8385539511384650 ) ) ;
#25713=CARTESIAN_POINT ( 'NONE',  ( 767.8955696845333705, -240.4527844766015221, -362.1676090361162323 ) ) ;
#25715=CARTESIAN_POINT ( 'NONE',  ( 755.3028492785439312, -159.2817908451529547, -335.9200461376539693 ) ) ;
#25718=CARTESIAN_POINT ( 'NONE',  ( 773.7943932421234194, -23.80559628986938847, -305.5313806188329409 ) ) ;
#25719=CARTESIAN_POINT ( 'NONE',  ( 792.3570229623691148, -357.1800572038739574, -373.1304606946836770 ) ) ;
#25723=CARTESIAN_POINT ( 'NONE',  ( 811.6461892240364477, -220.7146871989596661, -324.1737431748509835 ) ) ;
#25725=CARTESIAN_POINT ( 'NONE',  ( 777.4774526936600978, 13.72903370521577138, -304.7301800767027657 ) ) ;
#25730=CARTESIAN_POINT ( 'NONE',  ( 804.9511171171677688, -29.80559628986937781, -335.8780910478229202 ) ) ;
#25736=CARTESIAN_POINT ( 'NONE',  ( 795.9930595647434757, -291.0783235625957559, -320.7433823573372820 ) ) ;
#25738=CARTESIAN_POINT ( 'NONE',  ( 815.1787889125755555, -318.8965053807775121, -343.7953271457877804 ) ) ;
#25744=CARTESIAN_POINT ( 'NONE',  ( 760.5453621957607311, -93.07832356259645223, -323.8424801807151425 ) ) ;
#25748=CARTESIAN_POINT ( 'NONE',  ( 758.8095938919642549, -200.0891481129653187, -311.6929314249763365 ) ) ;
#25750=CARTESIAN_POINT ( 'NONE',  ( 795.1360043628808398, -140.0891481129655176, -360.2193346964456282 ) ) ;
#25752=CARTESIAN_POINT ( 'NONE',  ( 804.4086373105744769, -409.6454272087884760, -333.3843516231986541 ) ) ;
#25759=CARTESIAN_POINT ( 'NONE',  ( 802.5472867521000353, -388.3726999360613945, -350.8726784830461156 ) ) ;
#25761=CARTESIAN_POINT ( 'NONE',  ( 766.4474001241216001, -211.0999726633346540, -307.3154664389482491 ) ) ;
#25765=CARTESIAN_POINT ( 'NONE',  ( 769.1273215169530886, -310.7146871989593251, -317.4527132478988847 ) ) ;
#25767=CARTESIAN_POINT ( 'NONE',  ( 754.3581564841646241, -185.4636090269710280, -316.1443688327762516 ) ) ;
#25771=CARTESIAN_POINT ( 'NONE',  ( 772.5602148656447525, -249.7255117493288594, -305.7998596910095443 ) ) ;
#25773=CARTESIAN_POINT ( 'NONE',  ( 755.5713283507202505, -5.361875385693257279, -334.6858677611754729 ) ) ;
#25776=CARTESIAN_POINT ( 'NONE',  ( 773.7943932421234194, -143.8055962898690154, -305.5313806188329409 ) ) ;
#25778=CARTESIAN_POINT ( 'NONE',  ( 759.0252816721024374, -360.9982390220557704, -368.0189434323527280 ) ) ;
#25783=CARTESIAN_POINT ( 'NONE',  ( 773.7305795820266212, -9.281790845153418346, -374.8230680027170365 ) ) ;
#25788=CARTESIAN_POINT ( 'NONE',  ( 796.7845633553578182, -201.6237781080506863, -358.5707757039688204 ) ) ;
#25790=CARTESIAN_POINT ( 'NONE',  ( 783.7566961878529810, -240.8965053807777963, -305.1792804349288417 ) ) ;
#25796=CARTESIAN_POINT ( 'NONE',  ( 777.4774526936600978, -58.27096629478398171, -304.7301800767027657 ) ) ;
#25798=EDGE_LOOP ( 'NONE', ( #18713, #43964 ) ) ;
#25799=CARTESIAN_POINT ( 'NONE',  ( 776.2046728542105711, -452.1908817542428665, -304.8212110874238761 ) ) ;
#25801=CARTESIAN_POINT ( 'NONE',  ( 780.5236548040995785, -308.7363362996979390, -314.9735926884559944 ) ) ;
#25804=CARTESIAN_POINT ( 'NONE',  ( 755.3201227861273992, -291.7255117493285752, -345.3687786644892981 ) ) ;
#25807=CARTESIAN_POINT ( 'NONE',  ( 787.5531968255692163, -285.8272453906071178, -316.1348686366205811 ) ) ;
#25808=CARTESIAN_POINT ( 'NONE',  ( 768.0187753319979720, -296.6346026584195670, -318.0580252608186242 ) ) ;
#25810=CARTESIAN_POINT ( 'NONE',  ( 792.1044303154645831, -156.4527844766018916, -317.8323909638837677 ) ) ;
#25816=CARTESIAN_POINT ( 'NONE',  ( 749.5768839229115201, -84.55451811788046257, -358.0661480581553064 ) ) ;
#25822=CARTESIAN_POINT ( 'NONE',  ( 751.6929314249750860, -126.9982390220565094, -318.8095938919659034 ) ) ;
#25824=PLANE ( 'NONE',  #14578 ) ;
#25825=CARTESIAN_POINT ( 'NONE',  ( 766.7756240680305382, -422.5328690171408539, -361.5560724626415663 ) ) ;
#25827=CARTESIAN_POINT ( 'NONE',  ( 746.8695393053150156, -269.9073299311468190, -327.6429770376306010 ) ) ;
#25831=CARTESIAN_POINT ( 'NONE',  ( 801.9858362298568863, -315.0783235625957559, -312.7379699480935642 ) ) ;
#25834=CARTESIAN_POINT ( 'NONE',  ( 745.4481719005789273, -339.7255117493285184, -347.5162901302853129 ) ) ;
#25838=CARTESIAN_POINT ( 'NONE',  ( 755.0636971347428243, -412.2709662947829088, -341.7834795799807353 ) ) ;
#25840=CARTESIAN_POINT ( 'NONE',  ( 759.9864689768902508, -218.0891481129653187, -354.9819416627836404 ) ) ;
#25841=CARTESIAN_POINT ( 'NONE',  ( 749.8865473780648472, -116.5328690171418202, -322.1177392798429082 ) ) ;
#25846=CARTESIAN_POINT ( 'NONE',  ( 754.8983024940795303, -234.8965053807777963, -336.9254006560228163 ) ) ;
#25850=CARTESIAN_POINT ( 'NONE',  ( 813.2346286133761168, -53.26014174441475291, -328.9521613784389160 ) ) ;
#25854=CARTESIAN_POINT ( 'NONE',  ( 799.9636004259356241, -334.9181544815160692, -311.2241431872006956 ) ) ;
#25857=CARTESIAN_POINT ( 'NONE',  ( 754.7162404726377645, -182.7363362996983369, -339.4709603349214717 ) ) ;
#25858=CARTESIAN_POINT ( 'NONE',  ( 767.8955696845333705, -192.4527844766016926, -362.1676090361162323 ) ) ;
#25859=CARTESIAN_POINT ( 'NONE',  ( 781.7834795799800531, -370.8164208402375834, -315.0636971347436202 ) ) ;
#25861=CARTESIAN_POINT ( 'NONE',  ( 790.8050863131179540, -452.8379544210779954, -362.5841948692291226 ) ) ;
#25862=VERTEX_POINT ( 'NONE', #5707 ) ;
#25863=CARTESIAN_POINT ( 'NONE',  ( 779.9999999999992042, -452.9681489794448339, -339.9999999999999432 ) ) ;
#25868=CARTESIAN_POINT ( 'NONE',  ( 748.6759233522253680, -424.3726999360612808, -324.3348316497537098 ) ) ;
#25869=CARTESIAN_POINT ( 'NONE',  ( 748.9653473494365699, -26.63460265842046226, -356.9462024416520762 ) ) ;
#25871=CARTESIAN_POINT ( 'NONE',  ( 759.9864689768902508, -386.0891481129647786, -354.9819416627836404 ) ) ;
#25872=CARTESIAN_POINT ( 'NONE',  ( 804.9363028652555840, 7.729033705215793582, -338.2165204200192079 ) ) ;
#25875=CARTESIAN_POINT ( 'NONE',  ( 784.1219089521767955, -261.2817908451526705, -315.0488828828318333 ) ) ;
#25876=CARTESIAN_POINT ( 'NONE',  ( 792.2312462859673587, -179.9073299311472454, -307.2067596250082602 ) ) ;
#25884=CARTESIAN_POINT ( 'NONE',  ( 792.1044303154645831, -300.4527844766012663, -317.8323909638837677 ) ) ;
#25886=CARTESIAN_POINT ( 'NONE',  ( 745.5313806188320314, -63.28179084515324604, -333.7943932421247268 ) ) ;
#25887=CARTESIAN_POINT ( 'NONE',  ( 798.7617431975189675, -123.6237781080508569, -323.0428371773161871 ) ) ;
#25892=CARTESIAN_POINT ( 'NONE',  ( 805.1927285166397041, -16.81642084023866701, -341.8018195045277707 ) ) ;
#25893=CARTESIAN_POINT ( 'NONE',  ( 760.5453621957607311, -117.0783235625963528, -323.8424801807151425 ) ) ;
#25894=CARTESIAN_POINT ( 'NONE',  ( 792.1044303154645831, -132.4527844766018916, -317.8323909638837677 ) ) ;
#25895=CARTESIAN_POINT ( 'NONE',  ( 783.7566961878529810, 23.10349461922137237, -305.1792804349288417 ) ) ;
#25908=CARTESIAN_POINT ( 'NONE',  ( 790.0220218866281812, -79.09997266333503774, -363.2186876482849129 ) ) ;
#25910=CARTESIAN_POINT ( 'NONE',  ( 755.3201227861273992, -267.7255117493287457, -345.3687786644892981 ) ) ;
#25912=CARTESIAN_POINT ( 'NONE',  ( 754.8072714833581358, -388.8164208402374129, -338.1981804954720587 ) ) ;
#25913=CARTESIAN_POINT ( 'NONE',  ( 797.6776695296629214, -43.54369356751131903, -357.6776695296636603 ) ) ;
#25917=CARTESIAN_POINT ( 'NONE',  ( 802.2119215644370342, -30.00906357242607925, -367.5423716828165084 ) ) ;
#25920=CARTESIAN_POINT ( 'NONE',  ( 773.7305795820266212, -321.2817908451525000, -374.8230680027170365 ) ) ;
#25923=CARTESIAN_POINT ( 'NONE',  ( 788.8264449731200330, -309.1800572038740711, -363.6646147819171233 ) ) ;
#25925=CARTESIAN_POINT ( 'NONE',  ( 790.0220218866281812, -151.0999726633347677, -363.2186876482849129 ) ) ;
#25929=CARTESIAN_POINT ( 'NONE',  ( 812.6845335610512393, -7.987414471687621642, -353.5525998758768651 ) ) ;
#25930=CARTESIAN_POINT ( 'NONE',  ( 751.9810565676468741, -338.0891481129649492, -360.9747183278973921 ) ) ;
#25931=DIRECTION ( 'NONE',  ( 0.3826814224632300032, 0.000000000000000000, -0.9238803650373347276 ) ) ;
#25934=CARTESIAN_POINT ( 'NONE',  ( 791.1614460488616487, -251.2601417444141134, -373.5763878283158874 ) ) ;
#25936=CARTESIAN_POINT ( 'NONE',  ( 792.3570229623688874, 2.819942796124898177, -373.1304606946836202 ) ) ;
#25941=CARTESIAN_POINT ( 'NONE',  ( 798.7617431975189675, -3.623778108051270319, -323.0428371773161871 ) ) ;
#25946=CARTESIAN_POINT ( 'NONE',  ( 804.1601925771018387, -343.4419599262320162, -346.5483106153029098 ) ) ;
#25948=CARTESIAN_POINT ( 'NONE',  ( 768.8385539511368734, -335.2601417444137724, -306.4236121716840557 ) ) ;
#25953=CARTESIAN_POINT ( 'NONE',  ( 794.1144889064781864, -82.16923265350558836, -360.9840315886528401 ) ) ;
#25956=CARTESIAN_POINT ( 'NONE',  ( 810.7187646348534145, -186.4527844766017779, -356.7737145352016341 ) ) ;
#25959=CARTESIAN_POINT ( 'NONE',  ( 759.7806653035535192, -174.9982390220563673, -324.8639956371181370 ) ) ;
#25961=CARTESIAN_POINT ( 'NONE',  ( 804.1105419155481968, -435.8272453906066062, -347.6308680596136469 ) ) ;
#25968=CARTESIAN_POINT ( 'NONE',  ( 757.4527132478984868, -424.3726999360612808, -329.1273215169538844 ) ) ;
#25970=CARTESIAN_POINT ( 'NONE',  ( 809.0717654672305343, -220.9181544815164102, -360.1688906516309885 ) ) ;
#25974=CARTESIAN_POINT ( 'NONE',  ( 800.7704444035546203, -316.1692326535048210, -326.0291762391768771 ) ) ;
#25976=CARTESIAN_POINT ( 'NONE',  ( 814.2805881961230625, -217.6454272087891582, -331.2368401574024119 ) ) ;
#25981=CARTESIAN_POINT ( 'NONE',  ( 746.8695393053151292, -245.9073299311469896, -327.6429770376306578 ) ) ;
#25983=CARTESIAN_POINT ( 'NONE',  ( 757.8323909638827445, -26.63460265842045871, -352.1044303154654358 ) ) ;
#25985=CARTESIAN_POINT ( 'NONE',  ( 812.6845335610512393, -127.9874144716872308, -353.5525998758768651 ) ) ;
#25987=CARTESIAN_POINT ( 'NONE',  ( 751.6929314249748586, -366.9982390220556567, -318.8095938919659034 ) ) ;
#25992=CARTESIAN_POINT ( 'NONE',  ( 755.3201227861273992, -387.7255117493283478, -345.3687786644892981 ) ) ;
#25993=CARTESIAN_POINT ( 'NONE',  ( 812.3518521366052028, -1.099972663335260226, -326.5853460496235243 ) ) ;
#25994=DIRECTION ( 'NONE',  ( -1.000000000000000000, -0.000000000000000000, -0.000000000000000000 ) ) ;
#25997=CARTESIAN_POINT ( 'NONE',  ( 757.2208543904082489, -232.7146871989596377, -350.9844846989624330 ) ) ;
#25999=CARTESIAN_POINT ( 'NONE',  ( 744.8212110874229666, -210.8965053807778816, -336.2046728542121627 ) ) ;
#26004=CARTESIAN_POINT ( 'NONE',  ( 804.4286716492782716, -137.3618753856928265, -345.3141322388244703 ) ) ;
#26006=CARTESIAN_POINT ( 'NONE',  ( 747.2067596250078623, -75.18005720387485269, -352.2312462859687230 ) ) ;
#26008=CARTESIAN_POINT ( 'NONE',  ( 778.2165204200184689, -70.81642084023850714, -364.9363028652563230 ) ) ;
#26010=CARTESIAN_POINT ( 'NONE',  ( 769.0155153010367712, -10.37269993606250473, -362.7791456095907279 ) ) ;
#26012=CARTESIAN_POINT ( 'NONE',  ( 754.7162404726377645, -326.7363362996979390, -339.4709603349214717 ) ) ;
#26015=CARTESIAN_POINT ( 'NONE',  ( 785.3141322388236176, -333.7255117493286320, -364.4286716492789537 ) ) ;
#26020=CARTESIAN_POINT ( 'NONE',  ( 790.9844846989617508, -334.3726999360615082, -317.2208543904092721 ) ) ;
#26021=CARTESIAN_POINT ( 'NONE',  ( 800.2193346964447755, -282.9982390220558841, -355.1360043628815788 ) ) ;
#26023=CARTESIAN_POINT ( 'NONE',  ( 803.6646147819161570, -137.9073299311473875, -348.8264449731210561 ) ) ;
#26028=CARTESIAN_POINT ( 'NONE',  ( 814.4686193811664907, -75.28179084515321051, -346.2056067578752732 ) ) ;
#26029=DIRECTION ( 'NONE',  ( -1.000000000000000000, -0.000000000000000000, -0.000000000000000000 ) ) ;
#26035=CARTESIAN_POINT ( 'NONE',  ( 815.2698199232962679, -136.8164208402382656, -342.5225473063383674 ) ) ;
#26038=CARTESIAN_POINT ( 'NONE',  ( 811.0346526505616112, -278.6346026584196807, -323.0537975583477532 ) ) ;
#26043=CARTESIAN_POINT ( 'NONE',  ( 768.8385539511368734, -359.2601417444137724, -306.4236121716840557 ) ) ;
#26045=CARTESIAN_POINT ( 'NONE',  ( 777.4774526936600978, -106.2709662947838467, -304.7301800767027657 ) ) ;
#26047=CARTESIAN_POINT ( 'NONE',  ( 747.2067596250078623, -339.1800572038740142, -352.2312462859687230 ) ) ;
#26052=CARTESIAN_POINT ( 'NONE',  ( 774.6312213355099630, -431.3618753856918033, -364.6798772138717482 ) ) ;
#26053=CARTESIAN_POINT ( 'NONE',  ( 764.8639956371174549, -224.0891481129653187, -319.7806653035542013 ) ) ;
#26054=CARTESIAN_POINT ( 'NONE',  ( 746.0683387631852383, -115.4419599262327409, -331.3260364891676204 ) ) ;
#26059=CARTESIAN_POINT ( 'NONE',  ( 805.0264073115434940, -246.3510508353232638, -339.4763451958999099 ) ) ;
#26061=CARTESIAN_POINT ( 'NONE',  ( 805.9055244015594326, -435.6237781080499190, -315.8990559732753240 ) ) ;
#26062=CARTESIAN_POINT ( 'NONE',  ( 773.7943932421234194, -71.80559628986922860, -305.5313806188329409 ) ) ;
#26066=CARTESIAN_POINT ( 'NONE',  ( 811.3240766477731540, -388.3726999360613945, -355.6651683502462902 ) ) ;
#26069=CARTESIAN_POINT ( 'NONE',  ( 783.0745993439762742, -176.1908817542438328, -365.1016975059196739 ) ) ;
#26070=CARTESIAN_POINT ( 'NONE',  ( 759.9864689768902508, -170.0891481129654608, -354.9819416627836404 ) ) ;
#26072=CARTESIAN_POINT ( 'NONE',  ( 804.6798772138710092, -399.7255117493283478, -334.6312213355106451 ) ) ;
#26076=CARTESIAN_POINT ( 'NONE',  ( 780.5290396650775619, 11.64894916467595642, -365.2837595273619513 ) ) ;
#26082=DIRECTION ( 'NONE',  ( 0.000000000000000000, -1.000000000000000000, 0.000000000000000000 ) ) ;
#26087=ORIENTED_EDGE ( 'NONE', *, *, #11778, .F. ) ;
#26088=CARTESIAN_POINT ( 'NONE',  ( 781.2370466360911223, -404.7363362996975980, -304.9990715423533629 ) ) ;
#26089=CARTESIAN_POINT ( 'NONE',  ( 772.5602148656447525, -33.72551174932952733, -305.7998596910095443 ) ) ;
#26091=CARTESIAN_POINT ( 'NONE',  ( 800.2193346964447755, -402.9982390220555430, -355.1360043628815788 ) ) ;
#26092=CARTESIAN_POINT ( 'NONE',  ( 765.0180583372156207, -0.9982390220569063999, -360.0135310231089534 ) ) ;
#26096=CARTESIAN_POINT ( 'NONE',  ( 761.4292242960306112, -257.4636090269708575, -323.2154366446414429 ) ) ;
#26098=CARTESIAN_POINT ( 'NONE',  ( 787.4397851343537695, -165.7255117493291152, -374.2001403089903988 ) ) ;
#26102=CARTESIAN_POINT ( 'NONE',  ( 790.2803779376845341, 16.45630643248849623, -314.3272116953297086 ) ) ;
#26107=CARTESIAN_POINT ( 'NONE',  ( 785.3687786644884454, -323.3618753856923149, -315.3201227861279676 ) ) ;
#26111=CARTESIAN_POINT ( 'NONE',  ( 745.5313806188320314, -111.2817908451530968, -333.7943932421247268 ) ) ;
#26112=CARTESIAN_POINT ( 'NONE',  ( 787.6308680596127942, -107.2601417444145824, -364.1105419155492768 ) ) ;
#26118=CARTESIAN_POINT ( 'NONE',  ( 804.6798772138708955, -15.72551174932958951, -334.6312213355107019 ) ) ;
#26119=CARTESIAN_POINT ( 'NONE',  ( 766.7756240680305382, -134.5328690171417350, -361.5560724626415663 ) ) ;
#26120=CARTESIAN_POINT ( 'NONE',  ( 755.3201227861273992, -123.7255117493292147, -345.3687786644892981 ) ) ;
#26122=CARTESIAN_POINT ( 'NONE',  ( 796.7845633553578182, -441.6237781080499190, -358.5707757039688204 ) ) ;
#26128=CARTESIAN_POINT ( 'NONE',  ( 807.2620300519052989, -264.0090635724253616, -318.0141637701419768 ) ) ;
#26137=CARTESIAN_POINT ( 'NONE',  ( 759.0159684113467620, -64.91815448151686496, -325.8855110935213020 ) ) ;
#26138=CARTESIAN_POINT ( 'NONE',  ( 771.1735550268780344, -273.1800572038742985, -316.3353852180828198 ) ) ;
#26140=CARTESIAN_POINT ( 'NONE',  ( 778.2165204200184689, -406.8164208402375266, -364.9363028652563230 ) ) ;
#26141=CARTESIAN_POINT ( 'NONE',  ( 755.5713283507202505, -53.36187538569310362, -334.6858677611754729 ) ) ;
#26148=CARTESIAN_POINT ( 'NONE',  ( 791.0478386215596629, -21.82724539060792424, -306.7653713866226326 ) ) ;
#26151=CARTESIAN_POINT ( 'NONE',  ( 760.0363995740630116, -298.9181544815161828, -368.7758568127991907 ) ) ;
#26156=CARTESIAN_POINT ( 'NONE',  ( 785.3687786644884454, -275.3618753856923149, -315.3201227861279676 ) ) ;
#26158=CARTESIAN_POINT ( 'NONE',  ( 776.9254006560222479, -164.1908817542438612, -314.8983024940802125 ) ) ;
#26161=CARTESIAN_POINT ( 'NONE',  ( 748.3538107759620743, -16.71468719896031985, -355.8262568251490165 ) ) ;
#26162=CARTESIAN_POINT ( 'NONE',  ( 777.4774526936600978, -346.2709662947830225, -304.7301800767028226 ) ) ;
#26169=CARTESIAN_POINT ( 'NONE',  ( 792.2312462859673587, 12.09267006885214180, -307.2067596250082602 ) ) ;
#26175=CARTESIAN_POINT ( 'NONE',  ( 770.0799878456142551, -13.98741447168760033, -362.9823548866085616 ) ) ;
#26180=CARTESIAN_POINT ( 'NONE',  ( 795.1360043628807261, -44.08914811296584446, -360.2193346964456282 ) ) ;
#26182=CARTESIAN_POINT ( 'NONE',  ( 789.9200121543843807, -313.9874144716866908, -317.0176451133914384 ) ) ;
#26185=CARTESIAN_POINT ( 'NONE',  ( 778.7502325331095108, -312.3510508353230080, -304.6391490659818828 ) ) ;
#26190=VERTEX_POINT ( 'NONE', #34783 ) ;
#26192=CARTESIAN_POINT ( 'NONE',  ( 814.5518280994195948, -183.7255117493290015, -332.4837098697145734 ) ) ;
#26196=CARTESIAN_POINT ( 'NONE',  ( 755.3201227861273992, -171.7255117493290868, -345.3687786644892981 ) ) ;
#26198=CARTESIAN_POINT ( 'NONE',  ( 783.0745993439762742, -440.1908817542430370, -365.1016975059196739 ) ) ;
#26199=VECTOR ( 'NONE', #43557, 1000.000000000000000 ) ;
#26206=ORIENTED_EDGE ( 'NONE', *, *, #27246, .F. ) ;
#26207=CARTESIAN_POINT ( 'NONE',  ( 763.8424801807145741, -426.0090635724247932, -320.5453621957614700 ) ) ;
#26209=CARTESIAN_POINT ( 'NONE',  ( 752.7379699480933368, -204.0090635724255606, -361.9858362298580232 ) ) ;
#26212=CARTESIAN_POINT ( 'NONE',  ( 754.8072714833581358, -172.8164208402381234, -338.1981804954720587 ) ) ;
#26213=CARTESIAN_POINT ( 'NONE',  ( 761.2382568024794409, -327.6237781080502600, -356.9571628226838129 ) ) ;
#26215=CARTESIAN_POINT ( 'NONE',  ( 752.7379699480933368, -228.0090635724254753, -361.9858362298580232 ) ) ;
#26216=DIRECTION ( 'NONE',  ( 1.000000000000000000, 0.000000000000000000, -0.000000000000000000 ) ) ;
#26218=CARTESIAN_POINT ( 'NONE',  ( 779.4763451958990572, -56.73633629969872771, -365.0264073115438919 ) ) ;
#26221=CARTESIAN_POINT ( 'NONE',  ( 782.4968714119720516, -250.8164208402379245, -305.0891759886411023 ) ) ;
#26224=CARTESIAN_POINT ( 'NONE',  ( 788.8264449731200330, 2.819942796124898177, -363.6646147819171233 ) ) ;
#26227=CARTESIAN_POINT ( 'NONE',  ( 758.0141637701419768, -135.0783235625962959, -367.2620300519063790 ) ) ;
#26229=CARTESIAN_POINT ( 'NONE',  ( 748.9653473494363425, -362.6346026584194533, -356.9462024416521331 ) ) ;
#26235=CARTESIAN_POINT ( 'NONE',  ( 759.7806653035534055, -390.9982390220557136, -324.8639956371180801 ) ) ;
#26238=CARTESIAN_POINT ( 'NONE',  ( 804.7487373415286811, -451.5436935675099903, -364.7487373415288516 ) ) ;
#26243=CARTESIAN_POINT ( 'NONE',  ( 787.6308680596127942, -227.2601417444141987, -364.1105419155492768 ) ) ;
#26245=CARTESIAN_POINT ( 'NONE',  ( 752.4576283171824116, -213.0783235625960401, -317.7880784355627952 ) ) ;
#26249=CARTESIAN_POINT ( 'NONE',  ( 771.1735550268778070, -153.1800572038746395, -316.3353852180827630 ) ) ;
#26251=CARTESIAN_POINT ( 'NONE',  ( 812.7932403749906598, -63.18005720387488822, -327.7687537140311633 ) ) ;
#26252=CARTESIAN_POINT ( 'NONE',  ( 755.3201227861273992, -75.72551174932938522, -345.3687786644892981 ) ) ;
#26254=CARTESIAN_POINT ( 'NONE',  ( 757.0176451133909268, -13.09997266333522248, -349.9200121543848354 ) ) ;
#26256=ORIENTED_EDGE ( 'NONE', *, *, #40134, .F. ) ;
#26257=CARTESIAN_POINT ( 'NONE',  ( 786.5483106153019435, -319.6454272087888739, -364.1601925771022366 ) ) ;
#26264=CARTESIAN_POINT ( 'NONE',  ( 780.5236548040995785, -308.7363362996979390, -314.9735926884559944 ) ) ;
#26265=CARTESIAN_POINT ( 'NONE',  ( 755.0636971347428243, -316.2709662947832499, -341.7834795799807353 ) ) ;
#26266=CARTESIAN_POINT ( 'NONE',  ( 805.1927285166397041, -160.8164208402382371, -341.8018195045277707 ) ) ;
#26271=CARTESIAN_POINT ( 'NONE',  ( 804.1009440267234822, -119.4636090269712554, -314.0944755984392600 ) ) ;
#26278=CARTESIAN_POINT ( 'NONE',  ( 787.5162901302840055, -131.3618753856928549, -305.4481719005793252 ) ) ;
#26281=CARTESIAN_POINT ( 'NONE',  ( 796.9462024416508257, -276.4527844766013800, -308.9653473494370246 ) ) ;
#26282=CARTESIAN_POINT ( 'NONE',  ( 749.2812353651451076, -438.4527844766009821, -323.2262854647983090 ) ) ;
#26285=CARTESIAN_POINT ( 'NONE',  ( 758.0141637701419768, -351.0783235625955854, -367.2620300519063790 ) ) ;
#26286=CARTESIAN_POINT ( 'NONE',  ( 748.9653473494363425, -98.63460265842024910, -356.9462024416521331 ) ) ;
#26288=CARTESIAN_POINT ( 'NONE',  ( 758.8095938919642549, -344.0891481129647786, -311.6929314249763365 ) ) ;
#26294=CARTESIAN_POINT ( 'NONE',  ( 795.6651683502461765, -106.7146871989600498, -371.3240766477733814 ) ) ;
#26299=CARTESIAN_POINT ( 'NONE',  ( 804.1601925771018387, -223.4419599262323857, -346.5483106153029098 ) ) ;
#26302=CARTESIAN_POINT ( 'NONE',  ( 766.5853460496234675, -421.9874144716863498, -372.3518521366060554 ) ) ;
#26303=CARTESIAN_POINT ( 'NONE',  ( 744.9990715423526808, -66.35105083532378956, -341.2370466360926002 ) ) ;
#26308=CARTESIAN_POINT ( 'NONE',  ( 764.1737431748507561, -370.3726999360613377, -371.6461892240376415 ) ) ;
#26309=CARTESIAN_POINT ( 'NONE',  ( 774.6312213355099630, -239.3618753856924570, -364.6798772138717482 ) ) ;
#26313=CARTESIAN_POINT ( 'NONE',  ( 773.4516893846965786, -235.6454272087890729, -315.8398074228977066 ) ) ;
#26314=CARTESIAN_POINT ( 'NONE',  ( 755.3201227861273992, -195.7255117493289731, -345.3687786644892981 ) ) ;
#26315=CARTESIAN_POINT ( 'NONE',  ( 804.6798772138710092, -375.7255117493284047, -334.6312213355106451 ) ) ;
#26318=CARTESIAN_POINT ( 'NONE',  ( 804.4286716492782716, -113.3618753856929260, -345.3141322388244703 ) ) ;
#26319=ORIENTED_EDGE ( 'NONE', *, *, #42226, .F. ) ;
#26328=CARTESIAN_POINT ( 'NONE',  ( 763.8424801807145741, 5.990936427573807954, -320.5453621957614700 ) ) ;
#26329=CARTESIAN_POINT ( 'NONE',  ( 772.4837098697145166, -47.36187538569312494, -374.5518280994205611 ) ) ;
#26332=CARTESIAN_POINT ( 'NONE',  ( 756.3353852180819104, -413.9073299311465348, -331.1735550268788302 ) ) ;
#26333=CARTESIAN_POINT ( 'NONE',  ( 765.0180583372156207, -24.99823902205683268, -360.0135310231089534 ) ) ;
#26336=CARTESIAN_POINT ( 'NONE',  ( 800.9840315886518738, -268.9181544815162397, -354.1144889064786412 ) ) ;
#26337=CARTESIAN_POINT ( 'NONE',  ( 745.0891759886404770, -172.2709662947836478, -342.4968714119734159 ) ) ;
#26344=CARTESIAN_POINT ( 'NONE',  ( 755.5713283507202505, -317.3618753856922581, -334.6858677611754729 ) ) ;
#26346=CARTESIAN_POINT ( 'NONE',  ( 766.4474001241216001, -91.09997266333496668, -307.3154664389482491 ) ) ;
#26347=CARTESIAN_POINT ( 'NONE',  ( 757.2208543904082489, -112.7146871989600356, -350.9844846989624330 ) ) ;
#26351=CARTESIAN_POINT ( 'NONE',  ( 804.4286716492782716, -17.36187538569322086, -345.3141322388244703 ) ) ;
#26352=CARTESIAN_POINT ( 'NONE',  ( 757.2208543904082489, -136.7146871989600072, -350.9844846989624330 ) ) ;
#26353=CARTESIAN_POINT ( 'NONE',  ( 781.8018195045266339, -118.2709662947837899, -365.1927285166406705 ) ) ;
#26355=EDGE_CURVE ( 'NONE', #35219, #39264, #39623, .T. ) ;
#26356=CARTESIAN_POINT ( 'NONE',  ( 772.3691319403857278, -431.2601417444136018, -315.8894580844506663 ) ) ;
#26362=CARTESIAN_POINT ( 'NONE',  ( 762.1177392798416577, -258.5545181178799226, -309.8865473780659272 ) ) ;
#26371=CARTESIAN_POINT ( 'NONE',  ( 772.4468031744293057, -129.8272453906075725, -363.8651313633793620 ) ) ;
#26372=CARTESIAN_POINT ( 'NONE',  ( 771.1735550268780344, -297.1800572038741279, -316.3353852180828198 ) ) ;
#26374=CARTESIAN_POINT ( 'NONE',  ( 759.7806653035534055, -414.9982390220555430, -324.8639956371180801 ) ) ;
#26375=CARTESIAN_POINT ( 'NONE',  ( 803.4237431249931660, -87.18005720387481006, -331.2633955100225194 ) ) ;
#26379=CARTESIAN_POINT ( 'NONE',  ( 814.8207195650702488, -2.190881754244347945, -336.2433038121456548 ) ) ;
#26381=ORIENTED_EDGE ( 'NONE', *, *, #36022, .F. ) ;
#26382=CARTESIAN_POINT ( 'NONE',  ( 745.1792804349281596, -302.1908817542433781, -343.7566961878542884 ) ) ;
#26386=CARTESIAN_POINT ( 'NONE',  ( 765.0180583372156207, -288.9982390220559978, -360.0135310231089534 ) ) ;
#26389=CARTESIAN_POINT ( 'NONE',  ( 758.4439275373578084, -156.5545181178802636, -353.2243759319684386 ) ) ;
#26392=CARTESIAN_POINT ( 'NONE',  ( 800.9747183278959710, -348.9982390220558273, -311.9810565676471583 ) ) ;
#26398=CARTESIAN_POINT ( 'NONE',  ( 787.5162901302840055, 12.63812461430668321, -305.4481719005792684 ) ) ;
#26403=CARTESIAN_POINT ( 'NONE',  ( 794.1144889064781864, -10.16923265350579442, -360.9840315886528401 ) ) ;
#26410=CARTESIAN_POINT ( 'NONE',  ( 803.8651313633788504, -317.2601417444139429, -332.4468031744301015 ) ) ;
#26413=CARTESIAN_POINT ( 'NONE',  ( 747.3154664389472828, -331.9874144716865203, -326.4474001241230781 ) ) ;
#26414=CARTESIAN_POINT ( 'NONE',  ( 759.9999999999992042, -462.9681489794448339, -370.0000000000000568 ) ) ;
#26421=CARTESIAN_POINT ( 'NONE',  ( 759.0252816721024374, -168.9982390220563673, -368.0189434323527280 ) ) ;
#26424=CARTESIAN_POINT ( 'NONE',  ( 788.7366044899766848, -179.9073299311472454, -316.5762568750059813 ) ) ;
#26427=CARTESIAN_POINT ( 'NONE',  ( 801.5560724626406000, -456.5545181178792404, -326.7756240680316182 ) ) ;
#26433=EDGE_LOOP ( 'NONE', ( #12570, #31079, #22990, #44661 ) ) ;
#26434=CARTESIAN_POINT ( 'NONE',  ( 763.0428371773158460, -443.4636090269702322, -358.7617431975195359 ) ) ;
#26437=CARTESIAN_POINT ( 'NONE',  ( 773.7305795820266212, -201.2817908451528126, -374.8230680027170365 ) ) ;
#26439=CARTESIAN_POINT ( 'NONE',  ( 779.9999999999992042, 126.4563064324884465, -350.0000000000000000 ) ) ;
#26440=CARTESIAN_POINT ( 'NONE',  ( 791.9812246680005501, -188.6346026584199365, -361.9419747391813189 ) ) ;
#26441=CARTESIAN_POINT ( 'NONE',  ( 773.3843516231979720, -349.4419599262320162, -364.4086373105754433 ) ) ;
#26442=DIRECTION ( 'NONE',  ( 0.000000000000000000, -1.000000000000000000, 0.000000000000000000 ) ) ;
#26443=CARTESIAN_POINT ( 'NONE',  ( 745.5313806188320314, -207.2817908451527842, -333.7943932421247268 ) ) ;
#26446=CARTESIAN_POINT ( 'NONE',  ( 758.4439275373578084, -36.55451811788061178, -353.2243759319684386 ) ) ;
#26448=CARTESIAN_POINT ( 'NONE',  ( 800.9747183278959710, -228.9982390220561683, -311.9810565676471583 ) ) ;
#26452=CARTESIAN_POINT ( 'NONE',  ( 755.5713283507202505, -53.36187538569310362, -334.6858677611754729 ) ) ;
#26454=CARTESIAN_POINT ( 'NONE',  ( 746.0683387631852383, -139.4419599262326699, -331.3260364891676204 ) ) ;
#26456=CARTESIAN_POINT ( 'NONE',  ( 808.0189434323515343, -374.0891481129647786, -319.0252816721025511 ) ) ;
#26460=CARTESIAN_POINT ( 'NONE',  ( 774.6858677611749044, -393.7255117493283478, -315.5713283507209894 ) ) ;
#26463=CARTESIAN_POINT ( 'NONE',  ( 800.9747183278959710, -444.9982390220554862, -311.9810565676471583 ) ) ;
#26468=CARTESIAN_POINT ( 'NONE',  ( 805.0264073115434940, -222.3510508353233206, -339.4763451958999099 ) ) ;
#26470=CARTESIAN_POINT ( 'NONE',  ( 744.9990715423526808, -234.3510508353232638, -341.2370466360926002 ) ) ;
#26476=CARTESIAN_POINT ( 'NONE',  ( 787.4397851343537695, -69.72551174932942786, -374.2001403089903988 ) ) ;
#26477=CARTESIAN_POINT ( 'NONE',  ( 762.3223304703356007, -79.54369356751119824, -322.3223304703362828 ) ) ;
#26479=CARTESIAN_POINT ( 'NONE',  ( 787.5531968255692163, -21.82724539060792424, -316.1348686366205811 ) ) ;
#26481=CARTESIAN_POINT ( 'NONE',  ( 793.9708237608222134, -334.9181544815160692, -319.2295555964448681 ) ) ;
#26489=CARTESIAN_POINT ( 'NONE',  ( 790.0220218866281812, -319.0999726633342561, -363.2186876482849129 ) ) ;
#26490=CARTESIAN_POINT ( 'NONE',  ( 797.8594530101008786, -325.5436935675105019, -322.1405469898980982 ) ) ;
#26491=CARTESIAN_POINT ( 'NONE',  ( 794.9819416627830151, -156.9982390220564241, -319.9864689768909898 ) ) ;
#26495=CARTESIAN_POINT ( 'NONE',  ( 758.6633372737375112, -260.5328690171413086, -326.9102291470432533 ) ) ;
#26496=CARTESIAN_POINT ( 'NONE',  ( 754.3581564841646241, -113.4636090269712554, -316.1443688327762516 ) ) ;
#26501=CARTESIAN_POINT ( 'NONE',  ( 745.7998596910086917, -149.3618753856928265, -332.5602148656461168 ) ) ;
#26504=CARTESIAN_POINT ( 'NONE',  ( 777.5031285880264704, -262.8164208402379245, -374.9108240113588408 ) ) ;
#26508=CARTESIAN_POINT ( 'NONE',  ( 748.3538107759620743, -352.7146871989593251, -355.8262568251490165 ) ) ;
#26509=CARTESIAN_POINT ( 'NONE',  ( 745.0891759886404770, -76.27096629478394618, -342.4968714119734159 ) ) ;
#26511=CARTESIAN_POINT ( 'NONE',  ( 800.9747183278959710, -348.9982390220558273, -311.9810565676471583 ) ) ;
#26515=CARTESIAN_POINT ( 'NONE',  ( 767.8955696845333705, -216.4527844766016926, -362.1676090361162323 ) ) ;
#26517=CARTESIAN_POINT ( 'NONE',  ( 761.9338519418445230, -134.5328690171417350, -370.4231160770881957 ) ) ;
#26523=CARTESIAN_POINT ( 'NONE',  ( 787.6308680596127942, -11.26014174441488258, -364.1105419155492768 ) ) ;
#26525=CARTESIAN_POINT ( 'NONE',  ( 749.8865473780648472, -428.5328690171409107, -322.1177392798429082 ) ) ;
#26529=CARTESIAN_POINT ( 'NONE',  ( 754.3581564841646241, -377.4636090269704596, -316.1443688327762516 ) ) ;
#26530=CARTESIAN_POINT ( 'NONE',  ( 765.0180583372156207, -240.9982390220561683, -360.0135310231089534 ) ) ;
#26533=CARTESIAN_POINT ( 'NONE',  ( 769.9779781133707957, -211.0999726633346540, -316.7813123517150871 ) ) ;
#26534=CARTESIAN_POINT ( 'NONE',  ( 801.9419747391806368, -210.4527844766016926, -351.9812246680014027 ) ) ;
#26535=CARTESIAN_POINT ( 'NONE',  ( 762.3223304703356007, -391.5436935675101608, -322.3223304703362828 ) ) ;
#26536=ORIENTED_EDGE ( 'NONE', *, *, #17279, .F. ) ;
#26538=CARTESIAN_POINT ( 'NONE',  ( 801.9419747391806368, -114.4527844766020053, -351.9812246680014027 ) ) ;
#26547=CARTESIAN_POINT ( 'NONE',  ( 745.7194118038753459, -445.6454272087883055, -348.7631598425976449 ) ) ;
#26548=CARTESIAN_POINT ( 'NONE',  ( 787.5162901302840055, -35.36187538569316047, -305.4481719005793252 ) ) ;
#26550=CARTESIAN_POINT ( 'NONE',  ( 785.3141322388236176, -381.7255117493284615, -364.4286716492789537 ) ) ;
#26551=CARTESIAN_POINT ( 'NONE',  ( 797.8594530101009923, -13.54369356751140963, -322.1405469898982119 ) ) ;
#26554=CARTESIAN_POINT ( 'NONE',  ( 761.4292242960306112, -281.4636090269706870, -323.2154366446414429 ) ) ;
#26555=CARTESIAN_POINT ( 'NONE',  ( 758.8095938919642549, -152.0891481129655460, -311.6929314249763365 ) ) ;
#26562=CARTESIAN_POINT ( 'NONE',  ( 754.8072714833581358, -364.8164208402374697, -338.1981804954720587 ) ) ;
#26564=CARTESIAN_POINT ( 'NONE',  ( 788.6739635108323228, -103.6454272087894850, -373.9316612368139090 ) ) ;
#26565=CARTESIAN_POINT ( 'NONE',  ( 759.2295555964440155, -112.1692326535054889, -353.9708237608231229 ) ) ;
#26568=CARTESIAN_POINT ( 'NONE',  ( 762.1405469898971887, -25.54369356751136877, -357.8594530101015607 ) ) ;
#26569=CARTESIAN_POINT ( 'NONE',  ( 766.7756240680305382, -182.5328690171416497, -361.5560724626415663 ) ) ;
#26570=CARTESIAN_POINT ( 'NONE',  ( 801.9419747391806368, -138.4527844766019200, -351.9812246680014027 ) ) ;
#26572=CARTESIAN_POINT ( 'NONE',  ( 799.4546378042377910, -417.0783235625954148, -356.1575198192848006 ) ) ;
#26578=CARTESIAN_POINT ( 'NONE',  ( 797.8822607201568644, -270.5545181178798657, -370.1134526219340160 ) ) ;
#26585=CARTESIAN_POINT ( 'NONE',  ( 790.0220218866281812, -127.0999726633348672, -363.2186876482849129 ) ) ;
#26586=CARTESIAN_POINT ( 'NONE',  ( 765.0180583372156207, -96.99823902205660886, -360.0135310231089534 ) ) ;
#26587=CARTESIAN_POINT ( 'NONE',  ( 778.1981804954715471, -298.2709662947831930, -314.8072714833591021 ) ) ;
#26589=CARTESIAN_POINT ( 'NONE',  ( 785.3141322388236176, -429.7255117493282910, -364.4286716492789537 ) ) ;
#26590=CARTESIAN_POINT ( 'NONE',  ( 781.8018195045266339, -70.27096629478397460, -365.1927285166406705 ) ) ;
#26596=CARTESIAN_POINT ( 'NONE',  ( 750.9282345327678740, -352.9181544815159555, -319.8311093483690115 ) ) ;
#26599=CARTESIAN_POINT ( 'NONE',  ( 781.8018195045266339, -286.2709662947833635, -365.1927285166406705 ) ) ;
#26601=CARTESIAN_POINT ( 'NONE',  ( 775.8780910478218402, -201.2817908451528126, -364.9511171171680530 ) ) ;
#26605=CARTESIAN_POINT ( 'NONE',  ( 745.4481719005789273, -387.7255117493284047, -347.5162901302853697 ) ) ;
#26610=CARTESIAN_POINT ( 'NONE',  ( 800.9747183278959710, -12.99823902205686821, -311.9810565676471583 ) ) ;
#26612=CARTESIAN_POINT ( 'NONE',  ( 778.2165204200184689, -238.8164208402379813, -364.9363028652563230 ) ) ;
#26613=CARTESIAN_POINT ( 'NONE',  ( 799.9999999999993179, 205.0000000000000568, -319.9999999999999432 ) ) ;
#26617=CARTESIAN_POINT ( 'NONE',  ( 773.3843516231979720, -13.44195992623305713, -364.4086373105754433 ) ) ;
#26622=EDGE_LOOP ( 'NONE', ( #19619, #34109, #29503, #40045 ) ) ;
#26623=CARTESIAN_POINT ( 'NONE',  ( 769.1273215169530886, -334.7146871989593251, -317.4527132478988847 ) ) ;
#26626=CARTESIAN_POINT ( 'NONE',  ( 746.7653713866222915, -377.2601417444137724, -351.0478386215610271 ) ) ;
#26634=CARTESIAN_POINT ( 'NONE',  ( 748.9653473494363425, -194.6346026584198796, -356.9462024416521331 ) ) ;
#26638=CARTESIAN_POINT ( 'NONE',  ( 803.6646147819162707, -161.9073299311472738, -348.8264449731211130 ) ) ;
#26640=CARTESIAN_POINT ( 'NONE',  ( 760.7433823573367135, -444.0090635724249069, -355.9930595647440441 ) ) ;
#26646=CARTESIAN_POINT ( 'NONE',  ( 760.7433823573367135, -420.0090635724249069, -355.9930595647440441 ) ) ;
#26648=CARTESIAN_POINT ( 'NONE',  ( 768.9521613784389729, -249.8272453906072315, -373.2346286133773106 ) ) ;
#26652=CARTESIAN_POINT ( 'NONE',  ( 801.9419747391806368, -186.4527844766017779, -351.9812246680014027 ) ) ;
#26654=CARTESIAN_POINT ( 'NONE',  ( 784.0799538623451781, -347.8055962898683333, -364.6971507214555572 ) ) ;
#26656=CARTESIAN_POINT ( 'NONE',  ( 795.8262568251477660, -238.3726999360617640, -308.3538107759623585 ) ) ;
#26659=CARTESIAN_POINT ( 'NONE',  ( 786.5483106153019435, -31.64542720878970883, -364.1601925771022366 ) ) ;
#26663=CARTESIAN_POINT ( 'NONE',  ( 755.0488828828309806, -425.8055962898680491, -344.1219089521771934 ) ) ;
#26664=CARTESIAN_POINT ( 'NONE',  ( 801.1904061080338124, -284.0891481129651197, -368.3070685750236066 ) ) ;
#26668=CARTESIAN_POINT ( 'NONE',  ( 800.0135310231082713, -62.08914811296580183, -325.0180583372163028 ) ) ;
#26670=CARTESIAN_POINT ( 'NONE',  ( 788.7631598425961101, -121.4419599262327267, -305.7194118038759143 ) ) ;
#26672=CARTESIAN_POINT ( 'NONE',  ( 772.5602148656447525, -393.7255117493283478, -305.7998596910095443 ) ) ;
#26678=CARTESIAN_POINT ( 'NONE',  ( 804.6798772138708955, -399.7255117493283478, -334.6312213355107019 ) ) ;
#26680=CARTESIAN_POINT ( 'NONE',  ( 748.6759233522253680, -40.37269993606240348, -324.3348316497537098 ) ) ;
#26681=LINE ( 'NONE', #19763, #26199 ) ;
#26684=CARTESIAN_POINT ( 'NONE',  ( 804.1601925771018387, -223.4419599262323857, -346.5483106153029098 ) ) ;
#26685=CARTESIAN_POINT ( 'NONE',  ( 774.6858677611749044, -129.7255117493292289, -315.5713283507209894 ) ) ;
#26688=CARTESIAN_POINT ( 'NONE',  ( 744.9990715423526808, -210.3510508353233490, -341.2370466360926002 ) ) ;
#26693=CARTESIAN_POINT ( 'NONE',  ( 771.2633955100217236, -167.9073299311473022, -363.4237431249939618 ) ) ;
#26695=CARTESIAN_POINT ( 'NONE',  ( 787.5162901302840055, -83.36187538569296862, -305.4481719005792684 ) ) ;
#26696=CARTESIAN_POINT ( 'NONE',  ( 764.8639956371174549, -80.08914811296574499, -319.7806653035542581 ) ) ;
#26698=CARTESIAN_POINT ( 'NONE',  ( 775.8780910478218402, -9.281790845153418346, -364.9511171171680530 ) ) ;
#26700=CARTESIAN_POINT ( 'NONE',  ( 796.1575198192839480, -366.0090635724250774, -359.4546378042384163 ) ) ;
#26706=CARTESIAN_POINT ( 'NONE',  ( 804.6971507214547046, -315.2817908451525000, -344.0799538623459739 ) ) ;
#26707=CARTESIAN_POINT ( 'NONE',  ( 794.9819416627830151, -324.9982390220559409, -319.9864689768909898 ) ) ;
#26708=CARTESIAN_POINT ( 'NONE',  ( 812.3518521366052028, -145.0999726633347677, -326.5853460496235243 ) ) ;
#26713=CARTESIAN_POINT ( 'NONE',  ( 756.1348686366196716, -257.2601417444141134, -347.5531968255698416 ) ) ;
#26714=CARTESIAN_POINT ( 'NONE',  ( 747.6481478633932056, -133.0999726633348246, -353.4146539503763620 ) ) ;
#26722=CARTESIAN_POINT ( 'NONE',  ( 758.8095938919644823, -152.0891481129655460, -311.6929314249762797 ) ) ;
#26724=CARTESIAN_POINT ( 'NONE',  ( 792.3570229623688874, -261.1800572038741848, -373.1304606946836202 ) ) ;
#26725=CARTESIAN_POINT ( 'NONE',  ( 777.4774526936600978, -442.2709662947827383, -304.7301800767028226 ) ) ;
#26728=CARTESIAN_POINT ( 'NONE',  ( 752.4576283171824116, -357.0783235625956422, -317.7880784355627952 ) ) ;
#26729=CARTESIAN_POINT ( 'NONE',  ( 777.5031285880264704, -94.81642084023843609, -374.9108240113588408 ) ) ;
#26731=CARTESIAN_POINT ( 'NONE',  ( 751.6929314249748586, -342.9982390220557136, -318.8095938919659034 ) ) ;
#26736=CARTESIAN_POINT ( 'NONE',  ( 748.3538107759620743, -112.7146871989600356, -355.8262568251490165 ) ) ;
#26741=CARTESIAN_POINT ( 'NONE',  ( 790.8726784830453198, -10.71468719896033761, -362.5472867521010585 ) ) ;
#26743=CARTESIAN_POINT ( 'NONE',  ( 808.7758568127978833, -436.1692326535044231, -320.0363995740631822 ) ) ;
#26744=AXIS2_PLACEMENT_3D ( 'NONE', #14181, #31721, #42348 ) ;
#26748=CARTESIAN_POINT ( 'NONE',  ( 791.0478386215596629, -381.8272453906068336, -306.7653713866226326 ) ) ;
#26752=CARTESIAN_POINT ( 'NONE',  ( 754.7162404726377645, -206.7363362996982801, -339.4709603349214717 ) ) ;
#26753=CARTESIAN_POINT ( 'NONE',  ( 805.1927285166397041, -232.8164208402379245, -341.8018195045277707 ) ) ;
#26754=CARTESIAN_POINT ( 'NONE',  ( 801.9419747391806368, -426.4527844766010389, -351.9812246680014027 ) ) ;
#26757=CARTESIAN_POINT ( 'NONE',  ( 754.8072714833581358, -100.8164208402383792, -338.1981804954720587 ) ) ;
#26765=CARTESIAN_POINT ( 'NONE',  ( 812.3518521366052028, -457.0999726633339151, -326.5853460496235243 ) ) ;
#26766=VECTOR ( 'NONE', #23182, 1000.000000000000000 ) ;
#26767=CARTESIAN_POINT ( 'NONE',  ( 801.1904061080338124, -44.08914811296585157, -368.3070685750236066 ) ) ;
#26769=CARTESIAN_POINT ( 'NONE',  ( 791.9812246680005501, -404.6346026584193396, -361.9419747391813189 ) ) ;
#26770=CARTESIAN_POINT ( 'NONE',  ( 788.8264449731201466, -21.18005720387502322, -363.6646147819170665 ) ) ;
#26773=CARTESIAN_POINT ( 'NONE',  ( 757.4527132478984868, -280.3726999360616787, -329.1273215169538844 ) ) ;
#26774=CARTESIAN_POINT ( 'NONE',  ( 744.7301800767019131, -172.8164208402381234, -337.4774526936615757 ) ) ;
#26777=CARTESIAN_POINT ( 'NONE',  ( 764.4978033197144214, 16.45630643248849267, -320.3127214678681867 ) ) ;
#26779=CARTESIAN_POINT ( 'NONE',  ( 758.0141637701419768, -231.0783235625960401, -367.2620300519063790 ) ) ;
#26784=CARTESIAN_POINT ( 'NONE',  ( 791.9812246680005501, -356.6346026584193964, -361.9419747391813189 ) ) ;
#26786=CARTESIAN_POINT ( 'NONE',  ( 786.2694204179717872, -93.28179084515315367, -305.1769319972829067 ) ) ;
#26787=CARTESIAN_POINT ( 'NONE',  ( 756.7813123517142913, -163.9874144716871456, -329.9779781133712504 ) ) ;
#26790=CARTESIAN_POINT ( 'NONE',  ( 803.6646147819161570, -65.90732993114758642, -348.8264449731210561 ) ) ;
#26791=CARTESIAN_POINT ( 'NONE',  ( 793.2243759319678702, -170.5328690171416781, -318.4439275373583200 ) ) ;
#26792=CARTESIAN_POINT ( 'NONE',  ( 788.8264449731200330, -117.1800572038746964, -363.6646147819171233 ) ) ;
#26794=CARTESIAN_POINT ( 'NONE',  ( 752.4576283171824116, 2.921676437403253779, -317.7880784355627952 ) ) ;
#26798=ORIENTED_EDGE ( 'NONE', *, *, #43362, .F. ) ;
#26801=CARTESIAN_POINT ( 'NONE',  ( 754.3581564841646241, -257.4636090269708575, -316.1443688327762516 ) ) ;
#26807=CARTESIAN_POINT ( 'NONE',  ( 786.5483106153019435, -127.6454272087894140, -364.1601925771022366 ) ) ;
#26808=CARTESIAN_POINT ( 'NONE',  ( 804.6798772138708955, -111.7255117493293000, -334.6312213355107019 ) ) ;
#26809=CARTESIAN_POINT ( 'NONE',  ( 764.8639956371174549, -320.0891481129648923, -319.7806653035542581 ) ) ;
#26811=CARTESIAN_POINT ( 'NONE',  ( 764.8639956371174549, -416.0891481129645513, -319.7806653035542013 ) ) ;
#26812=CARTESIAN_POINT ( 'NONE',  ( 778.1981804954714335, -82.27096629478388934, -314.8072714833589885 ) ) ;
#26819=CARTESIAN_POINT ( 'NONE',  ( 745.5313806188320314, -351.2817908451523294, -333.7943932421247268 ) ) ;
#26821=CARTESIAN_POINT ( 'NONE',  ( 764.8639956371174549, -296.0891481129650629, -319.7806653035542013 ) ) ;
#26823=CARTESIAN_POINT ( 'NONE',  ( 763.0428371773158460, -179.4636090269710849, -358.7617431975195359 ) ) ;
#26826=CARTESIAN_POINT ( 'NONE',  ( 813.1304606946831655, -377.9073299311465917, -352.3570229623691716 ) ) ;
#26832=CARTESIAN_POINT ( 'NONE',  ( 767.6429770376289525, -33.18005720387498769, -306.8695393053162093 ) ) ;
#26833=CARTESIAN_POINT ( 'NONE',  ( 781.7834795799800531, -250.8164208402379245, -315.0636971347436202 ) ) ;
#26837=CARTESIAN_POINT ( 'NONE',  ( 796.7845633553578182, -33.62377810805116951, -358.5707757039688204 ) ) ;
#26845=VECTOR ( 'NONE', #45155, 1000.000000000000000 ) ;
#26846=CARTESIAN_POINT ( 'NONE',  ( 795.9930595647434757, -339.0783235625956422, -320.7433823573372820 ) ) ;
#26849=CARTESIAN_POINT ( 'NONE',  ( 795.6651683502461765, -370.7146871989592114, -371.3240766477733814 ) ) ;
#26854=CARTESIAN_POINT ( 'NONE',  ( 748.9653473494363425, -218.6346026584197944, -356.9462024416521331 ) ) ;
#26858=AXIS2_PLACEMENT_3D ( 'NONE', #23153, #34241, #6075 ) ;
#26859=CARTESIAN_POINT ( 'NONE',  ( 756.5762568750052424, -171.1800572038745543, -348.7366044899774238 ) ) ;
#26862=CARTESIAN_POINT ( 'NONE',  ( 762.1405469898971887, -337.5436935675102177, -357.8594530101015607 ) ) ;
#26863=CARTESIAN_POINT ( 'NONE',  ( 792.1044303154645831, 11.54721552339760038, -317.8323909638837677 ) ) ;
#26871=CARTESIAN_POINT ( 'NONE',  ( 760.7433823573367135, -444.0090635724249069, -355.9930595647440441 ) ) ;
#26875=CARTESIAN_POINT ( 'NONE',  ( 802.2119215644370342, -222.0090635724254184, -367.5423716828165084 ) ) ;
#26880=CARTESIAN_POINT ( 'NONE',  ( 788.8264449731200330, -189.1800572038744122, -363.6646147819171233 ) ) ;
#26881=CARTESIAN_POINT ( 'NONE',  ( 787.6308680596127942, -371.2601417444136587, -364.1105419155492768 ) ) ;
#26883=CARTESIAN_POINT ( 'NONE',  ( 814.8207195650702488, -218.1908817542437191, -336.2433038121456548 ) ) ;
#26885=LINE ( 'NONE', #9352, #9102 ) ;
#26886=CARTESIAN_POINT ( 'NONE',  ( 790.9844846989617508, -70.37269993606230400, -317.2208543904092721 ) ) ;
#26890=CARTESIAN_POINT ( 'NONE',  ( 804.9511171171677688, -437.8055962898679923, -335.8780910478229202 ) ) ;
#26891=CARTESIAN_POINT ( 'NONE',  ( 777.5031285880264704, -262.8164208402379245, -374.9108240113588408 ) ) ;
#26893=DIRECTION ( 'NONE',  ( 0.000000000000000000, 0.000000000000000000, -1.000000000000000000 ) ) ;
#26894=CARTESIAN_POINT ( 'NONE',  ( 788.7366044899766848, -59.90732993114762905, -316.5762568750059813 ) ) ;
#26896=CARTESIAN_POINT ( 'NONE',  ( 800.1688906516307043, -178.1692326535052473, -369.0717654672308186 ) ) ;
#26898=CARTESIAN_POINT ( 'NONE',  ( 801.1904061080336987, -404.0891481129646081, -368.3070685750235498 ) ) ;
#26899=CARTESIAN_POINT ( 'NONE',  ( 791.7608162188021197, 178.9475563372491251, -320.0000000000000000 ) ) ;
#26903=CARTESIAN_POINT ( 'NONE',  ( 765.0180583372156207, -408.9982390220556567, -360.0135310231089534 ) ) ;
#26904=VECTOR ( 'NONE', #35831, 1000.000000000000000 ) ;
#26906=DIRECTION ( 'NONE',  ( -1.000000000000000000, 0.000000000000000000, 0.000000000000000000 ) ) ;
#26909=CARTESIAN_POINT ( 'NONE',  ( 805.1016975059191054, -222.8965053807778531, -343.0745993439771837 ) ) ;
#26912=CARTESIAN_POINT ( 'NONE',  ( 749.8865473780648472, -260.5328690171413086, -322.1177392798429082 ) ) ;
#26919=CARTESIAN_POINT ( 'NONE',  ( 765.0180583372156207, -168.9982390220563673, -360.0135310231089534 ) ) ;
#26923=CARTESIAN_POINT ( 'NONE',  ( 815.2698199232961542, -112.8164208402383508, -342.5225473063383106 ) ) ;
#26925=CARTESIAN_POINT ( 'NONE',  ( 768.0187753319979720, -56.63460265842036279, -318.0580252608186242 ) ) ;
#26927=CARTESIAN_POINT ( 'NONE',  ( 784.1219089521767955, -45.28179084515329578, -315.0488828828318333 ) ) ;
#26928=CARTESIAN_POINT ( 'NONE',  ( 772.4468031744293057, -369.8272453906068904, -363.8651313633793620 ) ) ;
#26938=CARTESIAN_POINT ( 'NONE',  ( 793.0897708529556667, -318.5545181178796952, -361.3366627262616362 ) ) ;
#26939=CARTESIAN_POINT ( 'NONE',  ( 757.8323909638827445, -314.6346026584194533, -352.1044303154654358 ) ) ;
#26940=CARTESIAN_POINT ( 'NONE',  ( 805.6418435158337843, -149.4636090269711417, -363.8556311672236916 ) ) ;
#26946=CARTESIAN_POINT ( 'NONE',  ( 801.3366627262608972, -272.5328690171413086, -353.0897708529566899 ) ) ;
#26947=CARTESIAN_POINT ( 'NONE',  ( 766.4474001241216001, -115.0999726633348956, -307.3154664389482491 ) ) ;
#26949=CARTESIAN_POINT ( 'NONE',  ( 799.9999999999993179, -462.9681489794448339, -309.9999999999998863 ) ) ;
#26955=CARTESIAN_POINT ( 'NONE',  ( 796.7737145352015204, -164.6346026584200217, -370.7187646348536987 ) ) ;
#26956=EDGE_CURVE ( 'NONE', #41099, #11148, #35936, .T. ) ;
#26957=CARTESIAN_POINT ( 'NONE',  ( 759.0860845406687076, 19.76315572498245743, -318.4906424660488256 ) ) ;
#26960=CARTESIAN_POINT ( 'NONE',  ( 758.8095938919642549, -296.0891481129650629, -311.6929314249763365 ) ) ;
#26963=PRODUCT ( 'Treadle Extension Return Springs', 'Treadle Extension Return Springs', '', ( #28597 ) ) ;
#26967=CARTESIAN_POINT ( 'NONE',  ( 778.7502325331095108, -336.3510508353228943, -304.6391490659818828 ) ) ;
#26968=CARTESIAN_POINT ( 'NONE',  ( 796.7737145352015204, -116.6346026584201780, -370.7187646348536987 ) ) ;
#26970=CARTESIAN_POINT ( 'NONE',  ( 811.0346526505616112, -374.6346026584192828, -323.0537975583477532 ) ) ;
#26976=CARTESIAN_POINT ( 'NONE',  ( 773.7943932421234194, -167.8055962898689586, -305.5313806188329409 ) ) ;
#26982=EDGE_CURVE ( 'NONE', #17925, #12399, #35210, .T. ) ;
#26983=CARTESIAN_POINT ( 'NONE',  ( 760.5453621957607311, 2.921676437403253779, -323.8424801807151425 ) ) ;
#26986=CARTESIAN_POINT ( 'NONE',  ( 815.1787889125755555, -438.8965053807771710, -343.7953271457877804 ) ) ;
#26990=CARTESIAN_POINT ( 'NONE',  ( 813.5763878283155464, -363.8272453906068336, -351.1614460488615350 ) ) ;
#26997=CARTESIAN_POINT ( 'NONE',  ( 775.8780910478218402, -225.2817908451527273, -364.9511171171680530 ) ) ;
#26998=CARTESIAN_POINT ( 'NONE',  ( 778.1981804954714335, -226.2709662947834204, -314.8072714833589885 ) ) ;
#26999=CARTESIAN_POINT ( 'NONE',  ( 756.5762568750052424, -411.1800572038738437, -348.7366044899774238 ) ) ;
#27002=CARTESIAN_POINT ( 'NONE',  ( 774.6312213355099630, -95.36187538569294020, -364.6798772138717482 ) ) ;
#27010=ORIENTED_EDGE ( 'NONE', *, *, #43384, .F. ) ;
#27011=CARTESIAN_POINT ( 'NONE',  ( 815.3608509340175488, -458.7363362996973706, -341.2497674668889545 ) ) ;
#27012=CARTESIAN_POINT ( 'NONE',  ( 751.9810565676468741, -74.08914811296577341, -360.9747183278973921 ) ) ;
#27015=CARTESIAN_POINT ( 'NONE',  ( 757.8323909638827445, -434.6346026584190554, -352.1044303154654358 ) ) ;
#27016=CARTESIAN_POINT ( 'NONE',  ( 759.7806653035535192, -30.99823902205680781, -324.8639956371181370 ) ) ;
#27018=CARTESIAN_POINT ( 'NONE',  ( 804.9363028652555840, 7.729033705215793582, -338.2165204200192079 ) ) ;
#27019=CARTESIAN_POINT ( 'NONE',  ( 786.5483106153019435, -295.6454272087888739, -364.1601925771022366 ) ) ;
#27020=CARTESIAN_POINT ( 'NONE',  ( 804.7487373415286811, -187.5436935675108430, -364.7487373415288516 ) ) ;
#27026=CARTESIAN_POINT ( 'NONE',  ( 752.4576283171824116, -237.0783235625960117, -317.7880784355627952 ) ) ;
#27028=CARTESIAN_POINT ( 'NONE',  ( 767.6429770376289525, -297.1800572038740711, -306.8695393053162093 ) ) ;
#27032=CARTESIAN_POINT ( 'NONE',  ( 767.8955696845333705, -336.4527844766012095, -362.1676090361162323 ) ) ;
#27033=AXIS2_PLACEMENT_3D ( 'NONE', #2979, #10359, #39016 ) ;
#27035=CARTESIAN_POINT ( 'NONE',  ( 810.4231160770870019, -96.55451811788039151, -321.9338519418446936 ) ) ;
#27036=CARTESIAN_POINT ( 'NONE',  ( 765.8855110935204493, -166.1692326535053041, -319.0159684113471599 ) ) ;
#27041=CARTESIAN_POINT ( 'NONE',  ( 767.8955696845333705, -48.45278447660219712, -362.1676090361162323 ) ) ;
#27042=CARTESIAN_POINT ( 'NONE',  ( 805.0264073115434940, -150.3510508353235480, -339.4763451958999099 ) ) ;
#27044=CARTESIAN_POINT ( 'NONE',  ( 776.2433038121456548, -12.89650538077851216, -374.8207195650711014 ) ) ;
#27048=EDGE_LOOP ( 'NONE', ( #42471, #17566, #27692, #15307 ) ) ;
#27050=CARTESIAN_POINT ( 'NONE',  ( 776.2046728542105711, -284.1908817542434917, -304.8212110874238761 ) ) ;
#27060=CARTESIAN_POINT ( 'NONE',  ( 796.9571628226829034, -119.4636090269712554, -321.2382568024804641 ) ) ;
#27062=CARTESIAN_POINT ( 'NONE',  ( 762.1405469898971887, -97.54369356751112718, -357.8594530101015607 ) ) ;
#27063=CARTESIAN_POINT ( 'NONE',  ( 800.2193346964446619, -330.9982390220558273, -355.1360043628816925 ) ) ;
#27065=CARTESIAN_POINT ( 'NONE',  ( 759.9864689768902508, -434.0891481129646081, -354.9819416627836404 ) ) ;
#27074=CARTESIAN_POINT ( 'NONE',  ( 814.2805881961230625, -337.6454272087888171, -331.2368401574024119 ) ) ;
#27075=CARTESIAN_POINT ( 'NONE',  ( 774.6312213355099630, -335.3618753856920307, -364.6798772138717482 ) ) ;
#27077=CARTESIAN_POINT ( 'NONE',  ( 757.4527132478984868, -184.3726999360619629, -329.1273215169538844 ) ) ;
#27080=CARTESIAN_POINT ( 'NONE',  ( 787.4397851343537695, -381.7255117493284615, -374.2001403089903988 ) ) ;
#27085=CARTESIAN_POINT ( 'NONE',  ( 745.7998596910086917, -5.361875385693257279, -332.5602148656461168 ) ) ;
#27087=CARTESIAN_POINT ( 'NONE',  ( 805.1927285166397041, -256.8164208402379245, -341.8018195045277707 ) ) ;
#27091=CARTESIAN_POINT ( 'NONE',  ( 799.4546378042377910, -33.07832356259662987, -356.1575198192848006 ) ) ;
#27100=CARTESIAN_POINT ( 'NONE',  ( 804.6798772138708955, -63.72551174932939233, -334.6312213355107019 ) ) ;
#27101=CARTESIAN_POINT ( 'NONE',  ( 776.9566956441375396, -348.8965053807774552, -364.8461984189686405 ) ) ;
#27104=CARTESIAN_POINT ( 'NONE',  ( 791.1614460488616487, -371.2601417444136587, -373.5763878283158874 ) ) ;
#27110=CARTESIAN_POINT ( 'NONE',  ( 796.9462024416508257, -204.4527844766016926, -308.9653473494370246 ) ) ;
#27113=CARTESIAN_POINT ( 'NONE',  ( 755.5713283507202505, -221.3618753856925707, -334.6858677611754729 ) ) ;
#27115=CARTESIAN_POINT ( 'NONE',  ( 762.3223304703356007, -319.5436935675104451, -322.3223304703362828 ) ) ;
#27116=CARTESIAN_POINT ( 'NONE',  ( 755.1538015810308480, -446.1908817542429802, -343.0433043558613804 ) ) ;
#27123=CARTESIAN_POINT ( 'NONE',  ( 804.4086373105744769, -457.6454272087884760, -333.3843516231986541 ) ) ;
#27127=CARTESIAN_POINT ( 'NONE',  ( 744.6391490659812007, -230.7363362996981664, -338.7502325331110455 ) ) ;
#27131=CARTESIAN_POINT ( 'NONE',  ( 759.7806653035534055, -198.9982390220562252, -324.8639956371180801 ) ) ;
#27132=CARTESIAN_POINT ( 'NONE',  ( 763.2154366446407039, -357.6237781080501463, -321.4292242960311228 ) ) ;
#27133=CARTESIAN_POINT ( 'NONE',  ( 802.2119215644370342, -246.0090635724253900, -367.5423716828165084 ) ) ;
#27136=CARTESIAN_POINT ( 'NONE',  ( 766.9102291470427417, -66.55451811788050520, -318.6633372737382501 ) ) ;
#27139=FACE_BOUND ( 'NONE', #22947, .T. ) ;
#27140=CARTESIAN_POINT ( 'NONE',  ( 803.2186876482843445, -439.9874144716862929, -350.0220218866286928 ) ) ;
#27141=CARTESIAN_POINT ( 'NONE',  ( 812.7932403749906598, -279.1800572038741848, -327.7687537140311633 ) ) ;
#27144=CARTESIAN_POINT ( 'NONE',  ( 774.6858677611749044, -33.72551174932952733, -315.5713283507209894 ) ) ;
#27146=CARTESIAN_POINT ( 'NONE',  ( 781.2497674668890113, -156.3510508353235480, -375.3608509340180603 ) ) ;
#27148=CARTESIAN_POINT ( 'NONE',  ( 815.2698199232961542, -424.8164208402372992, -342.5225473063383106 ) ) ;
#27149=FACE_OUTER_BOUND ( 'NONE', #19997, .T. ) ;
#27152=CARTESIAN_POINT ( 'NONE',  ( 781.8018195045266339, -430.2709662947827383, -365.1927285166406705 ) ) ;
#27159=CARTESIAN_POINT ( 'NONE',  ( 755.0488828828309806, -257.8055962898686744, -344.1219089521771934 ) ) ;
#27161=CARTESIAN_POINT ( 'NONE',  ( 776.2433038121456548, -252.8965053807777394, -374.8207195650711014 ) ) ;
#27167=CARTESIAN_POINT ( 'NONE',  ( 769.1273215169530886, -22.71468719896029853, -317.4527132478988847 ) ) ;
#27168=CARTESIAN_POINT ( 'NONE',  ( 804.6798772138708955, -183.7255117493290015, -334.6312213355107019 ) ) ;
#27170=CARTESIAN_POINT ( 'NONE',  ( 808.0189434323515343, -110.0891481129656597, -319.0252816721025511 ) ) ;
#27171=CARTESIAN_POINT ( 'NONE',  ( 803.4237431249931660, -111.1800572038747532, -331.2633955100225194 ) ) ;
#27172=VERTEX_POINT ( 'NONE', #33825 ) ;
#27173=CARTESIAN_POINT ( 'NONE',  ( 783.0745993439762742, -32.19088175424425913, -365.1016975059196739 ) ) ;
#27174=CARTESIAN_POINT ( 'NONE',  ( 755.8894580844503253, -351.8272453906068336, -332.3691319403863531 ) ) ;
#27182=CARTESIAN_POINT ( 'NONE',  ( 779.4763451958990572, -368.7363362996977685, -365.0264073115438919 ) ) ;
#27183=CARTESIAN_POINT ( 'NONE',  ( 765.0180583372156207, -336.9982390220558273, -360.0135310231089534 ) ) ;
#27184=CARTESIAN_POINT ( 'NONE',  ( 786.2694204179717872, -117.2817908451530684, -305.1769319972829067 ) ) ;
#27187=CARTESIAN_POINT ( 'NONE',  ( 814.4686193811664907, -123.2817908451530542, -346.2056067578752732 ) ) ;
#27193=AXIS2_PLACEMENT_3D ( 'NONE', #392, #11025, #22089 ) ;
#27195=CARTESIAN_POINT ( 'NONE',  ( 749.2812353651451076, -294.4527844766013800, -323.2262854647983090 ) ) ;
#27202=CARTESIAN_POINT ( 'NONE',  ( 768.8385539511368734, -383.2601417444137155, -306.4236121716840557 ) ) ;
#27203=CARTESIAN_POINT ( 'NONE',  ( 801.1904061080336987, -116.0891481129656029, -368.3070685750235498 ) ) ;
#27205=CARTESIAN_POINT ( 'NONE',  ( 745.0891759886404770, -388.2709662947829656, -342.4968714119734159 ) ) ;
#27210=CARTESIAN_POINT ( 'NONE',  ( 808.7758568127978833, -148.1692326535053610, -320.0363995740631822 ) ) ;
#27215=CARTESIAN_POINT ( 'NONE',  ( 755.0488828828309806, 6.194403710130517382, -344.1219089521771934 ) ) ;
#27217=CARTESIAN_POINT ( 'NONE',  ( 810.7187646348534145, 5.547215523397618142, -356.7737145352016341 ) ) ;
#27222=CARTESIAN_POINT ( 'NONE',  ( 804.1009440267234822, -407.4636090269703459, -314.0944755984392600 ) ) ;
#27225=CARTESIAN_POINT ( 'NONE',  ( 804.4286716492782716, -257.3618753856924286, -345.3141322388244703 ) ) ;
#27228=CARTESIAN_POINT ( 'NONE',  ( 779.4763451958990572, -224.7363362996982232, -365.0264073115438919 ) ) ;
#27229=CARTESIAN_POINT ( 'NONE',  ( 800.0135310231082713, -206.0891481129653471, -325.0180583372163028 ) ) ;
#27230=CARTESIAN_POINT ( 'NONE',  ( 774.6858677611749044, -417.7255117493283478, -315.5713283507209894 ) ) ;
#27234=CARTESIAN_POINT ( 'NONE',  ( 789.7124813865536908, -452.9681489794450613, -363.0370378529873960 ) ) ;
#27235=CARTESIAN_POINT ( 'NONE',  ( 781.2370466360911223, -20.73633629969883430, -304.9990715423533629 ) ) ;
#27241=CARTESIAN_POINT ( 'NONE',  ( 813.5763878283155464, -435.8272453906066062, -351.1614460488615350 ) ) ;
#27242=CARTESIAN_POINT ( 'NONE',  ( 772.4837098697145166, -71.36187538569303968, -374.5518280994205611 ) ) ;
#27244=CARTESIAN_POINT ( 'NONE',  ( 778.1981804954714335, -418.2709662947827383, -314.8072714833589885 ) ) ;
#27245=CARTESIAN_POINT ( 'NONE',  ( 762.3223304703356007, -31.54369356751135456, -322.3223304703362828 ) ) ;
#27246=EDGE_CURVE ( 'NONE', #14459, #37618, #19067, .T. ) ;
#27249=CARTESIAN_POINT ( 'NONE',  ( 769.0155153010367712, -274.3726999360617356, -362.7791456095907279 ) ) ;
#27250=CARTESIAN_POINT ( 'NONE',  ( 754.9967657858570647, -217.5436935675107293, -365.0032342141425374 ) ) ;
#27256=CARTESIAN_POINT ( 'NONE',  ( 800.1688906516307043, -274.1692326535049915, -369.0717654672308186 ) ) ;
#27259=CARTESIAN_POINT ( 'NONE',  ( 800.9747183278959710, -276.9982390220559978, -311.9810565676471583 ) ) ;
#27264=CARTESIAN_POINT ( 'NONE',  ( 755.3201227861273992, -363.7255117493284047, -345.3687786644892981 ) ) ;
#27267=CARTESIAN_POINT ( 'NONE',  ( 778.7502325331095108, -48.35105083532386061, -304.6391490659818828 ) ) ;
#27268=CARTESIAN_POINT ( 'NONE',  ( 793.2243759319678702, -146.5328690171417350, -318.4439275373583200 ) ) ;
#27272=CARTESIAN_POINT ( 'NONE',  ( 791.9812246680005501, -68.63460265842033436, -361.9419747391813189 ) ) ;
#27273=CARTESIAN_POINT ( 'NONE',  ( 775.9200461376533440, -167.8055962898689586, -315.3028492785443291 ) ) ;
#27275=CARTESIAN_POINT ( 'NONE',  ( 754.0944755984390895, -15.62377810805123524, -364.1009440267246760 ) ) ;
#27280=CARTESIAN_POINT ( 'NONE',  ( 773.7305795820266212, -321.2817908451525000, -374.8230680027170365 ) ) ;
#27285=CARTESIAN_POINT ( 'NONE',  ( 805.2837595273609850, -98.73633629969859271, -340.5290396650784714 ) ) ;
#27286=CARTESIAN_POINT ( 'NONE',  ( 756.5762568750052424, -123.1800572038747106, -348.7366044899774238 ) ) ;
#27287=CARTESIAN_POINT ( 'NONE',  ( 795.1360043628808398, -332.0891481129649492, -360.2193346964456282 ) ) ;
#27289=CARTESIAN_POINT ( 'NONE',  ( 785.3687786644884454, -419.3618753856918033, -315.3201227861279676 ) ) ;
#27296=CARTESIAN_POINT ( 'NONE',  ( 781.2370466360911223, -332.7363362996979390, -304.9990715423533629 ) ) ;
#27298=CARTESIAN_POINT ( 'NONE',  ( 771.1735550268778070, -321.1800572038740142, -316.3353852180827630 ) ) ;
#27299=EDGE_CURVE ( 'NONE', #3536, #29825, #8440, .T. ) ;
#27301=CARTESIAN_POINT ( 'NONE',  ( 772.4468031744293057, -177.8272453906074304, -363.8651313633793620 ) ) ;
#27304=CARTESIAN_POINT ( 'NONE',  ( 744.7301800767020268, -388.8164208402374129, -337.4774526936615189 ) ) ;
#27309=CARTESIAN_POINT ( 'NONE',  ( 813.1304606946830518, -17.90732993114776406, -352.3570229623690580 ) ) ;
#27311=CARTESIAN_POINT ( 'NONE',  ( 802.1676090361156639, -230.6346026584197659, -327.8955696845344505 ) ) ;
#27315=CARTESIAN_POINT ( 'NONE',  ( 805.0264073115434940, -54.35105083532383219, -339.4763451958999099 ) ) ;
#27322=CARTESIAN_POINT ( 'NONE',  ( 755.0636971347428243, -76.27096629478394618, -341.7834795799807353 ) ) ;
#27323=CARTESIAN_POINT ( 'NONE',  ( 764.0069404352550464, -351.0783235625955854, -359.2566176426627180 ) ) ;
#27326=CARTESIAN_POINT ( 'NONE',  ( 749.8865473780648472, -356.5328690171410813, -322.1177392798429082 ) ) ;
#27332=CARTESIAN_POINT ( 'NONE',  ( 787.5162901302840055, -227.3618753856925707, -305.4481719005792684 ) ) ;
#27335=CARTESIAN_POINT ( 'NONE',  ( 756.5762568750052424, -195.1800572038744974, -348.7366044899774238 ) ) ;
#27337=CARTESIAN_POINT ( 'NONE',  ( 762.1405469898971887, -313.5436935675102745, -357.8594530101015607 ) ) ;
#27338=CARTESIAN_POINT ( 'NONE',  ( 803.4237431249931660, 8.819942796124882634, -331.2633955100225194 ) ) ;
#27344=CARTESIAN_POINT ( 'NONE',  ( 800.9840315886518738, -460.9181544815156713, -354.1144889064786412 ) ) ;
#27347=CARTESIAN_POINT ( 'NONE',  ( 745.7194118038753459, -253.6454272087889876, -348.7631598425976449 ) ) ;
#27350=CARTESIAN_POINT ( 'NONE',  ( 762.1405469898971887, -217.5436935675107293, -357.8594530101015607 ) ) ;
#27351=CARTESIAN_POINT ( 'NONE',  ( 803.8651313633788504, -365.2601417444137155, -332.4468031744301015 ) ) ;
#27352=CARTESIAN_POINT ( 'NONE',  ( 814.2805881961230625, -241.6454272087890729, -331.2368401574024119 ) ) ;
#27354=CARTESIAN_POINT ( 'NONE',  ( 780.5236548040995785, -92.73633629969860692, -314.9735926884559944 ) ) ;
#27357=CARTESIAN_POINT ( 'NONE',  ( 754.8983024940795303, -426.8965053807771142, -336.9254006560228163 ) ) ;
#27358=CARTESIAN_POINT ( 'NONE',  ( 777.5031285880264704, -286.8164208402378677, -374.9108240113588408 ) ) ;
#27360=DIRECTION ( 'NONE',  ( 0.000000000000000000, 0.000000000000000000, 1.000000000000000000 ) ) ;
#27361=CARTESIAN_POINT ( 'NONE',  ( 791.9812246680005501, -44.63460265842040542, -361.9419747391813189 ) ) ;
#27363=CARTESIAN_POINT ( 'NONE',  ( 747.3154664389472828, -163.9874144716871456, -326.4474001241230781 ) ) ;
#27365=CARTESIAN_POINT ( 'NONE',  ( 813.1304606946830518, -425.9073299311463074, -352.3570229623690580 ) ) ;
#27369=CARTESIAN_POINT ( 'NONE',  ( 795.1360043628807261, -428.0891481129644944, -360.2193346964456282 ) ) ;
#27375=CARTESIAN_POINT ( 'NONE',  ( 794.1144889064781864, -250.1692326535050199, -360.9840315886528401 ) ) ;
#27376=CARTESIAN_POINT ( 'NONE',  ( 792.1044303154645831, -132.4527844766018916, -317.8323909638837677 ) ) ;
#27378=CARTESIAN_POINT ( 'NONE',  ( 812.6845335610512393, -247.9874144716867761, -353.5525998758768651 ) ) ;
#27384=CARTESIAN_POINT ( 'NONE',  ( 776.9566956441375396, -60.89650538077837894, -364.8461984189686405 ) ) ;
#27385=CARTESIAN_POINT ( 'NONE',  ( 802.1676090361156639, -182.6346026584199649, -327.8955696845344505 ) ) ;
#27387=CARTESIAN_POINT ( 'NONE',  ( 792.2312462859673587, -107.9073299311474727, -307.2067596250082602 ) ) ;
#27388=CARTESIAN_POINT ( 'NONE',  ( 781.8018195045267476, -118.2709662947838041, -365.1927285166407273 ) ) ;
#27390=CARTESIAN_POINT ( 'NONE',  ( 793.0897708529556667, -54.55451811788054783, -361.3366627262616362 ) ) ;
#27391=CARTESIAN_POINT ( 'NONE',  ( 772.4468031744293057, -345.8272453906069472, -363.8651313633793620 ) ) ;
#27398=CARTESIAN_POINT ( 'NONE',  ( 783.0745993439762742, -368.1908817542433212, -365.1016975059196739 ) ) ;
#27399=CARTESIAN_POINT ( 'NONE',  ( 792.1044303154645831, -372.4527844766010958, -317.8323909638837677 ) ) ;
#27400=CARTESIAN_POINT ( 'NONE',  ( 748.6759233522253680, -136.3726999360621051, -324.3348316497537098 ) ) ;
#27404=CARTESIAN_POINT ( 'NONE',  ( 757.2208543904082489, -256.7146871989595525, -350.9844846989624330 ) ) ;
#27405=CARTESIAN_POINT ( 'NONE',  ( 771.3260364891663130, -163.6454272087893003, -306.0683387631859773 ) ) ;
#27412=CARTESIAN_POINT ( 'NONE',  ( 796.9462024416508257, -180.4527844766017495, -308.9653473494370246 ) ) ;
#27415=CARTESIAN_POINT ( 'NONE',  ( 759.0252816721024374, -312.9982390220559409, -368.0189434323527280 ) ) ;
#27416=FACE_OUTER_BOUND ( 'NONE', #2840, .T. ) ;
#27421=CARTESIAN_POINT ( 'NONE',  ( 810.1134526219336749, -392.5328690171409107, -357.8822607201570349 ) ) ;
#27422=CARTESIAN_POINT ( 'NONE',  ( 796.9462024416508257, -132.4527844766018916, -308.9653473494370246 ) ) ;
#27424=CARTESIAN_POINT ( 'NONE',  ( 758.8095938919642549, -392.0891481129648355, -311.6929314249763365 ) ) ;
#27428=CARTESIAN_POINT ( 'NONE',  ( 754.0944755984390895, -159.6237781080508285, -364.1009440267246760 ) ) ;
#27432=CARTESIAN_POINT ( 'NONE',  ( 754.9735926884551418, -18.35105083532395298, -340.5236548041000333 ) ) ;
#27434=CARTESIAN_POINT ( 'NONE',  ( 745.0891759886404770, -4.270966294784170003, -342.4968714119734159 ) ) ;
#27435=DIRECTION ( 'NONE',  ( -0.000000000000000000, 1.000000000000000000, -0.000000000000000000 ) ) ;
#27438=CARTESIAN_POINT ( 'NONE',  ( 744.6391490659812007, -398.7363362996976548, -338.7502325331110455 ) ) ;
#27439=CARTESIAN_POINT ( 'NONE',  ( 762.3223304703356007, -271.5436935675106156, -322.3223304703362828 ) ) ;
#27443=CARTESIAN_POINT ( 'NONE',  ( 754.7162404726377645, -254.7363362996981095, -339.4709603349214717 ) ) ;
#27444=CARTESIAN_POINT ( 'NONE',  ( 791.9812246680005501, -260.6346026584197375, -361.9419747391813189 ) ) ;
#27446=CARTESIAN_POINT ( 'NONE',  ( 757.8323909638828582, -434.6346026584190554, -352.1044303154654358 ) ) ;
#27451=CARTESIAN_POINT ( 'NONE',  ( 764.1737431748507561, -34.37269993606243901, -371.6461892240376415 ) ) ;
#27457=ORIENTED_EDGE ( 'NONE', *, *, #43102, .F. ) ;
#27458=CARTESIAN_POINT ( 'NONE',  ( 804.1105419155481968, -27.82724539060790292, -347.6308680596136469 ) ) ;
#27459=CARTESIAN_POINT ( 'NONE',  ( 787.4397851343537695, -69.72551174932942786, -374.2001403089903988 ) ) ;
#27461=CARTESIAN_POINT ( 'NONE',  ( 800.0135310231082713, -422.0891481129647218, -325.0180583372163028 ) ) ;
#27462=CARTESIAN_POINT ( 'NONE',  ( 797.8594530101009923, -37.54369356751133324, -322.1405469898982119 ) ) ;
#27464=CARTESIAN_POINT ( 'NONE',  ( 747.2067596250078623, -195.1800572038744974, -352.2312462859687230 ) ) ;
#27470=CARTESIAN_POINT ( 'NONE',  ( 752.4576283171824116, -261.0783235625959264, -317.7880784355627952 ) ) ;
#27473=CARTESIAN_POINT ( 'NONE',  ( 747.2067596250078623, -267.1800572038742985, -352.2312462859687230 ) ) ;
#27477=CARTESIAN_POINT ( 'NONE',  ( 803.4237431249931660, -351.1800572038740142, -331.2633955100225194 ) ) ;
#27479=CARTESIAN_POINT ( 'NONE',  ( 764.3348316497523456, -46.71468719896022748, -308.6759233522265617 ) ) ;
#27480=CARTESIAN_POINT ( 'NONE',  ( 754.8983024940795303, -138.8965053807781374, -336.9254006560228163 ) ) ;
#27484=CARTESIAN_POINT ( 'NONE',  ( 767.8955696845333705, -72.45278447660213317, -362.1676090361162323 ) ) ;
#27485=CARTESIAN_POINT ( 'NONE',  ( 796.7845633553578182, -177.6237781080507148, -358.5707757039688204 ) ) ;
#27488=CARTESIAN_POINT ( 'NONE',  ( 812.6845335610512393, 16.01258552831230375, -353.5525998758768651 ) ) ;
#27493=CARTESIAN_POINT ( 'NONE',  ( 788.6739635108323228, -295.6454272087888739, -373.9316612368139090 ) ) ;
#27499=CARTESIAN_POINT ( 'NONE',  ( 793.9708237608222134, -166.9181544815165523, -319.2295555964448681 ) ) ;
#27500=CARTESIAN_POINT ( 'NONE',  ( 771.1735550268778070, -105.1800572038747248, -316.3353852180827630 ) ) ;
#27510=CARTESIAN_POINT ( 'NONE',  ( 814.2805881961230625, -385.6454272087888171, -331.2368401574024119 ) ) ;
#27512=CARTESIAN_POINT ( 'NONE',  ( 785.3141322388236176, -333.7255117493286320, -364.4286716492789537 ) ) ;
#27513=CARTESIAN_POINT ( 'NONE',  ( 799.9999999999993179, -462.9681489794448339, -309.9999999999998863 ) ) ;
#27514=CARTESIAN_POINT ( 'NONE',  ( 755.3028492785439312, -183.2817908451528695, -335.9200461376539693 ) ) ;
#27517=CARTESIAN_POINT ( 'NONE',  ( 759.0252816721024374, -384.9982390220556567, -368.0189434323527280 ) ) ;
#27524=CARTESIAN_POINT ( 'NONE',  ( 745.0891759886404770, -4.270966294784170003, -342.4968714119734159 ) ) ;
#27525=CARTESIAN_POINT ( 'NONE',  ( 804.4286716492782716, -233.3618753856925423, -345.3141322388244703 ) ) ;
#27529=CARTESIAN_POINT ( 'NONE',  ( 747.6481478633932056, -37.09997266333514432, -353.4146539503763620 ) ) ;
#27530=CARTESIAN_POINT ( 'NONE',  ( 769.1273215169530886, -46.71468719896022748, -317.4527132478988847 ) ) ;
#27538=CARTESIAN_POINT ( 'NONE',  ( 764.8639956371174549, -80.08914811296574499, -319.7806653035542013 ) ) ;
#27539=CARTESIAN_POINT ( 'NONE',  ( 801.3366627262608972, -368.5328690171409676, -353.0897708529566899 ) ) ;
#27543=CARTESIAN_POINT ( 'NONE',  ( 747.3154664389472828, -379.9874144716865203, -326.4474001241230781 ) ) ;
#27550=CARTESIAN_POINT ( 'NONE',  ( 814.5518280994195948, -207.7255117493289447, -332.4837098697145734 ) ) ;
#27553=EDGE_LOOP ( 'NONE', ( #1465, #6327, #10515, #6015 ) ) ;
#27554=CARTESIAN_POINT ( 'NONE',  ( 774.6858677611749044, -201.7255117493290015, -315.5713283507209894 ) ) ;
#27556=CARTESIAN_POINT ( 'NONE',  ( 788.7366044899766848, -323.9073299311468190, -316.5762568750059813 ) ) ;
#27557=CARTESIAN_POINT ( 'NONE',  ( 800.2193346964447755, -18.99823902205683979, -355.1360043628815788 ) ) ;
#27563=CARTESIAN_POINT ( 'NONE',  ( 790.7339360641449275, -462.9631818684622999, -362.6136660859752965 ) ) ;
#27564=CARTESIAN_POINT ( 'NONE',  ( 770.0084009877317612, 19.77989614203463375, -311.3857915150574627 ) ) ;
#27566=VECTOR ( 'NONE', #22754, 1000.000000000000114 ) ;
#27568=CARTESIAN_POINT ( 'NONE',  ( 813.5763878283155464, -243.8272453906072030, -351.1614460488615350 ) ) ;
#27572=CARTESIAN_POINT ( 'NONE',  ( 771.2633955100217236, -215.9073299311471317, -363.4237431249939618 ) ) ;
#27573=CARTESIAN_POINT ( 'NONE',  ( 765.8855110935204493, -382.1692326535045936, -319.0159684113471599 ) ) ;
#27576=CARTESIAN_POINT ( 'NONE',  ( 755.5913626894240451, -85.64542720878952764, -346.6156483768012890 ) ) ;
#27580=CARTESIAN_POINT ( 'NONE',  ( 744.8212110874229666, 5.103494619221427442, -336.2046728542121627 ) ) ;
#27581=CARTESIAN_POINT ( 'NONE',  ( 744.7301800767020268, -292.8164208402378108, -337.4774526936615189 ) ) ;
#27584=CARTESIAN_POINT ( 'NONE',  ( 762.3223304703356007, -79.54369356751119824, -322.3223304703362828 ) ) ;
#27587=CARTESIAN_POINT ( 'NONE',  ( 815.0009284576459549, -174.3510508353234627, -338.7629533639073429 ) ) ;
#27589=CARTESIAN_POINT ( 'NONE',  ( 777.4774526936600978, -394.2709662947827951, -304.7301800767027657 ) ) ;
#27593=CARTESIAN_POINT ( 'NONE',  ( 794.9819416627830151, -420.9982390220555999, -319.9864689768909898 ) ) ;
#27595=FACE_BOUND ( 'NONE', #7968, .T. ) ;
#27599=CARTESIAN_POINT ( 'NONE',  ( 755.8398074228967971, -259.4419599262322436, -333.4516893846970333 ) ) ;
#27602=CARTESIAN_POINT ( 'NONE',  ( 771.2368401574024119, -253.4419599262323572, -374.2805881961240857 ) ) ;
#27607=CARTESIAN_POINT ( 'NONE',  ( 770.0799878456142551, -37.98741447168752927, -362.9823548866085616 ) ) ;
#27608=CARTESIAN_POINT ( 'NONE',  ( 754.8072714833581358, -172.8164208402381234, -338.1981804954720587 ) ) ;
#27610=CARTESIAN_POINT ( 'NONE',  ( 777.5031285880264704, -118.8164208402383508, -374.9108240113588408 ) ) ;
#27611=CARTESIAN_POINT ( 'NONE',  ( 803.6646147819162707, -113.9073299311474585, -348.8264449731211130 ) ) ;
#27613=CARTESIAN_POINT ( 'NONE',  ( 790.0220218866281812, -31.09997266333516919, -363.2186876482849129 ) ) ;
#27614=CARTESIAN_POINT ( 'NONE',  ( 798.5707757039680246, -341.4636090269705733, -356.7845633553585003 ) ) ;
#27622=CARTESIAN_POINT ( 'NONE',  ( 754.7162404726377645, -350.7363362996978253, -339.4709603349214717 ) ) ;
#27623=CARTESIAN_POINT ( 'NONE',  ( 805.1927285166397041, -352.8164208402374129, -341.8018195045277707 ) ) ;
#27624=CARTESIAN_POINT ( 'NONE',  ( 760.0363995740630116, -130.9181544815166660, -368.7758568127991907 ) ) ;
#27628=CARTESIAN_POINT ( 'NONE',  ( 756.7813123517142913, -307.9874144716866340, -329.9779781133712504 ) ) ;
#27629=CARTESIAN_POINT ( 'NONE',  ( 795.8262568251477660, -166.3726999360620198, -308.3538107759623585 ) ) ;
#27630=DIRECTION ( 'NONE',  ( 0.000000000000000000, -1.000000000000000000, 0.000000000000000000 ) ) ;
#27631=DIRECTION ( 'NONE',  ( 0.000000000000000000, 0.000000000000000000, -1.000000000000000000 ) ) ;
#27636=CARTESIAN_POINT ( 'NONE',  ( 748.9653473494365699, -170.6346026584199933, -356.9462024416520762 ) ) ;
#27640=CARTESIAN_POINT ( 'NONE',  ( 767.6429770376289525, -321.1800572038740142, -306.8695393053162093 ) ) ;
#27646=CARTESIAN_POINT ( 'NONE',  ( 800.1688906516307043, -370.1692326535045936, -369.0717654672308186 ) ) ;
#27647=CARTESIAN_POINT ( 'NONE',  ( 814.9108240113580450, -136.2709662947837330, -337.5031285880265273 ) ) ;
#27651=CARTESIAN_POINT ( 'NONE',  ( 782.4968714119720516, -370.8164208402375834, -305.0891759886411023 ) ) ;
#27657=CARTESIAN_POINT ( 'NONE',  ( 812.6845335610512393, -151.9874144716871740, -353.5525998758768651 ) ) ;
#27663=CARTESIAN_POINT ( 'NONE',  ( 755.8398074228967971, -19.44195992623303937, -333.4516893846970333 ) ) ;
#27666=CARTESIAN_POINT ( 'NONE',  ( 812.7932403749906598, -15.18005720387504631, -327.7687537140311633 ) ) ;
#27671=CARTESIAN_POINT ( 'NONE',  ( 783.7953271457878373, -416.1908817542430938, -375.1787889125761239 ) ) ;
#27673=CARTESIAN_POINT ( 'NONE',  ( 803.6646147819161570, -257.9073299311469896, -348.8264449731210561 ) ) ;
#27677=CARTESIAN_POINT ( 'NONE',  ( 802.5472867521000353, -268.3726999360616787, -350.8726784830461156 ) ) ;
#27678=CARTESIAN_POINT ( 'NONE',  ( 785.3141322388236176, -261.7255117493288026, -364.4286716492789537 ) ) ;
#27679=CARTESIAN_POINT ( 'NONE',  ( 803.6646147819162707, -401.9073299311464211, -348.8264449731211130 ) ) ;
#27680=CARTESIAN_POINT ( 'NONE',  ( 755.3201227861273992, -75.72551174932937101, -345.3687786644892981 ) ) ;
#27686=CARTESIAN_POINT ( 'NONE',  ( 752.7379699480933368, -60.00906357242598688, -361.9858362298580232 ) ) ;
#27692=ORIENTED_EDGE ( 'NONE', *, *, #33400, .F. ) ;
#27693=CARTESIAN_POINT ( 'NONE',  ( 796.9571628226829034, 0.5363909730283709099, -321.2382568024804641 ) ) ;
#27694=CARTESIAN_POINT ( 'NONE',  ( 763.2262854647970016, -56.63460265842036279, -309.2812353651462445 ) ) ;
#27696=CARTESIAN_POINT ( 'NONE',  ( 800.2193346964447755, -426.9982390220554862, -355.1360043628815788 ) ) ;
#27697=CARTESIAN_POINT ( 'NONE',  ( 754.8072714833583632, -52.81642084023856398, -338.1981804954721156 ) ) ;
#27699=CARTESIAN_POINT ( 'NONE',  ( 777.5031285880264704, -190.8164208402381234, -374.9108240113588408 ) ) ;
#27705=CARTESIAN_POINT ( 'NONE',  ( 746.0683387631852383, -283.4419599262321867, -331.3260364891676204 ) ) ;
#27708=CARTESIAN_POINT ( 'NONE',  ( 745.0891759886404770, -268.2709662947833067, -342.4968714119734159 ) ) ;
#27712=CARTESIAN_POINT ( 'NONE',  ( 778.1981804954714335, -394.2709662947827951, -314.8072714833589885 ) ) ;
#27714=CARTESIAN_POINT ( 'NONE',  ( 748.3538107759620743, -64.71468719896019195, -355.8262568251490165 ) ) ;
#27715=CARTESIAN_POINT ( 'NONE',  ( 759.2295555964440155, -160.1692326535053326, -353.9708237608231229 ) ) ;
#27720=CARTESIAN_POINT ( 'NONE',  ( 759.7806653035534055, -78.99823902205662307, -324.8639956371180801 ) ) ;
#27721=CARTESIAN_POINT ( 'NONE',  ( 789.9200121543843807, -193.9874144716870319, -317.0176451133914384 ) ) ;
#27725=CARTESIAN_POINT ( 'NONE',  ( 813.9316612368132837, 16.55804007376685050, -348.6739635108323228 ) ) ;
#27730=CARTESIAN_POINT ( 'NONE',  ( 814.4686193811664907, -291.2817908451525000, -346.2056067578752732 ) ) ;
#27734=CARTESIAN_POINT ( 'NONE',  ( 759.0159684113467620, -136.9181544815166376, -325.8855110935213020 ) ) ;
#27735=CARTESIAN_POINT ( 'NONE',  ( 758.0580252608178853, -150.4527844766018916, -328.0187753319985404 ) ) ;
#27736=CARTESIAN_POINT ( 'NONE',  ( 771.1735550268780344, -321.1800572038740711, -316.3353852180828198 ) ) ;
#27746=CARTESIAN_POINT ( 'NONE',  ( 811.3240766477731540, -364.3726999360614514, -355.6651683502462902 ) ) ;
#27750=CARTESIAN_POINT ( 'NONE',  ( 759.9864689768902508, -314.0891481129650629, -354.9819416627836404 ) ) ;
#27752=CARTESIAN_POINT ( 'NONE',  ( 757.4527132478984868, -232.3726999360617924, -329.1273215169538844 ) ) ;
#27756=CARTESIAN_POINT ( 'NONE',  ( 811.0346526505617248, -422.6346026584191691, -323.0537975583478101 ) ) ;
#27761=CARTESIAN_POINT ( 'NONE',  ( 808.0189434323515343, -62.08914811296580183, -319.0252816721025511 ) ) ;
#27762=CARTESIAN_POINT ( 'NONE',  ( 804.4286716492782716, -281.3618753856923718, -345.3141322388244703 ) ) ;
#27767=CARTESIAN_POINT ( 'NONE',  ( 744.6391490659812007, -14.73633629969885384, -338.7502325331110455 ) ) ;
#27768=CARTESIAN_POINT ( 'NONE',  ( 754.9735926884551418, -66.35105083532378956, -340.5236548041000333 ) ) ;
#27774=CARTESIAN_POINT ( 'NONE',  ( 781.8018195045266339, -70.27096629478397460, -365.1927285166406705 ) ) ;
#27776=VECTOR ( 'NONE', #26082, 1000.000000000000000 ) ;
#27778=CARTESIAN_POINT ( 'NONE',  ( 786.6156483768007774, -361.4419599262319593, -315.5913626894246136 ) ) ;
#27782=CARTESIAN_POINT ( 'NONE',  ( 793.4146539503750546, -385.9874144716864066, -307.6481478633938877 ) ) ;
#27789=CARTESIAN_POINT ( 'NONE',  ( 811.0346526505616112, -230.6346026584197659, -323.0537975583477532 ) ) ;
#27793=CARTESIAN_POINT ( 'NONE',  ( 764.8639956371174549, -224.0891481129652902, -319.7806653035542581 ) ) ;
#27796=CARTESIAN_POINT ( 'NONE',  ( 805.1927285166397041, -376.8164208402375834, -341.8018195045277707 ) ) ;
#27797=CARTESIAN_POINT ( 'NONE',  ( 804.9363028652555840, -16.27096629478413092, -338.2165204200192079 ) ) ;
#27803=CARTESIAN_POINT ( 'NONE',  ( 778.2165204200184689, 1.183579159761269040, -364.9363028652563230 ) ) ;
#27805=LINE ( 'NONE', #34953, #12289 ) ;
#27807=CARTESIAN_POINT ( 'NONE',  ( 755.8990559732751535, -275.4636090269708575, -365.9055244015606831 ) ) ;
#27810=CARTESIAN_POINT ( 'NONE',  ( 781.7834795799800531, -226.8164208402380098, -315.0636971347436202 ) ) ;
#27811=CARTESIAN_POINT ( 'NONE',  ( 804.9511171171677688, -389.8055962898682765, -335.8780910478229202 ) ) ;
#27813=CARTESIAN_POINT ( 'NONE',  ( 764.8639956371174549, 15.91085188703394593, -319.7806653035542581 ) ) ;
#27814=CARTESIAN_POINT ( 'NONE',  ( 804.4086373105744769, -97.64542720878949922, -333.3843516231986541 ) ) ;
#27818=CARTESIAN_POINT ( 'NONE',  ( 744.9990715423526808, 5.648949164675971524, -341.2370466360926002 ) ) ;
#27819=CARTESIAN_POINT ( 'NONE',  ( 801.1904061080338124, -308.0891481129650629, -368.3070685750236066 ) ) ;
#27822=CARTESIAN_POINT ( 'NONE',  ( 759.9864689768902508, -74.08914811296577341, -354.9819416627836404 ) ) ;
#27826=CARTESIAN_POINT ( 'NONE',  ( 748.3538107759620743, -184.7146871989598083, -355.8262568251490165 ) ) ;
#27828=CARTESIAN_POINT ( 'NONE',  ( 745.7998596910086917, -437.3618753856919170, -332.5602148656461168 ) ) ;
#27834=CARTESIAN_POINT ( 'NONE',  ( 757.8323909638827445, -434.6346026584190554, -352.1044303154654358 ) ) ;
#27836=PLANE ( 'NONE',  #44630 ) ;
#27841=CARTESIAN_POINT ( 'NONE',  ( 784.0799538623451781, -251.8055962898686744, -364.6971507214555572 ) ) ;
#27843=CARTESIAN_POINT ( 'NONE',  ( 783.7566961878529810, -264.8965053807776826, -305.1792804349288417 ) ) ;
#27848=CARTESIAN_POINT ( 'NONE',  ( 803.2186876482843445, -31.98741447168754348, -350.0220218866286928 ) ) ;
#27849=CARTESIAN_POINT ( 'NONE',  ( 758.0580252608178853, -150.4527844766018916, -328.0187753319985404 ) ) ;
#27850=CARTESIAN_POINT ( 'NONE',  ( 768.0187753319979720, -200.6346026584199365, -318.0580252608186242 ) ) ;
#27852=CARTESIAN_POINT ( 'NONE',  ( 749.2812353651451076, -126.4527844766019626, -323.2262854647983090 ) ) ;
#27854=CARTESIAN_POINT ( 'NONE',  ( 788.8264449731201466, -93.18005720387479585, -363.6646147819170665 ) ) ;
#27856=CARTESIAN_POINT ( 'NONE',  ( 804.6971507214547046, -51.28179084515328867, -344.0799538623459739 ) ) ;
#27858=CARTESIAN_POINT ( 'NONE',  ( 760.7433823573367135, -396.0090635724249637, -355.9930595647440441 ) ) ;
#27866=CARTESIAN_POINT ( 'NONE',  ( 804.6971507214547046, -363.2817908451523294, -344.0799538623459739 ) ) ;
#27867=CARTESIAN_POINT ( 'NONE',  ( 774.6312213355099630, -359.3618753856920875, -364.6798772138717482 ) ) ;
#27868=CARTESIAN_POINT ( 'NONE',  ( 745.5313806188320314, -159.2817908451529547, -333.7943932421247268 ) ) ;
#27872=CARTESIAN_POINT ( 'NONE',  ( 770.0799878456142551, -277.9874144716867477, -362.9823548866085616 ) ) ;
#27873=CARTESIAN_POINT ( 'NONE',  ( 756.5762568750052424, -435.1800572038737869, -348.7366044899774238 ) ) ;
#27874=CARTESIAN_POINT ( 'NONE',  ( 811.3240766477731540, -148.3726999360620198, -355.6651683502462902 ) ) ;
#27879=CARTESIAN_POINT ( 'NONE',  ( 772.4837098697145166, -167.3618753856927412, -374.5518280994205611 ) ) ;
#27883=CARTESIAN_POINT ( 'NONE',  ( 772.4837098697144029, -311.3618753856922581, -374.5518280994205611 ) ) ;
#27888=CARTESIAN_POINT ( 'NONE',  ( 773.7943932421234194, -383.8055962898682765, -305.5313806188329409 ) ) ;
#27889=VECTOR ( 'NONE', #754, 1000.000000000000000 ) ;
#27890=CARTESIAN_POINT ( 'NONE',  ( 804.7487373415286811, -139.5436935675110135, -364.7487373415288516 ) ) ;
#27891=CARTESIAN_POINT ( 'NONE',  ( 745.4481719005789273, -387.7255117493283478, -347.5162901302853129 ) ) ;
#27896=CARTESIAN_POINT ( 'NONE',  ( 813.9316612368132837, -151.4419599262326415, -348.6739635108323228 ) ) ;
#27902=CARTESIAN_POINT ( 'NONE',  ( 767.7687537140311633, -23.90732993114773919, -372.7932403749916830 ) ) ;
#27903=DIRECTION ( 'NONE',  ( -1.000000000000000000, -0.000000000000000000, -0.000000000000000000 ) ) ;
#27905=CARTESIAN_POINT ( 'NONE',  ( 807.2620300519052989, -408.0090635724249069, -318.0141637701419768 ) ) ;
#27908=CARTESIAN_POINT ( 'NONE',  ( 774.6312213355099630, -263.3618753856924855, -364.6798772138717482 ) ) ;
#27911=CARTESIAN_POINT ( 'NONE',  ( 775.8780910478218402, -249.2817908451526421, -364.9511171171680530 ) ) ;
#27912=CARTESIAN_POINT ( 'NONE',  ( 756.3353852180819104, -269.9073299311468190, -331.1735550268788302 ) ) ;
#27914=CARTESIAN_POINT ( 'NONE',  ( 765.0180583372156207, -72.99823902205667991, -360.0135310231089534 ) ) ;
#27920=CARTESIAN_POINT ( 'NONE',  ( 809.0717654672305343, -52.91815448151692891, -360.1688906516309885 ) ) ;
#27926=CARTESIAN_POINT ( 'NONE',  ( 793.0897708529556667, -6.554518117880697048, -361.3366627262616362 ) ) ;
#27927=CARTESIAN_POINT ( 'NONE',  ( 745.0891759886404770, -76.27096629478394618, -342.4968714119734159 ) ) ;
#27929=CARTESIAN_POINT ( 'NONE',  ( 801.9419747391806368, -426.4527844766010389, -351.9812246680014027 ) ) ;
#27931=CARTESIAN_POINT ( 'NONE',  ( 792.3570229623688874, -213.1800572038743553, -373.1304606946836202 ) ) ;
#27934=CARTESIAN_POINT ( 'NONE',  ( 747.3154664389472828, -259.9874144716869182, -326.4474001241230781 ) ) ;
#27936=CARTESIAN_POINT ( 'NONE',  ( 745.7998596910086917, -293.3618753856923718, -332.5602148656461168 ) ) ;
#27940=CARTESIAN_POINT ( 'NONE',  ( 785.3687786644884454, -371.3618753856919739, -315.3201227861279676 ) ) ;
#27942=CARTESIAN_POINT ( 'NONE',  ( 802.1676090361156639, -206.6346026584198512, -327.8955696845344505 ) ) ;
#27943=CARTESIAN_POINT ( 'NONE',  ( 744.8212110874229666, -42.89650538077842157, -336.2046728542121627 ) ) ;
#27944=CARTESIAN_POINT ( 'NONE',  ( 764.0069404352550464, -183.0783235625961538, -359.2566176426627180 ) ) ;
#27949=CARTESIAN_POINT ( 'NONE',  ( 783.0433043558608688, -192.8965053807779668, -315.1538015810313027 ) ) ;
#27951=CARTESIAN_POINT ( 'NONE',  ( 744.9990715423526808, -42.35105083532388193, -341.2370466360926002 ) ) ;
#27956=CARTESIAN_POINT ( 'NONE',  ( 754.3581564841646241, -305.4636090269706870, -316.1443688327762516 ) ) ;
#27960=CARTESIAN_POINT ( 'NONE',  ( 776.9254006560222479, -140.1908817542438896, -314.8983024940802125 ) ) ;
#27961=CARTESIAN_POINT ( 'NONE',  ( 795.1360043628807261, -140.0891481129654892, -360.2193346964456282 ) ) ;
#27962=CARTESIAN_POINT ( 'NONE',  ( 785.3141322388236176, -333.7255117493286320, -364.4286716492789537 ) ) ;
#27970=CARTESIAN_POINT ( 'NONE',  ( 793.5525998758768083, -367.0999726633342561, -372.6845335610516941 ) ) ;
#27975=CARTESIAN_POINT ( 'NONE',  ( 778.2165204200184689, -310.8164208402377540, -364.9363028652563230 ) ) ;
#27977=CARTESIAN_POINT ( 'NONE',  ( 787.5531968255692163, -213.8272453906073167, -316.1348686366205811 ) ) ;
#27981=CARTESIAN_POINT ( 'NONE',  ( 814.9108240113580450, -424.2709662947829088, -337.5031285880265273 ) ) ;
#27986=CARTESIAN_POINT ( 'NONE',  ( 792.3570229623688874, -69.18005720387488111, -373.1304606946836202 ) ) ;
#27987=CARTESIAN_POINT ( 'NONE',  ( 778.1981804954714335, -298.2709662947830793, -314.8072714833589885 ) ) ;
#27991=CARTESIAN_POINT ( 'NONE',  ( 814.4686193811664907, -27.28179084515336328, -346.2056067578752732 ) ) ;
#27992=CARTESIAN_POINT ( 'NONE',  ( 795.9930595647434757, -99.07832356259642381, -320.7433823573372820 ) ) ;
#27998=CARTESIAN_POINT ( 'NONE',  ( 803.8651313633788504, -101.2601417444146250, -332.4468031744301015 ) ) ;
#28000=CARTESIAN_POINT ( 'NONE',  ( 759.9864689768902508, -50.08914811296584446, -354.9819416627836404 ) ) ;
#28001=CARTESIAN_POINT ( 'NONE',  ( 757.2208543904082489, -376.7146871989592682, -350.9844846989624330 ) ) ;
#28005=CARTESIAN_POINT ( 'NONE',  ( 746.0683387631852383, -403.4419599262317888, -331.3260364891676204 ) ) ;
#28010=CARTESIAN_POINT ( 'NONE',  ( 782.5225473063381969, -262.2709662947831930, -375.2698199232970637 ) ) ;
#28014=CARTESIAN_POINT ( 'NONE',  ( 778.2165204200184689, -214.8164208402380666, -364.9363028652563230 ) ) ;
#28016=CARTESIAN_POINT ( 'NONE',  ( 771.2633955100217236, -359.9073299311467053, -363.4237431249939618 ) ) ;
#28017=CARTESIAN_POINT ( 'NONE',  ( 754.8072714833581358, -4.816420840238714085, -338.1981804954720587 ) ) ;
#28023=CARTESIAN_POINT ( 'NONE',  ( 774.6858677611749044, 14.27448825067031812, -315.5713283507209894 ) ) ;
#28024=FACE_OUTER_BOUND ( 'NONE', #27048, .T. ) ;
#28027=CARTESIAN_POINT ( 'NONE',  ( 762.1177392798416577, -258.5545181178799226, -309.8865473780659272 ) ) ;
#28030=CARTESIAN_POINT ( 'NONE',  ( 791.9812246680005501, -236.6346026584198228, -361.9419747391813189 ) ) ;
#28031=CARTESIAN_POINT ( 'NONE',  ( 754.8983024940795303, -402.8965053807773415, -336.9254006560228163 ) ) ;
#28034=CARTESIAN_POINT ( 'NONE',  ( 786.5483106153019435, -103.6454272087894850, -364.1601925771022366 ) ) ;
#28038=CARTESIAN_POINT ( 'NONE',  ( 815.1787889125755555, 17.10349461922139369, -343.7953271457877804 ) ) ;
#28039=CARTESIAN_POINT ( 'NONE',  ( 808.0189434323515343, -302.0891481129650629, -319.0252816721025511 ) ) ;
#28041=CARTESIAN_POINT ( 'NONE',  ( 795.1360043628807261, -92.08914811296568814, -360.2193346964456282 ) ) ;
#28043=CARTESIAN_POINT ( 'NONE',  ( 798.0661480581538854, -218.5328690171414792, -309.5768839229118043 ) ) ;
#28045=CARTESIAN_POINT ( 'NONE',  ( 772.5602148656447525, -441.7255117493282910, -305.7998596910095443 ) ) ;
#28050=CARTESIAN_POINT ( 'NONE',  ( 805.1927285166397041, -448.8164208402371855, -341.8018195045277707 ) ) ;
#28056=ORIENTED_EDGE ( 'NONE', *, *, #28958, .T. ) ;
#28057=CARTESIAN_POINT ( 'NONE',  ( 805.0264073115434940, -270.3510508353231216, -339.4763451958999099 ) ) ;
#28059=CARTESIAN_POINT ( 'NONE',  ( 764.3348316497523456, -286.7146871989594388, -308.6759233522265617 ) ) ;
#28064=CARTESIAN_POINT ( 'NONE',  ( 759.9864689768902508, -194.0891481129654039, -354.9819416627836404 ) ) ;
#28066=CARTESIAN_POINT ( 'NONE',  ( 800.9747183278959710, -156.9982390220564241, -311.9810565676471583 ) ) ;
#28067=CARTESIAN_POINT ( 'NONE',  ( 759.9864689768902508, -98.08914811296568814, -354.9819416627836404 ) ) ;
#28069=CARTESIAN_POINT ( 'NONE',  ( 783.0745993439762742, -392.1908817542432075, -365.1016975059196739 ) ) ;
#28070=ADVANCED_FACE ( 'NONE', ( #18787 ), #5352, .T. ) ;
#28079=CARTESIAN_POINT ( 'NONE',  ( 793.9708237608222134, -358.9181544815160123, -319.2295555964448681 ) ) ;
#28080=CARTESIAN_POINT ( 'NONE',  ( 762.1405469898971887, -361.5436935675103882, -357.8594530101015607 ) ) ;
#28081=CARTESIAN_POINT ( 'NONE',  ( 752.7379699480933368, -156.0090635724256742, -361.9858362298580232 ) ) ;
#28085=CARTESIAN_POINT ( 'NONE',  ( 754.9735926884551418, -282.3510508353230080, -340.5236548041000333 ) ) ;
#28086=CARTESIAN_POINT ( 'NONE',  ( 762.3223304703356007, -439.5436935675101040, -322.3223304703362828 ) ) ;
#28087=CARTESIAN_POINT ( 'NONE',  ( 762.1177392798416577, -138.5545181178802636, -309.8865473780659272 ) ) ;
#28091=EDGE_CURVE ( 'NONE', #37323, #29612, #31280, .T. ) ;
#28094=CARTESIAN_POINT ( 'NONE',  ( 746.8695393053151292, -197.9073299311472169, -327.6429770376306578 ) ) ;
#28098=CARTESIAN_POINT ( 'NONE',  ( 766.5853460496234675, -109.9874144716873019, -372.3518521366060554 ) ) ;
#28099=CARTESIAN_POINT ( 'NONE',  ( 782.4968714119720516, -322.8164208402377540, -305.0891759886411023 ) ) ;
#28103=ORIENTED_EDGE ( 'NONE', *, *, #42420, .T. ) ;
#28105=CARTESIAN_POINT ( 'NONE',  ( 813.2346286133761168, -365.2601417444137155, -328.9521613784389160 ) ) ;
#28106=CARTESIAN_POINT ( 'NONE',  ( 748.9653473494363425, -146.6346026584200217, -356.9462024416521331 ) ) ;
#28107=CARTESIAN_POINT ( 'NONE',  ( 763.0537975583475827, -408.4527844766009252, -371.0346526505627480 ) ) ;
#28114=CARTESIAN_POINT ( 'NONE',  ( 746.7653713866222915, -185.2601417444143692, -351.0478386215610271 ) ) ;
#28118=ORIENTED_EDGE ( 'NONE', *, *, #25160, .F. ) ;
#28120=CARTESIAN_POINT ( 'NONE',  ( 814.5518280994195948, -15.72551174932958951, -332.4837098697145734 ) ) ;
#28123=CARTESIAN_POINT ( 'NONE',  ( 745.5313806188320314, -423.2817908451521589, -333.7943932421247268 ) ) ;
#28124=ORIENTED_EDGE ( 'NONE', *, *, #43023, .T. ) ;
#28127=CARTESIAN_POINT ( 'NONE',  ( 781.7834795799800531, -274.8164208402378108, -315.0636971347436202 ) ) ;
#28132=CARTESIAN_POINT ( 'NONE',  ( 763.0428371773158460, -251.4636090269709143, -358.7617431975195359 ) ) ;
#28133=CARTESIAN_POINT ( 'NONE',  ( 771.1735550268778070, -249.1800572038742416, -316.3353852180827630 ) ) ;
#28134=CARTESIAN_POINT ( 'NONE',  ( 804.4286716492782716, -449.3618753856918602, -345.3141322388244703 ) ) ;
#28135=CARTESIAN_POINT ( 'NONE',  ( 754.8072714833581358, -124.8164208402383508, -338.1981804954720587 ) ) ;
#28140=CARTESIAN_POINT ( 'NONE',  ( 802.2119215644370342, -54.00906357242601530, -367.5423716828165084 ) ) ;
#28148=CARTESIAN_POINT ( 'NONE',  ( 801.5560724626406000, -24.55451811788064020, -326.7756240680316182 ) ) ;
#28150=CARTESIAN_POINT ( 'NONE',  ( 787.4397851343537695, -93.72551174932934259, -374.2001403089903988 ) ) ;
#28154=CARTESIAN_POINT ( 'NONE',  ( 777.4774526936600978, -250.2709662947832783, -304.7301800767027657 ) ) ;
#28158=CARTESIAN_POINT ( 'NONE',  ( 795.6651683502461765, -274.7146871989594388, -371.3240766477733814 ) ) ;
#28160=CARTESIAN_POINT ( 'NONE',  ( 787.5162901302840055, -323.3618753856923149, -305.4481719005792684 ) ) ;
#28164=CARTESIAN_POINT ( 'NONE',  ( 781.7834795799800531, -370.8164208402375834, -315.0636971347436202 ) ) ;
#28166=CARTESIAN_POINT ( 'NONE',  ( 744.9990715423526808, -42.35105083532388193, -341.2370466360926002 ) ) ;
#28167=CARTESIAN_POINT ( 'NONE',  ( 763.2154366446407039, -189.6237781080507148, -321.4292242960311228 ) ) ;
#28171=CARTESIAN_POINT ( 'NONE',  ( 759.2295555964440155, -184.1692326535052757, -353.9708237608231229 ) ) ;
#28173=CARTESIAN_POINT ( 'NONE',  ( 752.4576283171824116, -21.07832356259667250, -317.7880784355627952 ) ) ;
#28179=CARTESIAN_POINT ( 'NONE',  ( 781.2370466360911223, -308.7363362996979390, -304.9990715423533629 ) ) ;
#28182=CARTESIAN_POINT ( 'NONE',  ( 769.9779781133707957, -139.0999726633348530, -316.7813123517150871 ) ) ;
#28183=CARTESIAN_POINT ( 'NONE',  ( 803.4237431249931660, -159.1800572038746111, -331.2633955100225194 ) ) ;
#28184=CARTESIAN_POINT ( 'NONE',  ( 802.1676090361155502, -350.6346026584193396, -327.8955696845344505 ) ) ;
#28185=ORIENTED_EDGE ( 'NONE', *, *, #8376, .F. ) ;
#28193=CARTESIAN_POINT ( 'NONE',  ( 813.5763878283155464, -387.8272453906067767, -351.1614460488615350 ) ) ;
#28197=CARTESIAN_POINT ( 'NONE',  ( 801.9419747391806368, -378.4527844766011526, -351.9812246680014027 ) ) ;
#28199=CARTESIAN_POINT ( 'NONE',  ( 754.7162404726377645, -230.7363362996981664, -339.4709603349214717 ) ) ;
#28203=CARTESIAN_POINT ( 'NONE',  ( 744.7301800767020268, -412.8164208402373561, -337.4774526936615189 ) ) ;
#28208=CARTESIAN_POINT ( 'NONE',  ( 801.1904061080336987, -44.08914811296584446, -368.3070685750235498 ) ) ;
#28209=CARTESIAN_POINT ( 'NONE',  ( 805.1927285166397041, -280.8164208402378677, -341.8018195045277707 ) ) ;
#28213=CARTESIAN_POINT ( 'NONE',  ( 815.3608509340175488, -26.73633629969882008, -341.2497674668889545 ) ) ;
#28214=CARTESIAN_POINT ( 'NONE',  ( 794.1144889064781864, -82.16923265350558836, -360.9840315886528401 ) ) ;
#28217=CARTESIAN_POINT ( 'NONE',  ( 799.9999999999993179, 205.0000000000000568, -350.0000000000000000 ) ) ;
#28218=CARTESIAN_POINT ( 'NONE',  ( 774.6858677611749044, 14.27448825067031812, -315.5713283507209894 ) ) ;
#28220=CARTESIAN_POINT ( 'NONE',  ( 778.1981804954714335, -82.27096629478388934, -314.8072714833589885 ) ) ;
#28221=CARTESIAN_POINT ( 'NONE',  ( 776.9566956441375396, -396.8965053807772847, -364.8461984189686405 ) ) ;
#28225=CARTESIAN_POINT ( 'NONE',  ( 751.2241431872005251, -400.1692326535045936, -359.9636004259367610 ) ) ;
#28227=CARTESIAN_POINT ( 'NONE',  ( 772.4999999999993179, -512.9681489794448908, -350.0000000000000000 ) ) ;
#28231=CARTESIAN_POINT ( 'NONE',  ( 754.9967657858570647, -241.5436935675106156, -365.0032342141425374 ) ) ;
#28234=CARTESIAN_POINT ( 'NONE',  ( 758.0580252608178853, -246.4527844766016074, -328.0187753319985404 ) ) ;
#28236=CARTESIAN_POINT ( 'NONE',  ( 785.3687786644884454, -347.3618753856922012, -315.3201227861279676 ) ) ;
#28237=CARTESIAN_POINT ( 'NONE',  ( 767.8955696845333705, -24.45278447660229304, -362.1676090361162323 ) ) ;
#28240=CARTESIAN_POINT ( 'NONE',  ( 767.9999999999992042, 205.0000000000000568, -360.0000000000000000 ) ) ;
#28241=ORIENTED_EDGE ( 'NONE', *, *, #11776, .T. ) ;
#28242=CARTESIAN_POINT ( 'NONE',  ( 797.8594530101008786, -13.54369356751140785, -322.1405469898980982 ) ) ;
#28245=CARTESIAN_POINT ( 'NONE',  ( 797.8822607201568644, -270.5545181178798657, -370.1134526219340160 ) ) ;
#28247=CARTESIAN_POINT ( 'NONE',  ( 804.9363028652555840, -256.2709662947834204, -338.2165204200192079 ) ) ;
#28248=CARTESIAN_POINT ( 'NONE',  ( 804.1601925771018387, -391.4419599262317888, -346.5483106153029098 ) ) ;
#28250=CARTESIAN_POINT ( 'NONE',  ( 805.2837595273609850, -122.7363362996985074, -340.5290396650784714 ) ) ;
#28253=CARTESIAN_POINT ( 'NONE',  ( 759.8311093483677041, 1.830767346494167391, -310.9282345327691814 ) ) ;
#28254=CARTESIAN_POINT ( 'NONE',  ( 800.9747183278959710, -324.9982390220559409, -311.9810565676471583 ) ) ;
#28255=CARTESIAN_POINT ( 'NONE',  ( 799.9999999999993179, 205.0000000000000568, -339.9999999999999432 ) ) ;
#28257=CARTESIAN_POINT ( 'NONE',  ( 771.1735550268778070, -81.18005720387481006, -316.3353852180827630 ) ) ;
#28260=CARTESIAN_POINT ( 'NONE',  ( 814.8230680027162407, -197.8055962898688733, -333.7305795820267917 ) ) ;
#28262=CARTESIAN_POINT ( 'NONE',  ( 813.1304606946830518, -449.9073299311463643, -352.3570229623690580 ) ) ;
#28266=CARTESIAN_POINT ( 'NONE',  ( 763.2154366446407039, 26.37622189194863509, -321.4292242960311228 ) ) ;
#28272=ORIENTED_EDGE ( 'NONE', *, *, #45291, .T. ) ;
#28273=CARTESIAN_POINT ( 'NONE',  ( 769.1273215169530886, -310.7146871989593251, -317.4527132478988847 ) ) ;
#28275=CARTESIAN_POINT ( 'NONE',  ( 752.4576283171824116, -285.0783235625958127, -317.7880784355627952 ) ) ;
#28281=CARTESIAN_POINT ( 'NONE',  ( 804.1601925771018387, -55.44195992623293989, -346.5483106153029098 ) ) ;
#28282=CARTESIAN_POINT ( 'NONE',  ( 797.6776695296629214, -163.5436935675109567, -357.6776695296636603 ) ) ;
#28283=CARTESIAN_POINT ( 'NONE',  ( 778.2165204200184689, -214.8164208402380666, -364.9363028652563230 ) ) ;
#28286=CARTESIAN_POINT ( 'NONE',  ( 772.5602148656447525, -153.7255117493291721, -305.7998596910095443 ) ) ;
#28288=CARTESIAN_POINT ( 'NONE',  ( 794.9819416627830151, -132.9982390220564810, -319.9864689768909898 ) ) ;
#28290=CARTESIAN_POINT ( 'NONE',  ( 773.4516893846965786, -379.6454272087886466, -315.8398074228977066 ) ) ;
#28293=B_SPLINE_CURVE_WITH_KNOTS ( 'NONE', 3,
 ( #29101, #28648, #8306, #4606, #18701, #36249, #233, #25636, #10871, #39270, #21476, #4836, #15252, #18939, #21949, #32792, #14572, #14328, #699, #29340, #1144, #43412, #11090, #18024, #42726, #28406, #7625, #43185, #21702, #32102, #22158, #39515, #15013, #42505, #11780, #39053 ),
 .UNSPECIFIED., .F., .F.,
 ( 4, 2, 2, 2, 2, 2, 2, 2, 2, 2, 2, 2, 2, 2, 2, 2, 2, 4 ),
 ( 0.0008252806733485880007, 0.001104729680136533072, 0.001384178686924478251, 0.001943076700500593040, 0.002501974714076708045, 0.003060872727652823484, 0.004178668754804788950, 0.005296464781956755283, 0.007532056836260687949, 0.009767648890564618880, 0.01423883299917248421, 0.01871001710778034607, 0.02094560916208429782, 0.02318120121638824610, 0.02765238532499614266, 0.02988797737930003542, 0.03212356943360392819, 0.03659475354221209537 ),
 .UNSPECIFIED. ) ;
#28298=CARTESIAN_POINT ( 'NONE',  ( 779.4763451958990572, -392.7363362996977116, -365.0264073115438919 ) ) ;
#28299=CARTESIAN_POINT ( 'NONE',  ( 797.6776695296629214, -355.5436935675103882, -357.6776695296636603 ) ) ;
#28300=CARTESIAN_POINT ( 'NONE',  ( 805.6418435158337843, -173.4636090269710849, -363.8556311672236916 ) ) ;
#28303=DIRECTION ( 'NONE',  ( 0.000000000000000000, 0.000000000000000000, 1.000000000000000000 ) ) ;
#28305=CARTESIAN_POINT ( 'NONE',  ( 772.3691319403857278, -287.2601417444140566, -315.8894580844506663 ) ) ;
#28306=CARTESIAN_POINT ( 'NONE',  ( 758.0580252608178853, -438.4527844766009821, -328.0187753319985404 ) ) ;
#28307=CARTESIAN_POINT ( 'NONE',  ( 757.7880784355613741, -138.0090635724257311, -312.4576283171834916 ) ) ;
#28308=DIRECTION ( 'NONE',  ( 0.000000000000000000, 0.000000000000000000, 1.000000000000000000 ) ) ;
#28312=CARTESIAN_POINT ( 'NONE',  ( 759.0252816721024374, -192.9982390220562820, -368.0189434323527280 ) ) ;
#28317=CARTESIAN_POINT ( 'NONE',  ( 791.1614460488616487, -83.26014174441466764, -373.5763878283158874 ) ) ;
#28319=CARTESIAN_POINT ( 'NONE',  ( 748.9653473494363425, -338.6346026584195101, -356.9462024416521331 ) ) ;
#28323=AXIS2_PLACEMENT_3D ( 'NONE', #43042, #14663, #8394 ) ;
#28325=CARTESIAN_POINT ( 'NONE',  ( 805.9055244015594326, -411.6237781080499758, -315.8990559732753240 ) ) ;
#28326=CARTESIAN_POINT ( 'NONE',  ( 772.4837098697144029, -431.3618753856918033, -374.5518280994205611 ) ) ;
#28331=CARTESIAN_POINT ( 'NONE',  ( 815.1787889125755555, -198.8965053807779384, -343.7953271457877804 ) ) ;
#28340=CARTESIAN_POINT ( 'NONE',  ( 796.9462024416508257, -60.45278447660215448, -308.9653473494370246 ) ) ;
#28342=AXIS2_PLACEMENT_3D ( 'NONE', #10793, #3641, #38983 ) ;
#28344=CARTESIAN_POINT ( 'NONE',  ( 814.4686193811664907, -459.2817908451519884, -346.2056067578752732 ) ) ;
#28345=ORIENTED_EDGE ( 'NONE', *, *, #33741, .T. ) ;
#28348=CARTESIAN_POINT ( 'NONE',  ( 800.2193346964447755, -306.9982390220558273, -355.1360043628815788 ) ) ;
#28352=CARTESIAN_POINT ( 'NONE',  ( 766.9102291470427417, -306.5545181178797520, -318.6633372737382501 ) ) ;
#28353=CARTESIAN_POINT ( 'NONE',  ( 765.0180583372156207, -240.9982390220561683, -360.0135310231089534 ) ) ;
#28354=CARTESIAN_POINT ( 'NONE',  ( 764.8639956371174549, -440.0891481129645513, -319.7806653035542581 ) ) ;
#28355=CARTESIAN_POINT ( 'NONE',  ( 755.0636971347428243, -124.2709662947837899, -341.7834795799807353 ) ) ;
#28357=EDGE_CURVE ( 'NONE', #43845, #19525, #28293, .T. ) ;
#28360=VECTOR ( 'NONE', #21342, 1000.000000000000000 ) ;
#28364=CARTESIAN_POINT ( 'NONE',  ( 745.1792804349281596, -38.19088175424422360, -343.7566961878542884 ) ) ;
#28365=DIRECTION ( 'NONE',  ( 0.000000000000000000, 0.000000000000000000, -1.000000000000000000 ) ) ;
#28370=CARTESIAN_POINT ( 'NONE',  ( 759.0159684113467620, -16.91815448151702839, -325.8855110935213020 ) ) ;
#28371=CARTESIAN_POINT ( 'NONE',  ( 755.2512626584698410, -103.5436935675111272, -315.2512626584710915 ) ) ;
#28373=DIRECTION ( 'NONE',  ( 0.000000000000000000, -0.000000000000000000, -1.000000000000000000 ) ) ;
#28376=CARTESIAN_POINT ( 'NONE',  ( 801.1904061080336987, -236.0891481129651766, -368.3070685750235498 ) ) ;
#28381=CARTESIAN_POINT ( 'NONE',  ( 795.6651683502461765, -298.7146871989593251, -371.3240766477733814 ) ) ;
#28384=CARTESIAN_POINT ( 'NONE',  ( 814.9108240113580450, -328.2709662947831362, -337.5031285880265273 ) ) ;
#28388=CARTESIAN_POINT ( 'NONE',  ( 800.0135310231082713, -398.0891481129647218, -325.0180583372163028 ) ) ;
#28392=CARTESIAN_POINT ( 'NONE',  ( 765.0180583372156207, -192.9982390220562820, -360.0135310231089534 ) ) ;
#28394=CARTESIAN_POINT ( 'NONE',  ( 811.6461892240364477, -76.71468719896012090, -324.1737431748509835 ) ) ;
#28400=CARTESIAN_POINT ( 'NONE',  ( 756.7813123517142913, -211.9874144716869750, -329.9779781133712504 ) ) ;
#28403=CARTESIAN_POINT ( 'NONE',  ( 781.2497674668890113, -36.35105083532390324, -375.3608509340180603 ) ) ;
#28406=CARTESIAN_POINT ( 'NONE',  ( 801.4587497624105481, -452.9681489794446634, -353.8271441104080282 ) ) ;
#28408=SHAPE_REPRESENTATION ( 'Treadle Extension Return Springs', ( #26858 ), #7704 ) ;
#28411=CARTESIAN_POINT ( 'NONE',  ( 757.7880784355613741, -354.0090635724250774, -312.4576283171834916 ) ) ;
#28415=CARTESIAN_POINT ( 'NONE',  ( 804.4086373105744769, -145.6454272087893287, -333.3843516231986541 ) ) ;
#28416=CARTESIAN_POINT ( 'NONE',  ( 759.7806653035534055, -150.9982390220563957, -324.8639956371180801 ) ) ;
#28417=CARTESIAN_POINT ( 'NONE',  ( 756.3353852180820240, -341.9073299311466485, -331.1735550268787733 ) ) ;
#28420=CARTESIAN_POINT ( 'NONE',  ( 779.9999999999992042, -452.9681489794448339, -329.9999999999999432 ) ) ;
#28427=CARTESIAN_POINT ( 'NONE',  ( 760.0363995740630116, -394.9181544815158418, -368.7758568127991907 ) ) ;
#28429=CARTESIAN_POINT ( 'NONE',  ( 782.5225473063383106, 1.729033705215812233, -375.2698199232970637 ) ) ;
#28434=CARTESIAN_POINT ( 'NONE',  ( 781.7834795799800531, -346.8164208402376971, -315.0636971347436202 ) ) ;
#28437=CARTESIAN_POINT ( 'NONE',  ( 796.9571628226829034, -215.4636090269709712, -321.2382568024804641 ) ) ;
#28438=VECTOR ( 'NONE', #7318, 1000.000000000000000 ) ;
#28442=CARTESIAN_POINT ( 'NONE',  ( 754.9967657858570647, -409.5436935675101608, -365.0032342141425943 ) ) ;
#28448=CARTESIAN_POINT ( 'NONE',  ( 805.0032342141412300, -61.54369356751124087, -314.9967657858571783 ) ) ;
#28449=CARTESIAN_POINT ( 'NONE',  ( 800.2193346964447755, -282.9982390220558841, -355.1360043628815788 ) ) ;
#28450=AXIS2_PLACEMENT_3D ( 'NONE', #8671, #1485, #22735 ) ;
#28454=CARTESIAN_POINT ( 'NONE',  ( 807.2620300519052989, -72.00906357242594424, -318.0141637701419768 ) ) ;
#28455=CARTESIAN_POINT ( 'NONE',  ( 756.7813123517142913, -67.98741447168742980, -329.9779781133712504 ) ) ;
#28458=CARTESIAN_POINT ( 'NONE',  ( 800.0135310231082713, 9.910851887033969021, -325.0180583372163028 ) ) ;
#28459=CARTESIAN_POINT ( 'NONE',  ( 802.7791456095903868, -100.7146871989600356, -329.0155153010375102 ) ) ;
#28461=CARTESIAN_POINT ( 'NONE',  ( 804.6798772138708955, -111.7255117493293000, -334.6312213355107019 ) ) ;
#28462=CARTESIAN_POINT ( 'NONE',  ( 759.2295555964440155, -400.1692326535045936, -353.9708237608231229 ) ) ;
#28466=CARTESIAN_POINT ( 'NONE',  ( 801.9858362298568863, -411.0783235625954717, -312.7379699480935642 ) ) ;
#28473=CARTESIAN_POINT ( 'NONE',  ( 801.1904061080336987, -236.0891481129651766, -368.3070685750235498 ) ) ;
#28478=CARTESIAN_POINT ( 'NONE',  ( 804.9363028652555840, -256.2709662947834204, -338.2165204200192079 ) ) ;
#28480=CARTESIAN_POINT ( 'NONE',  ( 759.9864689768902508, -362.0891481129648923, -354.9819416627836404 ) ) ;
#28481=CARTESIAN_POINT ( 'NONE',  ( 755.3201227861273992, -3.725511749329622813, -345.3687786644892981 ) ) ;
#28489=CARTESIAN_POINT ( 'NONE',  ( 756.5762568750052424, -27.18005720387500901, -348.7366044899774238 ) ) ;
#28493=CARTESIAN_POINT ( 'NONE',  ( 807.2620300519052989, -264.0090635724253616, -318.0141637701419768 ) ) ;
#28496=CARTESIAN_POINT ( 'NONE',  ( 764.8639956371174549, -248.0891481129651481, -319.7806653035542013 ) ) ;
#28497=CARTESIAN_POINT ( 'NONE',  ( 803.8651313633788504, -389.2601417444136018, -332.4468031744301015 ) ) ;
#28499=CARTESIAN_POINT ( 'NONE',  ( 802.9823548866075953, -121.0999726633348956, -330.0799878456151077 ) ) ;
#28502=CARTESIAN_POINT ( 'NONE',  ( 814.8230680027162407, 18.19440371013048008, -333.7305795820267917 ) ) ;
#28503=CARTESIAN_POINT ( 'NONE',  ( 763.0537975583476964, -312.4527844766013800, -371.0346526505628617 ) ) ;
#28508=CARTESIAN_POINT ( 'NONE',  ( 754.0944755984390895, -207.6237781080506295, -364.1009440267246760 ) ) ;
#28510=CARTESIAN_POINT ( 'NONE',  ( 808.3070685750230950, -426.9982390220554862, -361.1904061080339261 ) ) ;
#28514=CIRCLE ( 'NONE', #32978, 30.00000000000008171 ) ;
#28517=CARTESIAN_POINT ( 'NONE',  ( 755.8398074228967971, 4.558040073766884248, -333.4516893846970333 ) ) ;
#28524=CARTESIAN_POINT ( 'NONE',  ( 775.9200461376533440, -311.8055962898685038, -315.3028492785443291 ) ) ;
#28526=CARTESIAN_POINT ( 'NONE',  ( 746.0683387631852383, -307.4419599262320730, -331.3260364891676204 ) ) ;
#28529=ORIENTED_EDGE ( 'NONE', *, *, #21559, .F. ) ;
#28531=CARTESIAN_POINT ( 'NONE',  ( 798.7617431975189675, -75.62377810805104161, -323.0428371773161871 ) ) ;
#28532=CARTESIAN_POINT ( 'NONE',  ( 785.3687786644884454, -155.3618753856927128, -315.3201227861279676 ) ) ;
#28533=CARTESIAN_POINT ( 'NONE',  ( 802.1676090361156639, -206.6346026584198512, -327.8955696845344505 ) ) ;
#28535=CARTESIAN_POINT ( 'NONE',  ( 759.0252816721024374, -144.9982390220564525, -368.0189434323527280 ) ) ;
#28537=CARTESIAN_POINT ( 'NONE',  ( 756.5762568750052424, -147.1800572038746395, -348.7366044899774238 ) ) ;
#28540=CARTESIAN_POINT ( 'NONE',  ( 759.0159684113467620, -400.9181544815159555, -325.8855110935213020 ) ) ;
#28543=CIRCLE ( 'NONE', #16010, 10.00000000000000888 ) ;
#28548=CARTESIAN_POINT ( 'NONE',  ( 755.8894580844503253, -399.8272453906067767, -332.3691319403863531 ) ) ;
#28551=CARTESIAN_POINT ( 'NONE',  ( 762.1177392798416577, -162.5545181178802352, -309.8865473780659272 ) ) ;
#28556=CARTESIAN_POINT ( 'NONE',  ( 757.2208543904082489, -304.7146871989594388, -350.9844846989624330 ) ) ;
#28558=CARTESIAN_POINT ( 'NONE',  ( 805.6418435158337843, -173.4636090269710849, -363.8556311672236916 ) ) ;
#28564=CARTESIAN_POINT ( 'NONE',  ( 748.9653473494365699, -194.6346026584199080, -356.9462024416520762 ) ) ;
#28565=EDGE_CURVE ( 'NONE', #911, #38644, #14795, .T. ) ;
#28567=CARTESIAN_POINT ( 'NONE',  ( 785.3687786644884454, 12.63812461430668321, -315.3201227861279676 ) ) ;
#28569=CARTESIAN_POINT ( 'NONE',  ( 800.1688906516307043, -82.16923265350558836, -369.0717654672308186 ) ) ;
#28571=CARTESIAN_POINT ( 'NONE',  ( 796.7737145352015204, -356.6346026584193964, -370.7187646348536987 ) ) ;
#28577=CARTESIAN_POINT ( 'NONE',  ( 744.8212110874229666, -402.8965053807773415, -336.2046728542121627 ) ) ;
#28579=CARTESIAN_POINT ( 'NONE',  ( 751.6929314249748586, -414.9982390220555430, -318.8095938919659034 ) ) ;
#28584=CARTESIAN_POINT ( 'NONE',  ( 793.4146539503750546, -193.9874144716870319, -307.6481478633938877 ) ) ;
#28591=CARTESIAN_POINT ( 'NONE',  ( 772.5602148656447525, -33.72551174932952733, -305.7998596910095443 ) ) ;
#28595=CARTESIAN_POINT ( 'NONE',  ( 760.0363995740630116, -442.9181544815157849, -368.7758568127991907 ) ) ;
#28597=PRODUCT_CONTEXT ( 'NONE', #16041, 'mechanical' ) ;
#28599=CARTESIAN_POINT ( 'NONE',  ( 764.8639956371174549, -296.0891481129650629, -319.7806653035542013 ) ) ;
#28603=CARTESIAN_POINT ( 'NONE',  ( 800.9840315886518738, -292.9181544815162397, -354.1144889064786412 ) ) ;
#28604=CARTESIAN_POINT ( 'NONE',  ( 771.1735550268778070, -273.1800572038742985, -316.3353852180827630 ) ) ;
#28605=CARTESIAN_POINT ( 'NONE',  ( 797.6776695296629214, -451.5436935675099903, -357.6776695296636603 ) ) ;
#28606=CARTESIAN_POINT ( 'NONE',  ( 788.7366044899766848, -107.9073299311474727, -316.5762568750059813 ) ) ;
#28608=ORIENTED_EDGE ( 'NONE', *, *, #2975, .T. ) ;
#28612=CARTESIAN_POINT ( 'NONE',  ( 776.2046728542105711, -92.19088175424406018, -304.8212110874238761 ) ) ;
#28619=CARTESIAN_POINT ( 'NONE',  ( 769.9779781133707957, -43.09997266333511590, -316.7813123517150871 ) ) ;
#28620=CARTESIAN_POINT ( 'NONE',  ( 812.7932403749906598, -111.1800572038747532, -327.7687537140311633 ) ) ;
#28626=CARTESIAN_POINT ( 'NONE',  ( 777.4774526936600978, -226.2709662947834204, -304.7301800767027657 ) ) ;
#28631=CARTESIAN_POINT ( 'NONE',  ( 813.2346286133761168, -293.2601417444139429, -328.9521613784389160 ) ) ;
#28633=CARTESIAN_POINT ( 'NONE',  ( 745.7998596910086917, -317.3618753856922581, -332.5602148656461168 ) ) ;
#28636=CARTESIAN_POINT ( 'NONE',  ( 792.1044303154645831, -372.4527844766010958, -317.8323909638837677 ) ) ;
#28638=CARTESIAN_POINT ( 'NONE',  ( 793.4146539503750546, -97.98741447168734453, -307.6481478633938877 ) ) ;
#28644=CARTESIAN_POINT ( 'NONE',  ( 765.8855110935204493, -190.1692326535052189, -319.0159684113471599 ) ) ;
#28646=CARTESIAN_POINT ( 'NONE',  ( 751.2241431872005251, -16.16923265350578021, -359.9636004259367610 ) ) ;
#28648=CARTESIAN_POINT ( 'NONE',  ( 809.5171784329539832, -452.9681489794445497, -335.1922280983832252 ) ) ;
#28652=CARTESIAN_POINT ( 'NONE',  ( 786.2694204179717872, -357.2817908451523294, -305.1769319972829067 ) ) ;
#28656=CARTESIAN_POINT ( 'NONE',  ( 799.2566176426618085, -192.0090635724255606, -324.0069404352559559 ) ) ;
#28657=CARTESIAN_POINT ( 'NONE',  ( 800.2193346964447755, -162.9982390220563673, -355.1360043628815788 ) ) ;
#28658=CARTESIAN_POINT ( 'NONE',  ( 755.0636971347428243, -364.2709662947830793, -341.7834795799807353 ) ) ;
#28669=CARTESIAN_POINT ( 'NONE',  ( 797.8822607201568644, -414.5545181178795247, -370.1134526219340160 ) ) ;
#28670=CARTESIAN_POINT ( 'NONE',  ( 804.7487373415286811, 4.456306432488530866, -364.7487373415288516 ) ) ;
#28673=CARTESIAN_POINT ( 'NONE',  ( 803.6646147819161570, -353.9073299311467053, -348.8264449731210561 ) ) ;
#28675=CARTESIAN_POINT ( 'NONE',  ( 776.9254006560222479, -212.1908817542436623, -314.8983024940802125 ) ) ;
#28681=CARTESIAN_POINT ( 'NONE',  ( 804.7487373415286811, -403.5436935675101608, -364.7487373415288516 ) ) ;
#28687=CARTESIAN_POINT ( 'NONE',  ( 811.0346526505616112, -38.63460265842041252, -323.0537975583477532 ) ) ;
#28688=CARTESIAN_POINT ( 'NONE',  ( 755.0636971347428243, -292.2709662947831930, -341.7834795799807353 ) ) ;
#28692=CARTESIAN_POINT ( 'NONE',  ( 776.2046728542105711, -68.19088175424413123, -304.8212110874238761 ) ) ;
#28693=CARTESIAN_POINT ( 'NONE',  ( 755.0488828828309806, -89.80559628986918597, -344.1219089521771934 ) ) ;
#28697=CARTESIAN_POINT ( 'NONE',  ( 791.9812246680005501, 3.365397341579444479, -361.9419747391813189 ) ) ;
#28699=CARTESIAN_POINT ( 'NONE',  ( 804.9363028652555840, -88.27096629478390355, -338.2165204200192079 ) ) ;
#28700=CARTESIAN_POINT ( 'NONE',  ( 754.8983024940795303, -402.8965053807773415, -336.9254006560228163 ) ) ;
#28703=CARTESIAN_POINT ( 'NONE',  ( 758.0141637701419768, -399.0783235625955285, -367.2620300519063790 ) ) ;
#28709=CARTESIAN_POINT ( 'NONE',  ( 772.4837098697144029, -263.3618753856924855, -374.5518280994205611 ) ) ;
#28714=CARTESIAN_POINT ( 'NONE',  ( 802.5472867521000353, -76.37269993606228979, -350.8726784830461156 ) ) ;
#28716=CARTESIAN_POINT ( 'NONE',  ( 765.0180583372156207, -240.9982390220561683, -360.0135310231089534 ) ) ;
#28719=CARTESIAN_POINT ( 'NONE',  ( 768.0187753319979720, -344.6346026584195101, -318.0580252608186242 ) ) ;
#28720=CARTESIAN_POINT ( 'NONE',  ( 803.4237431249931660, -39.18005720387496638, -331.2633955100225194 ) ) ;
#28726=CARTESIAN_POINT ( 'NONE',  ( 755.5713283507202505, -29.36187538569318178, -334.6858677611754729 ) ) ;
#28730=CARTESIAN_POINT ( 'NONE',  ( 786.2694204179717872, -261.2817908451526705, -305.1769319972829067 ) ) ;
#28733=CARTESIAN_POINT ( 'NONE',  ( 756.3353852180819104, -245.9073299311469896, -331.1735550268788302 ) ) ;
#28734=CARTESIAN_POINT ( 'NONE',  ( 769.0155153010367712, -106.3726999360621903, -362.7791456095907279 ) ) ;
#28738=CARTESIAN_POINT ( 'NONE',  ( 814.9108240113580450, -328.2709662947831362, -337.5031285880265273 ) ) ;
#28742=CARTESIAN_POINT ( 'NONE',  ( 746.0683387631852383, -211.4419599262324709, -331.3260364891676204 ) ) ;
#28744=CARTESIAN_POINT ( 'NONE',  ( 751.9810565676468741, -434.0891481129646081, -360.9747183278973921 ) ) ;
#28749=CARTESIAN_POINT ( 'NONE',  ( 764.0069404352550464, 8.921676437403235127, -359.2566176426627180 ) ) ;
#28756=CARTESIAN_POINT ( 'NONE',  ( 803.8651313633788504, -293.2601417444139429, -332.4468031744301015 ) ) ;
#28758=CARTESIAN_POINT ( 'NONE',  ( 771.2368401574024119, -301.4419599262320730, -374.2805881961240857 ) ) ;
#28763=CARTESIAN_POINT ( 'NONE',  ( 786.6156483768007774, -73.44195992623286884, -315.5913626894246136 ) ) ;
#28764=CARTESIAN_POINT ( 'NONE',  ( 759.7806653035534055, -174.9982390220563673, -324.8639956371180801 ) ) ;
#28765=CARTESIAN_POINT ( 'NONE',  ( 767.8955696845333705, -192.4527844766016926, -362.1676090361162323 ) ) ;
#28767=CARTESIAN_POINT ( 'NONE',  ( 755.2512626584698410, -151.5436935675109851, -315.2512626584710915 ) ) ;
#28769=CARTESIAN_POINT ( 'NONE',  ( 785.3687786644885591, -155.3618753856927697, -315.3201227861280813 ) ) ;
#28771=CARTESIAN_POINT ( 'NONE',  ( 759.0159684113467620, -376.9181544815159555, -325.8855110935213020 ) ) ;
#28779=CARTESIAN_POINT ( 'NONE',  ( 763.0428371773158460, -395.4636090269705164, -358.7617431975195359 ) ) ;
#28781=CARTESIAN_POINT ( 'NONE',  ( 757.7880784355613741, -186.0090635724255890, -312.4576283171834916 ) ) ;
#28785=CARTESIAN_POINT ( 'NONE',  ( 803.2186876482843445, -343.9874144716865771, -350.0220218866286928 ) ) ;
#28787=CARTESIAN_POINT ( 'NONE',  ( 812.3518521366052028, -193.0999726633346256, -326.5853460496235243 ) ) ;
#28792=CARTESIAN_POINT ( 'NONE',  ( 782.5225473063383106, -214.2709662947834772, -375.2698199232970637 ) ) ;
#28793=DIRECTION ( 'NONE',  ( 0.000000000000000000, -0.000000000000000000, -1.000000000000000000 ) ) ;
#28794=CARTESIAN_POINT ( 'NONE',  ( 758.0580252608178853, -30.45278447660226817, -328.0187753319985404 ) ) ;
#28796=CARTESIAN_POINT ( 'NONE',  ( 813.2346286133761168, -101.2601417444146250, -328.9521613784389160 ) ) ;
#28798=CARTESIAN_POINT ( 'NONE',  ( 813.1304606946830518, -329.9073299311467053, -352.3570229623690580 ) ) ;
#28803=CARTESIAN_POINT ( 'NONE',  ( 813.9316612368132837, -415.4419599262318457, -348.6739635108323228 ) ) ;
#28804=CARTESIAN_POINT ( 'NONE',  ( 746.8695393053150156, -413.9073299311465348, -327.6429770376306010 ) ) ;
#28808=CARTESIAN_POINT ( 'NONE',  ( 778.2165204200184689, -118.8164208402383508, -364.9363028652563230 ) ) ;
#28810=CARTESIAN_POINT ( 'NONE',  ( 807.5423716828161105, -177.0783235625961538, -362.2119215644372048 ) ) ;
#28815=CARTESIAN_POINT ( 'NONE',  ( 751.9810565676468741, -50.08914811296584446, -360.9747183278973921 ) ) ;
#28818=CARTESIAN_POINT ( 'NONE',  ( 796.2681130854250569, -462.7578698805381237, -371.0719813302654870 ) ) ;
#28823=CARTESIAN_POINT ( 'NONE',  ( 795.1360043628807261, -284.0891481129650629, -360.2193346964456282 ) ) ;
#28827=CARTESIAN_POINT ( 'NONE',  ( 757.0176451133909268, -301.0999726633342561, -349.9200121543848354 ) ) ;
#28828=CARTESIAN_POINT ( 'NONE',  ( 795.1360043628807261, -284.0891481129650629, -360.2193346964456282 ) ) ;
#28830=CARTESIAN_POINT ( 'NONE',  ( 785.3687786644884454, -107.3618753856928976, -315.3201227861279676 ) ) ;
#28836=CARTESIAN_POINT ( 'NONE',  ( 807.2620300519052989, -96.00906357242585898, -318.0141637701419768 ) ) ;
#28842=CARTESIAN_POINT ( 'NONE',  ( 783.0745993439762742, -32.19088175424425913, -365.1016975059196739 ) ) ;
#28843=CARTESIAN_POINT ( 'NONE',  ( 792.3570229623691148, -117.1800572038747106, -373.1304606946836770 ) ) ;
#28847=CARTESIAN_POINT ( 'NONE',  ( 804.7487373415286811, -235.5436935675107293, -364.7487373415288516 ) ) ;
#28851=CARTESIAN_POINT ( 'NONE',  ( 795.6651683502461765, -322.7146871989593819, -371.3240766477733814 ) ) ;
#28853=CARTESIAN_POINT ( 'NONE',  ( 814.5518280994195948, -327.7255117493285184, -332.4837098697145734 ) ) ;
#28854=DIRECTION ( 'NONE',  ( 0.000000000000000000, 0.000000000000000000, -1.000000000000000000 ) ) ;
#28857=CARTESIAN_POINT ( 'NONE',  ( 756.5762568750052424, -411.1800572038738437, -348.7366044899774238 ) ) ;
#28859=CARTESIAN_POINT ( 'NONE',  ( 756.3353852180819104, -197.9073299311472169, -331.1735550268788302 ) ) ;
#28860=CARTESIAN_POINT ( 'NONE',  ( 758.0141637701419768, -87.07832356259646645, -367.2620300519063790 ) ) ;
#28864=CARTESIAN_POINT ( 'NONE',  ( 775.9200461376533440, -239.8055962898687028, -315.3028492785443291 ) ) ;
#28867=CARTESIAN_POINT ( 'NONE',  ( 745.1769319972822814, -41.80559628986934229, -346.2694204179732083 ) ) ;
#28869=DIRECTION ( 'NONE',  ( 0.000000000000000000, -1.000000000000000000, 0.000000000000000000 ) ) ;
#28873=CARTESIAN_POINT ( 'NONE',  ( 795.8262568251477660, -334.3726999360615082, -308.3538107759623585 ) ) ;
#28877=CARTESIAN_POINT ( 'NONE',  ( 769.0155153010367712, -178.3726999360619629, -362.7791456095907279 ) ) ;
#28878=CARTESIAN_POINT ( 'NONE',  ( 768.0187753319979720, -176.6346026584199933, -318.0580252608186242 ) ) ;
#28879=CARTESIAN_POINT ( 'NONE',  ( 771.2633955100217236, -359.9073299311467053, -363.4237431249939618 ) ) ;
#28881=ORIENTED_EDGE ( 'NONE', *, *, #22448, .T. ) ;
#28890=CARTESIAN_POINT ( 'NONE',  ( 791.0478386215596629, -405.8272453906067199, -306.7653713866226326 ) ) ;
#28891=CARTESIAN_POINT ( 'NONE',  ( 755.2512626584698410, 16.45630643248848912, -315.2512626584710915 ) ) ;
#28894=CARTESIAN_POINT ( 'NONE',  ( 756.3353852180819104, -365.9073299311465917, -331.1735550268788302 ) ) ;
#28899=CARTESIAN_POINT ( 'NONE',  ( 763.8424801807145741, -258.0090635724253616, -320.5453621957614700 ) ) ;
#28909=CARTESIAN_POINT ( 'NONE',  ( 803.4237431249931660, -327.1800572038741279, -331.2633955100225194 ) ) ;
#28914=CARTESIAN_POINT ( 'NONE',  ( 807.2620300519052989, -48.00906357242602951, -318.0141637701419768 ) ) ;
#28915=CARTESIAN_POINT ( 'NONE',  ( 776.9566956441375396, -84.89650538077830788, -364.8461984189686405 ) ) ;
#28921=CARTESIAN_POINT ( 'NONE',  ( 785.3141322388236176, 2.274488250670355871, -364.4286716492789537 ) ) ;
#28922=CARTESIAN_POINT ( 'NONE',  ( 755.0488828828309806, -113.8055962898691149, -344.1219089521771934 ) ) ;
#28924=CARTESIAN_POINT ( 'NONE',  ( 801.9419747391806368, -90.45278447660209054, -351.9812246680014027 ) ) ;
#28926=CARTESIAN_POINT ( 'NONE',  ( 760.5453621957607311, -405.0783235625954148, -323.8424801807151425 ) ) ;
#28938=CARTESIAN_POINT ( 'NONE',  ( 804.1105419155481968, -75.82724539060775726, -347.6308680596136469 ) ) ;
#28940=CARTESIAN_POINT ( 'NONE',  ( 791.9812246680005501, -236.6346026584198228, -361.9419747391813189 ) ) ;
#28942=CARTESIAN_POINT ( 'NONE',  ( 781.8018195045266339, -382.2709662947828519, -365.1927285166406705 ) ) ;
#28943=CARTESIAN_POINT ( 'NONE',  ( 788.7366044899766848, -35.90732993114770011, -316.5762568750059813 ) ) ;
#28946=CARTESIAN_POINT ( 'NONE',  ( 771.1735550268778070, -9.180057203875058747, -316.3353852180827630 ) ) ;
#28949=CARTESIAN_POINT ( 'NONE',  ( 747.6481478633932056, -325.0999726633342561, -353.4146539503763620 ) ) ;
#28954=CARTESIAN_POINT ( 'NONE',  ( 759.7806653035534055, -270.9982390220561115, -324.8639956371180801 ) ) ;
#28957=CARTESIAN_POINT ( 'NONE',  ( 772.4468031744293057, -153.8272453906075157, -363.8651313633793620 ) ) ;
#28958=EDGE_CURVE ( 'NONE', #21104, #39743, #16835, .T. ) ;
#28961=CARTESIAN_POINT ( 'NONE',  ( 763.0537975583476964, -336.4527844766012663, -371.0346526505628617 ) ) ;
#28962=CARTESIAN_POINT ( 'NONE',  ( 759.9999999999992042, 205.0000000000000568, -319.9999999999999432 ) ) ;
#28965=CARTESIAN_POINT ( 'NONE',  ( 749.8865473780648472, -212.5328690171415076, -322.1177392798429082 ) ) ;
#28967=CARTESIAN_POINT ( 'NONE',  ( 792.2269492836462632, -443.1233509495419298, -372.8191558162650949 ) ) ;
#28974=CARTESIAN_POINT ( 'NONE',  ( 760.5453621957607311, 2.921676437403253779, -323.8424801807151425 ) ) ;
#28982=CARTESIAN_POINT ( 'NONE',  ( 794.1144889064781864, -298.1692326535049347, -360.9840315886528401 ) ) ;
#28983=CARTESIAN_POINT ( 'NONE',  ( 748.3538107759620743, -280.7146871989594956, -355.8262568251490165 ) ) ;
#28988=CARTESIAN_POINT ( 'NONE',  ( 755.0488828828309806, -65.80559628986925702, -344.1219089521771934 ) ) ;
#28990=ADVANCED_FACE ( 'NONE', ( #6872 ), #13361, .T. ) ;
#28991=CARTESIAN_POINT ( 'NONE',  ( 796.7737145352015204, -164.6346026584200217, -370.7187646348536987 ) ) ;
#28993=CARTESIAN_POINT ( 'NONE',  ( 785.3141322388236176, -141.7255117493291721, -364.4286716492789537 ) ) ;
#28995=CARTESIAN_POINT ( 'NONE',  ( 783.0745993439762742, -416.1908817542430938, -365.1016975059196739 ) ) ;
#28998=DIRECTION ( 'NONE',  ( 0.000000000000000000, -1.000000000000000000, 0.000000000000000000 ) ) ;
#29002=CARTESIAN_POINT ( 'NONE',  ( 775.8780910478218402, -393.2817908451522726, -364.9511171171680530 ) ) ;
#29005=CARTESIAN_POINT ( 'NONE',  ( 757.7880784355613741, -210.0090635724255321, -312.4576283171834916 ) ) ;
#29010=CARTESIAN_POINT ( 'NONE',  ( 759.2295555964440155, -328.1692326535048210, -353.9708237608231229 ) ) ;
#29012=CARTESIAN_POINT ( 'NONE',  ( 745.7194118038753459, -181.6454272087892434, -348.7631598425976449 ) ) ;
#29016=CARTESIAN_POINT ( 'NONE',  ( 749.2812353651451076, -222.4527844766016642, -323.2262854647983090 ) ) ;
#29018=CARTESIAN_POINT ( 'NONE',  ( 797.8594530101008786, -13.54369356751140785, -322.1405469898980982 ) ) ;
#29021=CARTESIAN_POINT ( 'NONE',  ( 813.9316612368132837, -103.4419599262327836, -348.6739635108323228 ) ) ;
#29023=CARTESIAN_POINT ( 'NONE',  ( 811.0346526505616112, -350.6346026584192828, -323.0537975583477532 ) ) ;
#29024=DIRECTION ( 'NONE',  ( -0.000000000000000000, -0.000000000000000000, 1.000000000000000000 ) ) ;
#29028=CARTESIAN_POINT ( 'NONE',  ( 786.2056067578752163, -419.8055962898681059, -374.4686193811670023 ) ) ;
#29029=CARTESIAN_POINT ( 'NONE',  ( 810.7187646348534145, -426.4527844766010389, -356.7737145352016341 ) ) ;
#29033=CARTESIAN_POINT ( 'NONE',  ( 760.5453621957607311, -189.0783235625961822, -323.8424801807151425 ) ) ;
#29036=CARTESIAN_POINT ( 'NONE',  ( 813.9316612368132837, -199.4419599262324709, -348.6739635108323228 ) ) ;
#29037=( NAMED_UNIT ( * ) PLANE_ANGLE_UNIT ( ) SI_UNIT ( $, .RADIAN. ) );
#29041=ORIENTED_EDGE ( 'NONE', *, *, #39154, .T. ) ;
#29043=CARTESIAN_POINT ( 'NONE',  ( 762.1405469898971887, -145.5436935675109851, -357.8594530101015607 ) ) ;
#29045=CARTESIAN_POINT ( 'NONE',  ( 811.0346526505616112, -38.63460265842041252, -323.0537975583477532 ) ) ;
#29047=CARTESIAN_POINT ( 'NONE',  ( 786.2694204179717872, -429.2817908451521021, -305.1769319972829067 ) ) ;
#29049=CARTESIAN_POINT ( 'NONE',  ( 802.9823548866075953, -337.0999726633342561, -330.0799878456151077 ) ) ;
#29053=CARTESIAN_POINT ( 'NONE',  ( 778.1981804954714335, -298.2709662947830793, -314.8072714833589885 ) ) ;
#29057=CARTESIAN_POINT ( 'NONE',  ( 783.0745993439762742, -296.1908817542434917, -365.1016975059196739 ) ) ;
#29058=CARTESIAN_POINT ( 'NONE',  ( 797.6776695296629214, -283.5436935675105019, -357.6776695296636603 ) ) ;
#29060=CARTESIAN_POINT ( 'NONE',  ( 774.6858677611749044, -105.7255117493293000, -315.5713283507209894 ) ) ;
#29066=CARTESIAN_POINT ( 'NONE',  ( 783.7953271457878373, -80.19088175424411702, -375.1787889125761239 ) ) ;
#29072=AXIS2_PLACEMENT_3D ( 'NONE', #21625, #35708, #28793 ) ;
#29074=CARTESIAN_POINT ( 'NONE',  ( 745.0891759886404770, -100.2709662947838609, -342.4968714119734159 ) ) ;
#29078=CARTESIAN_POINT ( 'NONE',  ( 745.0891759886404770, -244.2709662947834204, -342.4968714119734159 ) ) ;
#29081=CARTESIAN_POINT ( 'NONE',  ( 756.1443688327750579, -309.6237781080502600, -314.3581564841659315 ) ) ;
#29084=CARTESIAN_POINT ( 'NONE',  ( 804.7487373415286811, -307.5436935675104451, -364.7487373415288516 ) ) ;
#29088=CARTESIAN_POINT ( 'NONE',  ( 788.7366044899766848, -419.9073299311465348, -316.5762568750059813 ) ) ;
#29089=CARTESIAN_POINT ( 'NONE',  ( 755.5713283507202505, -221.3618753856925707, -334.6858677611754729 ) ) ;
#29090=EDGE_CURVE ( 'NONE', #16032, #17925, #40156, .T. ) ;
#29091=CARTESIAN_POINT ( 'NONE',  ( 756.1443688327750579, -93.62377810805098477, -314.3581564841659315 ) ) ;
#29096=CARTESIAN_POINT ( 'NONE',  ( 795.9930595647434757, -243.0783235625959833, -320.7433823573372820 ) ) ;
#29098=CIRCLE ( 'NONE', #7081, 4.999999999999984901 ) ;
#29099=CARTESIAN_POINT ( 'NONE',  ( 761.9338519418445230, -62.53286901714199786, -370.4231160770881957 ) ) ;
#29101=CARTESIAN_POINT ( 'NONE',  ( 809.6099558218720631, -452.9681489794449476, -335.1781210895659342 ) ) ;
#29104=CARTESIAN_POINT ( 'NONE',  ( 766.4474001241216001, -331.0999726633342561, -307.3154664389482491 ) ) ;
#29107=CARTESIAN_POINT ( 'NONE',  ( 779.4763451958990572, -176.7363362996983369, -365.0264073115438919 ) ) ;
#29108=CARTESIAN_POINT ( 'NONE',  ( 805.1927285166397041, -184.8164208402380950, -341.8018195045277707 ) ) ;
#29109=CARTESIAN_POINT ( 'NONE',  ( 800.2193346964446619, -378.9982390220557136, -355.1360043628816925 ) ) ;
#29116=DIRECTION ( 'NONE',  ( 1.000000000000000000, 0.000000000000000000, 0.000000000000000000 ) ) ;
#29117=VECTOR ( 'NONE', #29024, 1000.000000000000000 ) ;
#29121=CARTESIAN_POINT ( 'NONE',  ( 786.2694204179717872, -405.2817908451522158, -305.1769319972829067 ) ) ;
#29122=CARTESIAN_POINT ( 'NONE',  ( 800.9747183278959710, -12.99823902205686821, -311.9810565676471583 ) ) ;
#29125=CARTESIAN_POINT ( 'NONE',  ( 802.1676090361156639, -374.6346026584192828, -327.8955696845344505 ) ) ;
#29127=CARTESIAN_POINT ( 'NONE',  ( 779.4763451958990572, -248.7363362996981380, -365.0264073115438919 ) ) ;
#29139=CARTESIAN_POINT ( 'NONE',  ( 774.6858677611749044, -321.7255117493286320, -315.5713283507209894 ) ) ;
#29143=CARTESIAN_POINT ( 'NONE',  ( 771.3260364891663130, -67.64542720878958448, -306.0683387631859773 ) ) ;
#29144=CARTESIAN_POINT ( 'NONE',  ( 801.3366627262608972, -104.5328690171418913, -353.0897708529566899 ) ) ;
#29148=CARTESIAN_POINT ( 'NONE',  ( 791.9812246680005501, -44.63460265842040542, -361.9419747391813189 ) ) ;
#29149=CARTESIAN_POINT ( 'NONE',  ( 802.7791456095903868, -148.7146871989598935, -329.0155153010375102 ) ) ;
#29151=CARTESIAN_POINT ( 'NONE',  ( 767.8955696845333705, -96.45278447660203369, -362.1676090361162323 ) ) ;
#29153=CARTESIAN_POINT ( 'NONE',  ( 801.3366627262608972, -416.5328690171409107, -353.0897708529566899 ) ) ;
#29164=CARTESIAN_POINT ( 'NONE',  ( 793.9708237608222134, -70.91815448151683654, -319.2295555964448681 ) ) ;
#29166=CARTESIAN_POINT ( 'NONE',  ( 768.0187753319979720, -272.6346026584196807, -318.0580252608186242 ) ) ;
#29169=CARTESIAN_POINT ( 'NONE',  ( 801.9419747391806368, -402.4527844766010389, -351.9812246680014027 ) ) ;
#29170=CARTESIAN_POINT ( 'NONE',  ( 794.9819416627830151, -60.99823902205671544, -319.9864689768909898 ) ) ;
#29175=CARTESIAN_POINT ( 'NONE',  ( 746.4236121716829757, -15.82724539060794200, -328.8385539511384650 ) ) ;
#29176=CARTESIAN_POINT ( 'NONE',  ( 779.9999999999992042, 16.45630643248849267, -350.0000000000000000 ) ) ;
#29178=CARTESIAN_POINT ( 'NONE',  ( 814.2805881961230625, -313.6454272087888171, -331.2368401574024119 ) ) ;
#29183=CARTESIAN_POINT ( 'NONE',  ( 774.6858677611749044, -273.7255117493288026, -315.5713283507209894 ) ) ;
#29185=CARTESIAN_POINT ( 'NONE',  ( 802.9823548866075953, -145.0999726633347677, -330.0799878456151077 ) ) ;
#29191=CARTESIAN_POINT ( 'NONE',  ( 767.7687537140311633, -335.9073299311468190, -372.7932403749916830 ) ) ;
#29195=CARTESIAN_POINT ( 'NONE',  ( 781.2497674668890113, -228.3510508353232922, -375.3608509340180603 ) ) ;
#29197=CARTESIAN_POINT ( 'NONE',  ( 754.9967657858570647, -1.543693567511449150, -365.0032342141425374 ) ) ;
#29205=CARTESIAN_POINT ( 'NONE',  ( 786.6156483768007774, -25.44195992623301450, -315.5913626894246136 ) ) ;
#29212=CARTESIAN_POINT ( 'NONE',  ( 756.1348686366196716, -281.2601417444139997, -347.5531968255698416 ) ) ;
#29215=CARTESIAN_POINT ( 'NONE',  ( 812.6845335610512393, -319.9874144716866340, -353.5525998758768651 ) ) ;
#29221=VECTOR ( 'NONE', #14440, 1000.000000000000000 ) ;
#29223=CARTESIAN_POINT ( 'NONE',  ( 756.7813123517142913, -91.98741447168737295, -329.9779781133712504 ) ) ;
#29226=AXIS2_PLACEMENT_3D ( 'NONE', #14465, #28998, #18162 ) ;
#29227=CARTESIAN_POINT ( 'NONE',  ( 814.2001403089898304, -185.3618753856926844, -347.4397851343538264 ) ) ;
#29230=CARTESIAN_POINT ( 'NONE',  ( 803.6646147819162707, -137.9073299311473875, -348.8264449731211130 ) ) ;
#29231=VERTEX_POINT ( 'NONE', #4594 ) ;
#29232=CARTESIAN_POINT ( 'NONE',  ( 802.9823548866075953, -409.0999726633340288, -330.0799878456151077 ) ) ;
#29236=CARTESIAN_POINT ( 'NONE',  ( 779.9999999999992042, 126.4563064324884465, -309.9999999999998863 ) ) ;
#29239=CARTESIAN_POINT ( 'NONE',  ( 799.2566176426618085, -408.0090635724249069, -324.0069404352559559 ) ) ;
#29241=CARTESIAN_POINT ( 'NONE',  ( 766.4474001241216001, -187.0999726633346825, -307.3154664389482491 ) ) ;
#29247=CARTESIAN_POINT ( 'NONE',  ( 779.4709603349208464, -336.3510508353228943, -314.7162404726379918 ) ) ;
#29249=CARTESIAN_POINT ( 'NONE',  ( 749.5768839229115201, -180.5545181178801499, -358.0661480581553064 ) ) ;
#29255=CARTESIAN_POINT ( 'NONE',  ( 758.8095938919644823, -248.0891481129651766, -311.6929314249762797 ) ) ;
#29257=CARTESIAN_POINT ( 'NONE',  ( 762.1405469898971887, -1.543693567511449150, -357.8594530101015607 ) ) ;
#29259=CARTESIAN_POINT ( 'NONE',  ( 751.2241431872005251, -136.1692326535053894, -359.9636004259367610 ) ) ;
#29261=CARTESIAN_POINT ( 'NONE',  ( 745.0891759886404770, -364.2709662947830793, -342.4968714119734159 ) ) ;
#29267=CARTESIAN_POINT ( 'NONE',  ( 795.6651683502461765, -418.7146871989590409, -371.3240766477733814 ) ) ;
#29268=B_SPLINE_CURVE_WITH_KNOTS ( 'NONE', 3,
 ( #6201, #13154, #27234, #5758 ),
 .UNSPECIFIED., .F., .F.,
 ( 4, 4 ),
 ( 0.03659475354221209537, 0.03709560045499031566 ),
 .UNSPECIFIED. ) ;
#29269=CARTESIAN_POINT ( 'NONE',  ( 777.4774526936600978, -442.2709662947826814, -304.7301800767027657 ) ) ;
#29273=CARTESIAN_POINT ( 'NONE',  ( 794.1144889064781864, -202.1692326535051905, -360.9840315886528401 ) ) ;
#29275=CARTESIAN_POINT ( 'NONE',  ( 773.7943932421234194, -239.8055962898687028, -305.5313806188329409 ) ) ;
#29281=CARTESIAN_POINT ( 'NONE',  ( 788.8264449731200330, -141.1800572038746395, -363.6646147819171233 ) ) ;
#29284=CARTESIAN_POINT ( 'NONE',  ( 745.7998596910086917, -29.36187538569318178, -332.5602148656461168 ) ) ;
#29287=CARTESIAN_POINT ( 'NONE',  ( 748.6759233522253680, -448.3726999360611103, -324.3348316497537098 ) ) ;
#29290=CARTESIAN_POINT ( 'NONE',  ( 766.0291762391763086, -322.9181544815161260, -360.7704444035551319 ) ) ;
#29294=CARTESIAN_POINT ( 'NONE',  ( 762.1405469898971887, -289.5436935675103882, -357.8594530101015607 ) ) ;
#29299=CARTESIAN_POINT ( 'NONE',  ( 796.1575198192839480, -294.0090635724253048, -359.4546378042384163 ) ) ;
#29300=CARTESIAN_POINT ( 'NONE',  ( 754.8072714833581358, -292.8164208402376971, -338.1981804954720587 ) ) ;
#29302=CARTESIAN_POINT ( 'NONE',  ( 759.9864689768902508, -170.0891481129654608, -354.9819416627836404 ) ) ;
#29308=CARTESIAN_POINT ( 'NONE',  ( 781.2370466360911223, -92.73633629969860692, -304.9990715423533629 ) ) ;
#29309=CYLINDRICAL_SURFACE ( 'NONE', #19694, 10.00000000000000888 ) ;
#29314=CARTESIAN_POINT ( 'NONE',  ( 746.8695393053151292, -149.9073299311473875, -327.6429770376306578 ) ) ;
#29318=CARTESIAN_POINT ( 'NONE',  ( 792.3570229623688874, -285.1800572038740711, -373.1304606946836202 ) ) ;
#29324=CARTESIAN_POINT ( 'NONE',  ( 778.7502325331095108, -312.3510508353230080, -304.6391490659818828 ) ) ;
#29326=CARTESIAN_POINT ( 'NONE',  ( 745.7998596910086917, -365.3618753856920875, -332.5602148656461168 ) ) ;
#29330=CARTESIAN_POINT ( 'NONE',  ( 771.2633955100217236, -407.9073299311465348, -363.4237431249939618 ) ) ;
#29332=CARTESIAN_POINT ( 'NONE',  ( 757.8323909638827445, -218.6346026584197944, -352.1044303154654358 ) ) ;
#29333=CARTESIAN_POINT ( 'NONE',  ( 800.1688906516307043, -82.16923265350558836, -369.0717654672308186 ) ) ;
#29337=CARTESIAN_POINT ( 'NONE',  ( 794.1144889064781864, -226.1692326535051052, -360.9840315886528401 ) ) ;
#29339=CARTESIAN_POINT ( 'NONE',  ( 752.4576283171824116, -69.07832356259653750, -317.7880784355627952 ) ) ;
#29340=CARTESIAN_POINT ( 'NONE',  ( 806.2451613922657998, -452.9681489794450613, -344.7413990863497020 ) ) ;
#29343=CARTESIAN_POINT ( 'NONE',  ( 768.9521613784389729, -345.8272453906069472, -373.2346286133773106 ) ) ;
#29346=CARTESIAN_POINT ( 'NONE',  ( 769.9779781133707957, -187.0999726633346825, -316.7813123517150871 ) ) ;
#29347=CARTESIAN_POINT ( 'NONE',  ( 774.6312213355099630, -167.3618753856927412, -364.6798772138717482 ) ) ;
#29348=CARTESIAN_POINT ( 'NONE',  ( 792.1044303154646968, -372.4527844766012095, -317.8323909638837677 ) ) ;
#29350=CARTESIAN_POINT ( 'NONE',  ( 775.9200461376533440, 24.19440371013046231, -315.3028492785443291 ) ) ;
#29359=CARTESIAN_POINT ( 'NONE',  ( 745.1792804349281596, -422.1908817542430370, -343.7566961878542884 ) ) ;
#29362=CARTESIAN_POINT ( 'NONE',  ( 801.1904061080338124, -20.08914811296593328, -368.3070685750236066 ) ) ;
#29364=CARTESIAN_POINT ( 'NONE',  ( 771.2633955100217236, -407.9073299311465348, -363.4237431249939618 ) ) ;
#29365=CARTESIAN_POINT ( 'NONE',  ( 794.9819416627830151, -12.99823902205686821, -319.9864689768909898 ) ) ;
#29368=CARTESIAN_POINT ( 'NONE',  ( 801.5560724626406000, -240.5545181178798941, -326.7756240680316182 ) ) ;
#29376=CARTESIAN_POINT ( 'NONE',  ( 765.0180583372156207, -312.9982390220559409, -360.0135310231089534 ) ) ;
#29379=CARTESIAN_POINT ( 'NONE',  ( 768.9521613784389729, -81.82724539060772884, -373.2346286133773106 ) ) ;
#29380=CARTESIAN_POINT ( 'NONE',  ( 756.7813123517142913, -115.9874144716872877, -329.9779781133712504 ) ) ;
#29384=CARTESIAN_POINT ( 'NONE',  ( 768.0187753319979720, -32.63460265842044095, -318.0580252608186242 ) ) ;
#29385=CARTESIAN_POINT ( 'NONE',  ( 796.7845633553578182, -129.6237781080508853, -358.5707757039688204 ) ) ;
#29386=CARTESIAN_POINT ( 'NONE',  ( 788.4001350590139054, -443.1233509495419298, -363.5803521658918385 ) ) ;
#29397=CARTESIAN_POINT ( 'NONE',  ( 790.9844846989617508, -94.37269993606224716, -317.2208543904092721 ) ) ;
#29399=CARTESIAN_POINT ( 'NONE',  ( 757.8323909638828582, -266.6346026584197375, -352.1044303154654358 ) ) ;
#29401=CARTESIAN_POINT ( 'NONE',  ( 781.8018195045266339, -406.2709662947829088, -365.1927285166406705 ) ) ;
#29402=CARTESIAN_POINT ( 'NONE',  ( 805.1927285166397041, -40.81642084023859951, -341.8018195045277707 ) ) ;
#29406=CARTESIAN_POINT ( 'NONE',  ( 811.3240766477731540, -28.37269993606244967, -355.6651683502462902 ) ) ;
#29408=EDGE_LOOP ( 'NONE', ( #4807, #42314, #632, #40464 ) ) ;
#29409=CARTESIAN_POINT ( 'NONE',  ( 783.7953271457878373, -296.1908817542434917, -375.1787889125761239 ) ) ;
#29414=CARTESIAN_POINT ( 'NONE',  ( 758.0580252608178853, -294.4527844766013800, -328.0187753319985404 ) ) ;
#29416=CARTESIAN_POINT ( 'NONE',  ( 804.1105419155481968, -147.8272453906075157, -347.6308680596136469 ) ) ;
#29418=CARTESIAN_POINT ( 'NONE',  ( 782.5225473063383106, -358.2709662947830225, -375.2698199232970637 ) ) ;
#29422=CARTESIAN_POINT ( 'NONE',  ( 748.3538107759620743, -232.7146871989596377, -355.8262568251490165 ) ) ;
#29428=CARTESIAN_POINT ( 'NONE',  ( 755.8398074228967971, -19.44195992623303937, -333.4516893846970333 ) ) ;
#29429=CARTESIAN_POINT ( 'NONE',  ( 799.9999999999993179, -512.9681489794448908, -329.9999999999999432 ) ) ;
#29434=CARTESIAN_POINT ( 'NONE',  ( 775.9200461376533440, -335.8055962898683902, -315.3028492785443291 ) ) ;
#29436=CARTESIAN_POINT ( 'NONE',  ( 751.2241431872005251, -328.1692326535048210, -359.9636004259367610 ) ) ;
#29439=ORIENTED_EDGE ( 'NONE', *, *, #38242, .F. ) ;
#29442=CARTESIAN_POINT ( 'NONE',  ( 775.9200461376533440, -71.80559628986922860, -315.3028492785443291 ) ) ;
#29446=CARTESIAN_POINT ( 'NONE',  ( 813.1304606946830518, -185.9073299311472454, -352.3570229623690580 ) ) ;
#29448=CARTESIAN_POINT ( 'NONE',  ( 804.9363028652555840, -184.2709662947835909, -338.2165204200192079 ) ) ;
#29450=CARTESIAN_POINT ( 'NONE',  ( 800.9840315886518738, -436.9181544815157281, -354.1144889064786412 ) ) ;
#29453=LINE ( 'NONE', #19727, #20331 ) ;
#29454=DIRECTION ( 'NONE',  ( 0.000000000000000000, 0.000000000000000000, -1.000000000000000000 ) ) ;
#29457=CARTESIAN_POINT ( 'NONE',  ( 796.1575198192839480, -438.0090635724247932, -359.4546378042384163 ) ) ;
#29459=CARTESIAN_POINT ( 'NONE',  ( 795.8262568251477660, -214.3726999360618493, -308.3538107759623585 ) ) ;
#29463=CARTESIAN_POINT ( 'NONE',  ( 769.1273215169530886, -334.7146871989593251, -317.4527132478988847 ) ) ;
#29465=CARTESIAN_POINT ( 'NONE',  ( 755.8990559732751535, -203.4636090269709996, -365.9055244015606831 ) ) ;
#29467=DIRECTION ( 'NONE',  ( 0.000000000000000000, -1.000000000000000000, 0.000000000000000000 ) ) ;
#29469=CARTESIAN_POINT ( 'NONE',  ( 763.0537975583476964, -240.4527844766015789, -371.0346526505628617 ) ) ;
#29472=CARTESIAN_POINT ( 'NONE',  ( 757.8323909638827445, -2.634602658420536869, -352.1044303154654358 ) ) ;
#29476=CARTESIAN_POINT ( 'NONE',  ( 807.5423716828161105, -129.0783235625963243, -362.2119215644372048 ) ) ;
#29478=CARTESIAN_POINT ( 'NONE',  ( 751.9810565676468741, -362.0891481129648923, -360.9747183278973921 ) ) ;
#29484=CARTESIAN_POINT ( 'NONE',  ( 774.6312213355099630, -407.3618753856920307, -364.6798772138717482 ) ) ;
#29485=CARTESIAN_POINT ( 'NONE',  ( 808.3070685750230950, -450.9982390220554294, -361.1904061080339261 ) ) ;
#29489=CARTESIAN_POINT ( 'NONE',  ( 783.0433043558608688, -216.8965053807778816, -315.1538015810313027 ) ) ;
#29491=CARTESIAN_POINT ( 'NONE',  ( 746.7653713866222915, -233.2601417444141987, -351.0478386215610271 ) ) ;
#29496=EDGE_CURVE ( 'NONE', #34870, #811, #2555, .T. ) ;
#29499=CARTESIAN_POINT ( 'NONE',  ( 754.9967657858570647, -73.54369356751118403, -365.0032342141425374 ) ) ;
#29500=CARTESIAN_POINT ( 'NONE',  ( 800.2193346964446619, -66.99823902205670834, -355.1360043628816925 ) ) ;
#29502=CARTESIAN_POINT ( 'NONE',  ( 805.2837595273609850, -26.73633629969882008, -340.5290396650784714 ) ) ;
#29503=ORIENTED_EDGE ( 'NONE', *, *, #18785, .T. ) ;
#29504=CARTESIAN_POINT ( 'NONE',  ( 801.5560724626406000, -312.5545181178797520, -326.7756240680316182 ) ) ;
#29507=CARTESIAN_POINT ( 'NONE',  ( 767.8955696845333705, -336.4527844766012095, -362.1676090361162323 ) ) ;
#29512=CARTESIAN_POINT ( 'NONE',  ( 769.0155153010367712, -322.3726999360615082, -362.7791456095907279 ) ) ;
#29513=CARTESIAN_POINT ( 'NONE',  ( 803.4237431249931660, -303.1800572038740711, -331.2633955100225194 ) ) ;
#29515=CARTESIAN_POINT ( 'NONE',  ( 785.3141322388236176, -141.7255117493291721, -364.4286716492789537 ) ) ;
#29516=DIRECTION ( 'NONE',  ( 0.000000000000000000, 0.000000000000000000, -1.000000000000000000 ) ) ;
#29520=CARTESIAN_POINT ( 'NONE',  ( 747.6481478633932056, -85.09997266333499510, -353.4146539503763620 ) ) ;
#29521=DIRECTION ( 'NONE',  ( 0.000000000000000000, 0.000000000000000000, -1.000000000000000000 ) ) ;
#29526=CARTESIAN_POINT ( 'NONE',  ( 814.9108240113580450, -136.2709662947837330, -337.5031285880265273 ) ) ;
#29531=CARTESIAN_POINT ( 'NONE',  ( 810.7187646348534145, -282.4527844766014937, -356.7737145352016341 ) ) ;
#29535=CARTESIAN_POINT ( 'NONE',  ( 746.0683387631852383, -355.4419599262319593, -331.3260364891676204 ) ) ;
#29536=CARTESIAN_POINT ( 'NONE',  ( 754.9967657858570647, -97.54369356751112718, -365.0032342141425374 ) ) ;
#29538=CARTESIAN_POINT ( 'NONE',  ( 814.2001403089898304, -353.3618753856922012, -347.4397851343538264 ) ) ;
#29541=ORIENTED_EDGE ( 'NONE', *, *, #771, .F. ) ;
#29543=CARTESIAN_POINT ( 'NONE',  ( 804.4286716492782716, -425.3618753856919170, -345.3141322388244703 ) ) ;
#29544=CARTESIAN_POINT ( 'NONE',  ( 804.4286716492782716, -209.3618753856926276, -345.3141322388244703 ) ) ;
#29545=CARTESIAN_POINT ( 'NONE',  ( 771.2368401574024119, -109.4419599262327836, -374.2805881961240857 ) ) ;
#29550=CARTESIAN_POINT ( 'NONE',  ( 800.7704444035546203, -244.1692326535050768, -326.0291762391768771 ) ) ;
#29553=CARTESIAN_POINT ( 'NONE',  ( 767.6429770376289525, 14.81994279612486309, -306.8695393053162093 ) ) ;
#29554=CARTESIAN_POINT ( 'NONE',  ( 801.9858362298568863, -51.07832356259657303, -312.7379699480935642 ) ) ;
#29558=CARTESIAN_POINT ( 'NONE',  ( 762.1177392798416577, -378.5545181178795247, -309.8865473780659272 ) ) ;
#29562=CARTESIAN_POINT ( 'NONE',  ( 779.4763451958990572, -200.7363362996982801, -365.0264073115438919 ) ) ;
#29563=CARTESIAN_POINT ( 'NONE',  ( 778.2165204200184689, -166.8164208402382087, -364.9363028652563230 ) ) ;
#29564=CARTESIAN_POINT ( 'NONE',  ( 800.0135310231082713, -398.0891481129647218, -325.0180583372163028 ) ) ;
#29575=CARTESIAN_POINT ( 'NONE',  ( 791.0478386215596629, -429.8272453906067199, -306.7653713866226326 ) ) ;
#29576=CARTESIAN_POINT ( 'NONE',  ( 767.6429770376291799, -33.18005720387498769, -306.8695393053162093 ) ) ;
#29578=CARTESIAN_POINT ( 'NONE',  ( 755.3201227861273992, -387.7255117493283478, -345.3687786644892981 ) ) ;
#29579=CARTESIAN_POINT ( 'NONE',  ( 785.3687786644885591, -11.36187538569323863, -315.3201227861280813 ) ) ;
#29582=CARTESIAN_POINT ( 'NONE',  ( 757.4527132478984868, -256.3726999360617924, -329.1273215169538844 ) ) ;
#29583=CARTESIAN_POINT ( 'NONE',  ( 814.9108240113580450, -160.2709662947836762, -337.5031285880265273 ) ) ;
#29586=CARTESIAN_POINT ( 'NONE',  ( 779.2785047387700388, 16.45630643248848912, -314.0977342670951202 ) ) ;
#29591=CARTESIAN_POINT ( 'NONE',  ( 759.9864689768902508, -314.0891481129650629, -354.9819416627836404 ) ) ;
#29593=CARTESIAN_POINT ( 'NONE',  ( 745.7194118038753459, -85.64542720878952764, -348.7631598425976449 ) ) ;
#29594=CARTESIAN_POINT ( 'NONE',  ( 805.1016975059191054, -126.8965053807781516, -343.0745993439771837 ) ) ;
#29597=CARTESIAN_POINT ( 'NONE',  ( 792.1044303154645831, -12.45278447660232146, -317.8323909638837677 ) ) ;
#29598=CARTESIAN_POINT ( 'NONE',  ( 754.8983024940795303, -114.8965053807782226, -336.9254006560228163 ) ) ;
#29599=CARTESIAN_POINT ( 'NONE',  ( 774.6312213355099630, -119.3618753856928691, -364.6798772138717482 ) ) ;
#29601=CARTESIAN_POINT ( 'NONE',  ( 798.7617431975189675, -435.6237781080499190, -323.0428371773161871 ) ) ;
#29607=VERTEX_POINT ( 'NONE', #12433 ) ;
#29612=VERTEX_POINT ( 'NONE', #40402 ) ;
#29613=CARTESIAN_POINT ( 'NONE',  ( 757.4527132478984868, -64.37269993606231822, -329.1273215169538844 ) ) ;
#29614=CARTESIAN_POINT ( 'NONE',  ( 755.0636971347428243, -292.2709662947831930, -341.7834795799807353 ) ) ;
#29616=CARTESIAN_POINT ( 'NONE',  ( 764.8639956371174549, -392.0891481129648355, -319.7806653035542013 ) ) ;
#29617=CARTESIAN_POINT ( 'NONE',  ( 788.8264449731200330, -45.18005720387493085, -363.6646147819171233 ) ) ;
#29621=DIRECTION ( 'NONE',  ( -1.000000000000000000, -0.000000000000000000, -0.000000000000000000 ) ) ;
#29622=ORIENTED_EDGE ( 'NONE', *, *, #1300, .F. ) ;
#29623=CARTESIAN_POINT ( 'NONE',  ( 788.6739635108323228, -295.6454272087888739, -373.9316612368139090 ) ) ;
#29625=CARTESIAN_POINT ( 'NONE',  ( 803.6646147819161570, -281.9073299311468759, -348.8264449731210561 ) ) ;
#29627=CARTESIAN_POINT ( 'NONE',  ( 766.9102291470427417, -162.5545181178802352, -318.6633372737382501 ) ) ;
#29630=CARTESIAN_POINT ( 'NONE',  ( 758.0141637701419768, -15.07832356259669560, -367.2620300519063790 ) ) ;
#29631=CARTESIAN_POINT ( 'NONE',  ( 777.5031285880264704, -358.8164208402375834, -374.9108240113588408 ) ) ;
#29636=CARTESIAN_POINT ( 'NONE',  ( 803.8556311672234642, -441.6237781080499190, -365.6418435158340117 ) ) ;
#29641=CARTESIAN_POINT ( 'NONE',  ( 786.6156483768007774, -1.441959926233096656, -315.5913626894246136 ) ) ;
#29647=CARTESIAN_POINT ( 'NONE',  ( 804.9511171171677688, -317.8055962898684470, -335.8780910478229202 ) ) ;
#29651=CARTESIAN_POINT ( 'NONE',  ( 807.5423716828161105, -345.0783235625956991, -362.2119215644372048 ) ) ;
#29657=CARTESIAN_POINT ( 'NONE',  ( 814.9108240113580450, -184.2709662947835909, -337.5031285880265273 ) ) ;
#29661=CARTESIAN_POINT ( 'NONE',  ( 801.9419747391806368, -162.4527844766018632, -351.9812246680014027 ) ) ;
#29663=CARTESIAN_POINT ( 'NONE',  ( 761.4292242960306112, -425.4636090269703459, -323.2154366446414429 ) ) ;
#29668=ORIENTED_EDGE ( 'NONE', *, *, #37727, .T. ) ;
#29670=CARTESIAN_POINT ( 'NONE',  ( 773.4516893846965786, -427.6454272087885897, -315.8398074228977066 ) ) ;
#29671=CARTESIAN_POINT ( 'NONE',  ( 745.1792804349281596, -206.1908817542437191, -343.7566961878542884 ) ) ;
#29674=CARTESIAN_POINT ( 'NONE',  ( 755.3201227861273992, -171.7255117493291152, -345.3687786644892981 ) ) ;
#29675=CARTESIAN_POINT ( 'NONE',  ( 755.8398074228967971, -331.4419599262320162, -333.4516893846970333 ) ) ;
#29677=CARTESIAN_POINT ( 'NONE',  ( 797.8822607201568644, -222.5545181178800362, -370.1134526219340160 ) ) ;
#29680=CARTESIAN_POINT ( 'NONE',  ( 793.0897708529556667, -30.55451811788062244, -361.3366627262616362 ) ) ;
#29683=CARTESIAN_POINT ( 'NONE',  ( 751.6929314249750860, -246.9982390220560831, -318.8095938919659034 ) ) ;
#29686=CARTESIAN_POINT ( 'NONE',  ( 754.8072714833581358, -28.81642084023863148, -338.1981804954720587 ) ) ;
#29688=CARTESIAN_POINT ( 'NONE',  ( 747.3154664389472828, -115.9874144716872877, -326.4474001241230781 ) ) ;
#29690=CARTESIAN_POINT ( 'NONE',  ( 748.9653473494363425, -386.6346026584191691, -356.9462024416521331 ) ) ;
#29696=CARTESIAN_POINT ( 'NONE',  ( 778.1981804954714335, -394.2709662947827951, -314.8072714833589885 ) ) ;
#29698=CARTESIAN_POINT ( 'NONE',  ( 805.0032342141412300, -445.5436935675098766, -314.9967657858571783 ) ) ;
#29703=CARTESIAN_POINT ( 'NONE',  ( 764.0069404352550464, -231.0783235625960401, -359.2566176426627180 ) ) ;
#29705=CARTESIAN_POINT ( 'NONE',  ( 813.9316612368132837, -223.4419599262323857, -348.6739635108323228 ) ) ;
#29710=CARTESIAN_POINT ( 'NONE',  ( 782.4968714119720516, -82.81642084023846451, -305.0891759886411023 ) ) ;
#29712=CARTESIAN_POINT ( 'NONE',  ( 805.1927285166399315, -64.81642084023852135, -341.8018195045277707 ) ) ;
#29714=CARTESIAN_POINT ( 'NONE',  ( 804.1105419155481968, -3.827245390607979303, -347.6308680596136469 ) ) ;
#29716=CARTESIAN_POINT ( 'NONE',  ( 776.9254006560222479, -308.1908817542434349, -314.8983024940802125 ) ) ;
#29723=CARTESIAN_POINT ( 'NONE',  ( 761.4292242960306112, -329.4636090269706870, -323.2154366446414429 ) ) ;
#29724=CARTESIAN_POINT ( 'NONE',  ( 762.3223304703356007, -319.5436935675104451, -322.3223304703362828 ) ) ;
#29725=CARTESIAN_POINT ( 'NONE',  ( 804.9363028652555840, -160.2709662947836762, -338.2165204200192079 ) ) ;
#29729=CARTESIAN_POINT ( 'NONE',  ( 746.4236121716829757, -111.8272453906076151, -328.8385539511384650 ) ) ;
#29734=CARTESIAN_POINT ( 'NONE',  ( 801.1904061080338124, -140.0891481129655176, -368.3070685750236066 ) ) ;
#29737=CARTESIAN_POINT ( 'NONE',  ( 804.7487373415286811, -283.5436935675105019, -364.7487373415288516 ) ) ;
#29739=CARTESIAN_POINT ( 'NONE',  ( 751.6929314249750860, -438.9982390220554294, -318.8095938919659034 ) ) ;
#29743=CARTESIAN_POINT ( 'NONE',  ( 812.6845335610512393, -343.9874144716865771, -353.5525998758768651 ) ) ;
#29745=CARTESIAN_POINT ( 'NONE',  ( 767.6429770376289525, -81.18005720387481006, -306.8695393053162093 ) ) ;
#29747=CARTESIAN_POINT ( 'NONE',  ( 751.9810565676468741, -362.0891481129648923, -360.9747183278973921 ) ) ;
#29753=CARTESIAN_POINT ( 'NONE',  ( 755.0636971347428243, -220.2709662947834772, -341.7834795799807353 ) ) ;
#29754=CARTESIAN_POINT ( 'NONE',  ( 746.7653713866222915, -113.2601417444145682, -351.0478386215610271 ) ) ;
#29760=CARTESIAN_POINT ( 'NONE',  ( 799.4546378042377910, -225.0783235625959833, -356.1575198192848006 ) ) ;
#29762=CARTESIAN_POINT ( 'NONE',  ( 764.3348316497523456, -430.7146871989590409, -308.6759233522265617 ) ) ;
#29763=CARTESIAN_POINT ( 'NONE',  ( 808.7758568127978833, -76.16923265350557415, -320.0363995740631822 ) ) ;
#29768=CARTESIAN_POINT ( 'NONE',  ( 755.8990559732751535, -371.4636090269705164, -365.9055244015606831 ) ) ;
#29770=CARTESIAN_POINT ( 'NONE',  ( 803.4237431249931660, -231.1800572038743553, -331.2633955100225194 ) ) ;
#29774=CARTESIAN_POINT ( 'NONE',  ( 757.4527132478984868, -232.3726999360617924, -329.1273215169538844 ) ) ;
#29775=CARTESIAN_POINT ( 'NONE',  ( 764.8639956371174549, -176.0891481129653755, -319.7806653035542013 ) ) ;
#29777=CARTESIAN_POINT ( 'NONE',  ( 781.8018195045267476, -382.2709662947829088, -365.1927285166407273 ) ) ;
#29781=CARTESIAN_POINT ( 'NONE',  ( 757.8323909638827445, -98.63460265842024910, -352.1044303154654358 ) ) ;
#29790=CARTESIAN_POINT ( 'NONE',  ( 749.5768839229115201, -444.5545181178792973, -358.0661480581553064 ) ) ;
#29791=CARTESIAN_POINT ( 'NONE',  ( 804.7487373415286811, -43.54369356751131903, -364.7487373415288516 ) ) ;
#29793=CARTESIAN_POINT ( 'NONE',  ( 755.5713283507202505, -389.3618753856919739, -334.6858677611754729 ) ) ;
#29794=CARTESIAN_POINT ( 'NONE',  ( 788.8264449731201466, 2.819942796124898621, -363.6646147819170665 ) ) ;
#29796=ADVANCED_FACE ( 'NONE', ( #13575 ), #10111, .T. ) ;
#29799=CARTESIAN_POINT ( 'NONE',  ( 802.5472867521000353, -268.3726999360616787, -350.8726784830461156 ) ) ;
#29800=CARTESIAN_POINT ( 'NONE',  ( 810.7187646348534145, -162.4527844766018632, -356.7737145352016341 ) ) ;
#29804=CARTESIAN_POINT ( 'NONE',  ( 787.3558975768202117, 16.45630643248848557, -313.9911135047267408 ) ) ;
#29808=CARTESIAN_POINT ( 'NONE',  ( 762.1405469898971887, -313.5436935675102745, -357.8594530101015607 ) ) ;
#29811=AXIS2_PLACEMENT_3D ( 'NONE', #943, #42542, #11811 ) ;
#29812=CARTESIAN_POINT ( 'NONE',  ( 766.4474001241216001, -115.0999726633348956, -307.3154664389482491 ) ) ;
#29813=CARTESIAN_POINT ( 'NONE',  ( 796.7845633553578182, -129.6237781080508853, -358.5707757039688204 ) ) ;
#29817=CARTESIAN_POINT ( 'NONE',  ( 756.3353852180819104, -29.90732993114771787, -331.1735550268788302 ) ) ;
#29818=CARTESIAN_POINT ( 'NONE',  ( 775.9200461376533440, -143.8055962898690154, -315.3028492785443291 ) ) ;
#29819=CARTESIAN_POINT ( 'NONE',  ( 785.3141322388236176, -117.7255117493292715, -364.4286716492789537 ) ) ;
#29821=CARTESIAN_POINT ( 'NONE',  ( 765.8855110935204493, -430.1692326535043094, -319.0159684113471599 ) ) ;
#29825=VERTEX_POINT ( 'NONE', #2726 ) ;
#29827=CARTESIAN_POINT ( 'NONE',  ( 766.4474001241216001, -259.0999726633343698, -307.3154664389482491 ) ) ;
#29835=CARTESIAN_POINT ( 'NONE',  ( 800.9840315886518738, -124.9181544815167086, -354.1144889064786412 ) ) ;
#29836=CARTESIAN_POINT ( 'NONE',  ( 804.9363028652555840, -280.2709662947833067, -338.2165204200192079 ) ) ;
#29838=CARTESIAN_POINT ( 'NONE',  ( 762.1405469898971887, -409.5436935675101040, -357.8594530101015607 ) ) ;
#29839=CARTESIAN_POINT ( 'NONE',  ( 756.5762568750052424, -99.18005720387478164, -348.7366044899774238 ) ) ;
#29841=FACE_OUTER_BOUND ( 'NONE', #44283, .T. ) ;
#29844=CARTESIAN_POINT ( 'NONE',  ( 811.3240766477731540, -4.372699936062523385, -355.6651683502462902 ) ) ;
#29847=CARTESIAN_POINT ( 'NONE',  ( 802.2119215644370342, -294.0090635724253048, -367.5423716828165084 ) ) ;
#29851=CARTESIAN_POINT ( 'NONE',  ( 804.9363028652555840, -280.2709662947833067, -338.2165204200192079 ) ) ;
#29853=CARTESIAN_POINT ( 'NONE',  ( 801.5560724626406000, -168.5545181178802352, -326.7756240680316182 ) ) ;
#29855=CARTESIAN_POINT ( 'NONE',  ( 787.4397851343537695, -333.7255117493286320, -374.2001403089903988 ) ) ;
#29861=CARTESIAN_POINT ( 'NONE',  ( 755.2512626584698410, 16.45630643248849267, -315.2512626584710915 ) ) ;
#29868=CARTESIAN_POINT ( 'NONE',  ( 757.2208543904082489, -16.71468719896031985, -350.9844846989624330 ) ) ;
#29874=CARTESIAN_POINT ( 'NONE',  ( 776.9566956441375396, -324.8965053807775121, -364.8461984189686405 ) ) ;
#29877=CARTESIAN_POINT ( 'NONE',  ( 805.9055244015594326, -315.6237781080503169, -315.8990559732753240 ) ) ;
#29883=CARTESIAN_POINT ( 'NONE',  ( 808.3070685750230950, -186.9982390220563104, -361.1904061080339261 ) ) ;
#29886=CARTESIAN_POINT ( 'NONE',  ( 758.0580252608178853, -174.4527844766018063, -328.0187753319985404 ) ) ;
#29888=CARTESIAN_POINT ( 'NONE',  ( 755.3028492785439312, -423.2817908451521589, -335.9200461376539693 ) ) ;
#29896=CARTESIAN_POINT ( 'NONE',  ( 772.4468031744293057, -417.8272453906067199, -363.8651313633793620 ) ) ;
#29897=DIRECTION ( 'NONE',  ( 0.000000000000000000, 0.000000000000000000, 1.000000000000000000 ) ) ;
#29899=CARTESIAN_POINT ( 'NONE',  ( 814.2805881961230625, -193.6454272087891582, -331.2368401574024119 ) ) ;
#29901=DIRECTION ( 'NONE',  ( -0.000000000000000000, 1.000000000000000000, -0.000000000000000000 ) ) ;
#29902=CARTESIAN_POINT ( 'NONE',  ( 800.0135310231082713, -182.0891481129654323, -325.0180583372163028 ) ) ;
#29903=CARTESIAN_POINT ( 'NONE',  ( 794.1144889064781864, -346.1692326535047641, -360.9840315886528401 ) ) ;
#29905=CARTESIAN_POINT ( 'NONE',  ( 757.7880784355613741, -234.0090635724255037, -312.4576283171834916 ) ) ;
#29908=CARTESIAN_POINT ( 'NONE',  ( 758.4439275373578084, -60.55451811788051941, -353.2243759319684386 ) ) ;
#29910=EDGE_CURVE ( 'NONE', #14643, #10014, #10675, .T. ) ;
#29912=CARTESIAN_POINT ( 'NONE',  ( 808.3070685750232087, -258.9982390220561115, -361.1904061080339829 ) ) ;
#29916=CARTESIAN_POINT ( 'NONE',  ( 758.0580252608178853, -54.45278447660219001, -328.0187753319985404 ) ) ;
#29918=CARTESIAN_POINT ( 'NONE',  ( 776.2433038121456548, -132.8965053807781374, -374.8207195650711014 ) ) ;
#29920=CARTESIAN_POINT ( 'NONE',  ( 763.2262854647970016, -368.6346026584193964, -309.2812353651462445 ) ) ;
#29925=CARTESIAN_POINT ( 'NONE',  ( 764.8639956371174549, -392.0891481129648355, -319.7806653035542013 ) ) ;
#29928=CARTESIAN_POINT ( 'NONE',  ( 788.6739635108323228, -7.645427208789786100, -373.9316612368139090 ) ) ;
#29929=LINE ( 'NONE', #30155, #21020 ) ;
#29933=CARTESIAN_POINT ( 'NONE',  ( 759.2295555964440155, -232.1692326535051620, -353.9708237608231229 ) ) ;
#29935=CARTESIAN_POINT ( 'NONE',  ( 810.1134526219336749, -224.5328690171415076, -357.8822607201570349 ) ) ;
#29938=EDGE_LOOP ( 'NONE', ( #30963, #23413, #43792, #25335 ) ) ;
#29939=CARTESIAN_POINT ( 'NONE',  ( 785.3141322388236176, -141.7255117493291721, -364.4286716492789537 ) ) ;
#29941=CARTESIAN_POINT ( 'NONE',  ( 763.2262854647970016, -80.63460265842029173, -309.2812353651462445 ) ) ;
#29942=CARTESIAN_POINT ( 'NONE',  ( 774.6858677611749044, -81.72551174932937101, -315.5713283507209894 ) ) ;
#29944=CARTESIAN_POINT ( 'NONE',  ( 790.0220218866281812, -7.099972663335241130, -363.2186876482849129 ) ) ;
#29947=CARTESIAN_POINT ( 'NONE',  ( 796.1575198192839480, -318.0090635724251911, -359.4546378042384163 ) ) ;
#29955=CARTESIAN_POINT ( 'NONE',  ( 758.4439275373578084, -324.5545181178796952, -353.2243759319684386 ) ) ;
#29956=CARTESIAN_POINT ( 'NONE',  ( 757.8323909638827445, -338.6346026584195101, -352.1044303154654358 ) ) ;
#29957=CARTESIAN_POINT ( 'NONE',  ( 764.8639956371174549, -152.0891481129655460, -319.7806653035542013 ) ) ;
#29962=CARTESIAN_POINT ( 'NONE',  ( 799.4546378042377910, -273.0783235625958696, -356.1575198192848006 ) ) ;
#29963=CARTESIAN_POINT ( 'NONE',  ( 776.2046728542105711, -116.1908817542440033, -304.8212110874238761 ) ) ;
#29970=CARTESIAN_POINT ( 'NONE',  ( 808.3070685750232087, -138.9982390220564241, -361.1904061080339829 ) ) ;
#29973=CARTESIAN_POINT ( 'NONE',  ( 777.4774526936600978, -274.2709662947833067, -304.7301800767027657 ) ) ;
#29974=CARTESIAN_POINT ( 'NONE',  ( 763.2262854647970016, -440.6346026584191122, -309.2812353651462445 ) ) ;
#29976=ORIENTED_EDGE ( 'NONE', *, *, #151, .F. ) ;
#29977=CARTESIAN_POINT ( 'NONE',  ( 807.5423716828161105, -345.0783235625956991, -362.2119215644372048 ) ) ;
#29978=CARTESIAN_POINT ( 'NONE',  ( 751.9810565676468741, -74.08914811296577341, -360.9747183278973921 ) ) ;
#29980=CARTESIAN_POINT ( 'NONE',  ( 748.9653473494363425, -338.6346026584195101, -356.9462024416521331 ) ) ;
#29983=ORIENTED_EDGE ( 'NONE', *, *, #12485, .F. ) ;
#29985=CARTESIAN_POINT ( 'NONE',  ( 781.2497674668890113, -132.3510508353235764, -375.3608509340180603 ) ) ;
#29990=CARTESIAN_POINT ( 'NONE',  ( 805.0264073115434940, -6.351050835323991173, -339.4763451958999099 ) ) ;
#29993=CARTESIAN_POINT ( 'NONE',  ( 773.7943932421234194, -431.8055962898681059, -305.5313806188329409 ) ) ;
#29997=CARTESIAN_POINT ( 'NONE',  ( 814.4686193811664907, -363.2817908451523294, -346.2056067578752732 ) ) ;
#29998=CARTESIAN_POINT ( 'NONE',  ( 767.8955696845333705, -240.4527844766015221, -362.1676090361162323 ) ) ;
#30002=CARTESIAN_POINT ( 'NONE',  ( 790.9844846989617508, -214.3726999360618493, -317.2208543904092721 ) ) ;
#30003=CARTESIAN_POINT ( 'NONE',  ( 804.9363028652555840, -232.2709662947834488, -338.2165204200192079 ) ) ;
#30004=CARTESIAN_POINT ( 'NONE',  ( 788.7366044899766848, -395.9073299311465348, -316.5762568750059813 ) ) ;
#30007=CARTESIAN_POINT ( 'NONE',  ( 801.9419747391806368, -90.45278447660209054, -351.9812246680014027 ) ) ;
#30018=CARTESIAN_POINT ( 'NONE',  ( 814.2805881961230625, -457.6454272087884760, -331.2368401574024119 ) ) ;
#30019=CARTESIAN_POINT ( 'NONE',  ( 812.7932403749906598, -39.18005720387496638, -327.7687537140311633 ) ) ;
#30022=CARTESIAN_POINT ( 'NONE',  ( 785.3687786644884454, -395.3618753856918602, -315.3201227861279676 ) ) ;
#30023=CARTESIAN_POINT ( 'NONE',  ( 757.8323909638828582, -2.634602658420536425, -352.1044303154654358 ) ) ;
#30026=CARTESIAN_POINT ( 'NONE',  ( 755.1538015810308480, -302.1908817542433781, -343.0433043558613804 ) ) ;
#30027=CARTESIAN_POINT ( 'NONE',  ( 751.6929314249748586, -150.9982390220563957, -318.8095938919659034 ) ) ;
#30031=CARTESIAN_POINT ( 'NONE',  ( 794.6702036691820012, 16.45630643248850689, -314.5864782580647443 ) ) ;
#30037=CARTESIAN_POINT ( 'NONE',  ( 778.2165204200184689, -358.8164208402375834, -364.9363028652563230 ) ) ;
#30040=CARTESIAN_POINT ( 'NONE',  ( 807.2620300519052989, -96.00906357242585898, -318.0141637701419768 ) ) ;
#30041=CARTESIAN_POINT ( 'NONE',  ( 784.0799538623451781, -131.8055962898690439, -364.6971507214555572 ) ) ;
#30045=CARTESIAN_POINT ( 'NONE',  ( 804.6798772138708955, -39.72551174932951312, -334.6312213355107019 ) ) ;
#30046=CARTESIAN_POINT ( 'NONE',  ( 755.8398074228967971, -115.4419599262327409, -333.4516893846970333 ) ) ;
#30048=CARTESIAN_POINT ( 'NONE',  ( 805.9055244015594326, 20.37622189194865285, -315.8990559732753240 ) ) ;
#30054=CARTESIAN_POINT ( 'NONE',  ( 810.4231160770870019, -288.5545181178798657, -321.9338519418446936 ) ) ;
#30064=CARTESIAN_POINT ( 'NONE',  ( 796.1575198192839480, -126.0090635724257737, -359.4546378042384163 ) ) ;
#30065=CARTESIAN_POINT ( 'NONE',  ( 771.2633955100217236, -119.9073299311474443, -363.4237431249939618 ) ) ;
#30066=CARTESIAN_POINT ( 'NONE',  ( 768.0187753319979720, -296.6346026584195670, -318.0580252608186242 ) ) ;
#30068=CARTESIAN_POINT ( 'NONE',  ( 756.3353852180819104, -413.9073299311465348, -331.1735550268788302 ) ) ;
#30069=CARTESIAN_POINT ( 'NONE',  ( 759.9864689768902508, -74.08914811296577341, -354.9819416627836404 ) ) ;
#30077=CARTESIAN_POINT ( 'NONE',  ( 797.8822607201568644, -342.5545181178796952, -370.1134526219340160 ) ) ;
#30080=CARTESIAN_POINT ( 'NONE',  ( 795.1360043628807261, -284.0891481129650629, -360.2193346964456282 ) ) ;
#30082=CARTESIAN_POINT ( 'NONE',  ( 804.1105419155481968, -195.8272453906074304, -347.6308680596136469 ) ) ;
#30085=CARTESIAN_POINT ( 'NONE',  ( 812.7932403749906598, -375.1800572038739574, -327.7687537140311633 ) ) ;
#30091=CARTESIAN_POINT ( 'NONE',  ( 763.0537975583475827, -24.45278447660229304, -371.0346526505627480 ) ) ;
#30096=CARTESIAN_POINT ( 'NONE',  ( 801.3366627262608972, -8.532869017142163059, -353.0897708529566899 ) ) ;
#30101=CARTESIAN_POINT ( 'NONE',  ( 756.1348686366196716, -329.2601417444138860, -347.5531968255698416 ) ) ;
#30105=CARTESIAN_POINT ( 'NONE',  ( 815.1787889125755555, -342.8965053807773984, -343.7953271457877804 ) ) ;
#30111=CARTESIAN_POINT ( 'NONE',  ( 777.4774526936600978, -178.2709662947835625, -304.7301800767027657 ) ) ;
#30115=CARTESIAN_POINT ( 'NONE',  ( 788.8264449731201466, -165.1800572038745543, -363.6646147819170665 ) ) ;
#30116=ORIENTED_EDGE ( 'NONE', *, *, #40773, .F. ) ;
#30118=CARTESIAN_POINT ( 'NONE',  ( 758.4439275373578084, -444.5545181178792973, -353.2243759319684386 ) ) ;
#30124=CARTESIAN_POINT ( 'NONE',  ( 758.4439275373578084, -420.5545181178793541, -353.2243759319684386 ) ) ;
#30125=DIRECTION ( 'NONE',  ( 1.000000000000000000, 0.000000000000000000, -0.000000000000000000 ) ) ;
#30127=CARTESIAN_POINT ( 'NONE',  ( 755.8990559732751535, -227.4636090269709143, -365.9055244015606831 ) ) ;
#30130=CARTESIAN_POINT ( 'NONE',  ( 778.1981804954714335, -178.2709662947835625, -314.8072714833589885 ) ) ;
#30131=CARTESIAN_POINT ( 'NONE',  ( 796.7845633553578182, -345.6237781080501463, -358.5707757039688204 ) ) ;
#30133=CARTESIAN_POINT ( 'NONE',  ( 781.2370466360911223, -236.7363362996981380, -304.9990715423533629 ) ) ;
#30136=CARTESIAN_POINT ( 'NONE',  ( 802.9823548866075953, -49.09997266333511590, -330.0799878456151077 ) ) ;
#30139=CARTESIAN_POINT ( 'NONE',  ( 757.2208543904082489, -424.7146871989589840, -350.9844846989624330 ) ) ;
#30140=CARTESIAN_POINT ( 'NONE',  ( 800.9747183278959710, -276.9982390220559978, -311.9810565676471583 ) ) ;
#30143=CARTESIAN_POINT ( 'NONE',  ( 803.4237431249931660, -63.18005720387488822, -331.2633955100225194 ) ) ;
#30145=CARTESIAN_POINT ( 'NONE',  ( 752.4576283171824116, -141.0783235625962959, -317.7880784355627952 ) ) ;
#30147=CARTESIAN_POINT ( 'NONE',  ( 751.9810565676468741, -386.0891481129647786, -360.9747183278973921 ) ) ;
#30148=CARTESIAN_POINT ( 'NONE',  ( 759.9999999999992042, -462.9681489794448339, -317.6393202250019954 ) ) ;
#30151=CARTESIAN_POINT ( 'NONE',  ( 756.3353852180819104, -389.9073299311465348, -331.1735550268788302 ) ) ;
#30154=CARTESIAN_POINT ( 'NONE',  ( 745.5313806188320314, -39.28179084515331709, -333.7943932421247268 ) ) ;
#30155=CARTESIAN_POINT ( 'NONE',  ( 799.9999999999993179, -512.9681489794448908, -350.0000000000000000 ) ) ;
#30158=CARTESIAN_POINT ( 'NONE',  ( 763.2154366446407039, -213.6237781080506011, -321.4292242960311228 ) ) ;
#30160=CARTESIAN_POINT ( 'NONE',  ( 749.8865473780648472, -236.5328690171414792, -322.1177392798429082 ) ) ;
#30163=VERTEX_POINT ( 'NONE', #32962 ) ;
#30166=CARTESIAN_POINT ( 'NONE',  ( 756.3353852180819104, -173.9073299311472169, -331.1735550268788302 ) ) ;
#30168=CARTESIAN_POINT ( 'NONE',  ( 777.5031285880264704, -70.81642084023850714, -374.9108240113588408 ) ) ;
#30169=CARTESIAN_POINT ( 'NONE',  ( 791.9812246680005501, -68.63460265842033436, -361.9419747391813189 ) ) ;
#30171=CARTESIAN_POINT ( 'NONE',  ( 755.1538015810308480, -14.19088175424431242, -343.0433043558613804 ) ) ;
#30173=CARTESIAN_POINT ( 'NONE',  ( 779.4763451958990572, -368.7363362996977685, -365.0264073115438919 ) ) ;
#30180=CARTESIAN_POINT ( 'NONE',  ( 804.4086373105744769, -337.6454272087888171, -333.3843516231986541 ) ) ;
#30181=CARTESIAN_POINT ( 'NONE',  ( 759.7806653035534055, -318.9982390220557704, -324.8639956371180801 ) ) ;
#30182=CARTESIAN_POINT ( 'NONE',  ( 781.7834795799800531, -154.8164208402382371, -315.0636971347436202 ) ) ;
#30187=CARTESIAN_POINT ( 'NONE',  ( 776.9566956441375396, -276.8965053807776258, -364.8461984189686405 ) ) ;
#30188=CARTESIAN_POINT ( 'NONE',  ( 746.4236121716829757, -135.8272453906076009, -328.8385539511384650 ) ) ;
#30195=CARTESIAN_POINT ( 'NONE',  ( 754.9967657858570647, -145.5436935675109851, -365.0032342141425943 ) ) ;
#30196=CARTESIAN_POINT ( 'NONE',  ( 758.9356612065449781, 18.10977687916123813, -318.6379319222613731 ) ) ;
#30198=CARTESIAN_POINT ( 'NONE',  ( 805.0032342141412300, -253.5436935675104735, -314.9967657858571783 ) ) ;
#30203=CARTESIAN_POINT ( 'NONE',  ( 776.2433038121456548, -324.8965053807775121, -374.8207195650711014 ) ) ;
#30204=CARTESIAN_POINT ( 'NONE',  ( 745.7998596910086917, -101.3618753856929544, -332.5602148656461168 ) ) ;
#30206=CARTESIAN_POINT ( 'NONE',  ( 763.0537975583475827, -336.4527844766012095, -371.0346526505627480 ) ) ;
#30210=CARTESIAN_POINT ( 'NONE',  ( 781.2497674668890113, -108.3510508353236759, -375.3608509340180603 ) ) ;
#30217=CARTESIAN_POINT ( 'NONE',  ( 772.3691319403857278, 0.7398582555850804487, -315.8894580844506663 ) ) ;
#30219=CARTESIAN_POINT ( 'NONE',  ( 771.2368401574024119, -421.4419599262317888, -374.2805881961240857 ) ) ;
#30222=CARTESIAN_POINT ( 'NONE',  ( 745.5313806188320314, -375.2817908451523294, -333.7943932421247268 ) ) ;
#30226=CARTESIAN_POINT ( 'NONE',  ( 766.0291762391763086, -202.9181544815164386, -360.7704444035551319 ) ) ;
#30227=CARTESIAN_POINT ( 'NONE',  ( 764.8639956371174549, -224.0891481129653187, -319.7806653035542013 ) ) ;
#30228=CARTESIAN_POINT ( 'NONE',  ( 801.9419747391806368, -402.4527844766010389, -351.9812246680014027 ) ) ;
#30231=CARTESIAN_POINT ( 'NONE',  ( 759.9864689768902508, -98.08914811296568814, -354.9819416627836404 ) ) ;
#30233=CARTESIAN_POINT ( 'NONE',  ( 779.9999999999990905, 18.49609980828599376, -309.9999999999999432 ) ) ;
#30235=DIRECTION ( 'NONE',  ( 0.000000000000000000, 0.000000000000000000, 1.000000000000000000 ) ) ;
#30239=CARTESIAN_POINT ( 'NONE',  ( 796.2681130854250569, -462.7578698805381237, -371.0719813302654870 ) ) ;
#30240=CARTESIAN_POINT ( 'NONE',  ( 782.5225473063383106, -22.27096629478410605, -375.2698199232970637 ) ) ;
#30242=CARTESIAN_POINT ( 'NONE',  ( 795.1360043628807261, -404.0891481129646081, -360.2193346964456282 ) ) ;
#30243=CARTESIAN_POINT ( 'NONE',  ( 795.1360043628808398, -20.08914811296593328, -360.2193346964456282 ) ) ;
#30246=CARTESIAN_POINT ( 'NONE',  ( 773.4516893846965786, -283.6454272087889308, -315.8398074228977066 ) ) ;
#30247=CARTESIAN_POINT ( 'NONE',  ( 782.5225473063381969, -166.2709662947835909, -375.2698199232970637 ) ) ;
#30252=CARTESIAN_POINT ( 'NONE',  ( 747.3154664389472828, -235.9874144716868898, -326.4474001241230781 ) ) ;
#30256=CARTESIAN_POINT ( 'NONE',  ( 762.1405469898971887, -337.5436935675102177, -357.8594530101015607 ) ) ;
#30258=CARTESIAN_POINT ( 'NONE',  ( 746.4236121716829757, -111.8272453906076151, -328.8385539511384650 ) ) ;
#30259=CARTESIAN_POINT ( 'NONE',  ( 769.1273215169530886, -142.7146871989599219, -317.4527132478988847 ) ) ;
#30262=CARTESIAN_POINT ( 'NONE',  ( 764.8639956371174549, -56.08914811296580893, -319.7806653035542013 ) ) ;
#30263=CARTESIAN_POINT ( 'NONE',  ( 803.2186876482843445, -151.9874144716871740, -350.0220218866286928 ) ) ;
#30264=CARTESIAN_POINT ( 'NONE',  ( 765.0180583372156207, -120.9982390220565378, -360.0135310231089534 ) ) ;
#30267=CARTESIAN_POINT ( 'NONE',  ( 813.9316612368132837, -7.441959926233078448, -348.6739635108323228 ) ) ;
#30272=CARTESIAN_POINT ( 'NONE',  ( 788.6739635108323228, -271.6454272087889876, -373.9316612368139090 ) ) ;
#30279=CARTESIAN_POINT ( 'NONE',  ( 793.0897708529556667, -126.5545181178803205, -361.3366627262616362 ) ) ;
#30280=CARTESIAN_POINT ( 'NONE',  ( 785.3687786644884454, -107.3618753856928976, -315.3201227861279676 ) ) ;
#30281=CARTESIAN_POINT ( 'NONE',  ( 803.6646147819162707, -305.9073299311468190, -348.8264449731211130 ) ) ;
#30283=CARTESIAN_POINT ( 'NONE',  ( 797.6776695296629214, -427.5436935675101040, -357.6776695296636603 ) ) ;
#30284=CARTESIAN_POINT ( 'NONE',  ( 804.6798772138708955, -87.72551174932937101, -334.6312213355107019 ) ) ;
#30291=CARTESIAN_POINT ( 'NONE',  ( 802.2119215644370342, -342.0090635724251342, -367.5423716828165084 ) ) ;
#30292=CARTESIAN_POINT ( 'NONE',  ( 804.9363028652555840, -304.2709662947832499, -338.2165204200192079 ) ) ;
#30293=CARTESIAN_POINT ( 'NONE',  ( 799.9999999999993179, 205.0000000000000568, -350.0000000000000000 ) ) ;
#30294=CARTESIAN_POINT ( 'NONE',  ( 755.5913626894240451, -181.6454272087892434, -346.6156483768012890 ) ) ;
#30297=CARTESIAN_POINT ( 'NONE',  ( 746.8695393053151292, -365.9073299311466485, -327.6429770376306578 ) ) ;
#30303=CARTESIAN_POINT ( 'NONE',  ( 767.7687537140311633, -23.90732993114773919, -372.7932403749916830 ) ) ;
#30304=CARTESIAN_POINT ( 'NONE',  ( 756.5762568750052424, -243.1800572038743269, -348.7366044899774238 ) ) ;
#30306=CARTESIAN_POINT ( 'NONE',  ( 772.4999999999993179, -462.9681489794447202, -270.0000000000000568 ) ) ;
#30309=CARTESIAN_POINT ( 'NONE',  ( 783.0433043558608688, -48.89650538077840025, -315.1538015810313027 ) ) ;
#30316=CARTESIAN_POINT ( 'NONE',  ( 804.6798772138708955, -39.72551174932951312, -334.6312213355107019 ) ) ;
#30319=CARTESIAN_POINT ( 'NONE',  ( 757.2208543904082489, -328.7146871989592682, -350.9844846989624330 ) ) ;
#30322=CARTESIAN_POINT ( 'NONE',  ( 746.7653713866222915, -353.2601417444137724, -351.0478386215610271 ) ) ;
#30324=ORIENTED_EDGE ( 'NONE', *, *, #14574, .F. ) ;
#30326=EDGE_LOOP ( 'NONE', ( #11883, #18043, #36660, #2849 ) ) ;
#30327=CARTESIAN_POINT ( 'NONE',  ( 787.4397851343537695, -213.7255117493289731, -374.2001403089903988 ) ) ;
#30330=CARTESIAN_POINT ( 'NONE',  ( 804.9363028652555840, -160.2709662947836762, -338.2165204200192079 ) ) ;
#30333=CARTESIAN_POINT ( 'NONE',  ( 764.8639956371174549, -320.0891481129648355, -319.7806653035542013 ) ) ;
#30334=CARTESIAN_POINT ( 'NONE',  ( 764.8639956371174549, 15.91085188703394238, -319.7806653035542013 ) ) ;
#30339=CARTESIAN_POINT ( 'NONE',  ( 779.9999999999992042, -452.9681489794448339, -339.9999999999999432 ) ) ;
#30342=CARTESIAN_POINT ( 'NONE',  ( 766.0291762391763086, -442.9181544815157849, -360.7704444035551319 ) ) ;
#30345=ORIENTED_EDGE ( 'NONE', *, *, #8376, .T. ) ;
#30346=CARTESIAN_POINT ( 'NONE',  ( 811.3240766477731540, -244.3726999360617924, -355.6651683502462902 ) ) ;
#30347=VECTOR ( 'NONE', #33939, 1000.000000000000000 ) ;
#30350=CARTESIAN_POINT ( 'NONE',  ( 774.6858677611749044, -177.7255117493290868, -315.5713283507209894 ) ) ;
#30351=CARTESIAN_POINT ( 'NONE',  ( 790.8726784830453198, -370.7146871989592114, -362.5472867521010585 ) ) ;
#30353=CARTESIAN_POINT ( 'NONE',  ( 762.1177392798416577, -234.5545181178799794, -309.8865473780659272 ) ) ;
#30356=CARTESIAN_POINT ( 'NONE',  ( 766.9102291470427417, -90.55451811788041994, -318.6633372737382501 ) ) ;
#30359=CARTESIAN_POINT ( 'NONE',  ( 769.1273215169530886, -430.7146871989590409, -317.4527132478988847 ) ) ;
#30360=CARTESIAN_POINT ( 'NONE',  ( 804.7487373415286811, -283.5436935675105019, -364.7487373415288516 ) ) ;
#30362=CARTESIAN_POINT ( 'NONE',  ( 779.9999999999992042, 16.45630643248849267, -339.9999999999999432 ) ) ;
#30364=CARTESIAN_POINT ( 'NONE',  ( 804.4286716492782716, -65.36187538569306810, -345.3141322388244703 ) ) ;
#30367=CARTESIAN_POINT ( 'NONE',  ( 773.7943932421234194, -167.8055962898689586, -305.5313806188329409 ) ) ;
#30369=CARTESIAN_POINT ( 'NONE',  ( 814.5518280994195948, -399.7255117493283478, -332.4837098697145734 ) ) ;
#30374=CARTESIAN_POINT ( 'NONE',  ( 791.9812246680005501, -380.6346026584192828, -361.9419747391813189 ) ) ;
#30381=CARTESIAN_POINT ( 'NONE',  ( 780.5290396650775619, -228.3510508353232922, -365.2837595273619513 ) ) ;
#30384=CARTESIAN_POINT ( 'NONE',  ( 776.2433038121456548, -276.8965053807776258, -374.8207195650711014 ) ) ;
#30389=CARTESIAN_POINT ( 'NONE',  ( 794.9819416627830151, -180.9982390220563389, -319.9864689768909898 ) ) ;
#30391=CARTESIAN_POINT ( 'NONE',  ( 787.4397851343537695, -93.72551174932934259, -374.2001403089903988 ) ) ;
#30392=CARTESIAN_POINT ( 'NONE',  ( 792.1044303154646968, -84.45278447660207632, -317.8323909638837677 ) ) ;
#30394=CARTESIAN_POINT ( 'NONE',  ( 766.9102291470427417, -18.55451811788065797, -318.6633372737382501 ) ) ;
#30396=CARTESIAN_POINT ( 'NONE',  ( 757.4527132478984868, -352.3726999360614514, -329.1273215169538844 ) ) ;
#30402=CARTESIAN_POINT ( 'NONE',  ( 804.4086373105744769, -313.6454272087888171, -333.3843516231986541 ) ) ;
#30403=CARTESIAN_POINT ( 'NONE',  ( 802.1676090361156639, -326.6346026584193396, -327.8955696845344505 ) ) ;
#30405=CARTESIAN_POINT ( 'NONE',  ( 745.7194118038753459, -133.6454272087893571, -348.7631598425976449 ) ) ;
#30409=CARTESIAN_POINT ( 'NONE',  ( 795.9930595647434757, -267.0783235625958696, -320.7433823573372820 ) ) ;
#30410=CARTESIAN_POINT ( 'NONE',  ( 773.7305795820266212, -105.2817908451530968, -374.8230680027170365 ) ) ;
#30411=CARTESIAN_POINT ( 'NONE',  ( 772.4999999999993179, -512.9681489794448908, -329.9999999999999432 ) ) ;
#30416=CARTESIAN_POINT ( 'NONE',  ( 800.9747183278959710, -180.9982390220563389, -311.9810565676471583 ) ) ;
#30419=CARTESIAN_POINT ( 'NONE',  ( 767.7687537140311633, -287.9073299311468759, -372.7932403749916830 ) ) ;
#30422=VERTEX_POINT ( 'NONE', #5001 ) ;
#30424=CARTESIAN_POINT ( 'NONE',  ( 791.1614460488616487, -347.2601417444138860, -373.5763878283158874 ) ) ;
#30425=CARTESIAN_POINT ( 'NONE',  ( 749.2812353651451076, -102.4527844766020337, -323.2262854647983090 ) ) ;
#30427=CARTESIAN_POINT ( 'NONE',  ( 810.7187646348534145, -378.4527844766011526, -356.7737145352016341 ) ) ;
#30433=CARTESIAN_POINT ( 'NONE',  ( 754.0944755984390895, -111.6237781080509279, -364.1009440267246760 ) ) ;
#30434=LINE ( 'NONE', #6181, #462 ) ;
#30437=ORIENTED_EDGE ( 'NONE', *, *, #22046, .T. ) ;
#30439=CARTESIAN_POINT ( 'NONE',  ( 776.2433038121456548, -420.8965053807772279, -374.8207195650711014 ) ) ;
#30442=CARTESIAN_POINT ( 'NONE',  ( 778.1981804954714335, -178.2709662947835625, -314.8072714833589885 ) ) ;
#30443=CARTESIAN_POINT ( 'NONE',  ( 804.1009440267234822, -383.4636090269704596, -314.0944755984392600 ) ) ;
#30446=CARTESIAN_POINT ( 'NONE',  ( 755.1538015810308480, -230.1908817542436338, -343.0433043558613804 ) ) ;
#30447=CARTESIAN_POINT ( 'NONE',  ( 788.7366044899766848, -203.9073299311471885, -316.5762568750059813 ) ) ;
#30448=CARTESIAN_POINT ( 'NONE',  ( 755.5713283507202505, -413.3618753856920307, -334.6858677611754729 ) ) ;
#30451=CARTESIAN_POINT ( 'NONE',  ( 756.3353852180819104, -101.9073299311474727, -331.1735550268788302 ) ) ;
#30460=CARTESIAN_POINT ( 'NONE',  ( 752.7379699480933368, -444.0090635724249069, -361.9858362298580232 ) ) ;
#30462=CARTESIAN_POINT ( 'NONE',  ( 814.2001403089898304, -65.36187538569306810, -347.4397851343538264 ) ) ;
#30465=CARTESIAN_POINT ( 'NONE',  ( 767.8955696845333705, -432.4527844766008684, -362.1676090361162323 ) ) ;
#30466=CARTESIAN_POINT ( 'NONE',  ( 758.0580252608178853, -54.45278447660219001, -328.0187753319985404 ) ) ;
#30469=CARTESIAN_POINT ( 'NONE',  ( 758.4439275373578084, -300.5545181178797520, -353.2243759319684386 ) ) ;
#30470=CARTESIAN_POINT ( 'NONE',  ( 767.7687537140311633, -191.9073299311471885, -372.7932403749916830 ) ) ;
#30473=CARTESIAN_POINT ( 'NONE',  ( 772.4999999999993179, -462.9681489794448339, -370.0000000000000568 ) ) ;
#30475=CARTESIAN_POINT ( 'NONE',  ( 771.2368401574024119, -229.4419599262323572, -374.2805881961240857 ) ) ;
#30478=CARTESIAN_POINT ( 'NONE',  ( 758.8095938919642549, -296.0891481129650629, -311.6929314249763365 ) ) ;
#30482=CARTESIAN_POINT ( 'NONE',  ( 771.2633955100217236, -335.9073299311468190, -363.4237431249939618 ) ) ;
#30484=CARTESIAN_POINT ( 'NONE',  ( 755.8990559732751535, -83.46360902697136908, -365.9055244015606831 ) ) ;
#30485=CARTESIAN_POINT ( 'NONE',  ( 783.0433043558608688, -168.8965053807780237, -315.1538015810313027 ) ) ;
#30489=CARTESIAN_POINT ( 'NONE',  ( 756.3353852180819104, -53.90732993114765037, -331.1735550268788302 ) ) ;
#30490=CARTESIAN_POINT ( 'NONE',  ( 805.1016975059191054, -174.8965053807779952, -343.0745993439771837 ) ) ;
#30492=CARTESIAN_POINT ( 'NONE',  ( 781.2497674668890113, -12.35105083532396897, -375.3608509340180603 ) ) ;
#30500=CARTESIAN_POINT ( 'NONE',  ( 791.0478386215596629, -261.8272453906071746, -306.7653713866226326 ) ) ;
#30507=CARTESIAN_POINT ( 'NONE',  ( 755.8894580844503253, -111.8272453906076151, -332.3691319403863531 ) ) ;
#30508=CARTESIAN_POINT ( 'NONE',  ( 755.3201227861273992, -99.72551174932928575, -345.3687786644892981 ) ) ;
#30509=CARTESIAN_POINT ( 'NONE',  ( 805.1927285166399315, -328.8164208402375834, -341.8018195045277707 ) ) ;
#30511=CARTESIAN_POINT ( 'NONE',  ( 764.8639956371174549, -440.0891481129644944, -319.7806653035542013 ) ) ;
#30519=CARTESIAN_POINT ( 'NONE',  ( 760.0363995740630116, -346.9181544815160123, -368.7758568127991907 ) ) ;
#30521=CARTESIAN_POINT ( 'NONE',  ( 803.6646147819161570, -329.9073299311467053, -348.8264449731210561 ) ) ;
#30523=CARTESIAN_POINT ( 'NONE',  ( 800.9840315886518738, -172.9181544815165239, -354.1144889064786412 ) ) ;
#30529=CARTESIAN_POINT ( 'NONE',  ( 787.5162901302840055, -371.3618753856920307, -305.4481719005793252 ) ) ;
#30535=CARTESIAN_POINT ( 'NONE',  ( 772.4837098697144029, -23.36187538569318889, -374.5518280994205611 ) ) ;
#30536=CARTESIAN_POINT ( 'NONE',  ( 785.3141322388236176, -237.7255117493289163, -364.4286716492789537 ) ) ;
#30540=CARTESIAN_POINT ( 'NONE',  ( 755.0488828828309806, -65.80559628986925702, -344.1219089521771934 ) ) ;
#30549=CARTESIAN_POINT ( 'NONE',  ( 758.6633372737375112, -356.5328690171410813, -326.9102291470432533 ) ) ;
#30552=CARTESIAN_POINT ( 'NONE',  ( 758.0141637701419768, -351.0783235625955854, -367.2620300519063790 ) ) ;
#30557=CARTESIAN_POINT ( 'NONE',  ( 767.6429770376289525, -201.1800572038744690, -306.8695393053162093 ) ) ;
#30561=CARTESIAN_POINT ( 'NONE',  ( 791.9812246680005501, -212.6346026584198796, -361.9419747391813189 ) ) ;
#30564=CARTESIAN_POINT ( 'NONE',  ( 797.6776695296629214, -331.5436935675104451, -357.6776695296636603 ) ) ;
#30565=CARTESIAN_POINT ( 'NONE',  ( 788.7366044899766848, 12.09267006885214180, -316.5762568750059813 ) ) ;
#30568=CARTESIAN_POINT ( 'NONE',  ( 779.9999999999992042, -462.9681489794448339, -309.9999999999998863 ) ) ;
#30570=DIRECTION ( 'NONE',  ( 0.000000000000000000, 0.000000000000000000, -1.000000000000000000 ) ) ;
#30573=CARTESIAN_POINT ( 'NONE',  ( 781.7834795799800531, 13.18357915976123174, -315.0636971347436202 ) ) ;
#30577=CARTESIAN_POINT ( 'NONE',  ( 776.2046728542105711, -236.1908817542436338, -304.8212110874238761 ) ) ;
#30581=CARTESIAN_POINT ( 'NONE',  ( 764.8639956371174549, -176.0891481129653755, -319.7806653035542013 ) ) ;
#30582=CARTESIAN_POINT ( 'NONE',  ( 756.7813123517142913, -355.9874144716865203, -329.9779781133712504 ) ) ;
#30583=CARTESIAN_POINT ( 'NONE',  ( 788.6739635108323228, -247.6454272087890160, -373.9316612368139090 ) ) ;
#30586=CARTESIAN_POINT ( 'NONE',  ( 766.0291762391763086, -82.91815448151682233, -360.7704444035551319 ) ) ;
#30587=EDGE_CURVE ( 'NONE', #2036, #1585, #29929, .T. ) ;
#30591=DIRECTION ( 'NONE',  ( 1.000000000000000000, 0.000000000000000000, -0.000000000000000000 ) ) ;
#30592=CARTESIAN_POINT ( 'NONE',  ( 779.4709603349208464, -432.3510508353226669, -314.7162404726379918 ) ) ;
#30593=CARTESIAN_POINT ( 'NONE',  ( 767.6429770376291799, -273.1800572038742985, -306.8695393053162093 ) ) ;
#30596=CARTESIAN_POINT ( 'NONE',  ( 795.1360043628807261, -44.08914811296584446, -360.2193346964456282 ) ) ;
#30598=CARTESIAN_POINT ( 'NONE',  ( 805.9055244015594326, -171.6237781080507432, -315.8990559732753240 ) ) ;
#30600=CARTESIAN_POINT ( 'NONE',  ( 755.2512626584698410, -415.5436935675102177, -315.2512626584710915 ) ) ;
#30607=CARTESIAN_POINT ( 'NONE',  ( 805.1927285166397041, -424.8164208402372992, -341.8018195045277707 ) ) ;
#30608=AXIS2_PLACEMENT_3D ( 'NONE', #13674, #31218, #6512 ) ;
#30614=ORIENTED_EDGE ( 'NONE', *, *, #35064, .F. ) ;
#30615=CARTESIAN_POINT ( 'NONE',  ( 758.6633372737375112, -260.5328690171413086, -326.9102291470432533 ) ) ;
#30618=CARTESIAN_POINT ( 'NONE',  ( 778.7502325331095108, -264.3510508353232353, -304.6391490659818828 ) ) ;
#30619=DIRECTION ( 'NONE',  ( -1.000000000000000000, -0.000000000000000000, -0.000000000000000000 ) ) ;
#30625=CARTESIAN_POINT ( 'NONE',  ( 785.3687786644884454, -179.3618753856927128, -315.3201227861279676 ) ) ;
#30628=CARTESIAN_POINT ( 'NONE',  ( 758.8095938919642549, -104.0891481129656881, -311.6929314249763365 ) ) ;
#30630=CARTESIAN_POINT ( 'NONE',  ( 785.3687786644885591, -107.3618753856928976, -315.3201227861280813 ) ) ;
#30631=VERTEX_POINT ( 'NONE', #22980 ) ;
#30632=CARTESIAN_POINT ( 'NONE',  ( 779.4763451958990572, -32.73633629969879877, -365.0264073115438919 ) ) ;
#30633=CARTESIAN_POINT ( 'NONE',  ( 804.1105419155481968, -363.8272453906068336, -347.6308680596136469 ) ) ;
#30634=EDGE_CURVE ( 'NONE', #35055, #15183, #7020, .T. ) ;
#30642=CARTESIAN_POINT ( 'NONE',  ( 793.0897708529556667, -366.5545181178795815, -361.3366627262616362 ) ) ;
#30643=CARTESIAN_POINT ( 'NONE',  ( 801.9419747391806368, -330.4527844766013231, -351.9812246680014027 ) ) ;
#30644=CARTESIAN_POINT ( 'NONE',  ( 744.6391490659812007, -134.7363362996984790, -338.7502325331110455 ) ) ;
#30649=CARTESIAN_POINT ( 'NONE',  ( 778.7629533639073998, -104.7363362996985785, -375.0009284576466371 ) ) ;
#30652=EDGE_CURVE ( 'NONE', #14643, #20167, #26681, .T. ) ;
#30660=CARTESIAN_POINT ( 'NONE',  ( 745.0891759886404770, -292.2709662947831930, -342.4968714119734159 ) ) ;
#30662=DIRECTION ( 'NONE',  ( 0.000000000000000000, -1.000000000000000000, 0.000000000000000000 ) ) ;
#30668=CARTESIAN_POINT ( 'NONE',  ( 751.2241431872005251, -376.1692326535046504, -359.9636004259367610 ) ) ;
#30669=CARTESIAN_POINT ( 'NONE',  ( 787.4397851343537695, -117.7255117493292715, -374.2001403089903988 ) ) ;
#30671=CARTESIAN_POINT ( 'NONE',  ( 808.0189434323515343, -374.0891481129647786, -319.0252816721025511 ) ) ;
#30676=CARTESIAN_POINT ( 'NONE',  ( 761.9338519418445230, -158.5328690171417065, -370.4231160770881957 ) ) ;
#30682=CARTESIAN_POINT ( 'NONE',  ( 804.9511171171677688, -5.805596289869448867, -335.8780910478229202 ) ) ;
#30684=CARTESIAN_POINT ( 'NONE',  ( 777.5031285880264704, 1.183579159761269040, -374.9108240113588408 ) ) ;
#30687=CARTESIAN_POINT ( 'NONE',  ( 800.0135310231082713, -182.0891481129654323, -325.0180583372163028 ) ) ;
#30688=CARTESIAN_POINT ( 'NONE',  ( 757.7880784355613741, -426.0090635724247932, -312.4576283171834916 ) ) ;
#30691=CARTESIAN_POINT ( 'NONE',  ( 774.6858677611749044, -249.7255117493288594, -315.5713283507209894 ) ) ;
#30696=CARTESIAN_POINT ( 'NONE',  ( 796.9571628226829034, -215.4636090269709712, -321.2382568024804641 ) ) ;
#30697=CARTESIAN_POINT ( 'NONE',  ( 755.5713283507202505, -221.3618753856925707, -334.6858677611754729 ) ) ;
#30698=CARTESIAN_POINT ( 'NONE',  ( 759.9864689768902508, -410.0891481129647218, -354.9819416627836404 ) ) ;
#30702=CARTESIAN_POINT ( 'NONE',  ( 795.2725662613897839, 16.45630643248849267, -314.1785221222716586 ) ) ;
#30703=CARTESIAN_POINT ( 'NONE',  ( 805.6418435158337843, -5.463609026971610660, -363.8556311672236916 ) ) ;
#30708=CARTESIAN_POINT ( 'NONE',  ( 805.6418435158337843, -437.4636090269703459, -363.8556311672236916 ) ) ;
#30709=CARTESIAN_POINT ( 'NONE',  ( 745.7998596910086917, -53.36187538569310362, -332.5602148656461168 ) ) ;
#30712=CARTESIAN_POINT ( 'NONE',  ( 785.3141322388236176, -429.7255117493282910, -364.4286716492789537 ) ) ;
#30713=CARTESIAN_POINT ( 'NONE',  ( 756.5762568750052424, -27.18005720387500901, -348.7366044899774238 ) ) ;
#30716=CARTESIAN_POINT ( 'NONE',  ( 790.0220218866281812, -295.0999726633343698, -363.2186876482849129 ) ) ;
#30717=CARTESIAN_POINT ( 'NONE',  ( 777.5031285880264704, -214.8164208402380666, -374.9108240113588408 ) ) ;
#30724=CARTESIAN_POINT ( 'NONE',  ( 815.1787889125755555, -246.8965053807777679, -343.7953271457877804 ) ) ;
#30726=CARTESIAN_POINT ( 'NONE',  ( 772.5602148656447525, -273.7255117493288026, -305.7998596910095443 ) ) ;
#30730=CARTESIAN_POINT ( 'NONE',  ( 781.8018195045266339, -358.2709662947829088, -365.1927285166406705 ) ) ;
#30732=CARTESIAN_POINT ( 'NONE',  ( 752.4576283171824116, -45.07832356259660145, -317.7880784355627952 ) ) ;
#30733=CARTESIAN_POINT ( 'NONE',  ( 780.5290396650775619, -156.3510508353235480, -365.2837595273619513 ) ) ;
#30737=CARTESIAN_POINT ( 'NONE',  ( 781.8018195045266339, -46.27096629478404566, -365.1927285166406705 ) ) ;
#30738=CARTESIAN_POINT ( 'NONE',  ( 804.1601925771018387, -175.4419599262325562, -346.5483106153029098 ) ) ;
#30740=CARTESIAN_POINT ( 'NONE',  ( 758.0141637701419768, -15.07832356259669560, -367.2620300519063790 ) ) ;
#30745=CARTESIAN_POINT ( 'NONE',  ( 786.2694204179717872, -261.2817908451526705, -305.1769319972829067 ) ) ;
#30747=VECTOR ( 'NONE', #29521, 1000.000000000000000 ) ;
#30752=CARTESIAN_POINT ( 'NONE',  ( 763.0428371773158460, -131.4636090269711985, -358.7617431975195359 ) ) ;
#30754=CARTESIAN_POINT ( 'NONE',  ( 791.9812246680005501, -116.6346026584201780, -361.9419747391813189 ) ) ;
#30755=CARTESIAN_POINT ( 'NONE',  ( 804.4286716492782716, -329.3618753856922581, -345.3141322388244703 ) ) ;
#30757=CARTESIAN_POINT ( 'NONE',  ( 755.5713283507202505, -413.3618753856920307, -334.6858677611754729 ) ) ;
#30762=AXIS2_PLACEMENT_3D ( 'NONE', #14234, #37804, #28303 ) ;
#30766=CARTESIAN_POINT ( 'NONE',  ( 771.3260364891663130, -331.6454272087888171, -306.0683387631859773 ) ) ;
#30768=CARTESIAN_POINT ( 'NONE',  ( 804.6798772138708955, -327.7255117493285184, -334.6312213355107019 ) ) ;
#30770=CARTESIAN_POINT ( 'NONE',  ( 766.0291762391763086, -178.9181544815165239, -360.7704444035551319 ) ) ;
#30773=CARTESIAN_POINT ( 'NONE',  ( 796.9462024416508257, -396.4527844766010958, -308.9653473494370246 ) ) ;
#30779=CARTESIAN_POINT ( 'NONE',  ( 751.9810565676468741, -26.08914811296592262, -360.9747183278973921 ) ) ;
#30780=CARTESIAN_POINT ( 'NONE',  ( 765.0180583372156207, -264.9982390220561115, -360.0135310231089534 ) ) ;
#30784=CARTESIAN_POINT ( 'NONE',  ( 779.4709603349208464, -48.35105083532386061, -314.7162404726379918 ) ) ;
#30791=CARTESIAN_POINT ( 'NONE',  ( 756.3353852180819104, -53.90732993114765037, -331.1735550268788302 ) ) ;
#30792=CARTESIAN_POINT ( 'NONE',  ( 805.1016975059191054, -366.8965053807773984, -343.0745993439771837 ) ) ;
#30795=CARTESIAN_POINT ( 'NONE',  ( 768.8385539511368734, -359.2601417444137724, -306.4236121716840557 ) ) ;
#30800=CARTESIAN_POINT ( 'NONE',  ( 799.9999999999993179, 205.0000000000000568, -319.9999999999999432 ) ) ;
#30801=CARTESIAN_POINT ( 'NONE',  ( 745.7998596910086917, -221.3618753856925707, -332.5602148656461168 ) ) ;
#30804=CARTESIAN_POINT ( 'NONE',  ( 754.8072714833583632, -196.8164208402380950, -338.1981804954721156 ) ) ;
#30806=CARTESIAN_POINT ( 'NONE',  ( 803.6646147819161570, -329.9073299311467053, -348.8264449731210561 ) ) ;
#30807=CARTESIAN_POINT ( 'NONE',  ( 798.5707757039680246, -461.4636090269701754, -356.7845633553585003 ) ) ;
#30811=LINE ( 'NONE', #44905, #23540 ) ;
#30813=CARTESIAN_POINT ( 'NONE',  ( 778.1981804954714335, 13.72903370521577138, -314.8072714833589885 ) ) ;
#30816=CARTESIAN_POINT ( 'NONE',  ( 752.7379699480933368, -252.0090635724254184, -361.9858362298580232 ) ) ;
#30820=CARTESIAN_POINT ( 'NONE',  ( 803.4237431249931660, -207.1800572038744406, -331.2633955100225194 ) ) ;
#30821=CARTESIAN_POINT ( 'NONE',  ( 756.1348686366196716, -377.2601417444137724, -347.5531968255698416 ) ) ;
#30822=CARTESIAN_POINT ( 'NONE',  ( 812.3518521366052028, -241.0999726633345119, -326.5853460496235243 ) ) ;
#30825=CARTESIAN_POINT ( 'NONE',  ( 796.1575198192839480, -78.00906357242591582, -359.4546378042384163 ) ) ;
#30829=CARTESIAN_POINT ( 'NONE',  ( 787.4397851343537695, -261.7255117493288026, -374.2001403089903988 ) ) ;
#30832=CARTESIAN_POINT ( 'NONE',  ( 794.9819416627830151, -36.99823902205679360, -319.9864689768909898 ) ) ;
#30834=CARTESIAN_POINT ( 'NONE',  ( 745.1769319972822814, -161.8055962898689870, -346.2694204179732083 ) ) ;
#30836=CARTESIAN_POINT ( 'NONE',  ( 814.9108240113580450, -424.2709662947829088, -337.5031285880265273 ) ) ;
#30840=CARTESIAN_POINT ( 'NONE',  ( 781.7834795799800531, -418.8164208402374129, -315.0636971347436202 ) ) ;
#30847=CARTESIAN_POINT ( 'NONE',  ( 804.1601925771018387, -271.4419599262321867, -346.5483106153029098 ) ) ;
#30848=CARTESIAN_POINT ( 'NONE',  ( 756.3353852180819104, -125.9073299311474159, -331.1735550268788302 ) ) ;
#30850=CARTESIAN_POINT ( 'NONE',  ( 813.2346286133761168, -269.2601417444139997, -328.9521613784389160 ) ) ;
#30856=CARTESIAN_POINT ( 'NONE',  ( 798.7617431975189675, -27.62377810805120149, -323.0428371773161871 ) ) ;
#30857=CARTESIAN_POINT ( 'NONE',  ( 768.0187753319979720, -176.6346026584199933, -318.0580252608186242 ) ) ;
#30860=CARTESIAN_POINT ( 'NONE',  ( 810.7187646348534145, -114.4527844766020053, -356.7737145352016341 ) ) ;
#30861=CARTESIAN_POINT ( 'NONE',  ( 791.9812246680005501, -116.6346026584201780, -361.9419747391813189 ) ) ;
#30863=CARTESIAN_POINT ( 'NONE',  ( 769.0155153010367712, -34.37269993606243901, -362.7791456095907279 ) ) ;
#30864=CARTESIAN_POINT ( 'NONE',  ( 775.8780910478218402, -369.2817908451523294, -364.9511171171680530 ) ) ;
#30870=CARTESIAN_POINT ( 'NONE',  ( 779.4763451958990572, -344.7363362996978253, -365.0264073115438919 ) ) ;
#30871=CARTESIAN_POINT ( 'NONE',  ( 755.5713283507202505, -365.3618753856920875, -334.6858677611754729 ) ) ;
#30872=CARTESIAN_POINT ( 'NONE',  ( 804.1009440267234822, -143.4636090269711701, -314.0944755984392600 ) ) ;
#30876=CARTESIAN_POINT ( 'NONE',  ( 759.2295555964440155, -256.1692326535049915, -353.9708237608231229 ) ) ;
#30878=CARTESIAN_POINT ( 'NONE',  ( 788.6739635108323228, -151.6454272087892718, -373.9316612368139090 ) ) ;
#30885=CARTESIAN_POINT ( 'NONE',  ( 814.9108240113580450, -160.2709662947836762, -337.5031285880265273 ) ) ;
#30889=CARTESIAN_POINT ( 'NONE',  ( 747.2067596250078623, -291.1800572038741848, -352.2312462859687230 ) ) ;
#30895=CARTESIAN_POINT ( 'NONE',  ( 800.1688906516307043, -394.1692326535045368, -369.0717654672308186 ) ) ;
#30896=CARTESIAN_POINT ( 'NONE',  ( 759.0252816721024374, -120.9982390220565378, -368.0189434323527280 ) ) ;
#30899=CARTESIAN_POINT ( 'NONE',  ( 777.4774526936600978, -394.2709662947827951, -304.7301800767027657 ) ) ;
#30904=CARTESIAN_POINT ( 'NONE',  ( 788.7631598425961101, -145.4419599262326699, -305.7194118038759143 ) ) ;
#30912=CARTESIAN_POINT ( 'NONE',  ( 808.3070685750230950, -18.99823902205683979, -361.1904061080339261 ) ) ;
#30916=CARTESIAN_POINT ( 'NONE',  ( 781.2370466360911223, -404.7363362996975980, -304.9990715423533629 ) ) ;
#30918=CARTESIAN_POINT ( 'NONE',  ( 797.6776695296629214, -259.5436935675106156, -357.6776695296636603 ) ) ;
#30922=CARTESIAN_POINT ( 'NONE',  ( 790.9844846989617508, -262.3726999360617924, -317.2208543904092721 ) ) ;
#30923=CARTESIAN_POINT ( 'NONE',  ( 774.6858677611749044, -225.7255117493289163, -315.5713283507209894 ) ) ;
#30924=CARTESIAN_POINT ( 'NONE',  ( 765.0180583372156207, -432.9982390220555999, -360.0135310231089534 ) ) ;
#30931=CARTESIAN_POINT ( 'NONE',  ( 781.2370466360911223, -44.73633629969875614, -304.9990715423533629 ) ) ;
#30937=CARTESIAN_POINT ( 'NONE',  ( 780.5236548040995785, -20.73633629969883430, -314.9735926884559944 ) ) ;
#30938=CARTESIAN_POINT ( 'NONE',  ( 782.4968714119720516, -82.81642084023846451, -305.0891759886411023 ) ) ;
#30940=CARTESIAN_POINT ( 'NONE',  ( 788.8264449731200330, -429.1800572038737869, -363.6646147819171233 ) ) ;
#30941=CARTESIAN_POINT ( 'NONE',  ( 800.0135310231082713, -38.08914811296587999, -325.0180583372163028 ) ) ;
#30944=CARTESIAN_POINT ( 'NONE',  ( 749.2812353651451076, -198.4527844766017495, -323.2262854647983090 ) ) ;
#30949=CARTESIAN_POINT ( 'NONE',  ( 756.1443688327750579, -261.6237781080504305, -314.3581564841659315 ) ) ;
#30952=CARTESIAN_POINT ( 'NONE',  ( 815.2698199232961542, -280.8164208402378677, -342.5225473063383106 ) ) ;
#30953=CARTESIAN_POINT ( 'NONE',  ( 759.9999999999992042, -512.9681489794448908, -309.9999999999998863 ) ) ;
#30956=CARTESIAN_POINT ( 'NONE',  ( 765.0180583372156207, -360.9982390220557704, -360.0135310231089534 ) ) ;
#30957=ADVANCED_FACE ( 'NONE', ( #45160, #27595 ), #27836, .F. ) ;
#30959=CARTESIAN_POINT ( 'NONE',  ( 749.8865473780648472, -44.53286901714205470, -322.1177392798429082 ) ) ;
#30960=CARTESIAN_POINT ( 'NONE',  ( 798.7617431975189675, -147.6237781080508285, -323.0428371773161871 ) ) ;
#30963=ORIENTED_EDGE ( 'NONE', *, *, #30634, .F. ) ;
#30964=CARTESIAN_POINT ( 'NONE',  ( 759.9864689768902508, -74.08914811296577341, -354.9819416627836404 ) ) ;
#30965=CARTESIAN_POINT ( 'NONE',  ( 795.9930595647434757, -171.0783235625962106, -320.7433823573372820 ) ) ;
#30967=CARTESIAN_POINT ( 'NONE',  ( 778.7502325331095108, -0.3510508353240099355, -304.6391490659818828 ) ) ;
#30972=CARTESIAN_POINT ( 'NONE',  ( 778.7629533639073998, -296.7363362996979390, -375.0009284576466371 ) ) ;
#30976=CARTESIAN_POINT ( 'NONE',  ( 780.5236548040995785, -164.7363362996983938, -314.9735926884559944 ) ) ;
#30977=CARTESIAN_POINT ( 'NONE',  ( 754.8072714833581358, -124.8164208402383508, -338.1981804954720587 ) ) ;
#30978=CARTESIAN_POINT ( 'NONE',  ( 792.1044303154646968, -324.4527844766013231, -317.8323909638837677 ) ) ;
#30980=CARTESIAN_POINT ( 'NONE',  ( 758.0580252608178853, -414.4527844766010389, -328.0187753319985404 ) ) ;
#30987=CARTESIAN_POINT ( 'NONE',  ( 768.9521613784389729, -345.8272453906069472, -373.2346286133773106 ) ) ;
#30989=CARTESIAN_POINT ( 'NONE',  ( 794.9819416627830151, -324.9982390220559409, -319.9864689768909898 ) ) ;
#30991=CARTESIAN_POINT ( 'NONE',  ( 760.7433823573367135, -180.0090635724255890, -355.9930595647440441 ) ) ;
#30994=CARTESIAN_POINT ( 'NONE',  ( 748.9653473494365699, -386.6346026584192828, -356.9462024416520762 ) ) ;
#31000=CARTESIAN_POINT ( 'NONE',  ( 811.0346526505616112, -14.63460265842049424, -323.0537975583477532 ) ) ;
#31001=CARTESIAN_POINT ( 'NONE',  ( 797.8594530101008786, -253.5436935675104735, -322.1405469898980982 ) ) ;
#31005=CARTESIAN_POINT ( 'NONE',  ( 754.3581564841646241, -17.46360902697157513, -316.1443688327762516 ) ) ;
#31006=CARTESIAN_POINT ( 'NONE',  ( 793.2243759319678702, -50.53286901714203339, -318.4439275373583200 ) ) ;
#31010=PLANE ( 'NONE',  #18146 ) ;
#31013=CARTESIAN_POINT ( 'NONE',  ( 759.7806653035534055, -78.99823902205662307, -324.8639956371180801 ) ) ;
#31014=CARTESIAN_POINT ( 'NONE',  ( 754.9735926884551418, -378.3510508353227806, -340.5236548041000333 ) ) ;
#31018=CARTESIAN_POINT ( 'NONE',  ( 746.0683387631852383, -379.4419599262318457, -331.3260364891676204 ) ) ;
#31023=CARTESIAN_POINT ( 'NONE',  ( 815.2698199232961542, -232.8164208402379245, -342.5225473063383106 ) ) ;
#31026=CARTESIAN_POINT ( 'NONE',  ( 755.0636971347428243, -196.2709662947835909, -341.7834795799807353 ) ) ;
#31028=CARTESIAN_POINT ( 'NONE',  ( 804.9363028652555840, 7.729033705215793582, -338.2165204200192079 ) ) ;
#31032=EDGE_LOOP ( 'NONE', ( #44214, #37835, #43650, #21423, #10168, #39580 ) ) ;
#31033=CARTESIAN_POINT ( 'NONE',  ( 796.1575198192839480, -462.0090635724247932, -359.4546378042384163 ) ) ;
#31036=CARTESIAN_POINT ( 'NONE',  ( 814.2805881961230625, -241.6454272087890729, -331.2368401574024119 ) ) ;
#31039=CARTESIAN_POINT ( 'NONE',  ( 802.1676090361156639, -206.6346026584198512, -327.8955696845344505 ) ) ;
#31040=CARTESIAN_POINT ( 'NONE',  ( 804.9511171171677688, -413.8055962898681059, -335.8780910478229202 ) ) ;
#31041=CARTESIAN_POINT ( 'NONE',  ( 793.5525998758768083, -247.0999726633344835, -372.6845335610516941 ) ) ;
#31044=CARTESIAN_POINT ( 'NONE',  ( 793.9708237608222134, -70.91815448151683654, -319.2295555964448681 ) ) ;
#31047=CARTESIAN_POINT ( 'NONE',  ( 793.2243759319678702, -434.5328690171407970, -318.4439275373583200 ) ) ;
#31048=CARTESIAN_POINT ( 'NONE',  ( 745.4481719005789273, -291.7255117493286320, -347.5162901302853697 ) ) ;
#31051=CARTESIAN_POINT ( 'NONE',  ( 788.8264449731200330, -69.18005720387488111, -363.6646147819171233 ) ) ;
#31053=CARTESIAN_POINT ( 'NONE',  ( 801.9858362298568863, -171.0783235625962106, -312.7379699480935642 ) ) ;
#31055=CARTESIAN_POINT ( 'NONE',  ( 745.4481719005789273, -411.7255117493282910, -347.5162901302853129 ) ) ;
#31060=CARTESIAN_POINT ( 'NONE',  ( 788.8264449731200330, -429.1800572038737869, -363.6646147819171233 ) ) ;
#31066=CARTESIAN_POINT ( 'NONE',  ( 802.7791456095903868, -244.7146871989596093, -329.0155153010375102 ) ) ;
#31068=CARTESIAN_POINT ( 'NONE',  ( 812.6845335610512393, -271.9874144716868045, -353.5525998758768651 ) ) ;
#31073=CARTESIAN_POINT ( 'NONE',  ( 796.7845633553578182, -33.62377810805116951, -358.5707757039688204 ) ) ;
#31074=CARTESIAN_POINT ( 'NONE',  ( 755.0636971347428243, -172.2709662947836478, -341.7834795799807353 ) ) ;
#31076=CARTESIAN_POINT ( 'NONE',  ( 796.7737145352015204, -116.6346026584201780, -370.7187646348536987 ) ) ;
#31078=CARTESIAN_POINT ( 'NONE',  ( 756.5762568750052424, -99.18005720387478164, -348.7366044899774238 ) ) ;
#31079=ORIENTED_EDGE ( 'NONE', *, *, #34008, .F. ) ;
#31080=CARTESIAN_POINT ( 'NONE',  ( 763.0428371773158460, -59.46360902697142592, -358.7617431975195359 ) ) ;
#31081=CARTESIAN_POINT ( 'NONE',  ( 793.0897708529556667, -342.5545181178796952, -361.3366627262616362 ) ) ;
#31088=CARTESIAN_POINT ( 'NONE',  ( 786.5483106153019435, -343.6454272087887603, -364.1601925771022366 ) ) ;
#31089=CARTESIAN_POINT ( 'NONE',  ( 771.2633955100217236, -359.9073299311467053, -363.4237431249939618 ) ) ;
#31090=CARTESIAN_POINT ( 'NONE',  ( 795.8262568251477660, -142.3726999360620766, -308.3538107759623585 ) ) ;
#31094=CARTESIAN_POINT ( 'NONE',  ( 758.6633372737375112, -284.5328690171412518, -326.9102291470432533 ) ) ;
#31095=CARTESIAN_POINT ( 'NONE',  ( 766.4474001241216001, -163.0999726633347677, -307.3154664389482491 ) ) ;
#31100=CARTESIAN_POINT ( 'NONE',  ( 801.1904061080338124, -188.0891481129653755, -368.3070685750236066 ) ) ;
#31103=CARTESIAN_POINT ( 'NONE',  ( 758.8095938919642549, -320.0891481129648355, -311.6929314249763365 ) ) ;
#31112=CARTESIAN_POINT ( 'NONE',  ( 773.7943932421234194, -359.8055962898683333, -305.5313806188329409 ) ) ;
#31113=CARTESIAN_POINT ( 'NONE',  ( 745.4481719005789273, -123.7255117493292147, -347.5162901302853129 ) ) ;
#31115=CARTESIAN_POINT ( 'NONE',  ( 810.7187646348534145, -402.4527844766010389, -356.7737145352016341 ) ) ;
#31118=ORIENTED_EDGE ( 'NONE', *, *, #14855, .F. ) ;
#31120=CARTESIAN_POINT ( 'NONE',  ( 747.3154664389472828, -163.9874144716871456, -326.4474001241230781 ) ) ;
#31126=CARTESIAN_POINT ( 'NONE',  ( 813.1304606946830518, 6.092670068852159559, -352.3570229623690580 ) ) ;
#31128=CARTESIAN_POINT ( 'NONE',  ( 779.4709603349208464, -96.35105083532370429, -314.7162404726379918 ) ) ;
#31130=CARTESIAN_POINT ( 'NONE',  ( 804.4286716492782716, -185.3618753856926844, -345.3141322388244703 ) ) ;
#31131=CARTESIAN_POINT ( 'NONE',  ( 793.5525998758768083, -415.0999726633340288, -372.6845335610516941 ) ) ;
#31133=CARTESIAN_POINT ( 'NONE',  ( 788.7366044899766848, -251.9073299311470748, -316.5762568750059813 ) ) ;
#31136=CARTESIAN_POINT ( 'NONE',  ( 796.9571628226829034, -239.4636090269709143, -321.2382568024804641 ) ) ;
#31137=CARTESIAN_POINT ( 'NONE',  ( 755.3201227861273992, -243.7255117493287742, -345.3687786644892981 ) ) ;
#31139=CARTESIAN_POINT ( 'NONE',  ( 755.0636971347428243, -436.2709662947827951, -341.7834795799807353 ) ) ;
#31140=CARTESIAN_POINT ( 'NONE',  ( 764.8639956371174549, -80.08914811296574499, -319.7806653035542013 ) ) ;
#31145=CARTESIAN_POINT ( 'NONE',  ( 745.5313806188320314, -39.28179084515331709, -333.7943932421247268 ) ) ;
#31152=CARTESIAN_POINT ( 'NONE',  ( 761.4292242960306112, -17.46360902697157513, -323.2154366446414429 ) ) ;
#31153=CARTESIAN_POINT ( 'NONE',  ( 754.9967657858570647, -73.54369356751121245, -365.0032342141425943 ) ) ;
#31155=CARTESIAN_POINT ( 'NONE',  ( 800.0135310231082713, -446.0891481129646081, -325.0180583372163028 ) ) ;
#31156=CARTESIAN_POINT ( 'NONE',  ( 755.0636971347428243, -28.27096629478409540, -341.7834795799807353 ) ) ;
#31159=CARTESIAN_POINT ( 'NONE',  ( 808.3070685750230950, -186.9982390220563104, -361.1904061080339261 ) ) ;
#31163=VECTOR ( 'NONE', #41049, 1000.000000000000000 ) ;
#31166=CARTESIAN_POINT ( 'NONE',  ( 768.8385539511368734, -263.2601417444141134, -306.4236121716840557 ) ) ;
#31168=CARTESIAN_POINT ( 'NONE',  ( 746.8695393053150156, -269.9073299311468190, -327.6429770376306010 ) ) ;
#31169=CARTESIAN_POINT ( 'NONE',  ( 799.9999999999993179, -512.9681489794448908, -309.9999999999998863 ) ) ;
#31172=CARTESIAN_POINT ( 'NONE',  ( 813.9316612368132837, -31.44195992623299674, -348.6739635108323228 ) ) ;
#31173=CARTESIAN_POINT ( 'NONE',  ( 803.6646147819161570, -377.9073299311466485, -348.8264449731210561 ) ) ;
#31176=CARTESIAN_POINT ( 'NONE',  ( 795.6651683502461765, -58.71468719896019905, -371.3240766477733814 ) ) ;
#31177=CARTESIAN_POINT ( 'NONE',  ( 787.6308680596127942, -155.2601417444144261, -364.1105419155492768 ) ) ;
#31183=CARTESIAN_POINT ( 'NONE',  ( 755.0636971347428243, -52.27096629478401724, -341.7834795799807353 ) ) ;
#31184=CARTESIAN_POINT ( 'NONE',  ( 773.3843516231979720, -181.4419599262325278, -364.4086373105754433 ) ) ;
#31187=CARTESIAN_POINT ( 'NONE',  ( 748.3538107759620743, 7.285312801039605546, -355.8262568251490165 ) ) ;
#31192=CARTESIAN_POINT ( 'NONE',  ( 813.5763878283155464, -291.8272453906071746, -351.1614460488615350 ) ) ;
#31196=CARTESIAN_POINT ( 'NONE',  ( 786.5483106153019435, -151.6454272087892718, -364.1601925771022366 ) ) ;
#31197=CARTESIAN_POINT ( 'NONE',  ( 803.6646147819161570, -161.9073299311472454, -348.8264449731210561 ) ) ;
#31199=CARTESIAN_POINT ( 'NONE',  ( 804.6798772138710092, -303.7255117493286889, -334.6312213355106451 ) ) ;
#31205=EDGE_CURVE ( 'NONE', #8202, #3566, #3806, .T. ) ;
#31209=CARTESIAN_POINT ( 'NONE',  ( 754.3581564841646241, -377.4636090269704596, -316.1443688327762516 ) ) ;
#31213=CARTESIAN_POINT ( 'NONE',  ( 762.3223304703356007, -343.5436935675103314, -322.3223304703362828 ) ) ;
#31215=CARTESIAN_POINT ( 'NONE',  ( 763.0428371773158460, -227.4636090269709143, -358.7617431975195359 ) ) ;
#31218=DIRECTION ( 'NONE',  ( -1.000000000000000000, 0.000000000000000000, 0.000000000000000000 ) ) ;
#31219=CARTESIAN_POINT ( 'NONE',  ( 772.5602148656447525, -417.7255117493283478, -305.7998596910095443 ) ) ;
#31222=CARTESIAN_POINT ( 'NONE',  ( 792.0613484971601110, -458.0032201311295807, -367.4685979341032294 ) ) ;
#31224=CARTESIAN_POINT ( 'NONE',  ( 751.9810565676468741, -50.08914811296584446, -360.9747183278973921 ) ) ;
#31225=CARTESIAN_POINT ( 'NONE',  ( 791.9812246680005501, -236.6346026584198228, -361.9419747391813189 ) ) ;
#31230=CARTESIAN_POINT ( 'NONE',  ( 745.5313806188320314, -15.28179084515340058, -333.7943932421247268 ) ) ;
#31231=CARTESIAN_POINT ( 'NONE',  ( 784.0799538623451781, -59.80559628986927834, -364.6971507214555572 ) ) ;
#31236=DIRECTION ( 'NONE',  ( -1.000000000000000000, 0.000000000000000000, -0.000000000000000000 ) ) ;
#31239=CARTESIAN_POINT ( 'NONE',  ( 771.2633955100217236, -71.90732993114760063, -363.4237431249939618 ) ) ;
#31240=CARTESIAN_POINT ( 'NONE',  ( 760.5453621957607311, -357.0783235625956422, -323.8424801807151425 ) ) ;
#31244=CARTESIAN_POINT ( 'NONE',  ( 754.0944755984390895, -375.6237781080501463, -364.1009440267246760 ) ) ;
#31250=CARTESIAN_POINT ( 'NONE',  ( 755.2512626584698410, -223.5436935675107577, -315.2512626584710915 ) ) ;
#31251=ORIENTED_EDGE ( 'NONE', *, *, #32638, .T. ) ;
#31253=CARTESIAN_POINT ( 'NONE',  ( 788.8264449731201466, -213.1800572038743837, -363.6646147819170665 ) ) ;
#31255=CARTESIAN_POINT ( 'NONE',  ( 778.1981804954714335, -346.2709662947830793, -314.8072714833589885 ) ) ;
#31256=CARTESIAN_POINT ( 'NONE',  ( 785.3687786644884454, -11.36187538569323863, -315.3201227861279676 ) ) ;
#31261=VERTEX_POINT ( 'NONE', #18134 ) ;
#31262=CARTESIAN_POINT ( 'NONE',  ( 804.1105419155481968, -459.8272453906066062, -347.6308680596136469 ) ) ;
#31265=CARTESIAN_POINT ( 'NONE',  ( 810.4231160770870019, -288.5545181178798657, -321.9338519418446936 ) ) ;
#31269=CARTESIAN_POINT ( 'NONE',  ( 797.6776695296629214, -211.5436935675107861, -357.6776695296636603 ) ) ;
#31270=CARTESIAN_POINT ( 'NONE',  ( 783.0433043558608688, -384.8965053807772847, -315.1538015810313027 ) ) ;
#31271=FACE_OUTER_BOUND ( 'NONE', #26622, .T. ) ;
#31272=CARTESIAN_POINT ( 'NONE',  ( 771.1735550268780344, 14.81994279612486309, -316.3353852180828198 ) ) ;
#31273=CARTESIAN_POINT ( 'NONE',  ( 793.9708237608222134, -94.91815448151677970, -319.2295555964448681 ) ) ;
#31276=CARTESIAN_POINT ( 'NONE',  ( 771.2368401574024119, 10.55804007376686826, -374.2805881961240857 ) ) ;
#31277=CARTESIAN_POINT ( 'NONE',  ( 787.5162901302840055, -299.3618753856923149, -305.4481719005793252 ) ) ;
#31279=CARTESIAN_POINT ( 'NONE',  ( 756.3353852180819104, -77.90732993114757221, -331.1735550268788302 ) ) ;
#31280=CIRCLE ( 'NONE', #3987, 10.00000000000000888 ) ;
#31282=CARTESIAN_POINT ( 'NONE',  ( 751.2241431872005251, -184.1692326535052757, -359.9636004259367610 ) ) ;
#31284=CARTESIAN_POINT ( 'NONE',  ( 814.5518280994195948, -447.7255117493280636, -332.4837098697145734 ) ) ;
#31285=DIRECTION ( 'NONE',  ( 0.000000000000000000, -1.000000000000000000, 1.110223024625155554E-15 ) ) ;
#31288=CARTESIAN_POINT ( 'NONE',  ( 792.1044303154645831, -420.4527844766009252, -317.8323909638837677 ) ) ;
#31294=CARTESIAN_POINT ( 'NONE',  ( 780.5290396650775619, -252.3510508353232353, -365.2837595273619513 ) ) ;
#31296=CARTESIAN_POINT ( 'NONE',  ( 811.6461892240364477, -268.7146871989595525, -324.1737431748509835 ) ) ;
#31301=CARTESIAN_POINT ( 'NONE',  ( 800.7704444035546203, -52.16923265350567362, -326.0291762391768771 ) ) ;
#31302=CARTESIAN_POINT ( 'NONE',  ( 803.6646147819161570, -161.9073299311472454, -348.8264449731210561 ) ) ;
#31303=CARTESIAN_POINT ( 'NONE',  ( 758.0580252608178853, -198.4527844766017495, -328.0187753319985404 ) ) ;
#31305=CARTESIAN_POINT ( 'NONE',  ( 745.0891759886404770, -100.2709662947838609, -342.4968714119734159 ) ) ;
#31306=CARTESIAN_POINT ( 'NONE',  ( 755.0636971347428243, -124.2709662947837899, -341.7834795799807353 ) ) ;
#31308=CARTESIAN_POINT ( 'NONE',  ( 802.5472867521000353, -28.37269993606244967, -350.8726784830461156 ) ) ;
#31309=CARTESIAN_POINT ( 'NONE',  ( 755.1538015810308480, -398.1908817542431507, -343.0433043558613804 ) ) ;
#31319=CARTESIAN_POINT ( 'NONE',  ( 805.2837595273609850, -362.7363362996977116, -340.5290396650784714 ) ) ;
#31320=CARTESIAN_POINT ( 'NONE',  ( 803.4237431249931660, -351.1800572038740142, -331.2633955100225194 ) ) ;
#31321=CARTESIAN_POINT ( 'NONE',  ( 762.1177392798416577, -138.5545181178802636, -309.8865473780659272 ) ) ;
#31325=CARTESIAN_POINT ( 'NONE',  ( 756.1348686366196716, -281.2601417444139997, -347.5531968255698416 ) ) ;
#31326=CARTESIAN_POINT ( 'NONE',  ( 790.8050863131179540, -452.8379544210779954, -362.5841948692291226 ) ) ;
#31327=CARTESIAN_POINT ( 'NONE',  ( 745.1792804349281596, -158.1908817542438612, -343.7566961878542884 ) ) ;
#31333=CARTESIAN_POINT ( 'NONE',  ( 796.7737145352015204, -188.6346026584199365, -370.7187646348536987 ) ) ;
#31335=VECTOR ( 'NONE', #9526, 1000.000000000000000 ) ;
#31337=CARTESIAN_POINT ( 'NONE',  ( 808.3070685750230950, -306.9982390220558273, -361.1904061080339261 ) ) ;
#31338=CARTESIAN_POINT ( 'NONE',  ( 779.9999999999992042, 126.4563064324884465, -339.9999999999999432 ) ) ;
#31343=CARTESIAN_POINT ( 'NONE',  ( 746.0683387631852383, -379.4419599262318457, -331.3260364891676204 ) ) ;
#31344=CARTESIAN_POINT ( 'NONE',  ( 772.5602148656447525, -129.7255117493292289, -305.7998596910095443 ) ) ;
#31345=AXIS2_PLACEMENT_3D ( 'NONE', #10553, #45687, #17735 ) ;
#31346=CARTESIAN_POINT ( 'NONE',  ( 787.5162901302840055, -395.3618753856918602, -305.4481719005792684 ) ) ;
#31351=CIRCLE ( 'NONE', #39490, 10.00000000000000888 ) ;
#31352=CARTESIAN_POINT ( 'NONE',  ( 781.2497674668890113, -156.3510508353235480, -375.3608509340180603 ) ) ;
#31359=CARTESIAN_POINT ( 'NONE',  ( 782.5225473063381969, -22.27096629478410250, -375.2698199232970637 ) ) ;
#31363=CARTESIAN_POINT ( 'NONE',  ( 814.4686193811664907, -411.2817908451521589, -346.2056067578752732 ) ) ;
#31367=CARTESIAN_POINT ( 'NONE',  ( 756.5762568750052424, -267.1800572038742985, -348.7366044899774238 ) ) ;
#31370=CARTESIAN_POINT ( 'NONE',  ( 804.6971507214547046, -243.2817908451526705, -344.0799538623459739 ) ) ;
#31371=CARTESIAN_POINT ( 'NONE',  ( 754.8072714833581358, -244.8164208402378961, -338.1981804954720587 ) ) ;
#31372=CARTESIAN_POINT ( 'NONE',  ( 785.3687786644885591, -443.3618753856917465, -315.3201227861280813 ) ) ;
#31373=CARTESIAN_POINT ( 'NONE',  ( 778.2165204200184689, -94.81642084023843609, -364.9363028652563230 ) ) ;
#31380=CARTESIAN_POINT ( 'NONE',  ( 791.0478386215596629, -45.82724539060783542, -306.7653713866226326 ) ) ;
#31383=VECTOR ( 'NONE', #33559, 1000.000000000000000 ) ;
#31387=CARTESIAN_POINT ( 'NONE',  ( 769.9779781133707957, 4.900027336664720679, -316.7813123517150871 ) ) ;
#31388=CARTESIAN_POINT ( 'NONE',  ( 811.0346526505617248, -62.63460265842032726, -323.0537975583478101 ) ) ;
#31390=CARTESIAN_POINT ( 'NONE',  ( 803.4237431249931660, -447.1800572038736732, -331.2633955100225194 ) ) ;
#31392=CARTESIAN_POINT ( 'NONE',  ( 808.3070685750230950, -210.9982390220561967, -361.1904061080339261 ) ) ;
#31399=CARTESIAN_POINT ( 'NONE',  ( 747.3154664389472828, -283.9874144716867477, -326.4474001241230781 ) ) ;
#31402=CARTESIAN_POINT ( 'NONE',  ( 744.7301800767019131, -292.8164208402376971, -337.4774526936615757 ) ) ;
#31406=CARTESIAN_POINT ( 'NONE',  ( 803.4237431249931660, -375.1800572038739574, -331.2633955100225194 ) ) ;
#31408=CARTESIAN_POINT ( 'NONE',  ( 800.1688906516307043, -34.16923265350572336, -369.0717654672308186 ) ) ;
#31409=CARTESIAN_POINT ( 'NONE',  ( 795.9930595647434757, -195.0783235625961538, -320.7433823573372820 ) ) ;
#31412=ORIENTED_EDGE ( 'NONE', *, *, #19891, .T. ) ;
#31413=CARTESIAN_POINT ( 'NONE',  ( 754.8983024940795303, -186.8965053807779668, -336.9254006560228163 ) ) ;
#31415=CIRCLE ( 'NONE', #29226, 30.00000000000008171 ) ;
#31417=CARTESIAN_POINT ( 'NONE',  ( 749.8865473780648472, -44.53286901714205470, -322.1177392798429082 ) ) ;
#31422=CARTESIAN_POINT ( 'NONE',  ( 805.6418435158337843, -293.4636090269707438, -363.8556311672236916 ) ) ;
#31427=CARTESIAN_POINT ( 'NONE',  ( 793.0897708529556667, -150.5545181178802352, -361.3366627262616362 ) ) ;
#31428=CARTESIAN_POINT ( 'NONE',  ( 755.3201227861273992, -147.7255117493291152, -345.3687786644892981 ) ) ;
#31429=CARTESIAN_POINT ( 'NONE',  ( 765.0180583372156207, -360.9982390220557704, -360.0135310231089534 ) ) ;
#31435=DIRECTION ( 'NONE',  ( -1.000000000000000000, -0.000000000000000000, -0.000000000000000000 ) ) ;
#31439=CARTESIAN_POINT ( 'NONE',  ( 812.3518521366052028, -385.0999726633340856, -326.5853460496235243 ) ) ;
#31445=CARTESIAN_POINT ( 'NONE',  ( 804.4286716492782716, -329.3618753856922581, -345.3141322388244703 ) ) ;
#31447=CARTESIAN_POINT ( 'NONE',  ( 775.8780910478218402, -225.2817908451527273, -364.9511171171680530 ) ) ;
#31453=CARTESIAN_POINT ( 'NONE',  ( 787.4397851343537695, -405.7255117493283478, -374.2001403089903988 ) ) ;
#31458=CARTESIAN_POINT ( 'NONE',  ( 787.5162901302840055, -59.36187538569306810, -305.4481719005792684 ) ) ;
#31459=CARTESIAN_POINT ( 'NONE',  ( 774.6858677611749044, -273.7255117493288026, -315.5713283507209894 ) ) ;
#31463=CARTESIAN_POINT ( 'NONE',  ( 756.1348686366196716, -89.26014174441463922, -347.5531968255698416 ) ) ;
#31472=CARTESIAN_POINT ( 'NONE',  ( 759.7806653035534055, -54.99823902205672255, -324.8639956371180801 ) ) ;
#31475=CARTESIAN_POINT ( 'NONE',  ( 770.0799878456142551, -373.9874144716864066, -362.9823548866085616 ) ) ;
#31478=CARTESIAN_POINT ( 'NONE',  ( 773.7943932421234194, -383.8055962898682765, -305.5313806188329409 ) ) ;
#31486=CARTESIAN_POINT ( 'NONE',  ( 813.1304606946830518, -257.9073299311469896, -352.3570229623690580 ) ) ;
#31489=CARTESIAN_POINT ( 'NONE',  ( 757.8323909638828582, -218.6346026584198228, -352.1044303154654358 ) ) ;
#31491=CARTESIAN_POINT ( 'NONE',  ( 762.3223304703356007, -343.5436935675103314, -322.3223304703362828 ) ) ;
#31492=CARTESIAN_POINT ( 'NONE',  ( 778.2165204200184689, 1.183579159761269040, -364.9363028652563230 ) ) ;
#31496=ORIENTED_EDGE ( 'NONE', *, *, #40773, .T. ) ;
#31497=CARTESIAN_POINT ( 'NONE',  ( 766.9102291470427417, -450.5545181178793541, -318.6633372737382501 ) ) ;
#31501=CARTESIAN_POINT ( 'NONE',  ( 795.8262568251477660, -262.3726999360617924, -308.3538107759623585 ) ) ;
#31504=CARTESIAN_POINT ( 'NONE',  ( 767.8955696845333705, -216.4527844766016926, -362.1676090361162323 ) ) ;
#31505=CARTESIAN_POINT ( 'NONE',  ( 763.2154366446407039, -405.6237781080500326, -321.4292242960311228 ) ) ;
#31509=CARTESIAN_POINT ( 'NONE',  ( 804.6971507214547046, -123.2817908451530542, -344.0799538623459739 ) ) ;
#31513=CARTESIAN_POINT ( 'NONE',  ( 783.7566961878529810, 23.10349461922137237, -305.1792804349288417 ) ) ;
#31514=CARTESIAN_POINT ( 'NONE',  ( 782.4968714119720516, -298.8164208402377540, -305.0891759886411023 ) ) ;
#31517=CARTESIAN_POINT ( 'NONE',  ( 800.0135310231082713, -86.08914811296573077, -325.0180583372163028 ) ) ;
#31520=CARTESIAN_POINT ( 'NONE',  ( 744.8212110874229666, -186.8965053807779668, -336.2046728542121627 ) ) ;
#31522=CARTESIAN_POINT ( 'NONE',  ( 748.9653473494363425, -434.6346026584190554, -356.9462024416521331 ) ) ;
#31527=CARTESIAN_POINT ( 'NONE',  ( 758.0580252608178853, -438.4527844766009821, -328.0187753319985404 ) ) ;
#31536=CARTESIAN_POINT ( 'NONE',  ( 805.1016975059191054, -270.8965053807777394, -343.0745993439771837 ) ) ;
#31538=CARTESIAN_POINT ( 'NONE',  ( 746.0683387631852383, -283.4419599262321867, -331.3260364891676204 ) ) ;
#31543=CARTESIAN_POINT ( 'NONE',  ( 805.0264073115434940, -54.35105083532383219, -339.4763451958999099 ) ) ;
#31544=CARTESIAN_POINT ( 'NONE',  ( 755.3201227861273992, -195.7255117493289731, -345.3687786644892981 ) ) ;
#31547=CARTESIAN_POINT ( 'NONE',  ( 745.4481719005789273, -99.72551174932928575, -347.5162901302853129 ) ) ;
#31548=CARTESIAN_POINT ( 'NONE',  ( 756.5762568750052424, -123.1800572038747106, -348.7366044899774238 ) ) ;
#31551=CARTESIAN_POINT ( 'NONE',  ( 755.8894580844503253, -375.8272453906069472, -332.3691319403863531 ) ) ;
#31559=CARTESIAN_POINT ( 'NONE',  ( 787.5531968255692163, -357.8272453906068904, -316.1348686366205811 ) ) ;
#31560=CARTESIAN_POINT ( 'NONE',  ( 804.9363028652555840, -352.2709662947830225, -338.2165204200192079 ) ) ;
#31561=CARTESIAN_POINT ( 'NONE',  ( 795.8262568251477660, -166.3726999360620198, -308.3538107759623585 ) ) ;
#31565=CARTESIAN_POINT ( 'NONE',  ( 799.4546378042377910, -297.0783235625957559, -356.1575198192848006 ) ) ;
#31567=CARTESIAN_POINT ( 'NONE',  ( 744.6391490659812007, -158.7363362996984222, -338.7502325331110455 ) ) ;
#31572=CARTESIAN_POINT ( 'NONE',  ( 745.0891759886404770, -196.2709662947835909, -342.4968714119734159 ) ) ;
#31575=CARTESIAN_POINT ( 'NONE',  ( 767.6429770376289525, -345.1800572038739006, -306.8695393053162093 ) ) ;
#31581=CARTESIAN_POINT ( 'NONE',  ( 807.5423716828161105, -393.0783235625954717, -362.2119215644372048 ) ) ;
#31583=CARTESIAN_POINT ( 'NONE',  ( 808.3070685750230950, -138.9982390220563957, -361.1904061080339261 ) ) ;
#31584=CARTESIAN_POINT ( 'NONE',  ( 744.7301800767019131, -436.8164208402372992, -337.4774526936615757 ) ) ;
#31588=CARTESIAN_POINT ( 'NONE',  ( 788.7631598425961101, -193.4419599262325278, -305.7194118038759143 ) ) ;
#31594=CARTESIAN_POINT ( 'NONE',  ( 772.5602148656447525, -9.725511749329603717, -305.7998596910095443 ) ) ;
#31597=CARTESIAN_POINT ( 'NONE',  ( 797.8822607201568644, -414.5545181178795247, -370.1134526219340160 ) ) ;
#31600=CARTESIAN_POINT ( 'NONE',  ( 778.1981804954714335, -274.2709662947833067, -314.8072714833589885 ) ) ;
#31604=CARTESIAN_POINT ( 'NONE',  ( 757.0176451133909268, -253.0999726633345119, -349.9200121543848354 ) ) ;
#31605=CARTESIAN_POINT ( 'NONE',  ( 768.0187753319979720, -248.6346026584197659, -318.0580252608186242 ) ) ;
#31607=CARTESIAN_POINT ( 'NONE',  ( 778.1981804954714335, -130.2709662947837899, -314.8072714833589885 ) ) ;
#31612=CARTESIAN_POINT ( 'NONE',  ( 807.2620300519052989, -48.00906357242602951, -318.0141637701419768 ) ) ;
#31618=CARTESIAN_POINT ( 'NONE',  ( 786.5483106153019435, -7.645427208789786100, -364.1601925771022366 ) ) ;
#31619=CARTESIAN_POINT ( 'NONE',  ( 810.7187646348534145, -114.4527844766020053, -356.7737145352016341 ) ) ;
#31623=CARTESIAN_POINT ( 'NONE',  ( 751.9810565676468741, -218.0891481129653187, -360.9747183278973921 ) ) ;
#31626=CARTESIAN_POINT ( 'NONE',  ( 746.7653713866222915, -257.2601417444141134, -351.0478386215610271 ) ) ;
#31628=CARTESIAN_POINT ( 'NONE',  ( 804.7487373415286811, -331.5436935675104451, -364.7487373415288516 ) ) ;
#31632=CARTESIAN_POINT ( 'NONE',  ( 758.0580252608178853, -390.4527844766011526, -328.0187753319985404 ) ) ;
#31634=CARTESIAN_POINT ( 'NONE',  ( 744.9990715423526808, -66.35105083532378956, -341.2370466360926002 ) ) ;
#31635=CARTESIAN_POINT ( 'NONE',  ( 766.7756240680305382, -206.5328690171415360, -361.5560724626415663 ) ) ;
#31639=CARTESIAN_POINT ( 'NONE',  ( 773.3843516231979720, -205.4419599262324425, -364.4086373105754433 ) ) ;
#31641=CARTESIAN_POINT ( 'NONE',  ( 768.8385539511368734, -23.26014174441484883, -306.4236121716840557 ) ) ;
#31646=CARTESIAN_POINT ( 'NONE',  ( 746.4236121716829757, -303.8272453906071178, -328.8385539511384650 ) ) ;
#31649=CARTESIAN_POINT ( 'NONE',  ( 772.4468031744293057, -153.8272453906075157, -363.8651313633793620 ) ) ;
#31650=CARTESIAN_POINT ( 'NONE',  ( 800.0135310231082713, -158.0891481129655176, -325.0180583372163028 ) ) ;
#31651=CARTESIAN_POINT ( 'NONE',  ( 788.8264449731201466, -333.1800572038740142, -363.6646147819170665 ) ) ;
#31653=CARTESIAN_POINT ( 'NONE',  ( 804.4286716492782716, -449.3618753856918602, -345.3141322388244703 ) ) ;
#31661=CARTESIAN_POINT ( 'NONE',  ( 791.0478386215596629, -381.8272453906068336, -306.7653713866226326 ) ) ;
#31665=CARTESIAN_POINT ( 'NONE',  ( 771.1735550268778070, -369.1800572038739574, -316.3353852180827630 ) ) ;
#31667=CARTESIAN_POINT ( 'NONE',  ( 793.0897708529556667, -222.5545181178800362, -361.3366627262616362 ) ) ;
#31670=CARTESIAN_POINT ( 'NONE',  ( 801.1904061080338124, -404.0891481129646650, -368.3070685750236066 ) ) ;
#31675=CARTESIAN_POINT ( 'NONE',  ( 782.4968714119720516, -58.81642084023854267, -305.0891759886411023 ) ) ;
#31677=CARTESIAN_POINT ( 'NONE',  ( 804.9363028652555840, -280.2709662947833067, -338.2165204200192079 ) ) ;
#31681=CARTESIAN_POINT ( 'NONE',  ( 752.7379699480933368, -36.00906357242605793, -361.9858362298580232 ) ) ;
#31682=CARTESIAN_POINT ( 'NONE',  ( 804.9511171171677688, -101.8055962898691718, -335.8780910478229202 ) ) ;
#31687=CARTESIAN_POINT ( 'NONE',  ( 767.8955696845333705, -0.4527844766023628176, -362.1676090361162323 ) ) ;
#31688=CARTESIAN_POINT ( 'NONE',  ( 776.9566956441375396, -108.8965053807782084, -364.8461984189686405 ) ) ;
#31690=CARTESIAN_POINT ( 'NONE',  ( 785.3687786644884454, -107.3618753856928976, -315.3201227861279676 ) ) ;
#31691=CARTESIAN_POINT ( 'NONE',  ( 796.7845633553578182, -393.6237781080500326, -358.5707757039688204 ) ) ;
#31694=CARTESIAN_POINT ( 'NONE',  ( 800.1688906516307043, -394.1692326535045368, -369.0717654672308186 ) ) ;
#31700=CARTESIAN_POINT ( 'NONE',  ( 782.4968714119720516, -250.8164208402379245, -305.0891759886411023 ) ) ;
#31704=CARTESIAN_POINT ( 'NONE',  ( 756.5762568750052424, -243.1800572038743269, -348.7366044899774238 ) ) ;
#31706=CARTESIAN_POINT ( 'NONE',  ( 801.9419747391806368, -354.4527844766012095, -351.9812246680014027 ) ) ;
#31707=CARTESIAN_POINT ( 'NONE',  ( 781.8018195045266339, -22.27096629478410250, -365.1927285166406705 ) ) ;
#31712=CARTESIAN_POINT ( 'NONE',  ( 771.1735550268778070, -33.18005720387498769, -316.3353852180827630 ) ) ;
#31716=CARTESIAN_POINT ( 'NONE',  ( 752.7379699480933368, -276.0090635724253048, -361.9858362298580232 ) ) ;
#31719=CARTESIAN_POINT ( 'NONE',  ( 801.9419747391806368, -210.4527844766016926, -351.9812246680014027 ) ) ;
#31720=CARTESIAN_POINT ( 'NONE',  ( 756.7813123517142913, -403.9874144716863498, -329.9779781133712504 ) ) ;
#31721=DIRECTION ( 'NONE',  ( -1.000000000000000000, -0.000000000000000000, 0.000000000000000000 ) ) ;
#31722=CARTESIAN_POINT ( 'NONE',  ( 769.9779781133707957, -115.0999726633348956, -316.7813123517150871 ) ) ;
#31726=CARTESIAN_POINT ( 'NONE',  ( 748.3538107759620743, 7.285312801039605546, -355.8262568251490165 ) ) ;
#31727=CARTESIAN_POINT ( 'NONE',  ( 751.6929314249750860, -318.9982390220558841, -318.8095938919659034 ) ) ;
#31729=CARTESIAN_POINT ( 'NONE',  ( 767.8955696845333705, -72.45278447660213317, -362.1676090361162323 ) ) ;
#31731=CARTESIAN_POINT ( 'NONE',  ( 811.6461892240364477, -196.7146871989598083, -324.1737431748509835 ) ) ;
#31733=CARTESIAN_POINT ( 'NONE',  ( 766.4474001241216001, 4.900027336664720679, -307.3154664389482491 ) ) ;
#31738=CARTESIAN_POINT ( 'NONE',  ( 792.1044303154645831, -444.4527844766009821, -317.8323909638837677 ) ) ;
#31744=CARTESIAN_POINT ( 'NONE',  ( 773.3843516231979720, -301.4419599262320730, -364.4086373105754433 ) ) ;
#31746=CARTESIAN_POINT ( 'NONE',  ( 744.8212110874229666, -282.8965053807776258, -336.2046728542121627 ) ) ;
#31753=CARTESIAN_POINT ( 'NONE',  ( 802.7791456095903868, -52.71468719896020616, -329.0155153010375102 ) ) ;
#31754=CARTESIAN_POINT ( 'NONE',  ( 758.0580252608178853, -174.4527844766018063, -328.0187753319985404 ) ) ;
#31755=CARTESIAN_POINT ( 'NONE',  ( 756.5762568750052424, -195.1800572038744974, -348.7366044899774238 ) ) ;
#31757=CARTESIAN_POINT ( 'NONE',  ( 751.6929314249748586, -150.9982390220563957, -318.8095938919659034 ) ) ;
#31759=CARTESIAN_POINT ( 'NONE',  ( 804.9363028652555840, -136.2709662947837330, -338.2165204200192079 ) ) ;
#31761=CARTESIAN_POINT ( 'NONE',  ( 805.2837595273609850, -386.7363362996977116, -340.5290396650784714 ) ) ;
#31766=CYLINDRICAL_SURFACE ( 'NONE', #18132, 10.00000000000000888 ) ;
#31769=CARTESIAN_POINT ( 'NONE',  ( 802.9823548866075953, -385.0999726633340856, -330.0799878456151077 ) ) ;
#31770=CARTESIAN_POINT ( 'NONE',  ( 804.6798772138708955, -351.7255117493284047, -334.6312213355107019 ) ) ;
#31771=CARTESIAN_POINT ( 'NONE',  ( 746.4236121716829757, -159.8272453906075157, -328.8385539511384650 ) ) ;
#31776=CARTESIAN_POINT ( 'NONE',  ( 783.0433043558608688, -288.8965053807775121, -315.1538015810313027 ) ) ;
#31777=CARTESIAN_POINT ( 'NONE',  ( 805.1927285166397041, -448.8164208402371855, -341.8018195045277707 ) ) ;
#31778=CARTESIAN_POINT ( 'NONE',  ( 812.3518521366052028, -169.0999726633347393, -326.5853460496235243 ) ) ;
#31784=CARTESIAN_POINT ( 'NONE',  ( 747.2067596250078623, -195.1800572038744974, -352.2312462859687230 ) ) ;
#31788=CARTESIAN_POINT ( 'NONE',  ( 758.0141637701419768, -111.0783235625964096, -367.2620300519063790 ) ) ;
#31790=CARTESIAN_POINT ( 'NONE',  ( 814.9108240113580450, -328.2709662947831362, -337.5031285880265273 ) ) ;
#31796=CARTESIAN_POINT ( 'NONE',  ( 781.2497674668890113, -396.3510508353228374, -375.3608509340180603 ) ) ;
#31797=CARTESIAN_POINT ( 'NONE',  ( 772.4837098697144029, -407.3618753856920307, -374.5518280994205611 ) ) ;
#31802=CARTESIAN_POINT ( 'NONE',  ( 791.1614460488616487, -179.2601417444143692, -373.5763878283158874 ) ) ;
#31807=CARTESIAN_POINT ( 'NONE',  ( 762.1405469898971887, -145.5436935675109851, -357.8594530101015607 ) ) ;
#31809=CARTESIAN_POINT ( 'NONE',  ( 787.5162901302840055, -59.36187538569306810, -305.4481719005792684 ) ) ;
#31812=CARTESIAN_POINT ( 'NONE',  ( 809.0717654672305343, -436.9181544815157281, -360.1688906516309885 ) ) ;
#31813=VERTEX_POINT ( 'NONE', #23384 ) ;
#31816=CARTESIAN_POINT ( 'NONE',  ( 771.2633955100217236, -287.9073299311468759, -363.4237431249939618 ) ) ;
#31820=CARTESIAN_POINT ( 'NONE',  ( 796.9571628226829034, -263.4636090269708006, -321.2382568024804641 ) ) ;
#31821=CARTESIAN_POINT ( 'NONE',  ( 781.7834795799800531, -250.8164208402379245, -315.0636971347436202 ) ) ;
#31822=CARTESIAN_POINT ( 'NONE',  ( 797.8594530101009923, -445.5436935675099335, -322.1405469898982119 ) ) ;
#31823=CARTESIAN_POINT ( 'NONE',  ( 804.6798772138708955, -111.7255117493293000, -334.6312213355107019 ) ) ;
#31827=CARTESIAN_POINT ( 'NONE',  ( 799.9999999999993179, -462.9681489794448339, -370.0000000000000568 ) ) ;
#31829=CARTESIAN_POINT ( 'NONE',  ( 746.4236121716829757, -63.82724539060779279, -328.8385539511384650 ) ) ;
#31835=CARTESIAN_POINT ( 'NONE',  ( 790.0220218866281812, -7.099972663335241130, -363.2186876482849129 ) ) ;
#31837=CARTESIAN_POINT ( 'NONE',  ( 782.4968714119720516, -106.8164208402383935, -305.0891759886411023 ) ) ;
#31839=CARTESIAN_POINT ( 'NONE',  ( 779.9999999999992042, -462.9681489794448339, -339.9999999999999432 ) ) ;
#31841=CARTESIAN_POINT ( 'NONE',  ( 755.2512626584698410, -223.5436935675107577, -315.2512626584710915 ) ) ;
#31844=CARTESIAN_POINT ( 'NONE',  ( 749.8865473780648472, -284.5328690171412518, -322.1177392798429082 ) ) ;
#31846=CARTESIAN_POINT ( 'NONE',  ( 777.5031285880264704, -310.8164208402377540, -374.9108240113588408 ) ) ;
#31850=CARTESIAN_POINT ( 'NONE',  ( 794.9819416627830151, -396.9982390220556567, -319.9864689768909898 ) ) ;
#31852=CARTESIAN_POINT ( 'NONE',  ( 794.9819416627830151, -204.9982390220562820, -319.9864689768909898 ) ) ;
#31853=CARTESIAN_POINT ( 'NONE',  ( 814.8230680027162407, -77.80559628986920018, -333.7305795820267917 ) ) ;
#31857=CARTESIAN_POINT ( 'NONE',  ( 788.7366044899766848, -83.90732993114754379, -316.5762568750059813 ) ) ;
#31858=CARTESIAN_POINT ( 'NONE',  ( 769.1273215169530886, -214.7146871989597230, -317.4527132478988847 ) ) ;
#31860=CARTESIAN_POINT ( 'NONE',  ( 748.3538107759620743, -40.71468719896024879, -355.8262568251490165 ) ) ;
#31866=CARTESIAN_POINT ( 'NONE',  ( 778.7629533639073998, -320.7363362996979390, -375.0009284576466371 ) ) ;
#31870=CARTESIAN_POINT ( 'NONE',  ( 757.4527132478984868, -136.3726999360621051, -329.1273215169538844 ) ) ;
#31871=CARTESIAN_POINT ( 'NONE',  ( 778.1981804954714335, -154.2709662947836478, -314.8072714833589885 ) ) ;
#31872=CARTESIAN_POINT ( 'NONE',  ( 757.8323909638828582, -338.6346026584195101, -352.1044303154654358 ) ) ;
#31877=LINE ( 'NONE', #24, #17483 ) ;
#31881=CARTESIAN_POINT ( 'NONE',  ( 745.7194118038753459, -373.6454272087887034, -348.7631598425976449 ) ) ;
#31884=CARTESIAN_POINT ( 'NONE',  ( 787.5162901302840055, 12.63812461430668677, -305.4481719005793252 ) ) ;
#31887=CARTESIAN_POINT ( 'NONE',  ( 755.5713283507202505, -365.3618753856920875, -334.6858677611754729 ) ) ;
#31889=CARTESIAN_POINT ( 'NONE',  ( 754.7162404726377645, -206.7363362996982801, -339.4709603349214717 ) ) ;
#31894=CARTESIAN_POINT ( 'NONE',  ( 800.9747183278959710, -420.9982390220555999, -311.9810565676471583 ) ) ;
#31897=CARTESIAN_POINT ( 'NONE',  ( 806.6271908675616942, -455.4127378225107350, -353.8200110890837777 ) ) ;
#31899=CARTESIAN_POINT ( 'NONE',  ( 792.2312462859673587, -59.90732993114762905, -307.2067596250082602 ) ) ;
#31900=CARTESIAN_POINT ( 'NONE',  ( 804.6798772138708955, -279.7255117493288026, -334.6312213355107019 ) ) ;
#31904=CARTESIAN_POINT ( 'NONE',  ( 815.3608509340175488, -74.73633629969866377, -341.2497674668889545 ) ) ;
#31905=CARTESIAN_POINT ( 'NONE',  ( 801.3366627262608972, -80.53286901714194812, -353.0897708529566899 ) ) ;
#31909=CARTESIAN_POINT ( 'NONE',  ( 774.6312213355099630, 0.6381246143067236254, -364.6798772138717482 ) ) ;
#31911=CARTESIAN_POINT ( 'NONE',  ( 801.9419747391806368, -114.4527844766020053, -351.9812246680014027 ) ) ;
#31912=CARTESIAN_POINT ( 'NONE',  ( 755.8398074228967971, -403.4419599262317888, -333.4516893846970333 ) ) ;
#31916=CARTESIAN_POINT ( 'NONE',  ( 788.7631598425961101, -409.4419599262317320, -305.7194118038759143 ) ) ;
#31921=CARTESIAN_POINT ( 'NONE',  ( 801.1904061080336987, -260.0891481129650060, -368.3070685750235498 ) ) ;
#31926=CARTESIAN_POINT ( 'NONE',  ( 771.1735550268780344, -249.1800572038742700, -316.3353852180828198 ) ) ;
#31929=CARTESIAN_POINT ( 'NONE',  ( 792.1044303154645831, -372.4527844766010958, -317.8323909638837677 ) ) ;
#31930=CARTESIAN_POINT ( 'NONE',  ( 756.5762568750052424, -27.18005720387500901, -348.7366044899774238 ) ) ;
#31934=CARTESIAN_POINT ( 'NONE',  ( 799.9999999999993179, 205.0000000000000568, -329.9999999999999432 ) ) ;
#31936=CARTESIAN_POINT ( 'NONE',  ( 755.3201227861273992, -3.725511749329622813, -345.3687786644892981 ) ) ;
#31939=CARTESIAN_POINT ( 'NONE',  ( 811.3240766477731540, -268.3726999360616787, -355.6651683502462902 ) ) ;
#31942=CARTESIAN_POINT ( 'NONE',  ( 759.9864689768902508, -242.0891481129652618, -354.9819416627836404 ) ) ;
#31943=CARTESIAN_POINT ( 'NONE',  ( 758.6633372737375112, -380.5328690171409676, -326.9102291470432533 ) ) ;
#31945=CARTESIAN_POINT ( 'NONE',  ( 786.5483106153019435, -127.6454272087894140, -364.1601925771022366 ) ) ;
#31949=CARTESIAN_POINT ( 'NONE',  ( 801.9858362298568863, -3.078323562596726681, -312.7379699480935642 ) ) ;
#31950=CARTESIAN_POINT ( 'NONE',  ( 804.7487373415286811, -307.5436935675104451, -364.7487373415288516 ) ) ;
#31955=CARTESIAN_POINT ( 'NONE',  ( 761.9338519418445230, -206.5328690171415360, -370.4231160770881957 ) ) ;
#31957=CARTESIAN_POINT ( 'NONE',  ( 754.9967657858570647, -433.5436935675099903, -365.0032342141425374 ) ) ;
#31962=CARTESIAN_POINT ( 'NONE',  ( 754.9735926884551418, 5.648949164675971524, -340.5236548041000333 ) ) ;
#31965=DIRECTION ( 'NONE',  ( 0.000000000000000000, 0.000000000000000000, 1.000000000000000000 ) ) ;
#31969=CARTESIAN_POINT ( 'NONE',  ( 772.3691319403857278, -287.2601417444140566, -315.8894580844506663 ) ) ;
#31972=CARTESIAN_POINT ( 'NONE',  ( 795.6651683502461765, -298.7146871989593251, -371.3240766477733814 ) ) ;
#31977=CARTESIAN_POINT ( 'NONE',  ( 780.5290396650775619, -60.35105083532383219, -365.2837595273619513 ) ) ;
#31978=CARTESIAN_POINT ( 'NONE',  ( 755.0636971347428243, -172.2709662947836478, -341.7834795799807353 ) ) ;
#31979=CARTESIAN_POINT ( 'NONE',  ( 795.1360043628807261, -212.0891481129652902, -360.2193346964456282 ) ) ;
#31982=CARTESIAN_POINT ( 'NONE',  ( 804.7487373415286811, -139.5436935675110135, -364.7487373415288516 ) ) ;
#31985=CARTESIAN_POINT ( 'NONE',  ( 756.3353852180820240, -149.9073299311473875, -331.1735550268787733 ) ) ;
#31988=CARTESIAN_POINT ( 'NONE',  ( 784.1219089521767955, -405.2817908451522158, -315.0488828828318333 ) ) ;
#31994=ADVANCED_FACE ( 'NONE', ( #16930 ), #31010, .F. ) ;
#31996=CARTESIAN_POINT ( 'NONE',  ( 804.6971507214547046, -411.2817908451521589, -344.0799538623459739 ) ) ;
#31998=CARTESIAN_POINT ( 'NONE',  ( 768.9521613784389729, -153.8272453906075157, -373.2346286133773106 ) ) ;
#32003=CARTESIAN_POINT ( 'NONE',  ( 764.0069404352550464, -303.0783235625957559, -359.2566176426627180 ) ) ;
#32005=CARTESIAN_POINT ( 'NONE',  ( 795.8262568251477660, -190.3726999360619629, -308.3538107759623585 ) ) ;
#32006=CARTESIAN_POINT ( 'NONE',  ( 779.9999999999992042, 126.4563064324884465, -339.9999999999999432 ) ) ;
#32010=CARTESIAN_POINT ( 'NONE',  ( 767.6429770376291799, -201.1800572038744690, -306.8695393053162093 ) ) ;
#32016=CARTESIAN_POINT ( 'NONE',  ( 776.2433038121456548, -108.8965053807782084, -374.8207195650711014 ) ) ;
#32018=CARTESIAN_POINT ( 'NONE',  ( 787.5162901302840055, -347.3618753856922012, -305.4481719005792684 ) ) ;
#32025=CARTESIAN_POINT ( 'NONE',  ( 748.3538107759620743, -424.7146871989589840, -355.8262568251490165 ) ) ;
#32026=CARTESIAN_POINT ( 'NONE',  ( 751.9810565676468741, -410.0891481129647218, -360.9747183278973921 ) ) ;
#32030=CARTESIAN_POINT ( 'NONE',  ( 756.1443688327750579, -189.6237781080507148, -314.3581564841659315 ) ) ;
#32039=EDGE_CURVE ( 'NONE', #19801, #3816, #4388, .T. ) ;
#32040=CARTESIAN_POINT ( 'NONE',  ( 745.7998596910086917, -53.36187538569310362, -332.5602148656461168 ) ) ;
#32043=CARTESIAN_POINT ( 'NONE',  ( 768.9521613784389729, -441.8272453906066630, -373.2346286133773106 ) ) ;
#32046=CARTESIAN_POINT ( 'NONE',  ( 803.6646147819161570, -305.9073299311467622, -348.8264449731210561 ) ) ;
#32051=CARTESIAN_POINT ( 'NONE',  ( 772.4468031744293057, -297.8272453906070041, -363.8651313633793620 ) ) ;
#32052=CARTESIAN_POINT ( 'NONE',  ( 802.1676090361156639, -254.6346026584196238, -327.8955696845344505 ) ) ;
#32054=CARTESIAN_POINT ( 'NONE',  ( 768.0187753319979720, -128.6346026584201354, -318.0580252608186242 ) ) ;
#32060=CARTESIAN_POINT ( 'NONE',  ( 759.9999999999992042, 166.4563064324884465, -319.9999999999999432 ) ) ;
#32061=CARTESIAN_POINT ( 'NONE',  ( 805.6418435158337843, -77.46360902697138329, -363.8556311672236916 ) ) ;
#32067=CARTESIAN_POINT ( 'NONE',  ( 799.2566176426618085, -48.00906357242602951, -324.0069404352559559 ) ) ;
#32068=CARTESIAN_POINT ( 'NONE',  ( 763.0537975583476964, -96.45278447660204790, -371.0346526505628617 ) ) ;
#32073=CARTESIAN_POINT ( 'NONE',  ( 747.2067596250078623, -219.1800572038744122, -352.2312462859687230 ) ) ;
#32079=CARTESIAN_POINT ( 'NONE',  ( 815.1787889125755555, -294.8965053807775689, -343.7953271457877804 ) ) ;
#32081=CARTESIAN_POINT ( 'NONE',  ( 792.3570229623688874, -309.1800572038740711, -373.1304606946836202 ) ) ;
#32085=CARTESIAN_POINT ( 'NONE',  ( 757.8323909638827445, -386.6346026584191691, -352.1044303154654358 ) ) ;
#32087=CARTESIAN_POINT ( 'NONE',  ( 805.1927285166397041, -208.8164208402380666, -341.8018195045277707 ) ) ;
#32088=AXIS2_PLACEMENT_3D ( 'NONE', #20312, #3459, #45043 ) ;
#32089=CARTESIAN_POINT ( 'NONE',  ( 808.7758568127978833, -76.16923265350557415, -320.0363995740631822 ) ) ;
#32097=CARTESIAN_POINT ( 'NONE',  ( 755.0488828828309806, -185.8055962898689302, -344.1219089521771934 ) ) ;
#32099=CARTESIAN_POINT ( 'NONE',  ( 749.8865473780648472, -20.53286901714212931, -322.1177392798429082 ) ) ;
#32102=CARTESIAN_POINT ( 'NONE',  ( 796.9142768083648889, -452.9681489794446634, -358.6301678913937963 ) ) ;
#32106=CARTESIAN_POINT ( 'NONE',  ( 750.9282345327678740, -352.9181544815159555, -319.8311093483690115 ) ) ;
#32112=CARTESIAN_POINT ( 'NONE',  ( 793.9708237608222134, -190.9181544815164955, -319.2295555964448681 ) ) ;
#32113=CARTESIAN_POINT ( 'NONE',  ( 792.1044303154645831, -156.4527844766018916, -317.8323909638837677 ) ) ;
#32114=CARTESIAN_POINT ( 'NONE',  ( 765.0180583372156207, -336.9982390220558273, -360.0135310231089534 ) ) ;
#32116=CARTESIAN_POINT ( 'NONE',  ( 773.3843516231979720, 10.55804007376686826, -364.4086373105754433 ) ) ;
#32124=CARTESIAN_POINT ( 'NONE',  ( 783.7953271457878373, -368.1908817542433212, -375.1787889125761239 ) ) ;
#32126=CARTESIAN_POINT ( 'NONE',  ( 787.4397851343537695, 2.274488250670355871, -374.2001403089903988 ) ) ;
#32130=CARTESIAN_POINT ( 'NONE',  ( 794.9819416627830151, -348.9982390220558273, -319.9864689768909898 ) ) ;
#32133=CARTESIAN_POINT ( 'NONE',  ( 772.4468031744293057, -225.8272453906072599, -363.8651313633793620 ) ) ;
#32137=CARTESIAN_POINT ( 'NONE',  ( 763.0537975583476964, -432.4527844766009252, -371.0346526505628617 ) ) ;
#32143=CARTESIAN_POINT ( 'NONE',  ( 813.1304606946830518, -41.90732993114767169, -352.3570229623690580 ) ) ;
#32144=CARTESIAN_POINT ( 'NONE',  ( 755.5713283507202505, -293.3618753856923718, -334.6858677611754729 ) ) ;
#32149=CARTESIAN_POINT ( 'NONE',  ( 804.1009440267234822, -71.46360902697141171, -314.0944755984392600 ) ) ;
#32150=CARTESIAN_POINT ( 'NONE',  ( 796.7845633553578182, -81.62377810805104161, -358.5707757039688204 ) ) ;
#32154=CARTESIAN_POINT ( 'NONE',  ( 792.1044303154645831, 11.54721552339760038, -317.8323909638837677 ) ) ;
#32156=CARTESIAN_POINT ( 'NONE',  ( 804.6798772138708955, -87.72551174932937101, -334.6312213355107019 ) ) ;
#32157=CARTESIAN_POINT ( 'NONE',  ( 756.1348686366196716, -401.2601417444137155, -347.5531968255698416 ) ) ;
#32160=CARTESIAN_POINT ( 'NONE',  ( 811.6461892240364477, -412.7146871989590409, -324.1737431748509835 ) ) ;
#32164=CIRCLE ( 'NONE', #42484, 10.00000000000000888 ) ;
#32169=CARTESIAN_POINT ( 'NONE',  ( 777.4774526936600978, -250.2709662947832783, -304.7301800767027657 ) ) ;
#32173=CARTESIAN_POINT ( 'NONE',  ( 769.0155153010367712, -58.37269993606236085, -362.7791456095907279 ) ) ;
#32175=CARTESIAN_POINT ( 'NONE',  ( 804.6798772138710092, -231.7255117493288594, -334.6312213355106451 ) ) ;
#32177=CARTESIAN_POINT ( 'NONE',  ( 805.1927285166397041, -352.8164208402374129, -341.8018195045277707 ) ) ;
#32178=CARTESIAN_POINT ( 'NONE',  ( 767.8955696845333705, -48.45278447660219712, -362.1676090361162323 ) ) ;
#32185=CARTESIAN_POINT ( 'NONE',  ( 759.7806653035534055, -6.998239022056885972, -324.8639956371180801 ) ) ;
#32189=CARTESIAN_POINT ( 'NONE',  ( 766.4474001241216001, -283.0999726633344267, -307.3154664389482491 ) ) ;
#32192=CARTESIAN_POINT ( 'NONE',  ( 805.1927285166397041, -256.8164208402379245, -341.8018195045277707 ) ) ;
#32194=CARTESIAN_POINT ( 'NONE',  ( 755.3028492785439312, -111.2817908451530968, -335.9200461376539693 ) ) ;
#32196=CARTESIAN_POINT ( 'NONE',  ( 744.8212110874229666, -18.89650538077849617, -336.2046728542121627 ) ) ;
#32197=CARTESIAN_POINT ( 'NONE',  ( 763.2262854647970016, -296.6346026584195670, -309.2812353651462445 ) ) ;
#32201=CARTESIAN_POINT ( 'NONE',  ( 745.1769319972822814, -209.8055962898687881, -346.2694204179732083 ) ) ;
#32203=CARTESIAN_POINT ( 'NONE',  ( 814.9108240113580450, -448.2709662947827951, -337.5031285880265273 ) ) ;
#32210=CARTESIAN_POINT ( 'NONE',  ( 794.1144889064781864, 13.83076734649413098, -360.9840315886528401 ) ) ;
#32217=CARTESIAN_POINT ( 'NONE',  ( 765.8855110935204493, -286.1692326535048778, -319.0159684113471599 ) ) ;
#32220=CARTESIAN_POINT ( 'NONE',  ( 746.7653713866222915, -281.2601417444139997, -351.0478386215610271 ) ) ;
#32225=CARTESIAN_POINT ( 'NONE',  ( 764.0069404352550464, -63.07832356259653750, -359.2566176426627180 ) ) ;
#32226=CARTESIAN_POINT ( 'NONE',  ( 764.8639956371174549, -152.0891481129655460, -319.7806653035542013 ) ) ;
#32227=CARTESIAN_POINT ( 'NONE',  ( 774.6312213355099630, -215.3618753856925423, -364.6798772138717482 ) ) ;
#32229=CARTESIAN_POINT ( 'NONE',  ( 808.0189434323515343, -134.0891481129655745, -319.0252816721025511 ) ) ;
#32231=CARTESIAN_POINT ( 'NONE',  ( 778.2165204200184689, -142.8164208402382656, -364.9363028652563230 ) ) ;
#32233=CARTESIAN_POINT ( 'NONE',  ( 802.9823548866075953, -385.0999726633340856, -330.0799878456151077 ) ) ;
#32238=CARTESIAN_POINT ( 'NONE',  ( 779.9999999999992042, 126.4563064324884465, -339.9999999999999432 ) ) ;
#32242=CARTESIAN_POINT ( 'NONE',  ( 784.1219089521767955, -381.2817908451523294, -315.0488828828318333 ) ) ;
#32244=CARTESIAN_POINT ( 'NONE',  ( 811.3240766477731540, -172.3726999360619914, -355.6651683502462902 ) ) ;
#32249=CARTESIAN_POINT ( 'NONE',  ( 783.0433043558608688, -312.8965053807775689, -315.1538015810313027 ) ) ;
#32250=CARTESIAN_POINT ( 'NONE',  ( 755.3201227861273992, -435.7255117493282341, -345.3687786644892981 ) ) ;
#32251=CARTESIAN_POINT ( 'NONE',  ( 810.4231160770870019, -192.5545181178801215, -321.9338519418446936 ) ) ;
#32252=PLANE ( 'NONE',  #39269 ) ;
#32257=CARTESIAN_POINT ( 'NONE',  ( 814.2001403089898304, -209.3618753856926276, -347.4397851343538264 ) ) ;
#32259=CARTESIAN_POINT ( 'NONE',  ( 754.8072714833581358, -4.816420840238714085, -338.1981804954720587 ) ) ;
#32261=CARTESIAN_POINT ( 'NONE',  ( 745.1769319972822814, -89.80559628986918597, -346.2694204179732083 ) ) ;
#32263=CARTESIAN_POINT ( 'NONE',  ( 796.9462024416508257, -348.4527844766012663, -308.9653473494370246 ) ) ;
#32269=CARTESIAN_POINT ( 'NONE',  ( 815.0009284576459549, -414.3510508353227237, -338.7629533639073429 ) ) ;
#32271=CARTESIAN_POINT ( 'NONE',  ( 801.1904061080336987, -428.0891481129644944, -368.3070685750235498 ) ) ;
#32277=CARTESIAN_POINT ( 'NONE',  ( 813.2346286133761168, -173.2601417444143692, -328.9521613784389160 ) ) ;
#32284=CARTESIAN_POINT ( 'NONE',  ( 767.7687537140311633, -47.90732993114767169, -372.7932403749916830 ) ) ;
#32287=CARTESIAN_POINT ( 'NONE',  ( 781.2370466360911223, -452.7363362996975411, -304.9990715423533629 ) ) ;
#32293=CARTESIAN_POINT ( 'NONE',  ( 755.5713283507202505, -293.3618753856923718, -334.6858677611754729 ) ) ;
#32298=CARTESIAN_POINT ( 'NONE',  ( 763.0428371773158460, -299.4636090269707438, -358.7617431975195359 ) ) ;
#32299=CARTESIAN_POINT ( 'NONE',  ( 764.8639956371174549, -296.0891481129650629, -319.7806653035542013 ) ) ;
#32301=CARTESIAN_POINT ( 'NONE',  ( 804.4286716492782716, -113.3618753856929260, -345.3141322388244703 ) ) ;
#32307=CARTESIAN_POINT ( 'NONE',  ( 746.4236121716829757, -87.82724539060770041, -328.8385539511384650 ) ) ;
#32313=CARTESIAN_POINT ( 'NONE',  ( 755.1538015810308480, -38.19088175424422360, -343.0433043558613804 ) ) ;
#32314=CARTESIAN_POINT ( 'NONE',  ( 814.9108240113580450, -88.27096629478390355, -337.5031285880265273 ) ) ;
#32317=DIRECTION ( 'NONE',  ( 0.000000000000000000, 0.000000000000000000, 1.000000000000000000 ) ) ;
#32320=CARTESIAN_POINT ( 'NONE',  ( 814.2001403089898304, -233.3618753856925423, -347.4397851343538264 ) ) ;
#32325=CARTESIAN_POINT ( 'NONE',  ( 800.1688906516307043, -298.1692326535049347, -369.0717654672308186 ) ) ;
#32327=CARTESIAN_POINT ( 'NONE',  ( 805.0032342141412300, -325.5436935675105019, -314.9967657858571783 ) ) ;
#32331=CARTESIAN_POINT ( 'NONE',  ( 771.1735550268778070, -417.1800572038736163, -316.3353852180827630 ) ) ;
#32334=CARTESIAN_POINT ( 'NONE',  ( 759.9864689768902508, -194.0891481129654039, -354.9819416627836404 ) ) ;
#32335=CARTESIAN_POINT ( 'NONE',  ( 771.2368401574024119, -85.44195992623282621, -374.2805881961240857 ) ) ;
#32339=CARTESIAN_POINT ( 'NONE',  ( 760.5453621957607311, -189.0783235625961822, -323.8424801807151425 ) ) ;
#32341=CARTESIAN_POINT ( 'NONE',  ( 756.1443688327750579, -21.62377810805121570, -314.3581564841659315 ) ) ;
#32346=ORIENTED_EDGE ( 'NONE', *, *, #19891, .F. ) ;
#32348=CARTESIAN_POINT ( 'NONE',  ( 745.5313806188320314, -351.2817908451523294, -333.7943932421247268 ) ) ;
#32352=CARTESIAN_POINT ( 'NONE',  ( 757.4527132478984868, -184.3726999360619629, -329.1273215169538844 ) ) ;
#32353=CARTESIAN_POINT ( 'NONE',  ( 756.3353852180819104, -197.9073299311472169, -331.1735550268788302 ) ) ;
#32354=CARTESIAN_POINT ( 'NONE',  ( 767.8955696845334842, -360.4527844766011526, -362.1676090361161755 ) ) ;
#32363=CARTESIAN_POINT ( 'NONE',  ( 745.1792804349281596, -398.1908817542431507, -343.7566961878542884 ) ) ;
#32365=CARTESIAN_POINT ( 'NONE',  ( 814.5518280994195948, 8.274488250670337663, -332.4837098697145166 ) ) ;
#32369=CARTESIAN_POINT ( 'NONE',  ( 801.9419747391806368, -354.4527844766012095, -351.9812246680014027 ) ) ;
#32374=CARTESIAN_POINT ( 'NONE',  ( 786.5483106153019435, -271.6454272087889876, -364.1601925771022366 ) ) ;
#32383=CARTESIAN_POINT ( 'NONE',  ( 779.9999999999992042, 166.4563064324884465, -350.0000000000000000 ) ) ;
#32385=CARTESIAN_POINT ( 'NONE',  ( 749.2812353651451076, -78.45278447660211896, -323.2262854647983090 ) ) ;
#32387=CARTESIAN_POINT ( 'NONE',  ( 797.6776695296629214, -307.5436935675104451, -357.6776695296636603 ) ) ;
#32388=DIRECTION ( 'NONE',  ( 1.000000000000000000, 0.000000000000000000, 0.000000000000000000 ) ) ;
#32391=CARTESIAN_POINT ( 'NONE',  ( 744.6391490659812007, -62.73633629969871350, -338.7502325331110455 ) ) ;
#32392=CARTESIAN_POINT ( 'NONE',  ( 799.4546378042377910, -81.07832356259649487, -356.1575198192848006 ) ) ;
#32397=CARTESIAN_POINT ( 'NONE',  ( 803.6646147819161570, 6.092670068852159559, -348.8264449731210561 ) ) ;
#32398=CARTESIAN_POINT ( 'NONE',  ( 761.2382568024794409, -111.6237781080509279, -356.9571628226838129 ) ) ;
#32400=CARTESIAN_POINT ( 'NONE',  ( 759.7806653035534055, -102.9982390220565520, -324.8639956371180801 ) ) ;
#32401=CARTESIAN_POINT ( 'NONE',  ( 764.0069404352550464, -399.0783235625955285, -359.2566176426627180 ) ) ;
#32404=CARTESIAN_POINT ( 'NONE',  ( 800.1688906516307043, -442.1692326535044231, -369.0717654672308186 ) ) ;
#32412=CARTESIAN_POINT ( 'NONE',  ( 798.5707757039680246, -77.46360902697138329, -356.7845633553585003 ) ) ;
#32414=CARTESIAN_POINT ( 'NONE',  ( 805.1927285166399315, -232.8164208402379529, -341.8018195045277707 ) ) ;
#32417=CARTESIAN_POINT ( 'NONE',  ( 774.6312213355099630, -383.3618753856921444, -364.6798772138717482 ) ) ;
#32418=CARTESIAN_POINT ( 'NONE',  ( 778.2165204200184689, -46.81642084023858530, -364.9363028652563230 ) ) ;
#32422=CARTESIAN_POINT ( 'NONE',  ( 767.8955696845333705, -24.45278447660229304, -362.1676090361162323 ) ) ;
#32426=CARTESIAN_POINT ( 'NONE',  ( 802.2119215644370342, -318.0090635724251911, -367.5423716828165084 ) ) ;
#32429=CARTESIAN_POINT ( 'NONE',  ( 762.1405469898971887, -265.5436935675106156, -357.8594530101015607 ) ) ;
#32431=CARTESIAN_POINT ( 'NONE',  ( 754.7162404726377645, -110.7363362996985501, -339.4709603349214717 ) ) ;
#32434=CARTESIAN_POINT ( 'NONE',  ( 751.2241431872005251, -16.16923265350578021, -359.9636004259367610 ) ) ;
#32435=CARTESIAN_POINT ( 'NONE',  ( 782.5225473063383106, -334.2709662947830793, -375.2698199232970637 ) ) ;
#32439=CARTESIAN_POINT ( 'NONE',  ( 805.9055244015594326, -195.6237781080506863, -315.8990559732753240 ) ) ;
#32441=CARTESIAN_POINT ( 'NONE',  ( 808.0189434323515343, 9.910851887033969021, -319.0252816721025511 ) ) ;
#32446=CARTESIAN_POINT ( 'NONE',  ( 790.8726784830453198, 13.28531280103958423, -362.5472867521010585 ) ) ;
#32452=CARTESIAN_POINT ( 'NONE',  ( 804.9511171171677688, -293.8055962898685607, -335.8780910478229202 ) ) ;
#32453=CARTESIAN_POINT ( 'NONE',  ( 773.7943932421234194, -311.8055962898685038, -305.5313806188329409 ) ) ;
#32454=DIRECTION ( 'NONE',  ( 0.000000000000000000, -1.000000000000000000, 0.000000000000000000 ) ) ;
#32458=CARTESIAN_POINT ( 'NONE',  ( 779.4709603349208464, -72.35105083532378956, -314.7162404726379918 ) ) ;
#32460=CARTESIAN_POINT ( 'NONE',  ( 796.9462024416508257, -156.4527844766018916, -308.9653473494370246 ) ) ;
#32462=CARTESIAN_POINT ( 'NONE',  ( 794.9819416627830151, -156.9982390220564241, -319.9864689768909898 ) ) ;
#32464=CARTESIAN_POINT ( 'NONE',  ( 772.4468031744293057, -441.8272453906066630, -363.8651313633793620 ) ) ;
#32472=CARTESIAN_POINT ( 'NONE',  ( 759.0159684113467620, -376.9181544815159555, -325.8855110935213020 ) ) ;
#32474=CARTESIAN_POINT ( 'NONE',  ( 745.1792804349281596, -158.1908817542438612, -343.7566961878542884 ) ) ;
#32476=DIRECTION ( 'NONE',  ( -1.000000000000000000, -0.000000000000000000, -0.000000000000000000 ) ) ;
#32478=CARTESIAN_POINT ( 'NONE',  ( 786.6156483768007774, -313.4419599262320730, -315.5913626894246136 ) ) ;
#32480=CARTESIAN_POINT ( 'NONE',  ( 778.7629533639073998, -176.7363362996983369, -375.0009284576466371 ) ) ;
#32484=CARTESIAN_POINT ( 'NONE',  ( 777.4774526936600978, -202.2709662947835341, -304.7301800767028226 ) ) ;
#32486=CARTESIAN_POINT ( 'NONE',  ( 774.6312213355099630, 0.6381246143067236254, -364.6798772138717482 ) ) ;
#32488=CARTESIAN_POINT ( 'NONE',  ( 756.1443688327750579, -93.62377810805098477, -314.3581564841659315 ) ) ;
#32490=CARTESIAN_POINT ( 'NONE',  ( 808.3070685750230950, -330.9982390220558273, -361.1904061080339261 ) ) ;
#32495=CARTESIAN_POINT ( 'NONE',  ( 800.1688906516307043, -418.1692326535044799, -369.0717654672308186 ) ) ;
#32496=CARTESIAN_POINT ( 'NONE',  ( 787.4397851343537695, -405.7255117493283478, -374.2001403089903988 ) ) ;
#32499=ORIENTED_EDGE ( 'NONE', *, *, #22985, .F. ) ;
#32501=CARTESIAN_POINT ( 'NONE',  ( 773.3843516231979720, -181.4419599262325278, -364.4086373105754433 ) ) ;
#32503=CARTESIAN_POINT ( 'NONE',  ( 761.9338519418445230, -206.5328690171415360, -370.4231160770881957 ) ) ;
#32508=CARTESIAN_POINT ( 'NONE',  ( 804.6798772138708955, -135.7255117493291152, -334.6312213355107019 ) ) ;
#32510=CARTESIAN_POINT ( 'NONE',  ( 772.4837098697144029, -47.36187538569312494, -374.5518280994205611 ) ) ;
#32512=CARTESIAN_POINT ( 'NONE',  ( 799.9636004259356241, -454.9181544815156713, -311.2241431872006956 ) ) ;
#32514=CARTESIAN_POINT ( 'NONE',  ( 802.5472867521000353, -316.3726999360615082, -350.8726784830461156 ) ) ;
#32517=CARTESIAN_POINT ( 'NONE',  ( 797.8594530101008786, -301.5436935675105588, -322.1405469898980982 ) ) ;
#32521=CARTESIAN_POINT ( 'NONE',  ( 754.7162404726377645, -302.7363362996979959, -339.4709603349214717 ) ) ;
#32522=CARTESIAN_POINT ( 'NONE',  ( 756.5762568750052424, -291.1800572038741848, -348.7366044899774238 ) ) ;
#32524=CARTESIAN_POINT ( 'NONE',  ( 797.8594530101008786, -109.5436935675110988, -322.1405469898980982 ) ) ;
#32529=CARTESIAN_POINT ( 'NONE',  ( 759.9999999999992042, -462.9681489794448339, -309.9999999999998863 ) ) ;
#32531=CARTESIAN_POINT ( 'NONE',  ( 766.4474001241216001, -67.09997266333506616, -307.3154664389482491 ) ) ;
#32538=CARTESIAN_POINT ( 'NONE',  ( 767.7687537140311633, -95.90732993114751537, -372.7932403749916830 ) ) ;
#32542=CARTESIAN_POINT ( 'NONE',  ( 796.7737145352015204, -236.6346026584198228, -370.7187646348536987 ) ) ;
#32546=CARTESIAN_POINT ( 'NONE',  ( 808.7758568127978833, -316.1692326535048210, -320.0363995740631822 ) ) ;
#32548=CARTESIAN_POINT ( 'NONE',  ( 759.0252816721024374, -312.9982390220559409, -368.0189434323527280 ) ) ;
#32553=CARTESIAN_POINT ( 'NONE',  ( 757.8323909638827445, -410.6346026584191122, -352.1044303154654358 ) ) ;
#32555=CARTESIAN_POINT ( 'NONE',  ( 774.6312213355099630, -215.3618753856925423, -364.6798772138717482 ) ) ;
#32556=CARTESIAN_POINT ( 'NONE',  ( 781.2497674668890113, -84.35105083532374692, -375.3608509340180603 ) ) ;
#32561=CARTESIAN_POINT ( 'NONE',  ( 757.2208543904082489, -232.7146871989596377, -350.9844846989624330 ) ) ;
#32563=CARTESIAN_POINT ( 'NONE',  ( 814.8230680027162407, -53.80559628986930676, -333.7305795820267917 ) ) ;
#32567=CARTESIAN_POINT ( 'NONE',  ( 748.6759233522253680, -352.3726999360614514, -324.3348316497537098 ) ) ;
#32572=CARTESIAN_POINT ( 'NONE',  ( 793.0897708529556667, -174.5545181178801784, -361.3366627262616362 ) ) ;
#32573=CARTESIAN_POINT ( 'NONE',  ( 759.9864689768902508, -194.0891481129654039, -354.9819416627836404 ) ) ;
#32574=VECTOR ( 'NONE', #21501, 1000.000000000000000 ) ;
#32575=CARTESIAN_POINT ( 'NONE',  ( 759.7806653035535192, -390.9982390220556567, -324.8639956371181370 ) ) ;
#32577=CARTESIAN_POINT ( 'NONE',  ( 769.1273215169530886, 25.28531280103955226, -317.4527132478988847 ) ) ;
#32580=DIRECTION ( 'NONE',  ( 0.000000000000000000, -1.000000000000000000, 0.000000000000000000 ) ) ;
#32587=CARTESIAN_POINT ( 'NONE',  ( 764.1737431748507561, -418.3726999360612808, -371.6461892240376415 ) ) ;
#32588=CARTESIAN_POINT ( 'NONE',  ( 813.1304606946831655, 6.092670068852160448, -352.3570229623691716 ) ) ;
#32591=CARTESIAN_POINT ( 'NONE',  ( 774.6858677611749044, -369.7255117493284615, -315.5713283507209894 ) ) ;
#32595=CARTESIAN_POINT ( 'NONE',  ( 760.7433823573367135, -252.0090635724254184, -355.9930595647440441 ) ) ;
#32605=CARTESIAN_POINT ( 'NONE',  ( 778.2165204200184689, -334.8164208402376403, -364.9363028652563230 ) ) ;
#32610=CARTESIAN_POINT ( 'NONE',  ( 786.2694204179717872, -69.28179084515321051, -305.1769319972829067 ) ) ;
#32611=CARTESIAN_POINT ( 'NONE',  ( 773.3843516231979720, -109.4419599262327836, -364.4086373105754433 ) ) ;
#32614=CARTESIAN_POINT ( 'NONE',  ( 764.8639956371174549, 15.91085188703394238, -319.7806653035542013 ) ) ;
#32615=CARTESIAN_POINT ( 'NONE',  ( 795.9930595647434757, -147.0783235625962959, -320.7433823573372820 ) ) ;
#32617=CARTESIAN_POINT ( 'NONE',  ( 803.4237431249931660, -111.1800572038747532, -331.2633955100225194 ) ) ;
#32618=CARTESIAN_POINT ( 'NONE',  ( 804.9511171171677688, -389.8055962898682765, -335.8780910478229202 ) ) ;
#32625=EDGE_LOOP ( 'NONE', ( #23284, #34928 ) ) ;
#32631=CARTESIAN_POINT ( 'NONE',  ( 779.4763451958990572, -80.73633629969864955, -365.0264073115438919 ) ) ;
#32633=CARTESIAN_POINT ( 'NONE',  ( 805.1927285166399315, -256.8164208402379245, -341.8018195045277707 ) ) ;
#32635=CARTESIAN_POINT ( 'NONE',  ( 785.3141322388236176, -381.7255117493284615, -364.4286716492789537 ) ) ;
#32636=CARTESIAN_POINT ( 'NONE',  ( 781.8018195045266339, -46.27096629478404566, -365.1927285166406705 ) ) ;
#32638=EDGE_CURVE ( 'NONE', #19609, #3824, #30434, .T. ) ;
#32642=CARTESIAN_POINT ( 'NONE',  ( 765.0180583372156207, -24.99823902205683268, -360.0135310231089534 ) ) ;
#32645=CARTESIAN_POINT ( 'NONE',  ( 755.8990559732751535, -299.4636090269707438, -365.9055244015606831 ) ) ;
#32646=AXIS2_PLACEMENT_3D ( 'NONE', #44686, #26216, #13044 ) ;
#32649=CARTESIAN_POINT ( 'NONE',  ( 771.1735550268778070, -249.1800572038742416, -316.3353852180827630 ) ) ;
#32651=CARTESIAN_POINT ( 'NONE',  ( 755.1538015810308480, -158.1908817542438612, -343.0433043558613804 ) ) ;
#32655=CARTESIAN_POINT ( 'NONE',  ( 744.9990715423526808, -18.35105083532395298, -341.2370466360926002 ) ) ;
#32656=CARTESIAN_POINT ( 'NONE',  ( 759.0252816721024374, -360.9982390220557704, -368.0189434323527280 ) ) ;
#32660=CARTESIAN_POINT ( 'NONE',  ( 814.8230680027162407, -245.8055962898686460, -333.7305795820267917 ) ) ;
#32662=CARTESIAN_POINT ( 'NONE',  ( 763.2262854647970016, 15.36539734157940629, -309.2812353651462445 ) ) ;
#32668=CARTESIAN_POINT ( 'NONE',  ( 761.2382568024794409, 8.376221891948691933, -356.9571628226838129 ) ) ;
#32673=ORIENTED_EDGE ( 'NONE', *, *, #43384, .T. ) ;
#32674=CARTESIAN_POINT ( 'NONE',  ( 770.0799878456142551, -301.9874144716867477, -362.9823548866085616 ) ) ;
#32676=CARTESIAN_POINT ( 'NONE',  ( 812.6845335610512393, -343.9874144716865771, -353.5525998758768651 ) ) ;
#32677=DIRECTION ( 'NONE',  ( 0.000000000000000000, -1.000000000000000000, 0.000000000000000000 ) ) ;
#32682=CARTESIAN_POINT ( 'NONE',  ( 803.2186876482843445, -79.98741447168740137, -350.0220218866286928 ) ) ;
#32685=CARTESIAN_POINT ( 'NONE',  ( 748.9653473494363425, -146.6346026584200217, -356.9462024416521331 ) ) ;
#32687=CARTESIAN_POINT ( 'NONE',  ( 801.9419747391806368, -138.4527844766019200, -351.9812246680014027 ) ) ;
#32689=CARTESIAN_POINT ( 'NONE',  ( 766.0291762391763086, -418.9181544815157849, -360.7704444035551319 ) ) ;
#32696=CARTESIAN_POINT ( 'NONE',  ( 755.3028492785439312, -399.2817908451522726, -335.9200461376539693 ) ) ;
#32699=CARTESIAN_POINT ( 'NONE',  ( 814.8207195650702488, -218.1908817542437191, -336.2433038121456548 ) ) ;
#32704=CARTESIAN_POINT ( 'NONE',  ( 775.9200461376533440, -311.8055962898685038, -315.3028492785443291 ) ) ;
#32706=CARTESIAN_POINT ( 'NONE',  ( 811.3240766477731540, -196.3726999360619061, -355.6651683502462902 ) ) ;
#32710=CARTESIAN_POINT ( 'NONE',  ( 759.0252816721024374, -240.9982390220561683, -368.0189434323527280 ) ) ;
#32712=CARTESIAN_POINT ( 'NONE',  ( 781.8018195045266339, -22.27096629478410250, -365.1927285166406705 ) ) ;
#32715=CARTESIAN_POINT ( 'NONE',  ( 746.0683387631852383, -115.4419599262327409, -331.3260364891676204 ) ) ;
#32717=CARTESIAN_POINT ( 'NONE',  ( 772.4837098697144029, -359.3618753856920875, -374.5518280994205611 ) ) ;
#32722=CARTESIAN_POINT ( 'NONE',  ( 751.2241431872005251, -400.1692326535045936, -359.9636004259367610 ) ) ;
#32723=CARTESIAN_POINT ( 'NONE',  ( 792.2312462859673587, -443.9073299311464780, -307.2067596250082602 ) ) ;
#32727=CARTESIAN_POINT ( 'NONE',  ( 805.1016975059191054, -198.8965053807779384, -343.0745993439771837 ) ) ;
#32730=CARTESIAN_POINT ( 'NONE',  ( 754.0944755984390895, -207.6237781080506295, -364.1009440267246760 ) ) ;
#32737=CARTESIAN_POINT ( 'NONE',  ( 781.7834795799800531, -154.8164208402382371, -315.0636971347436202 ) ) ;
#32739=CARTESIAN_POINT ( 'NONE',  ( 812.7932403749906598, -39.18005720387496638, -327.7687537140311633 ) ) ;
#32741=CARTESIAN_POINT ( 'NONE',  ( 791.0478386215596629, -429.8272453906067199, -306.7653713866226326 ) ) ;
#32742=ORIENTED_EDGE ( 'NONE', *, *, #18974, .F. ) ;
#32743=CARTESIAN_POINT ( 'NONE',  ( 755.8894580844503253, -303.8272453906071178, -332.3691319403863531 ) ) ;
#32750=CARTESIAN_POINT ( 'NONE',  ( 775.8780910478218402, -273.2817908451526137, -364.9511171171680530 ) ) ;
#32751=CARTESIAN_POINT ( 'NONE',  ( 797.8594530101008786, -277.5436935675105019, -322.1405469898980982 ) ) ;
#32753=CARTESIAN_POINT ( 'NONE',  ( 765.0180583372156207, -168.9982390220563673, -360.0135310231089534 ) ) ;
#32755=EDGE_LOOP ( 'NONE', ( #30345, #29976, #34129, #30116, #26087, #14273 ) ) ;
#32759=CARTESIAN_POINT ( 'NONE',  ( 814.4686193811664907, -99.28179084515313946, -346.2056067578752732 ) ) ;
#32766=CIRCLE ( 'NONE', #28323, 10.00000000000000888 ) ;
#32767=CARTESIAN_POINT ( 'NONE',  ( 748.9653473494365699, -122.6346026584201496, -356.9462024416520762 ) ) ;
#32771=CARTESIAN_POINT ( 'NONE',  ( 796.7737145352015204, -284.6346026584196807, -370.7187646348536987 ) ) ;
#32774=CARTESIAN_POINT ( 'NONE',  ( 754.0944755984390895, -303.6237781080503169, -364.1009440267246760 ) ) ;
#32775=AXIS2_PLACEMENT_3D ( 'NONE', #20954, #27435, #40159 ) ;
#32777=CARTESIAN_POINT ( 'NONE',  ( 808.3070685750230950, -354.9982390220557704, -361.1904061080339261 ) ) ;
#32781=CARTESIAN_POINT ( 'NONE',  ( 754.8072714833581358, -412.8164208402372992, -338.1981804954720587 ) ) ;
#32782=CARTESIAN_POINT ( 'NONE',  ( 805.9055244015594326, -99.62377810805098477, -315.8990559732753240 ) ) ;
#32788=CARTESIAN_POINT ( 'NONE',  ( 800.7704444035546203, -220.1692326535051052, -326.0291762391768771 ) ) ;
#32790=CARTESIAN_POINT ( 'NONE',  ( 795.6651683502461765, -58.71468719896019905, -371.3240766477733814 ) ) ;
#32792=CARTESIAN_POINT ( 'NONE',  ( 807.6521310549275086, -452.9681489794448339, -339.7933401739554711 ) ) ;
#32795=CARTESIAN_POINT ( 'NONE',  ( 815.3608509340175488, -338.7363362996978822, -341.2497674668889545 ) ) ;
#32798=CARTESIAN_POINT ( 'NONE',  ( 755.8894580844503253, -183.8272453906074020, -332.3691319403863531 ) ) ;
#32799=CARTESIAN_POINT ( 'NONE',  ( 801.9419747391806368, -186.4527844766017779, -351.9812246680014027 ) ) ;
#32800=CARTESIAN_POINT ( 'NONE',  ( 762.1405469898973024, -385.5436935675102745, -357.8594530101016176 ) ) ;
#32801=ORIENTED_EDGE ( 'NONE', *, *, #7988, .T. ) ;
#32804=AXIS2_PLACEMENT_3D ( 'NONE', #35270, #16822, #24188 ) ;
#32813=CARTESIAN_POINT ( 'NONE',  ( 752.7379699480933368, -420.0090635724249069, -361.9858362298580232 ) ) ;
#32814=CARTESIAN_POINT ( 'NONE',  ( 796.9462024416508257, -12.45278447660232324, -308.9653473494370246 ) ) ;
#32817=CARTESIAN_POINT ( 'NONE',  ( 774.6312213355099630, -407.3618753856920307, -364.6798772138717482 ) ) ;
#32818=CARTESIAN_POINT ( 'NONE',  ( 791.9812246680005501, 3.365397341579444479, -361.9419747391813189 ) ) ;
#32821=CARTESIAN_POINT ( 'NONE',  ( 766.0291762391763086, -250.9181544815163534, -360.7704444035551319 ) ) ;
#32832=CARTESIAN_POINT ( 'NONE',  ( 802.1676090361156639, -326.6346026584193396, -327.8955696845344505 ) ) ;
#32836=CARTESIAN_POINT ( 'NONE',  ( 773.7305795820266212, -81.28179084515319630, -374.8230680027170365 ) ) ;
#32837=CARTESIAN_POINT ( 'NONE',  ( 756.1348686366196716, -137.2601417444144829, -347.5531968255698416 ) ) ;
#32841=CARTESIAN_POINT ( 'NONE',  ( 800.0135310231082713, -14.08914811296595460, -325.0180583372163028 ) ) ;
#32842=CARTESIAN_POINT ( 'NONE',  ( 769.1273215169530886, -118.7146871989600072, -317.4527132478988847 ) ) ;
#32843=CARTESIAN_POINT ( 'NONE',  ( 762.3223304703356007, -127.5436935675110561, -322.3223304703362828 ) ) ;
#32847=CARTESIAN_POINT ( 'NONE',  ( 789.9200121543843807, -433.9874144716862361, -317.0176451133914384 ) ) ;
#32857=CARTESIAN_POINT ( 'NONE',  ( 763.0428371773158460, -83.46360902697136908, -358.7617431975195359 ) ) ;
#32859=CARTESIAN_POINT ( 'NONE',  ( 767.8955696845334842, -264.4527844766016074, -362.1676090361161755 ) ) ;
#32863=CARTESIAN_POINT ( 'NONE',  ( 804.6798772138708955, -399.7255117493283478, -334.6312213355107019 ) ) ;
#32864=CARTESIAN_POINT ( 'NONE',  ( 805.1927285166397041, -64.81642084023852135, -341.8018195045277707 ) ) ;
#32870=CARTESIAN_POINT ( 'NONE',  ( 814.8207195650702488, -26.19088175424427334, -336.2433038121456548 ) ) ;
#32874=CARTESIAN_POINT ( 'NONE',  ( 793.5525998758768083, -319.0999726633342561, -372.6845335610516941 ) ) ;
#32877=CARTESIAN_POINT ( 'NONE',  ( 759.9999999999992042, 205.0000000000000568, -339.9999999999999432 ) ) ;
#32878=CARTESIAN_POINT ( 'NONE',  ( 791.9812246680005501, -260.6346026584197375, -361.9419747391813189 ) ) ;
#32880=CARTESIAN_POINT ( 'NONE',  ( 755.5913626894240451, -157.6454272087893287, -346.6156483768012890 ) ) ;
#32883=AXIS2_PLACEMENT_3D ( 'NONE', #16811, #44517, #41513 ) ;
#32885=CARTESIAN_POINT ( 'NONE',  ( 748.9653473494365699, -362.6346026584193964, -356.9462024416520762 ) ) ;
#32886=FACE_OUTER_BOUND ( 'NONE', #19840, .T. ) ;
#32890=CARTESIAN_POINT ( 'NONE',  ( 749.8865473780648472, -236.5328690171414792, -322.1177392798429082 ) ) ;
#32892=CARTESIAN_POINT ( 'NONE',  ( 793.9861285913068514, -442.9180389616178672, -372.1637643035757606 ) ) ;
#32899=CARTESIAN_POINT ( 'NONE',  ( 800.7704444035546203, -4.169232653505813069, -326.0291762391768771 ) ) ;
#32909=CARTESIAN_POINT ( 'NONE',  ( 770.0799878456142551, -325.9874144716865771, -362.9823548866085616 ) ) ;
#32912=CARTESIAN_POINT ( 'NONE',  ( 788.7631598425961101, -313.4419599262320730, -305.7194118038759143 ) ) ;
#32913=CARTESIAN_POINT ( 'NONE',  ( 799.9999999999993179, 166.4563064324884465, -319.9999999999999432 ) ) ;
#32917=CARTESIAN_POINT ( 'NONE',  ( 755.8398074228967971, -67.44195992623289726, -333.4516893846970333 ) ) ;
#32919=DIRECTION ( 'NONE',  ( -1.000000000000000000, -0.000000000000000000, -0.000000000000000000 ) ) ;
#32921=CARTESIAN_POINT ( 'NONE',  ( 796.9462024416508257, -180.4527844766017211, -308.9653473494370246 ) ) ;
#32923=CARTESIAN_POINT ( 'NONE',  ( 762.1405469898973024, -169.5436935675108998, -357.8594530101016176 ) ) ;
#32925=CARTESIAN_POINT ( 'NONE',  ( 804.4086373105744769, -433.6454272087884760, -333.3843516231986541 ) ) ;
#32933=CARTESIAN_POINT ( 'NONE',  ( 757.0176451133909268, -445.0999726633338582, -349.9200121543848354 ) ) ;
#32935=CARTESIAN_POINT ( 'NONE',  ( 812.3518521366052028, -217.0999726633345972, -326.5853460496235243 ) ) ;
#32938=FACE_OUTER_BOUND ( 'NONE', #32755, .T. ) ;
#32939=CARTESIAN_POINT ( 'NONE',  ( 776.9566956441375396, -324.8965053807775121, -364.8461984189686405 ) ) ;
#32941=CARTESIAN_POINT ( 'NONE',  ( 747.6481478633932056, -181.0999726633347109, -353.4146539503763620 ) ) ;
#32946=CARTESIAN_POINT ( 'NONE',  ( 814.2001403089898304, -257.3618753856924286, -347.4397851343538264 ) ) ;
#32948=CARTESIAN_POINT ( 'NONE',  ( 795.1360043628807261, -20.08914811296592973, -360.2193346964456282 ) ) ;
#32951=CARTESIAN_POINT ( 'NONE',  ( 766.5853460496234675, -133.9874144716872024, -372.3518521366060554 ) ) ;
#32953=CARTESIAN_POINT ( 'NONE',  ( 787.4397851343537695, -381.7255117493284615, -374.2001403089903988 ) ) ;
#32960=CARTESIAN_POINT ( 'NONE',  ( 797.8594530101008786, -397.5436935675100472, -322.1405469898980982 ) ) ;
#32961=CARTESIAN_POINT ( 'NONE',  ( 813.1304606946830518, -449.9073299311463643, -352.3570229623690580 ) ) ;
#32962=CARTESIAN_POINT ( 'NONE',  ( 799.9999999999993179, -512.9681489794448908, -370.0000000000000000 ) ) ;
#32966=CARTESIAN_POINT ( 'NONE',  ( 804.9511171171677688, -173.8055962898689302, -335.8780910478229202 ) ) ;
#32968=CARTESIAN_POINT ( 'NONE',  ( 766.5853460496234675, -229.9874144716869466, -372.3518521366060554 ) ) ;
#32971=CARTESIAN_POINT ( 'NONE',  ( 803.4237431249931660, -87.18005720387481006, -331.2633955100225194 ) ) ;
#32974=CARTESIAN_POINT ( 'NONE',  ( 797.6776695296629214, -139.5436935675110135, -357.6776695296636603 ) ) ;
#32977=CARTESIAN_POINT ( 'NONE',  ( 745.7998596910086917, -77.36187538569302546, -332.5602148656461168 ) ) ;
#32978=AXIS2_PLACEMENT_3D ( 'NONE', #5819, #14067, #10589 ) ;
#32980=EDGE_LOOP ( 'NONE', ( #31412, #38361, #39898, #44030, #1645, #34421 ) ) ;
#32981=CARTESIAN_POINT ( 'NONE',  ( 796.9571628226829034, -23.46360902697155026, -321.2382568024804641 ) ) ;
#32984=CARTESIAN_POINT ( 'NONE',  ( 755.5913626894240451, -325.6454272087888739, -346.6156483768012890 ) ) ;
#32987=CARTESIAN_POINT ( 'NONE',  ( 759.7806653035534055, -318.9982390220557704, -324.8639956371180801 ) ) ;
#32988=VECTOR ( 'NONE', #6668, 1000.000000000000000 ) ;
#32992=CARTESIAN_POINT ( 'NONE',  ( 759.0159684113467620, -304.9181544815161828, -325.8855110935213020 ) ) ;
#32993=CARTESIAN_POINT ( 'NONE',  ( 785.3687786644884454, -299.3618753856922581, -315.3201227861279676 ) ) ;
#32995=CARTESIAN_POINT ( 'NONE',  ( 757.8323909638827445, -146.6346026584200217, -352.1044303154654358 ) ) ;
#33000=CARTESIAN_POINT ( 'NONE',  ( 802.2119215644370342, -78.00906357242591582, -367.5423716828165084 ) ) ;
#33001=CARTESIAN_POINT ( 'NONE',  ( 767.9999999999992042, 178.9475563372491251, -320.0000000000000000 ) ) ;
#33006=CARTESIAN_POINT ( 'NONE',  ( 800.9747183278959710, -132.9982390220564810, -311.9810565676471583 ) ) ;
#33010=CARTESIAN_POINT ( 'NONE',  ( 801.3366627262608972, -416.5328690171409107, -353.0897708529566899 ) ) ;
#33012=CARTESIAN_POINT ( 'NONE',  ( 814.9108240113580450, -280.2709662947833067, -337.5031285880265273 ) ) ;
#33016=CARTESIAN_POINT ( 'NONE',  ( 805.9055244015594326, -315.6237781080503169, -315.8990559732753240 ) ) ;
#33019=CARTESIAN_POINT ( 'NONE',  ( 744.7301800767019131, -364.8164208402374697, -337.4774526936615757 ) ) ;
#33020=DIRECTION ( 'NONE',  ( 0.000000000000000000, -1.000000000000000000, 0.000000000000000000 ) ) ;
#33024=CARTESIAN_POINT ( 'NONE',  ( 795.1360043628807261, -428.0891481129644944, -360.2193346964456282 ) ) ;
#33025=CARTESIAN_POINT ( 'NONE',  ( 759.7806653035534055, -222.9982390220561399, -324.8639956371180801 ) ) ;
#33026=CARTESIAN_POINT ( 'NONE',  ( 746.7653713866222915, -137.2601417444144829, -351.0478386215610271 ) ) ;
#33030=CARTESIAN_POINT ( 'NONE',  ( 760.5453621957607311, -237.0783235625960117, -323.8424801807151425 ) ) ;
#33032=CARTESIAN_POINT ( 'NONE',  ( 815.0009284576459549, -54.35105083532383219, -338.7629533639073429 ) ) ;
#33036=CARTESIAN_POINT ( 'NONE',  ( 815.3608509340175488, -362.7363362996977116, -341.2497674668889545 ) ) ;
#33039=MANIFOLD_SOLID_BREP ( 'Move Face1', #36504 ) ;
#33041=CARTESIAN_POINT ( 'NONE',  ( 783.0745993439762742, -200.1908817542436907, -365.1016975059196739 ) ) ;
#33042=CARTESIAN_POINT ( 'NONE',  ( 757.8323909638827445, -194.6346026584198796, -352.1044303154654358 ) ) ;
#33043=CARTESIAN_POINT ( 'NONE',  ( 768.0187753319979720, -368.6346026584193964, -318.0580252608186242 ) ) ;
#33044=ORIENTED_EDGE ( 'NONE', *, *, #771, .T. ) ;
#33045=CARTESIAN_POINT ( 'NONE',  ( 805.1016975059191054, 17.10349461922139369, -343.0745993439771837 ) ) ;
#33054=CARTESIAN_POINT ( 'NONE',  ( 793.5525998758768083, -415.0999726633340288, -372.6845335610516941 ) ) ;
#33055=CARTESIAN_POINT ( 'NONE',  ( 759.0252816721024374, -24.99823902205683268, -368.0189434323527280 ) ) ;
#33057=CARTESIAN_POINT ( 'NONE',  ( 788.7366044899766848, -395.9073299311465348, -316.5762568750059813 ) ) ;
#33058=CARTESIAN_POINT ( 'NONE',  ( 759.9864689768902508, -2.089148112965993231, -354.9819416627836404 ) ) ;
#33061=CARTESIAN_POINT ( 'NONE',  ( 802.9823548866075953, -241.0999726633345119, -330.0799878456151077 ) ) ;
#33062=CARTESIAN_POINT ( 'NONE',  ( 782.4968714119720516, -154.8164208402382371, -305.0891759886411023 ) ) ;
#33069=CARTESIAN_POINT ( 'NONE',  ( 804.9363028652555840, -304.2709662947832499, -338.2165204200192079 ) ) ;
#33071=CARTESIAN_POINT ( 'NONE',  ( 811.3240766477731540, -100.3726999360622187, -355.6651683502462902 ) ) ;
#33072=CARTESIAN_POINT ( 'NONE',  ( 783.0433043558608688, -120.8965053807781800, -315.1538015810313027 ) ) ;
#33077=CARTESIAN_POINT ( 'NONE',  ( 794.9819416627830151, -36.99823902205679360, -319.9864689768909898 ) ) ;
#33078=CARTESIAN_POINT ( 'NONE',  ( 789.9200121543843807, -121.9874144716872593, -317.0176451133914384 ) ) ;
#33079=CARTESIAN_POINT ( 'NONE',  ( 759.9864689768902508, -122.0891481129656171, -354.9819416627836404 ) ) ;
#33081=CARTESIAN_POINT ( 'NONE',  ( 756.7813123517142913, -427.9874144716862929, -329.9779781133712504 ) ) ;
#33088=EDGE_LOOP ( 'NONE', ( #29668, #39911, #35241, #21826, #11935, #38660, #17641, #13847 ) ) ;
#33092=ORIENTED_EDGE ( 'NONE', *, *, #6544, .F. ) ;
#33093=CARTESIAN_POINT ( 'NONE',  ( 761.4292242960306112, -89.46360902697134065, -323.2154366446414429 ) ) ;
#33094=CARTESIAN_POINT ( 'NONE',  ( 774.6312213355098493, -287.3618753856923718, -364.6798772138717482 ) ) ;
#33096=CARTESIAN_POINT ( 'NONE',  ( 768.0187753319979720, -392.6346026584193396, -318.0580252608186242 ) ) ;
#33097=CARTESIAN_POINT ( 'NONE',  ( 781.7834795799800531, -34.81642084023861372, -315.0636971347436202 ) ) ;
#33101=CARTESIAN_POINT ( 'NONE',  ( 788.6739635108323228, -31.64542720878970883, -373.9316612368139090 ) ) ;
#33104=CARTESIAN_POINT ( 'NONE',  ( 747.6481478633932056, -301.0999726633342561, -353.4146539503763620 ) ) ;
#33108=CARTESIAN_POINT ( 'NONE',  ( 801.9419747391806368, -282.4527844766014937, -351.9812246680014027 ) ) ;
#33109=CARTESIAN_POINT ( 'NONE',  ( 761.4292242960306112, -161.4636090269711133, -323.2154366446414429 ) ) ;
#33112=CARTESIAN_POINT ( 'NONE',  ( 771.2368401574024119, -13.44195992623305713, -374.2805881961240857 ) ) ;
#33113=CARTESIAN_POINT ( 'NONE',  ( 810.7187646348534145, -354.4527844766012095, -356.7737145352016341 ) ) ;
#33118=CARTESIAN_POINT ( 'NONE',  ( 805.9055244015594326, -243.6237781080504590, -315.8990559732753240 ) ) ;
#33120=CARTESIAN_POINT ( 'NONE',  ( 801.9858362298568863, -435.0783235625953580, -312.7379699480935642 ) ) ;
#33121=DIRECTION ( 'NONE',  ( 0.000000000000000000, 0.000000000000000000, -1.000000000000000000 ) ) ;
#33125=CARTESIAN_POINT ( 'NONE',  ( 779.4709603349208464, -24.35105083532392811, -314.7162404726379918 ) ) ;
#33130=CARTESIAN_POINT ( 'NONE',  ( 799.4546378042377910, -321.0783235625956991, -356.1575198192848006 ) ) ;
#33132=CARTESIAN_POINT ( 'NONE',  ( 791.1614460488616487, -323.2601417444138860, -373.5763878283158874 ) ) ;
#33137=CARTESIAN_POINT ( 'NONE',  ( 769.1273215169530886, -70.71468719896014932, -317.4527132478988847 ) ) ;
#33140=CARTESIAN_POINT ( 'NONE',  ( 745.0891759886404770, -172.2709662947836478, -342.4968714119734159 ) ) ;
#33143=CARTESIAN_POINT ( 'NONE',  ( 797.6776695296629214, -163.5436935675109567, -357.6776695296636603 ) ) ;
#33145=CARTESIAN_POINT ( 'NONE',  ( 796.1575198192839480, -438.0090635724247932, -359.4546378042384163 ) ) ;
#33152=CARTESIAN_POINT ( 'NONE',  ( 804.6971507214547046, -435.2817908451521021, -344.0799538623459739 ) ) ;
#33154=CARTESIAN_POINT ( 'NONE',  ( 810.4231160770870019, -192.5545181178801215, -321.9338519418446936 ) ) ;
#33157=CARTESIAN_POINT ( 'NONE',  ( 778.2165204200184689, -190.8164208402381234, -364.9363028652563230 ) ) ;
#33158=CARTESIAN_POINT ( 'NONE',  ( 795.9930595647434757, -339.0783235625956422, -320.7433823573372820 ) ) ;
#33160=CARTESIAN_POINT ( 'NONE',  ( 810.4231160770870019, -216.5545181178800931, -321.9338519418446936 ) ) ;
#33163=CARTESIAN_POINT ( 'NONE',  ( 766.9102291470427417, -42.55451811788057626, -318.6633372737382501 ) ) ;
#33166=CARTESIAN_POINT ( 'NONE',  ( 801.1904061080338124, -236.0891481129652334, -368.3070685750236066 ) ) ;
#33169=CARTESIAN_POINT ( 'NONE',  ( 756.5762568750052424, -27.18005720387500901, -348.7366044899774238 ) ) ;
#33170=AXIS2_PLACEMENT_3D ( 'NONE', #14170, #42585, #17649 ) ;
#33172=CARTESIAN_POINT ( 'NONE',  ( 805.9055244015594326, -147.6237781080508285, -315.8990559732753240 ) ) ;
#33174=CARTESIAN_POINT ( 'NONE',  ( 746.8695393053150156, -365.9073299311465917, -327.6429770376306010 ) ) ;
#33180=CARTESIAN_POINT ( 'NONE',  ( 804.4286716492782716, -401.3618753856920307, -345.3141322388244703 ) ) ;
#33181=CARTESIAN_POINT ( 'NONE',  ( 758.8095938919642549, -440.0891481129644944, -311.6929314249763365 ) ) ;
#33186=CARTESIAN_POINT ( 'NONE',  ( 761.2382568024794409, -207.6237781080506295, -356.9571628226838129 ) ) ;
#33188=CARTESIAN_POINT ( 'NONE',  ( 773.7943932421234194, -215.8055962898687881, -305.5313806188329409 ) ) ;
#33192=CARTESIAN_POINT ( 'NONE',  ( 759.7806653035534055, -150.9982390220563957, -324.8639956371180801 ) ) ;
#33194=CARTESIAN_POINT ( 'NONE',  ( 755.2512626584698410, -79.54369356751119824, -315.2512626584710915 ) ) ;
#33195=CARTESIAN_POINT ( 'NONE',  ( 792.1044303154646968, -60.45278447660216159, -317.8323909638837677 ) ) ;
#33197=CARTESIAN_POINT ( 'NONE',  ( 786.5483106153019435, -7.645427208789786100, -364.1601925771022366 ) ) ;
#33199=CARTESIAN_POINT ( 'NONE',  ( 763.8424801807145741, -306.0090635724252479, -320.5453621957614700 ) ) ;
#33208=CARTESIAN_POINT ( 'NONE',  ( 784.1219089521767955, -309.2817908451525568, -315.0488828828318333 ) ) ;
#33209=CARTESIAN_POINT ( 'NONE',  ( 802.1676090361156639, -302.6346026584196238, -327.8955696845344505 ) ) ;
#33210=CARTESIAN_POINT ( 'NONE',  ( 801.9419747391806368, -138.4527844766019200, -351.9812246680014027 ) ) ;
#33214=CARTESIAN_POINT ( 'NONE',  ( 802.2119215644370342, -102.0090635724258448, -367.5423716828165084 ) ) ;
#33220=CARTESIAN_POINT ( 'NONE',  ( 796.7737145352015204, -140.6346026584201070, -370.7187646348536987 ) ) ;
#33223=CARTESIAN_POINT ( 'NONE',  ( 787.4397851343537695, -285.7255117493286889, -374.2001403089903988 ) ) ;
#33224=CARTESIAN_POINT ( 'NONE',  ( 767.6429770376291799, -441.1800572038736163, -306.8695393053162093 ) ) ;
#33226=CARTESIAN_POINT ( 'NONE',  ( 798.0661480581538854, -338.5328690171411381, -309.5768839229118043 ) ) ;
#33227=CARTESIAN_POINT ( 'NONE',  ( 759.0252816721024374, -72.99823902205667991, -368.0189434323527280 ) ) ;
#33229=CARTESIAN_POINT ( 'NONE',  ( 745.0891759886404770, -364.2709662947830793, -342.4968714119734159 ) ) ;
#33233=CARTESIAN_POINT ( 'NONE',  ( 801.9858362298568863, -123.0783235625963385, -312.7379699480935642 ) ) ;
#33238=CARTESIAN_POINT ( 'NONE',  ( 801.3366627262608972, -248.5328690171414223, -353.0897708529566899 ) ) ;
#33240=CARTESIAN_POINT ( 'NONE',  ( 808.0189434323515343, 9.910851887033969021, -319.0252816721025511 ) ) ;
#33241=CARTESIAN_POINT ( 'NONE',  ( 745.1769319972822814, -65.80559628986925702, -346.2694204179732083 ) ) ;
#33244=CARTESIAN_POINT ( 'NONE',  ( 797.8822607201568644, -390.5545181178794678, -370.1134526219340160 ) ) ;
#33247=CARTESIAN_POINT ( 'NONE',  ( 759.0159684113467620, -208.9181544815164102, -325.8855110935213020 ) ) ;
#33248=CARTESIAN_POINT ( 'NONE',  ( 765.0180583372156207, -168.9982390220563673, -360.0135310231089534 ) ) ;
#33249=CARTESIAN_POINT ( 'NONE',  ( 800.0135310231082713, -374.0891481129647786, -325.0180583372163028 ) ) ;
#33252=CARTESIAN_POINT ( 'NONE',  ( 795.1360043628807261, -116.0891481129656029, -360.2193346964456282 ) ) ;
#33262=CARTESIAN_POINT ( 'NONE',  ( 771.3260364891663130, -403.6454272087884760, -306.0683387631859773 ) ) ;
#33263=CARTESIAN_POINT ( 'NONE',  ( 804.7487373415286811, -19.54369356751139364, -364.7487373415288516 ) ) ;
#33265=CARTESIAN_POINT ( 'NONE',  ( 805.1927285166397041, -400.8164208402373561, -341.8018195045277707 ) ) ;
#33266=CARTESIAN_POINT ( 'NONE',  ( 797.6776695296629214, -19.54369356751139364, -357.6776695296636603 ) ) ;
#33269=CARTESIAN_POINT ( 'NONE',  ( 805.2837595273609850, -266.7363362996981095, -340.5290396650784714 ) ) ;
#33270=CARTESIAN_POINT ( 'NONE',  ( 744.7301800767019131, -148.8164208402382656, -337.4774526936615757 ) ) ;
#33273=CARTESIAN_POINT ( 'NONE',  ( 795.1616405723528942, 16.45630643248848912, -314.3282859078202591 ) ) ;
#33275=DIRECTION ( 'NONE',  ( -0.3826814224632280603, -1.110223024625159854E-14, 0.9238803650373355048 ) ) ;
#33277=CARTESIAN_POINT ( 'NONE',  ( 781.7834795799800531, -322.8164208402377540, -315.0636971347436202 ) ) ;
#33280=CARTESIAN_POINT ( 'NONE',  ( 773.7305795820266212, -105.2817908451530968, -374.8230680027170365 ) ) ;
#33281=CARTESIAN_POINT ( 'NONE',  ( 801.3366627262608972, -128.5328690171417634, -353.0897708529566899 ) ) ;
#33284=CARTESIAN_POINT ( 'NONE',  ( 797.8594530101008786, -37.54369356751132614, -322.1405469898980982 ) ) ;
#33285=CARTESIAN_POINT ( 'NONE',  ( 789.9200121543843807, -145.9874144716871740, -317.0176451133914384 ) ) ;
#33286=CARTESIAN_POINT ( 'NONE',  ( 768.0187753319979720, -128.6346026584201354, -318.0580252608186242 ) ) ;
#33288=CARTESIAN_POINT ( 'NONE',  ( 756.1443688327750579, 26.37622189194863509, -314.3581564841659315 ) ) ;
#33292=VERTEX_POINT ( 'NONE', #1741 ) ;
#33294=CARTESIAN_POINT ( 'NONE',  ( 760.0363995740630116, -274.9181544815161828, -368.7758568127991907 ) ) ;
#33301=CARTESIAN_POINT ( 'NONE',  ( 804.4086373105744769, -97.64542720878949922, -333.3843516231986541 ) ) ;
#33302=CARTESIAN_POINT ( 'NONE',  ( 762.3223304703356007, -295.5436935675105588, -322.3223304703362828 ) ) ;
#33304=CARTESIAN_POINT ( 'NONE',  ( 765.0180583372156207, -408.9982390220556567, -360.0135310231089534 ) ) ;
#33305=CARTESIAN_POINT ( 'NONE',  ( 788.8264449731200330, -93.18005720387481006, -363.6646147819171233 ) ) ;
#33309=CARTESIAN_POINT ( 'NONE',  ( 813.5763878283155464, -3.827245390607979303, -351.1614460488615350 ) ) ;
#33312=CARTESIAN_POINT ( 'NONE',  ( 768.9521613784389729, -297.8272453906070041, -373.2346286133773106 ) ) ;
#33314=CARTESIAN_POINT ( 'NONE',  ( 802.1676090361156639, -278.6346026584196807, -327.8955696845344505 ) ) ;
#33316=CARTESIAN_POINT ( 'NONE',  ( 780.5236548040995785, -140.7363362996984506, -314.9735926884559944 ) ) ;
#33320=CARTESIAN_POINT ( 'NONE',  ( 763.0537975583476964, -360.4527844766011526, -371.0346526505628617 ) ) ;
#33325=CARTESIAN_POINT ( 'NONE',  ( 782.5225473063381969, 1.729033705215812011, -375.2698199232970637 ) ) ;
#33330=CARTESIAN_POINT ( 'NONE',  ( 789.9200121543843807, -25.98741447168755769, -317.0176451133914384 ) ) ;
#33336=CARTESIAN_POINT ( 'NONE',  ( 754.9735926884551418, -330.3510508353229511, -340.5236548041000333 ) ) ;
#33339=CARTESIAN_POINT ( 'NONE',  ( 752.4576283171824116, -333.0783235625956991, -317.7880784355627952 ) ) ;
#33341=ORIENTED_EDGE ( 'NONE', *, *, #26355, .F. ) ;
#33346=CARTESIAN_POINT ( 'NONE',  ( 772.4837098697144029, -191.3618753856925991, -374.5518280994205611 ) ) ;
#33350=CARTESIAN_POINT ( 'NONE',  ( 778.2165204200184689, -190.8164208402381234, -364.9363028652563230 ) ) ;
#33352=CARTESIAN_POINT ( 'NONE',  ( 793.0897708529556667, -414.5545181178795247, -361.3366627262616362 ) ) ;
#33355=DIRECTION ( 'NONE',  ( -0.000000000000000000, -1.110223024625155554E-15, -1.000000000000000000 ) ) ;
#33358=CARTESIAN_POINT ( 'NONE',  ( 798.5707757039680246, -413.4636090269704027, -356.7845633553585003 ) ) ;
#33360=CARTESIAN_POINT ( 'NONE',  ( 813.5763878283155464, -195.8272453906074304, -351.1614460488615350 ) ) ;
#33362=DIRECTION ( 'NONE',  ( 0.000000000000000000, -1.000000000000000000, 0.000000000000000000 ) ) ;
#33363=CARTESIAN_POINT ( 'NONE',  ( 762.1405469898971887, -193.5436935675108714, -357.8594530101015607 ) ) ;
#33364=CARTESIAN_POINT ( 'NONE',  ( 755.0488828828309806, -377.8055962898682765, -344.1219089521771934 ) ) ;
#33366=CARTESIAN_POINT ( 'NONE',  ( 799.9636004259356241, -214.9181544815164386, -311.2241431872006956 ) ) ;
#33369=CARTESIAN_POINT ( 'NONE',  ( 793.0897708529556667, -54.55451811788054783, -361.3366627262616362 ) ) ;
#33372=CARTESIAN_POINT ( 'NONE',  ( 805.0032342141413437, -253.5436935675105588, -314.9967657858572352 ) ) ;
#33375=CARTESIAN_POINT ( 'NONE',  ( 805.1927285166397041, -64.81642084023852135, -341.8018195045277707 ) ) ;
#33377=CARTESIAN_POINT ( 'NONE',  ( 813.2346286133761168, -125.2601417444145255, -328.9521613784389160 ) ) ;
#33379=CARTESIAN_POINT ( 'NONE',  ( 745.7998596910086917, -365.3618753856920875, -332.5602148656461168 ) ) ;
#33384=CARTESIAN_POINT ( 'NONE',  ( 762.1405469898971887, -385.5436935675102745, -357.8594530101015607 ) ) ;
#33386=CARTESIAN_POINT ( 'NONE',  ( 767.6429770376289525, -441.1800572038735027, -306.8695393053162093 ) ) ;
#33390=ADVANCED_FACE ( 'NONE', ( #5221 ), #8709, .F. ) ;
#33392=CARTESIAN_POINT ( 'NONE',  ( 793.2243759319678702, -218.5328690171414792, -318.4439275373583200 ) ) ;
#33394=CARTESIAN_POINT ( 'NONE',  ( 800.1688906516307043, -226.1692326535051052, -369.0717654672308186 ) ) ;
#33398=CARTESIAN_POINT ( 'NONE',  ( 774.6312213355099630, -143.3618753856927697, -364.6798772138717482 ) ) ;
#33400=EDGE_CURVE ( 'NONE', #45689, #911, #15844, .T. ) ;
#33401=CARTESIAN_POINT ( 'NONE',  ( 814.9108240113580450, -88.27096629478390355, -337.5031285880265273 ) ) ;
#33403=CARTESIAN_POINT ( 'NONE',  ( 759.9864689768902508, -74.08914811296577341, -354.9819416627836404 ) ) ;
#33405=CARTESIAN_POINT ( 'NONE',  ( 761.4292242960306112, 6.536390973028352924, -323.2154366446414429 ) ) ;
#33407=CARTESIAN_POINT ( 'NONE',  ( 787.5531968255692163, -333.8272453906070041, -316.1348686366205811 ) ) ;
#33414=CARTESIAN_POINT ( 'NONE',  ( 799.2566176426618085, -336.0090635724251911, -324.0069404352559559 ) ) ;
#33415=CARTESIAN_POINT ( 'NONE',  ( 771.2633955100217236, -311.9073299311468759, -363.4237431249939618 ) ) ;
#33416=CARTESIAN_POINT ( 'NONE',  ( 758.0580252608178853, -150.4527844766018916, -328.0187753319985404 ) ) ;
#33422=CARTESIAN_POINT ( 'NONE',  ( 773.7305795820266212, -129.2817908451530400, -374.8230680027170365 ) ) ;
#33428=CARTESIAN_POINT ( 'NONE',  ( 763.0537975583476964, -144.4527844766018632, -371.0346526505628617 ) ) ;
#33431=CARTESIAN_POINT ( 'NONE',  ( 748.9653473494363425, -266.6346026584197375, -356.9462024416521331 ) ) ;
#33432=CARTESIAN_POINT ( 'NONE',  ( 796.7737145352015204, -452.6346026584191691, -370.7187646348536987 ) ) ;
#33436=CARTESIAN_POINT ( 'NONE',  ( 768.8385539511368734, -335.2601417444137724, -306.4236121716840557 ) ) ;
#33438=CARTESIAN_POINT ( 'NONE',  ( 777.4774526936600978, -82.27096629478388934, -304.7301800767027657 ) ) ;
#33441=CARTESIAN_POINT ( 'NONE',  ( 772.4837098697144029, -335.3618753856920307, -374.5518280994205611 ) ) ;
#33446=CARTESIAN_POINT ( 'NONE',  ( 768.0187753319979720, -224.6346026584198228, -318.0580252608186242 ) ) ;
#33447=CARTESIAN_POINT ( 'NONE',  ( 803.8556311672234642, -105.6237781080509421, -365.6418435158340117 ) ) ;
#33452=AXIS2_PLACEMENT_3D ( 'NONE', #12162, #37548, #41021 ) ;
#33455=CARTESIAN_POINT ( 'NONE',  ( 811.0346526505616112, 9.365397341579420498, -323.0537975583477532 ) ) ;
#33459=CARTESIAN_POINT ( 'NONE',  ( 812.3518521366052028, -385.0999726633340856, -326.5853460496235243 ) ) ;
#33460=CARTESIAN_POINT ( 'NONE',  ( 795.1360043628807261, -236.0891481129651766, -360.2193346964456282 ) ) ;
#33463=CARTESIAN_POINT ( 'NONE',  ( 804.8461984189677878, -218.1908817542437191, -336.9566956441385628 ) ) ;
#33464=CARTESIAN_POINT ( 'NONE',  ( 758.0580252608178853, -222.4527844766016642, -328.0187753319985404 ) ) ;
#33466=CARTESIAN_POINT ( 'NONE',  ( 792.1044303154646968, -396.4527844766010958, -317.8323909638837677 ) ) ;
#33470=CARTESIAN_POINT ( 'NONE',  ( 755.5713283507202505, -101.3618753856929544, -334.6858677611754729 ) ) ;
#33480=CARTESIAN_POINT ( 'NONE',  ( 786.2694204179717872, -453.2817908451519315, -305.1769319972829067 ) ) ;
#33481=CARTESIAN_POINT ( 'NONE',  ( 815.2698199232962679, -40.81642084023859951, -342.5225473063383674 ) ) ;
#33483=CARTESIAN_POINT ( 'NONE',  ( 758.0580252608178853, -390.4527844766011526, -328.0187753319985404 ) ) ;
#33484=CARTESIAN_POINT ( 'NONE',  ( 755.5713283507202505, -5.361875385693257279, -334.6858677611754729 ) ) ;
#33488=CARTESIAN_POINT ( 'NONE',  ( 783.0745993439762742, -296.1908817542434917, -365.1016975059196739 ) ) ;
#33489=CARTESIAN_POINT ( 'NONE',  ( 812.7932403749906598, -159.1800572038746111, -327.7687537140311633 ) ) ;
#33492=CARTESIAN_POINT ( 'NONE',  ( 779.9999999999992042, -462.9681489794448339, -339.9999999999999432 ) ) ;
#33497=CARTESIAN_POINT ( 'NONE',  ( 756.5762568750052424, -363.1800572038739006, -348.7366044899774238 ) ) ;
#33500=AXIS2_PLACEMENT_3D ( 'NONE', #14908, #4506, #1030 ) ;
#33502=CARTESIAN_POINT ( 'NONE',  ( 745.1792804349281596, -86.19088175424408860, -343.7566961878542884 ) ) ;
#33503=CARTESIAN_POINT ( 'NONE',  ( 756.1348686366196716, -113.2601417444145682, -347.5531968255698416 ) ) ;
#33507=CARTESIAN_POINT ( 'NONE',  ( 771.1735550268778070, -33.18005720387498769, -316.3353852180827630 ) ) ;
#33508=CARTESIAN_POINT ( 'NONE',  ( 793.2243759319678702, -122.5328690171417918, -318.4439275373583200 ) ) ;
#33509=CARTESIAN_POINT ( 'NONE',  ( 778.2165204200184689, -118.8164208402383508, -364.9363028652563230 ) ) ;
#33512=CARTESIAN_POINT ( 'NONE',  ( 763.2154366446407039, -429.6237781080499190, -321.4292242960311228 ) ) ;
#33517=CARTESIAN_POINT ( 'NONE',  ( 791.0478386215596629, -285.8272453906071178, -306.7653713866226326 ) ) ;
#33525=CARTESIAN_POINT ( 'NONE',  ( 799.2566176426618085, -120.0090635724258021, -324.0069404352559559 ) ) ;
#33526=CARTESIAN_POINT ( 'NONE',  ( 756.5762568750052424, -99.18005720387478164, -348.7366044899774238 ) ) ;
#33527=CARTESIAN_POINT ( 'NONE',  ( 781.7834795799800531, -274.8164208402378108, -315.0636971347436202 ) ) ;
#33529=CARTESIAN_POINT ( 'NONE',  ( 767.8955696845333705, -432.4527844766008684, -362.1676090361162323 ) ) ;
#33530=CARTESIAN_POINT ( 'NONE',  ( 778.2165204200184689, -70.81642084023850714, -364.9363028652563230 ) ) ;
#33537=CARTESIAN_POINT ( 'NONE',  ( 795.8262568251477660, -358.3726999360613945, -308.3538107759623585 ) ) ;
#33541=CARTESIAN_POINT ( 'NONE',  ( 803.4237431249931660, -303.1800572038740711, -331.2633955100225194 ) ) ;
#33543=CARTESIAN_POINT ( 'NONE',  ( 800.9840315886518738, -148.9181544815166092, -354.1144889064786412 ) ) ;
#33546=CARTESIAN_POINT ( 'NONE',  ( 805.0032342141413437, -397.5436935675101040, -314.9967657858572352 ) ) ;
#33551=CARTESIAN_POINT ( 'NONE',  ( 782.5225473063381969, -22.27096629478410250, -375.2698199232970637 ) ) ;
#33558=CARTESIAN_POINT ( 'NONE',  ( 795.9930595647434757, -3.078323562596726681, -320.7433823573372820 ) ) ;
#33559=DIRECTION ( 'NONE',  ( -0.3826814224632300032, 0.000000000000000000, 0.9238803650373347276 ) ) ;
#33563=CARTESIAN_POINT ( 'NONE',  ( 804.9363028652555840, -40.27096629478405987, -338.2165204200192079 ) ) ;
#33565=CARTESIAN_POINT ( 'NONE',  ( 790.8726784830453198, -322.7146871989593819, -362.5472867521010585 ) ) ;
#33568=CARTESIAN_POINT ( 'NONE',  ( 811.6461892240364477, -340.7146871989592114, -324.1737431748509835 ) ) ;
#33575=CARTESIAN_POINT ( 'NONE',  ( 777.5031285880264704, -190.8164208402381234, -374.9108240113588408 ) ) ;
#33579=CARTESIAN_POINT ( 'NONE',  ( 800.2193346964446619, -162.9982390220563673, -355.1360043628816925 ) ) ;
#33581=CARTESIAN_POINT ( 'NONE',  ( 804.6798772138708955, 8.274488250670337663, -334.6312213355107019 ) ) ;
#33589=CARTESIAN_POINT ( 'NONE',  ( 786.5483106153019435, -415.6454272087885897, -364.1601925771022366 ) ) ;
#33592=CARTESIAN_POINT ( 'NONE',  ( 799.9636004259356241, -238.9181544815163534, -311.2241431872006956 ) ) ;
#33595=CARTESIAN_POINT ( 'NONE',  ( 762.3223304703356007, -199.5436935675108430, -322.3223304703362828 ) ) ;
#33596=CARTESIAN_POINT ( 'NONE',  ( 804.9511171171677688, -365.8055962898682765, -335.8780910478229202 ) ) ;
#33598=CARTESIAN_POINT ( 'NONE',  ( 760.0363995740630116, -226.9181544815163534, -368.7758568127991907 ) ) ;
#33601=CARTESIAN_POINT ( 'NONE',  ( 755.3028492785439312, -63.28179084515324604, -335.9200461376539693 ) ) ;
#33604=CARTESIAN_POINT ( 'NONE',  ( 745.0891759886404770, -244.2709662947834204, -342.4968714119734159 ) ) ;
#33608=CARTESIAN_POINT ( 'NONE',  ( 759.7806653035534055, -54.99823902205672255, -324.8639956371180801 ) ) ;
#33611=CARTESIAN_POINT ( 'NONE',  ( 778.7502325331095108, -144.3510508353235764, -304.6391490659818828 ) ) ;
#33613=CARTESIAN_POINT ( 'NONE',  ( 811.0346526505616112, -374.6346026584192828, -323.0537975583477532 ) ) ;
#33618=CARTESIAN_POINT ( 'NONE',  ( 800.0135310231082713, -398.0891481129647218, -325.0180583372163028 ) ) ;
#33621=CARTESIAN_POINT ( 'NONE',  ( 755.2512626584698410, -439.5436935675101040, -315.2512626584710915 ) ) ;
#33622=DIRECTION ( 'NONE',  ( 0.000000000000000000, 0.000000000000000000, 1.000000000000000000 ) ) ;
#33625=CARTESIAN_POINT ( 'NONE',  ( 755.8398074228967971, -211.4419599262324709, -333.4516893846970333 ) ) ;
#33626=CARTESIAN_POINT ( 'NONE',  ( 755.5713283507202505, -125.3618753856928834, -334.6858677611754729 ) ) ;
#33628=CARTESIAN_POINT ( 'NONE',  ( 746.0683387631852383, -235.4419599262323857, -331.3260364891676204 ) ) ;
#33632=CARTESIAN_POINT ( 'NONE',  ( 803.4237431249931660, -183.1800572038744974, -331.2633955100225194 ) ) ;
#33634=CARTESIAN_POINT ( 'NONE',  ( 792.3570229623688874, -69.18005720387488111, -373.1304606946836202 ) ) ;
#33635=CARTESIAN_POINT ( 'NONE',  ( 768.0187753319979720, -80.63460265842029173, -318.0580252608186242 ) ) ;
#33637=CARTESIAN_POINT ( 'NONE',  ( 769.9779781133707957, -19.09997266333520116, -316.7813123517150871 ) ) ;
#33640=CARTESIAN_POINT ( 'NONE',  ( 755.3028492785439312, -351.2817908451523294, -335.9200461376539693 ) ) ;
#33648=CARTESIAN_POINT ( 'NONE',  ( 793.9708237608222134, -334.9181544815160692, -319.2295555964448681 ) ) ;
#33649=CARTESIAN_POINT ( 'NONE',  ( 758.0580252608178853, -318.4527844766014368, -328.0187753319985404 ) ) ;
#33650=CARTESIAN_POINT ( 'NONE',  ( 791.9812246680005501, -164.6346026584200217, -361.9419747391813189 ) ) ;
#33655=CARTESIAN_POINT ( 'NONE',  ( 754.8983024940795303, -258.8965053807777963, -336.9254006560228163 ) ) ;
#33656=CARTESIAN_POINT ( 'NONE',  ( 764.1737431748507561, -106.3726999360621903, -371.6461892240376415 ) ) ;
#33665=CARTESIAN_POINT ( 'NONE',  ( 782.4968714119720516, -154.8164208402382371, -305.0891759886411023 ) ) ;
#33668=CARTESIAN_POINT ( 'NONE',  ( 796.9462024416508257, -252.4527844766015789, -308.9653473494370246 ) ) ;
#33672=CARTESIAN_POINT ( 'NONE',  ( 771.2368401574024119, -325.4419599262320162, -374.2805881961240857 ) ) ;
#33674=CARTESIAN_POINT ( 'NONE',  ( 745.0891759886404770, -100.2709662947838609, -342.4968714119734159 ) ) ;
#33676=CARTESIAN_POINT ( 'NONE',  ( 758.8095938919642549, -368.0891481129647786, -311.6929314249763365 ) ) ;
#33681=CARTESIAN_POINT ( 'NONE',  ( 807.5423716828161105, -105.0783235625964096, -362.2119215644372048 ) ) ;
#33688=CARTESIAN_POINT ( 'NONE',  ( 764.0069404352550464, -15.07832356259669560, -359.2566176426627180 ) ) ;
#33691=CARTESIAN_POINT ( 'NONE',  ( 768.8385539511368734, -431.2601417444136018, -306.4236121716840557 ) ) ;
#33695=CARTESIAN_POINT ( 'NONE',  ( 788.6739635108323228, -367.6454272087886466, -373.9316612368139090 ) ) ;
#33699=CARTESIAN_POINT ( 'NONE',  ( 804.6971507214547046, -219.2817908451527558, -344.0799538623459739 ) ) ;
#33700=CARTESIAN_POINT ( 'NONE',  ( 792.1044303154645831, -204.4527844766016926, -317.8323909638837677 ) ) ;
#33701=CARTESIAN_POINT ( 'NONE',  ( 771.1735550268780344, -417.1800572038736732, -316.3353852180828198 ) ) ;
#33704=CARTESIAN_POINT ( 'NONE',  ( 795.1360043628807261, -92.08914811296568814, -360.2193346964456282 ) ) ;
#33709=CARTESIAN_POINT ( 'NONE',  ( 787.0645410984409409, 17.59807796021646098, -310.5263297651933954 ) ) ;
#33716=CARTESIAN_POINT ( 'NONE',  ( 771.3260364891663130, -451.6454272087884192, -306.0683387631859773 ) ) ;
#33717=CARTESIAN_POINT ( 'NONE',  ( 751.6929314249750860, -30.99823902205680781, -318.8095938919659034 ) ) ;
#33719=CARTESIAN_POINT ( 'NONE',  ( 803.4237431249931660, -399.1800572038738437, -331.2633955100225194 ) ) ;
#33720=CARTESIAN_POINT ( 'NONE',  ( 803.4237431249931660, -15.18005720387504631, -331.2633955100225194 ) ) ;
#33723=CARTESIAN_POINT ( 'NONE',  ( 754.7162404726377645, -278.7363362996980527, -339.4709603349214717 ) ) ;
#33724=CARTESIAN_POINT ( 'NONE',  ( 814.2001403089898304, -161.3618753856927697, -347.4397851343538264 ) ) ;
#33729=CARTESIAN_POINT ( 'NONE',  ( 793.9408588713487234, 16.45630643248830438, -314.6714885282663090 ) ) ;
#33734=CARTESIAN_POINT ( 'NONE',  ( 755.3201227861273992, -339.7255117493285184, -345.3687786644892981 ) ) ;
#33736=CARTESIAN_POINT ( 'NONE',  ( 745.7194118038753459, -109.6454272087894566, -348.7631598425976449 ) ) ;
#33737=CARTESIAN_POINT ( 'NONE',  ( 794.1144889064781864, -154.1692326535053894, -360.9840315886528401 ) ) ;
#33741=EDGE_CURVE ( 'NONE', #15749, #37618, #16046, .T. ) ;
#33742=CARTESIAN_POINT ( 'NONE',  ( 797.6776695296629214, -43.54369356751131903, -357.6776695296636603 ) ) ;
#33743=CARTESIAN_POINT ( 'NONE',  ( 754.9735926884551418, -162.3510508353235196, -340.5236548041000333 ) ) ;
#33746=CARTESIAN_POINT ( 'NONE',  ( 805.0264073115434940, -438.3510508353226669, -339.4763451958999099 ) ) ;
#33748=CARTESIAN_POINT ( 'NONE',  ( 767.9999999999992042, 205.0000000000000568, -319.9999999999999432 ) ) ;
#33751=CARTESIAN_POINT ( 'NONE',  ( 754.3581564841646241, -281.4636090269706870, -316.1443688327762516 ) ) ;
#33758=CARTESIAN_POINT ( 'NONE',  ( 787.5531968255692163, -117.8272453906076151, -316.1348686366205811 ) ) ;
#33759=CARTESIAN_POINT ( 'NONE',  ( 785.3141322388236176, -117.7255117493292715, -364.4286716492789537 ) ) ;
#33760=CARTESIAN_POINT ( 'NONE',  ( 778.2165204200184689, -286.8164208402378677, -364.9363028652563230 ) ) ;
#33763=CARTESIAN_POINT ( 'NONE',  ( 800.2193346964447755, -426.9982390220554862, -355.1360043628815788 ) ) ;
#33764=CARTESIAN_POINT ( 'NONE',  ( 756.3353852180819104, -77.90732993114757221, -331.1735550268788302 ) ) ;
#33767=CARTESIAN_POINT ( 'NONE',  ( 779.9999999999992042, 16.45630643248849267, -339.9999999999999432 ) ) ;
#33772=CARTESIAN_POINT ( 'NONE',  ( 757.7880784355613741, -354.0090635724250774, -312.4576283171834916 ) ) ;
#33774=CARTESIAN_POINT ( 'NONE',  ( 774.6858677611749044, -297.7255117493286889, -315.5713283507209894 ) ) ;
#33776=CARTESIAN_POINT ( 'NONE',  ( 804.4086373105744769, -169.6454272087892718, -333.3843516231986541 ) ) ;
#33780=CARTESIAN_POINT ( 'NONE',  ( 763.2262854647970016, -392.6346026584193396, -309.2812353651462445 ) ) ;
#33785=CARTESIAN_POINT ( 'NONE',  ( 763.2262854647970016, -32.63460265842044095, -309.2812353651462445 ) ) ;
#33786=CARTESIAN_POINT ( 'NONE',  ( 771.1735550268778070, -249.1800572038742416, -316.3353852180827630 ) ) ;
#33787=DIRECTION ( 'NONE',  ( -0.000000000000000000, -1.110223024625155554E-15, -1.000000000000000000 ) ) ;
#33790=CARTESIAN_POINT ( 'NONE',  ( 775.9200461376533440, -23.80559628986938847, -315.3028492785443291 ) ) ;
#33796=CARTESIAN_POINT ( 'NONE',  ( 754.8983024940795303, -330.8965053807774552, -336.9254006560228163 ) ) ;
#33799=CARTESIAN_POINT ( 'NONE',  ( 756.1443688327750579, -381.6237781080500326, -314.3581564841659315 ) ) ;
#33805=CARTESIAN_POINT ( 'NONE',  ( 796.7737145352015204, -212.6346026584198796, -370.7187646348536987 ) ) ;
#33808=CARTESIAN_POINT ( 'NONE',  ( 756.3353852180820240, -173.9073299311472454, -331.1735550268787733 ) ) ;
#33811=CARTESIAN_POINT ( 'NONE',  ( 756.5762568750052424, -339.1800572038740142, -348.7366044899774238 ) ) ;
#33812=CARTESIAN_POINT ( 'NONE',  ( 802.9823548866075953, -457.0999726633339151, -330.0799878456151077 ) ) ;
#33819=CARTESIAN_POINT ( 'NONE',  ( 755.3028492785439312, -423.2817908451521589, -335.9200461376539693 ) ) ;
#33823=CARTESIAN_POINT ( 'NONE',  ( 745.1792804349281596, -230.1908817542436338, -343.7566961878542884 ) ) ;
#33825=CARTESIAN_POINT ( 'NONE',  ( 799.9999999999993179, 205.0000000000000568, -360.0000000000000000 ) ) ;
#33826=CARTESIAN_POINT ( 'NONE',  ( 765.0180583372156207, -192.9982390220562820, -360.0135310231089534 ) ) ;
#33827=CARTESIAN_POINT ( 'NONE',  ( 754.8983024940795303, -354.8965053807774552, -336.9254006560228163 ) ) ;
#33829=CARTESIAN_POINT ( 'NONE',  ( 807.2620300519052989, -240.0090635724253900, -318.0141637701419768 ) ) ;
#33832=CARTESIAN_POINT ( 'NONE',  ( 804.6971507214547046, -99.28179084515313946, -344.0799538623459739 ) ) ;
#33835=CARTESIAN_POINT ( 'NONE',  ( 782.5225473063383106, -262.2709662947832499, -375.2698199232970637 ) ) ;
#33838=CARTESIAN_POINT ( 'NONE',  ( 804.6798772138708955, -63.72551174932939233, -334.6312213355107019 ) ) ;
#33840=CARTESIAN_POINT ( 'NONE',  ( 808.7758568127978833, -172.1692326535052757, -320.0363995740631822 ) ) ;
#33842=CARTESIAN_POINT ( 'NONE',  ( 763.2262854647970016, -392.6346026584193396, -309.2812353651462445 ) ) ;
#33846=CARTESIAN_POINT ( 'NONE',  ( 758.0580252608178853, -390.4527844766011526, -328.0187753319985404 ) ) ;
#33853=CARTESIAN_POINT ( 'NONE',  ( 758.6633372737375112, -236.5328690171414792, -326.9102291470432533 ) ) ;
#33855=CARTESIAN_POINT ( 'NONE',  ( 800.1688906516307043, -250.1692326535050199, -369.0717654672308186 ) ) ;
#33860=CARTESIAN_POINT ( 'NONE',  ( 803.6646147819161570, -161.9073299311472454, -348.8264449731210561 ) ) ;
#33862=CARTESIAN_POINT ( 'NONE',  ( 796.7737145352015204, -92.63460265842026331, -370.7187646348536987 ) ) ;
#33863=CARTESIAN_POINT ( 'NONE',  ( 757.8323909638828582, -74.63460265842030594, -352.1044303154654358 ) ) ;
#33865=CARTESIAN_POINT ( 'NONE',  ( 802.9823548866075953, -1.099972663335260226, -330.0799878456151077 ) ) ;
#33867=CARTESIAN_POINT ( 'NONE',  ( 802.5472867521000353, -364.3726999360614514, -350.8726784830461156 ) ) ;
#33873=CARTESIAN_POINT ( 'NONE',  ( 776.9254006560222479, -308.1908817542434349, -314.8983024940802125 ) ) ;
#33874=CARTESIAN_POINT ( 'NONE',  ( 756.3353852180819104, -317.9073299311468190, -331.1735550268788302 ) ) ;
#33875=CARTESIAN_POINT ( 'NONE',  ( 771.3260364891663130, -139.6454272087893571, -306.0683387631859773 ) ) ;
#33876=VECTOR ( 'NONE', #33949, 1000.000000000000000 ) ;
#33880=CARTESIAN_POINT ( 'NONE',  ( 744.6391490659812007, -110.7363362996985501, -338.7502325331110455 ) ) ;
#33887=CARTESIAN_POINT ( 'NONE',  ( 777.4774526936600978, -178.2709662947835909, -304.7301800767028226 ) ) ;
#33890=CARTESIAN_POINT ( 'NONE',  ( 813.1304606946830518, -305.9073299311467622, -352.3570229623690580 ) ) ;
#33891=CARTESIAN_POINT ( 'NONE',  ( 814.9108240113580450, -448.2709662947827951, -337.5031285880265273 ) ) ;
#33895=CARTESIAN_POINT ( 'NONE',  ( 808.7758568127978833, -340.1692326535047641, -320.0363995740631822 ) ) ;
#33896=CARTESIAN_POINT ( 'NONE',  ( 751.9810565676468741, -98.08914811296568814, -360.9747183278973921 ) ) ;
#33898=CARTESIAN_POINT ( 'NONE',  ( 777.5031285880264704, -382.8164208402374697, -374.9108240113588408 ) ) ;
#33903=CARTESIAN_POINT ( 'NONE',  ( 813.9316612368132837, -103.4419599262327836, -348.6739635108323228 ) ) ;
#33908=CARTESIAN_POINT ( 'NONE',  ( 802.7791456095903868, -4.714687198960358039, -329.0155153010375102 ) ) ;
#33910=CARTESIAN_POINT ( 'NONE',  ( 793.4146539503750546, -433.9874144716862361, -307.6481478633938877 ) ) ;
#33914=CARTESIAN_POINT ( 'NONE',  ( 815.3608509340175488, -386.7363362996977116, -341.2497674668889545 ) ) ;
#33915=CARTESIAN_POINT ( 'NONE',  ( 788.8264449731200330, -237.1800572038742985, -363.6646147819171233 ) ) ;
#33919=CARTESIAN_POINT ( 'NONE',  ( 763.8424801807145741, -210.0090635724255321, -320.5453621957614700 ) ) ;
#33920=CARTESIAN_POINT ( 'NONE',  ( 797.6776695296629214, -211.5436935675107861, -357.6776695296636603 ) ) ;
#33921=CARTESIAN_POINT ( 'NONE',  ( 788.8264449731201466, -429.1800572038737300, -363.6646147819170665 ) ) ;
#33924=CARTESIAN_POINT ( 'NONE',  ( 764.8639956371174549, -104.0891481129656881, -319.7806653035542013 ) ) ;
#33933=CARTESIAN_POINT ( 'NONE',  ( 778.7629533639073998, -440.7363362996975980, -375.0009284576466371 ) ) ;
#33934=CARTESIAN_POINT ( 'NONE',  ( 749.2812353651451076, -30.45278447660226817, -323.2262854647983090 ) ) ;
#33936=CARTESIAN_POINT ( 'NONE',  ( 758.0580252608178853, -438.4527844766009821, -328.0187753319985404 ) ) ;
#33937=CARTESIAN_POINT ( 'NONE',  ( 756.3353852180820240, -53.90732993114765037, -331.1735550268787733 ) ) ;
#33939=DIRECTION ( 'NONE',  ( -1.000000000000000000, -0.000000000000000000, -0.000000000000000000 ) ) ;
#33940=CARTESIAN_POINT ( 'NONE',  ( 769.0155153010367712, -298.3726999360616787, -362.7791456095907279 ) ) ;
#33941=CARTESIAN_POINT ( 'NONE',  ( 763.2262854647970016, -176.6346026584199933, -309.2812353651462445 ) ) ;
#33947=CARTESIAN_POINT ( 'NONE',  ( 808.7758568127978833, -220.1692326535051052, -320.0363995740631822 ) ) ;
#33949=DIRECTION ( 'NONE',  ( -1.000000000000000000, -0.000000000000000000, -0.000000000000000000 ) ) ;
#33952=CARTESIAN_POINT ( 'NONE',  ( 788.8264449731200330, -357.1800572038739006, -363.6646147819171233 ) ) ;
#33954=CARTESIAN_POINT ( 'NONE',  ( 747.6481478633932056, -85.09997266333499510, -353.4146539503763620 ) ) ;
#33955=CARTESIAN_POINT ( 'NONE',  ( 796.7845633553578182, -153.6237781080508000, -358.5707757039688204 ) ) ;
#33958=CARTESIAN_POINT ( 'NONE',  ( 765.0180583372156207, -48.99823902205675807, -360.0135310231089534 ) ) ;
#33959=CARTESIAN_POINT ( 'NONE',  ( 757.2208543904082489, -160.7146871989598651, -350.9844846989624330 ) ) ;
#33961=EDGE_CURVE ( 'NONE', #40052, #3816, #34477, .T. ) ;
#33963=CARTESIAN_POINT ( 'NONE',  ( 746.0683387631852383, 4.558040073766884248, -331.3260364891676204 ) ) ;
#33968=CARTESIAN_POINT ( 'NONE',  ( 745.7194118038753459, -277.6454272087889308, -348.7631598425976449 ) ) ;
#33976=CARTESIAN_POINT ( 'NONE',  ( 754.7162404726377645, -110.7363362996985501, -339.4709603349214717 ) ) ;
#33977=CARTESIAN_POINT ( 'NONE',  ( 758.0580252608178853, -126.4527844766019626, -328.0187753319985404 ) ) ;
#33978=CARTESIAN_POINT ( 'NONE',  ( 781.8018195045267476, -310.2709662947832499, -365.1927285166407273 ) ) ;
#33980=CARTESIAN_POINT ( 'NONE',  ( 756.3353852180819104, -437.9073299311463074, -331.1735550268788302 ) ) ;
#33986=CARTESIAN_POINT ( 'NONE',  ( 762.1177392798416577, -330.5545181178796952, -309.8865473780659272 ) ) ;
#33988=CARTESIAN_POINT ( 'NONE',  ( 795.1360043628807261, -308.0891481129650629, -360.2193346964456282 ) ) ;
#33991=CARTESIAN_POINT ( 'NONE',  ( 769.0155153010367712, -202.3726999360618777, -362.7791456095907279 ) ) ;
#33994=CARTESIAN_POINT ( 'NONE',  ( 782.4968714119720516, -370.8164208402375834, -305.0891759886411023 ) ) ;
#33999=CARTESIAN_POINT ( 'NONE',  ( 792.2312462859673587, -35.90732993114770011, -307.2067596250082602 ) ) ;
#34000=CARTESIAN_POINT ( 'NONE',  ( 803.6646147819161570, -257.9073299311469896, -348.8264449731210561 ) ) ;
#34004=CARTESIAN_POINT ( 'NONE',  ( 756.1348686366196716, -41.26014174441479554, -347.5531968255698416 ) ) ;
#34008=EDGE_CURVE ( 'NONE', #24267, #14504, #11613, .T. ) ;
#34013=CARTESIAN_POINT ( 'NONE',  ( 756.7813123517142913, -379.9874144716865203, -329.9779781133712504 ) ) ;
#34016=CARTESIAN_POINT ( 'NONE',  ( 751.2241431872005251, -376.1692326535046504, -359.9636004259367610 ) ) ;
#34022=CARTESIAN_POINT ( 'NONE',  ( 808.3070685750230950, -210.9982390220561967, -361.1904061080339261 ) ) ;
#34025=CARTESIAN_POINT ( 'NONE',  ( 765.0180583372156207, -216.9982390220562252, -360.0135310231089534 ) ) ;
#34027=CARTESIAN_POINT ( 'NONE',  ( 754.8072714833581358, -340.8164208402376971, -338.1981804954720587 ) ) ;
#34028=CARTESIAN_POINT ( 'NONE',  ( 776.9254006560222479, -452.1908817542428665, -314.8983024940802125 ) ) ;
#34035=CARTESIAN_POINT ( 'NONE',  ( 803.4237431249931660, 8.819942796124882634, -331.2633955100225194 ) ) ;
#34039=CARTESIAN_POINT ( 'NONE',  ( 750.9282345327678740, -232.9181544815163249, -319.8311093483690115 ) ) ;
#34043=CARTESIAN_POINT ( 'NONE',  ( 788.7366044899766848, -179.9073299311472454, -316.5762568750059813 ) ) ;
#34044=CARTESIAN_POINT ( 'NONE',  ( 798.7617431975189675, -363.6237781080502032, -323.0428371773161871 ) ) ;
#34045=CARTESIAN_POINT ( 'NONE',  ( 746.4236121716829757, -231.8272453906072315, -328.8385539511384650 ) ) ;
#34048=CARTESIAN_POINT ( 'NONE',  ( 757.4527132478984868, -88.37269993606226137, -329.1273215169538844 ) ) ;
#34050=CARTESIAN_POINT ( 'NONE',  ( 787.4999999999992042, -462.9681489794447202, -270.0000000000000568 ) ) ;
#34051=CARTESIAN_POINT ( 'NONE',  ( 794.1144889064781864, -418.1692326535044799, -360.9840315886528401 ) ) ;
#34052=CARTESIAN_POINT ( 'NONE',  ( 763.0537975583476964, -264.4527844766016074, -371.0346526505628617 ) ) ;
#34055=CARTESIAN_POINT ( 'NONE',  ( 759.9864689768902508, -50.08914811296584446, -354.9819416627836404 ) ) ;
#34057=CARTESIAN_POINT ( 'NONE',  ( 786.2056067578752163, -155.8055962898689586, -374.4686193811670023 ) ) ;
#34059=CARTESIAN_POINT ( 'NONE',  ( 782.5225473063381969, -406.2709662947829088, -375.2698199232970637 ) ) ;
#34063=CARTESIAN_POINT ( 'NONE',  ( 771.1735550268778070, -417.1800572038736163, -316.3353852180827630 ) ) ;
#34065=EDGE_CURVE ( 'NONE', #41099, #21104, #4717, .T. ) ;
#34069=CARTESIAN_POINT ( 'NONE',  ( 769.1273215169530886, -238.7146871989596661, -317.4527132478988847 ) ) ;
#34072=CARTESIAN_POINT ( 'NONE',  ( 795.6651683502461765, -250.7146871989595809, -371.3240766477733814 ) ) ;
#34075=ORIENTED_EDGE ( 'NONE', *, *, #7988, .F. ) ;
#34076=CARTESIAN_POINT ( 'NONE',  ( 778.2165204200184689, -166.8164208402382087, -364.9363028652563230 ) ) ;
#34078=CARTESIAN_POINT ( 'NONE',  ( 745.0891759886404770, -124.2709662947837899, -342.4968714119734159 ) ) ;
#34079=CARTESIAN_POINT ( 'NONE',  ( 804.4286716492782716, -65.36187538569306810, -345.3141322388244703 ) ) ;
#34081=CARTESIAN_POINT ( 'NONE',  ( 790.9844846989617508, -46.37269993606239638, -317.2208543904092721 ) ) ;
#34082=CARTESIAN_POINT ( 'NONE',  ( 763.0428371773158460, -371.4636090269705164, -358.7617431975195359 ) ) ;
#34088=CARTESIAN_POINT ( 'NONE',  ( 787.5531968255692163, -333.8272453906070041, -316.1348686366205811 ) ) ;
#34089=CARTESIAN_POINT ( 'NONE',  ( 797.6776695296629214, -331.5436935675104451, -357.6776695296636603 ) ) ;
#34091=CARTESIAN_POINT ( 'NONE',  ( 815.3608509340175488, -146.7363362996984506, -341.2497674668889545 ) ) ;
#34095=CARTESIAN_POINT ( 'NONE',  ( 760.0363995740630116, -106.9181544815167371, -368.7758568127991907 ) ) ;
#34102=CARTESIAN_POINT ( 'NONE',  ( 747.2067596250078623, -171.1800572038745543, -352.2312462859687230 ) ) ;
#34105=CARTESIAN_POINT ( 'NONE',  ( 792.3570229623688874, -309.1800572038740711, -373.1304606946836202 ) ) ;
#34109=ORIENTED_EDGE ( 'NONE', *, *, #27246, .T. ) ;
#34111=CARTESIAN_POINT ( 'NONE',  ( 808.7758568127978833, -364.1692326535046504, -320.0363995740631822 ) ) ;
#34112=CARTESIAN_POINT ( 'NONE',  ( 814.2001403089898304, -137.3618753856928265, -347.4397851343538264 ) ) ;
#34114=CARTESIAN_POINT ( 'NONE',  ( 800.9747183278959710, -396.9982390220556567, -311.9810565676471583 ) ) ;
#34118=CIRCLE ( 'NONE', #20866, 10.00000000000000888 ) ;
#34119=CARTESIAN_POINT ( 'NONE',  ( 759.8311093483677041, -166.1692326535053041, -310.9282345327691814 ) ) ;
#34124=CARTESIAN_POINT ( 'NONE',  ( 775.9200461376533440, 0.1944037101305369775, -315.3028492785443291 ) ) ;
#34126=CARTESIAN_POINT ( 'NONE',  ( 801.1904061080336987, 3.910851887033985896, -368.3070685750235498 ) ) ;
#34127=CARTESIAN_POINT ( 'NONE',  ( 799.9999999999993179, 166.4563064324884465, -360.0000000000000000 ) ) ;
#34129=ORIENTED_EDGE ( 'NONE', *, *, #24044, .F. ) ;
#34130=CARTESIAN_POINT ( 'NONE',  ( 764.1737431748507561, -418.3726999360612808, -371.6461892240376415 ) ) ;
#34133=CARTESIAN_POINT ( 'NONE',  ( 755.5913626894240451, -229.6454272087890729, -346.6156483768012890 ) ) ;
#34134=CARTESIAN_POINT ( 'NONE',  ( 771.2633955100217236, -215.9073299311471317, -363.4237431249939618 ) ) ;
#34135=CARTESIAN_POINT ( 'NONE',  ( 762.1405469898973024, -433.5436935675100472, -357.8594530101016176 ) ) ;
#34145=CARTESIAN_POINT ( 'NONE',  ( 812.3518521366052028, -433.0999726633339151, -326.5853460496235243 ) ) ;
#34147=CARTESIAN_POINT ( 'NONE',  ( 796.9462024416508257, -60.45278447660216159, -308.9653473494370246 ) ) ;
#34149=CARTESIAN_POINT ( 'NONE',  ( 762.1405469898971887, -433.5436935675099903, -357.8594530101015607 ) ) ;
#34150=CARTESIAN_POINT ( 'NONE',  ( 785.3687786644885591, -35.36187538569316047, -315.3201227861280813 ) ) ;
#34153=CARTESIAN_POINT ( 'NONE',  ( 779.4763451958990572, -296.7363362996979390, -365.0264073115438919 ) ) ;
#34154=CARTESIAN_POINT ( 'NONE',  ( 814.9108240113580450, -208.2709662947835341, -337.5031285880265273 ) ) ;
#34159=CARTESIAN_POINT ( 'NONE',  ( 766.5853460496234675, -229.9874144716869466, -372.3518521366060554 ) ) ;
#34162=CARTESIAN_POINT ( 'NONE',  ( 748.9653473494363425, -266.6346026584197375, -356.9462024416521331 ) ) ;
#34166=CARTESIAN_POINT ( 'NONE',  ( 765.0180583372156207, -336.9982390220558273, -360.0135310231089534 ) ) ;
#34168=CARTESIAN_POINT ( 'NONE',  ( 751.2241431872005251, -40.16923265350570915, -359.9636004259367610 ) ) ;
#34169=CARTESIAN_POINT ( 'NONE',  ( 773.3843516231979720, -157.4419599262326130, -364.4086373105754433 ) ) ;
#34174=CARTESIAN_POINT ( 'NONE',  ( 797.6776695296629214, -67.54369356751125508, -357.6776695296636603 ) ) ;
#34175=CARTESIAN_POINT ( 'NONE',  ( 763.2154366446407039, -165.6237781080507716, -321.4292242960311228 ) ) ;
#34177=CARTESIAN_POINT ( 'NONE',  ( 749.8865473780648472, 3.467130982857797417, -322.1177392798429082 ) ) ;
#34184=CARTESIAN_POINT ( 'NONE',  ( 812.3518521366052028, -289.0999726633343698, -326.5853460496235243 ) ) ;
#34192=CARTESIAN_POINT ( 'NONE',  ( 802.5472867521000353, -124.3726999360621619, -350.8726784830461156 ) ) ;
#34193=CARTESIAN_POINT ( 'NONE',  ( 794.9819416627830151, -108.9982390220565804, -319.9864689768909898 ) ) ;
#34194=CARTESIAN_POINT ( 'NONE',  ( 785.3687786644885591, -323.3618753856922581, -315.3201227861280813 ) ) ;
#34196=CARTESIAN_POINT ( 'NONE',  ( 758.0580252608178853, -438.4527844766009821, -328.0187753319985404 ) ) ;
#34200=LINE ( 'NONE', #9960, #4236 ) ;
#34204=CARTESIAN_POINT ( 'NONE',  ( 805.6418435158337843, -341.4636090269705733, -363.8556311672236916 ) ) ;
#34206=CARTESIAN_POINT ( 'NONE',  ( 755.3201227861273992, -315.7255117493286320, -345.3687786644892981 ) ) ;
#34207=CARTESIAN_POINT ( 'NONE',  ( 783.0745993439762742, -176.1908817542438328, -365.1016975059196739 ) ) ;
#34212=CARTESIAN_POINT ( 'NONE',  ( 772.4837098697145166, -383.3618753856920875, -374.5518280994205611 ) ) ;
#34217=CARTESIAN_POINT ( 'NONE',  ( 810.7187646348534145, -18.45278447660230725, -356.7737145352016341 ) ) ;
#34219=CARTESIAN_POINT ( 'NONE',  ( 804.6798772138708955, -255.7255117493287742, -334.6312213355107019 ) ) ;
#34223=CARTESIAN_POINT ( 'NONE',  ( 775.9200461376533440, -47.80559628986931386, -315.3028492785443291 ) ) ;
#34230=CARTESIAN_POINT ( 'NONE',  ( 758.0580252608178853, -54.45278447660219001, -328.0187753319985404 ) ) ;
#34232=CARTESIAN_POINT ( 'NONE',  ( 755.0488828828309806, -353.8055962898683333, -344.1219089521771934 ) ) ;
#34235=CARTESIAN_POINT ( 'NONE',  ( 776.2433038121456548, -372.8965053807773415, -374.8207195650711014 ) ) ;
#34237=ORIENTED_EDGE ( 'NONE', *, *, #6961, .F. ) ;
#34241=DIRECTION ( 'NONE',  ( 0.000000000000000000, 0.000000000000000000, 1.000000000000000000 ) ) ;
#34242=CARTESIAN_POINT ( 'NONE',  ( 810.7187646348534145, -210.4527844766016926, -356.7737145352016341 ) ) ;
#34247=CARTESIAN_POINT ( 'NONE',  ( 768.0187753319979720, -200.6346026584199365, -318.0580252608186242 ) ) ;
#34250=CARTESIAN_POINT ( 'NONE',  ( 758.0580252608178853, -318.4527844766014368, -328.0187753319985404 ) ) ;
#34251=CARTESIAN_POINT ( 'NONE',  ( 757.0176451133909268, -445.0999726633338582, -349.9200121543848354 ) ) ;
#34254=DIRECTION ( 'NONE',  ( -0.000000000000000000, 1.000000000000000000, -0.000000000000000000 ) ) ;
#34256=DIRECTION ( 'NONE',  ( 0.000000000000000000, -0.000000000000000000, -1.000000000000000000 ) ) ;
#34258=CARTESIAN_POINT ( 'NONE',  ( 805.1927285166397041, 7.183579159761247723, -341.8018195045277707 ) ) ;
#34261=CARTESIAN_POINT ( 'NONE',  ( 778.7629533639073998, -248.7363362996981380, -375.0009284576466371 ) ) ;
#34266=CARTESIAN_POINT ( 'NONE',  ( 805.1927285166397041, -232.8164208402379245, -341.8018195045277707 ) ) ;
#34268=CARTESIAN_POINT ( 'NONE',  ( 766.7756240680305382, -374.5328690171410813, -361.5560724626415663 ) ) ;
#34269=CARTESIAN_POINT ( 'NONE',  ( 747.6481478633932056, -253.0999726633345119, -353.4146539503763620 ) ) ;
#34272=CARTESIAN_POINT ( 'NONE',  ( 793.0897708529556667, -78.55451811788046257, -361.3366627262616362 ) ) ;
#34276=CARTESIAN_POINT ( 'NONE',  ( 803.2186876482843445, -415.9874144716862361, -350.0220218866286928 ) ) ;
#34277=CARTESIAN_POINT ( 'NONE',  ( 755.2512626584698410, -271.5436935675106156, -315.2512626584710915 ) ) ;
#34280=CARTESIAN_POINT ( 'NONE',  ( 788.7366044899766848, -35.90732993114770011, -316.5762568750059813 ) ) ;
#34282=CARTESIAN_POINT ( 'NONE',  ( 759.8311093483677041, -166.1692326535053041, -310.9282345327691814 ) ) ;
#34284=CARTESIAN_POINT ( 'NONE',  ( 754.9967657858570647, -409.5436935675101040, -365.0032342141425374 ) ) ;
#34292=CARTESIAN_POINT ( 'NONE',  ( 797.8594530101008786, -421.5436935675101040, -322.1405469898980982 ) ) ;
#34299=CARTESIAN_POINT ( 'NONE',  ( 796.7845633553578182, -273.6237781080504305, -358.5707757039688204 ) ) ;
#34301=AXIS2_PLACEMENT_3D ( 'NONE', #9241, #5771, #39199 ) ;
#34302=CARTESIAN_POINT ( 'NONE',  ( 807.5423716828161105, -249.0783235625959549, -362.2119215644372048 ) ) ;
#34307=AXIS2_PLACEMENT_3D ( 'NONE', #1732, #26906, #33622 ) ;
#34310=CARTESIAN_POINT ( 'NONE',  ( 772.3691319403857278, -23.26014174441484883, -315.8894580844506663 ) ) ;
#34311=CARTESIAN_POINT ( 'NONE',  ( 804.9363028652555840, -160.2709662947836762, -338.2165204200192079 ) ) ;
#34314=CARTESIAN_POINT ( 'NONE',  ( 755.2512626584698410, -103.5436935675111272, -315.2512626584710915 ) ) ;
#34315=CARTESIAN_POINT ( 'NONE',  ( 801.9419747391806368, -114.4527844766020053, -351.9812246680014027 ) ) ;
#34317=CARTESIAN_POINT ( 'NONE',  ( 760.7433823573367135, -36.00906357242605793, -355.9930595647440441 ) ) ;
#34318=CARTESIAN_POINT ( 'NONE',  ( 754.7162404726377645, -350.7363362996978253, -339.4709603349214717 ) ) ;
#34325=CARTESIAN_POINT ( 'NONE',  ( 780.5236548040995785, -356.7363362996978253, -314.9735926884559944 ) ) ;
#34326=CARTESIAN_POINT ( 'NONE',  ( 774.6858677611749044, -345.7255117493285184, -315.5713283507209894 ) ) ;
#34327=CARTESIAN_POINT ( 'NONE',  ( 795.8262568251477660, -118.3726999360621619, -308.3538107759623585 ) ) ;
#34334=CARTESIAN_POINT ( 'NONE',  ( 790.8726784830453198, -274.7146871989594388, -362.5472867521010585 ) ) ;
#34335=CARTESIAN_POINT ( 'NONE',  ( 813.5763878283155464, -147.8272453906075157, -351.1614460488615350 ) ) ;
#34342=CARTESIAN_POINT ( 'NONE',  ( 808.3070685750232087, -186.9982390220563104, -361.1904061080339829 ) ) ;
#34346=CARTESIAN_POINT ( 'NONE',  ( 805.0032342141412300, -301.5436935675105588, -314.9967657858571783 ) ) ;
#34353=CARTESIAN_POINT ( 'NONE',  ( 813.9316612368132837, -391.4419599262317888, -348.6739635108323228 ) ) ;
#34354=CARTESIAN_POINT ( 'NONE',  ( 745.0891759886404770, -124.2709662947837899, -342.4968714119734159 ) ) ;
#34356=CARTESIAN_POINT ( 'NONE',  ( 813.1304606946830518, -377.9073299311466485, -352.3570229623690580 ) ) ;
#34361=CARTESIAN_POINT ( 'NONE',  ( 744.8212110874229666, -138.8965053807781374, -336.2046728542121627 ) ) ;
#34365=VERTEX_POINT ( 'NONE', #26414 ) ;
#34367=CARTESIAN_POINT ( 'NONE',  ( 755.0488828828309806, -17.80559628986940979, -344.1219089521771934 ) ) ;
#34369=CARTESIAN_POINT ( 'NONE',  ( 815.2698199232961542, 7.183579159761247723, -342.5225473063383106 ) ) ;
#34372=CARTESIAN_POINT ( 'NONE',  ( 804.6798772138708955, -183.7255117493290015, -334.6312213355107019 ) ) ;
#34373=CARTESIAN_POINT ( 'NONE',  ( 745.1792804349281596, -398.1908817542431507, -343.7566961878542884 ) ) ;
#34375=CARTESIAN_POINT ( 'NONE',  ( 762.3223304703356007, -247.5436935675106724, -322.3223304703362828 ) ) ;
#34379=CARTESIAN_POINT ( 'NONE',  ( 793.0897708529556667, -270.5545181178798657, -361.3366627262616362 ) ) ;
#34380=CARTESIAN_POINT ( 'NONE',  ( 774.6312213355099630, -215.3618753856925423, -364.6798772138717482 ) ) ;
#34381=CARTESIAN_POINT ( 'NONE',  ( 785.3141322388236176, -429.7255117493282910, -364.4286716492789537 ) ) ;
#34383=ORIENTED_EDGE ( 'NONE', *, *, #9705, .T. ) ;
#34386=CARTESIAN_POINT ( 'NONE',  ( 768.9521613784389729, -9.827245390607961539, -373.2346286133773106 ) ) ;
#34392=CARTESIAN_POINT ( 'NONE',  ( 784.1219089521767955, -21.28179084515337749, -315.0488828828318333 ) ) ;
#34393=CARTESIAN_POINT ( 'NONE',  ( 777.4774526936600978, -58.27096629478398881, -304.7301800767028226 ) ) ;
#34396=CARTESIAN_POINT ( 'NONE',  ( 804.6798772138708955, -423.7255117493281205, -334.6312213355107019 ) ) ;
#34397=CARTESIAN_POINT ( 'NONE',  ( 765.0180583372156207, -48.99823902205675807, -360.0135310231089534 ) ) ;
#34400=CARTESIAN_POINT ( 'NONE',  ( 763.0537975583475827, -216.4527844766016926, -371.0346526505627480 ) ) ;
#34407=CARTESIAN_POINT ( 'NONE',  ( 791.1614460488616487, -275.2601417444140566, -373.5763878283158874 ) ) ;
#34409=CARTESIAN_POINT ( 'NONE',  ( 814.9108240113580450, -280.2709662947833067, -337.5031285880265273 ) ) ;
#34413=CARTESIAN_POINT ( 'NONE',  ( 798.0661480581538854, -26.53286901714210799, -309.5768839229118043 ) ) ;
#34414=CARTESIAN_POINT ( 'NONE',  ( 759.9864689768902508, -338.0891481129649492, -354.9819416627836404 ) ) ;
#34417=CARTESIAN_POINT ( 'NONE',  ( 813.9316612368132837, -55.44195992623293989, -348.6739635108323228 ) ) ;
#34418=CARTESIAN_POINT ( 'NONE',  ( 779.4709603349208464, -168.3510508353234911, -314.7162404726379918 ) ) ;
#34421=ORIENTED_EDGE ( 'NONE', *, *, #6961, .T. ) ;
#34422=CARTESIAN_POINT ( 'NONE',  ( 754.8072714833581358, -76.81642084023845030, -338.1981804954720587 ) ) ;
#34423=CARTESIAN_POINT ( 'NONE',  ( 805.1016975059191054, -150.8965053807781089, -343.0745993439771837 ) ) ;
#34426=CARTESIAN_POINT ( 'NONE',  ( 781.2497674668890113, 11.64894916467595642, -375.3608509340180603 ) ) ;
#34430=ORIENTED_EDGE ( 'NONE', *, *, #4683, .F. ) ;
#34432=CARTESIAN_POINT ( 'NONE',  ( 812.3518521366052028, -313.0999726633342561, -326.5853460496235243 ) ) ;
#34434=CIRCLE ( 'NONE', #7183, 10.00000000000000888 ) ;
#34438=CARTESIAN_POINT ( 'NONE',  ( 804.6971507214547046, -147.2817908451529547, -344.0799538623459739 ) ) ;
#34440=CARTESIAN_POINT ( 'NONE',  ( 764.8639956371174549, -128.0891481129655176, -319.7806653035542013 ) ) ;
#34441=CARTESIAN_POINT ( 'NONE',  ( 785.3687786644885591, -299.3618753856923149, -315.3201227861280813 ) ) ;
#34442=EDGE_LOOP ( 'NONE', ( #21993, #44675, #32499, #19951 ) ) ;
#34443=CARTESIAN_POINT ( 'NONE',  ( 802.1676090361156639, -422.6346026584192259, -327.8955696845344505 ) ) ;
#34452=CARTESIAN_POINT ( 'NONE',  ( 814.4686193811664907, -339.2817908451524431, -346.2056067578752732 ) ) ;
#34456=CARTESIAN_POINT ( 'NONE',  ( 797.6776695296629214, -331.5436935675104451, -357.6776695296636603 ) ) ;
#34458=CARTESIAN_POINT ( 'NONE',  ( 790.0220218866281812, -175.0999726633346825, -363.2186876482849129 ) ) ;
#34461=CARTESIAN_POINT ( 'NONE',  ( 814.5518280994195948, -375.7255117493284047, -332.4837098697145166 ) ) ;
#34467=CARTESIAN_POINT ( 'NONE',  ( 805.0032342141412300, -13.54369356751140785, -314.9967657858571783 ) ) ;
#34469=CARTESIAN_POINT ( 'NONE',  ( 759.9864689768902508, -242.0891481129652618, -354.9819416627836404 ) ) ;
#34473=CARTESIAN_POINT ( 'NONE',  ( 744.6391490659812007, -38.73633629969877035, -338.7502325331110455 ) ) ;
#34474=CARTESIAN_POINT ( 'NONE',  ( 772.3691319403857278, -47.26014174441477422, -315.8894580844506663 ) ) ;
#34477=CIRCLE ( 'NONE', #19702, 10.00000000000000888 ) ;
#34481=ORIENTED_EDGE ( 'NONE', *, *, #44997, .F. ) ;
#34482=CARTESIAN_POINT ( 'NONE',  ( 756.3353852180819104, -77.90732993114757221, -331.1735550268788302 ) ) ;
#34483=CARTESIAN_POINT ( 'NONE',  ( 800.7704444035546203, -364.1692326535046504, -326.0291762391768771 ) ) ;
#34486=CARTESIAN_POINT ( 'NONE',  ( 746.0683387631852383, -355.4419599262319593, -331.3260364891676204 ) ) ;
#34491=CARTESIAN_POINT ( 'NONE',  ( 814.2001403089898304, -233.3618753856925423, -347.4397851343538264 ) ) ;
#34494=CARTESIAN_POINT ( 'NONE',  ( 759.7806653035535192, -222.9982390220561683, -324.8639956371181370 ) ) ;
#34497=CARTESIAN_POINT ( 'NONE',  ( 771.2633955100217236, -311.9073299311468759, -363.4237431249939618 ) ) ;
#34498=CARTESIAN_POINT ( 'NONE',  ( 797.6776695296629214, 4.456306432488530866, -357.6776695296636603 ) ) ;
#34505=CARTESIAN_POINT ( 'NONE',  ( 796.9571628226829034, -455.4636090269701754, -321.2382568024804641 ) ) ;
#34506=CARTESIAN_POINT ( 'NONE',  ( 766.1799889109151991, 20.32535068748918050, -313.3728091324376237 ) ) ;
#34509=CARTESIAN_POINT ( 'NONE',  ( 745.5313806188320314, -255.2817908451526705, -333.7943932421247268 ) ) ;
#34512=CARTESIAN_POINT ( 'NONE',  ( 754.8072714833581358, -220.8164208402379529, -338.1981804954720587 ) ) ;
#34513=CARTESIAN_POINT ( 'NONE',  ( 802.7791456095903868, -412.7146871989590409, -329.0155153010375102 ) ) ;
#34514=CARTESIAN_POINT ( 'NONE',  ( 811.3240766477731540, -244.3726999360617924, -355.6651683502462902 ) ) ;
#34517=CARTESIAN_POINT ( 'NONE',  ( 776.9254006560222479, -92.19088175424406018, -314.8983024940802125 ) ) ;
#34521=CARTESIAN_POINT ( 'NONE',  ( 760.5453621957607311, -429.0783235625953580, -323.8424801807151425 ) ) ;
#34522=CARTESIAN_POINT ( 'NONE',  ( 748.9653473494365699, -290.6346026584196238, -356.9462024416520762 ) ) ;
#34525=CARTESIAN_POINT ( 'NONE',  ( 768.0187753319979720, -80.63460265842029173, -318.0580252608186242 ) ) ;
#34527=CARTESIAN_POINT ( 'NONE',  ( 771.2368401574024119, -157.4419599262326130, -374.2805881961240857 ) ) ;
#34529=CARTESIAN_POINT ( 'NONE',  ( 763.2262854647970016, -416.6346026584192259, -309.2812353651462445 ) ) ;
#34533=CARTESIAN_POINT ( 'NONE',  ( 768.0187753319979720, -440.6346026584191122, -318.0580252608186242 ) ) ;
#34539=CARTESIAN_POINT ( 'NONE',  ( 805.1016975059191054, -246.8965053807777679, -343.0745993439771837 ) ) ;
#34541=CARTESIAN_POINT ( 'NONE',  ( 759.8311093483677041, -262.1692326535049347, -310.9282345327691814 ) ) ;
#34547=CARTESIAN_POINT ( 'NONE',  ( 756.7813123517142913, -43.98741447168752217, -329.9779781133712504 ) ) ;
#34548=CARTESIAN_POINT ( 'NONE',  ( 785.3141322388236176, -165.7255117493291152, -364.4286716492789537 ) ) ;
#34551=CARTESIAN_POINT ( 'NONE',  ( 808.3070685750230950, -114.9982390220565236, -361.1904061080339261 ) ) ;
#34552=CARTESIAN_POINT ( 'NONE',  ( 767.8955696845334842, -96.45278447660204790, -362.1676090361161755 ) ) ;
#34554=CARTESIAN_POINT ( 'NONE',  ( 766.0291762391763086, -58.91815448151690759, -360.7704444035551319 ) ) ;
#34555=CARTESIAN_POINT ( 'NONE',  ( 783.0745993439762742, -344.1908817542433212, -365.1016975059196739 ) ) ;
#34564=CARTESIAN_POINT ( 'NONE',  ( 755.8894580844503253, -375.8272453906069472, -332.3691319403863531 ) ) ;
#34565=CARTESIAN_POINT ( 'NONE',  ( 794.9819416627830151, -372.9982390220557704, -319.9864689768909898 ) ) ;
#34566=CARTESIAN_POINT ( 'NONE',  ( 776.2046728542105711, -140.1908817542438896, -304.8212110874238761 ) ) ;
#34570=CARTESIAN_POINT ( 'NONE',  ( 804.9511171171677688, -269.8055962898686175, -335.8780910478229202 ) ) ;
#34571=CARTESIAN_POINT ( 'NONE',  ( 776.2046728542105711, -140.1908817542438896, -304.8212110874238761 ) ) ;
#34576=CARTESIAN_POINT ( 'NONE',  ( 811.0346526505617248, -182.6346026584199649, -323.0537975583478101 ) ) ;
#34582=CARTESIAN_POINT ( 'NONE',  ( 755.2512626584698410, -319.5436935675104451, -315.2512626584710915 ) ) ;
#34589=CARTESIAN_POINT ( 'NONE',  ( 788.7631598425961101, -385.4419599262319593, -305.7194118038759143 ) ) ;
#34590=CARTESIAN_POINT ( 'NONE',  ( 751.9810565676468741, -122.0891481129656171, -360.9747183278973921 ) ) ;
#34592=CARTESIAN_POINT ( 'NONE',  ( 815.2698199232961542, -400.8164208402373561, -342.5225473063383106 ) ) ;
#34596=CARTESIAN_POINT ( 'NONE',  ( 778.7502325331095108, -168.3510508353234911, -304.6391490659818828 ) ) ;
#34604=CARTESIAN_POINT ( 'NONE',  ( 777.4774526936600978, -10.27096629478414691, -304.7301800767027657 ) ) ;
#34608=CARTESIAN_POINT ( 'NONE',  ( 762.1177392798416577, -402.5545181178795247, -309.8865473780659272 ) ) ;
#34611=CARTESIAN_POINT ( 'NONE',  ( 803.4237431249931660, -255.1800572038742700, -331.2633955100225194 ) ) ;
#34616=CARTESIAN_POINT ( 'NONE',  ( 798.5707757039680246, -245.4636090269709143, -356.7845633553585003 ) ) ;
#34617=CARTESIAN_POINT ( 'NONE',  ( 762.1405469898971887, -265.5436935675106156, -357.8594530101015607 ) ) ;
#34618=CARTESIAN_POINT ( 'NONE',  ( 795.1360043628808398, -428.0891481129645513, -360.2193346964456282 ) ) ;
#34619=CARTESIAN_POINT ( 'NONE',  ( 800.2193346964447755, -66.99823902205672255, -355.1360043628815788 ) ) ;
#34624=CARTESIAN_POINT ( 'NONE',  ( 793.5525998758768083, -55.09997266333508747, -372.6845335610516941 ) ) ;
#34630=CARTESIAN_POINT ( 'NONE',  ( 787.5531968255692163, 2.172754609392001601, -316.1348686366205811 ) ) ;
#34631=CARTESIAN_POINT ( 'NONE',  ( 800.9747183278959710, -84.99823902205663728, -311.9810565676471583 ) ) ;
#34633=CARTESIAN_POINT ( 'NONE',  ( 802.1676090361156639, -446.6346026584189985, -327.8955696845344505 ) ) ;
#34634=CARTESIAN_POINT ( 'NONE',  ( 792.1044303154646968, -36.45278447660224685, -317.8323909638837677 ) ) ;
#34636=CARTESIAN_POINT ( 'NONE',  ( 751.9810565676468741, -194.0891481129654039, -360.9747183278973921 ) ) ;
#34641=CARTESIAN_POINT ( 'NONE',  ( 783.7566961878529810, -264.8965053807776826, -305.1792804349288417 ) ) ;
#34644=CARTESIAN_POINT ( 'NONE',  ( 763.2262854647970016, -272.6346026584196807, -309.2812353651462445 ) ) ;
#34648=CARTESIAN_POINT ( 'NONE',  ( 778.1981804954714335, -370.2709662947831362, -314.8072714833589885 ) ) ;
#34650=CARTESIAN_POINT ( 'NONE',  ( 814.8230680027162407, -53.80559628986930676, -333.7305795820267917 ) ) ;
#34651=CARTESIAN_POINT ( 'NONE',  ( 779.4709603349208464, -144.3510508353235764, -314.7162404726379918 ) ) ;
#34656=CARTESIAN_POINT ( 'NONE',  ( 771.2633955100217236, -47.90732993114767169, -363.4237431249939618 ) ) ;
#34657=CARTESIAN_POINT ( 'NONE',  ( 780.5290396650775619, -180.3510508353234343, -365.2837595273619513 ) ) ;
#34659=CARTESIAN_POINT ( 'NONE',  ( 798.0661480581538854, -2.532869017142183932, -309.5768839229118043 ) ) ;
#34662=ORIENTED_EDGE ( 'NONE', *, *, #22985, .T. ) ;
#34664=CARTESIAN_POINT ( 'NONE',  ( 802.2119215644370342, -294.0090635724253048, -367.5423716828165084 ) ) ;
#34669=CARTESIAN_POINT ( 'NONE',  ( 784.1219089521767955, -165.2817908451529547, -315.0488828828318333 ) ) ;
#34670=CARTESIAN_POINT ( 'NONE',  ( 791.9812246680005501, -164.6346026584200217, -361.9419747391813189 ) ) ;
#34671=CARTESIAN_POINT ( 'NONE',  ( 756.3353852180820240, -317.9073299311467622, -331.1735550268787733 ) ) ;
#34679=CARTESIAN_POINT ( 'NONE',  ( 805.6418435158337843, -365.4636090269705164, -363.8556311672236916 ) ) ;
#34682=CARTESIAN_POINT ( 'NONE',  ( 756.3353852180819104, -341.9073299311465917, -331.1735550268788302 ) ) ;
#34684=CARTESIAN_POINT ( 'NONE',  ( 786.5483106153019435, -199.6454272087891582, -364.1601925771022366 ) ) ;
#34687=CARTESIAN_POINT ( 'NONE',  ( 745.7998596910086917, -413.3618753856920307, -332.5602148656461168 ) ) ;
#34692=CARTESIAN_POINT ( 'NONE',  ( 808.3070685750230950, -42.99823902205675807, -361.1904061080339261 ) ) ;
#34693=CARTESIAN_POINT ( 'NONE',  ( 767.8955696845333705, -240.4527844766015221, -362.1676090361162323 ) ) ;
#34697=CARTESIAN_POINT ( 'NONE',  ( 813.5763878283155464, -27.82724539060790292, -351.1614460488615350 ) ) ;
#34698=CARTESIAN_POINT ( 'NONE',  ( 776.9566956441375396, -60.89650538077837894, -364.8461984189686405 ) ) ;
#34705=CARTESIAN_POINT ( 'NONE',  ( 797.6776695296629214, -67.54369356751125508, -357.6776695296636603 ) ) ;
#34706=CARTESIAN_POINT ( 'NONE',  ( 779.4709603349208464, -360.3510508353228374, -314.7162404726379918 ) ) ;
#34709=CARTESIAN_POINT ( 'NONE',  ( 798.0661480581538854, -362.5328690171410813, -309.5768839229118043 ) ) ;
#34714=CARTESIAN_POINT ( 'NONE',  ( 777.4774526936600978, -226.2709662947834204, -304.7301800767027657 ) ) ;
#34717=CARTESIAN_POINT ( 'NONE',  ( 795.1360043628808398, -212.0891481129653187, -360.2193346964456282 ) ) ;
#34719=CARTESIAN_POINT ( 'NONE',  ( 802.1676090361156639, -374.6346026584192828, -327.8955696845344505 ) ) ;
#34720=CARTESIAN_POINT ( 'NONE',  ( 758.0580252608178853, -30.45278447660226817, -328.0187753319985404 ) ) ;
#34725=CARTESIAN_POINT ( 'NONE',  ( 795.1360043628807261, 3.910851887033985896, -360.2193346964456282 ) ) ;
#34729=CARTESIAN_POINT ( 'NONE',  ( 754.3581564841646241, -281.4636090269706870, -316.1443688327762516 ) ) ;
#34732=CARTESIAN_POINT ( 'NONE',  ( 797.8594530101008786, -229.5436935675106440, -322.1405469898980982 ) ) ;
#34733=CARTESIAN_POINT ( 'NONE',  ( 755.8398074228967971, -403.4419599262317888, -333.4516893846970333 ) ) ;
#34735=CARTESIAN_POINT ( 'NONE',  ( 768.0187753319979720, 15.36539734157940629, -318.0580252608186242 ) ) ;
#34736=CARTESIAN_POINT ( 'NONE',  ( 796.9571628226829034, -95.46360902697132644, -321.2382568024804641 ) ) ;
#34738=CARTESIAN_POINT ( 'NONE',  ( 805.9055244015594326, -3.623778108051270319, -315.8990559732753240 ) ) ;
#34739=CARTESIAN_POINT ( 'NONE',  ( 811.0346526505617248, -278.6346026584196807, -323.0537975583478101 ) ) ;
#34742=CARTESIAN_POINT ( 'NONE',  ( 755.3201227861273992, -75.72551174932937101, -345.3687786644892981 ) ) ;
#34744=CARTESIAN_POINT ( 'NONE',  ( 758.0141637701419768, -183.0783235625961538, -367.2620300519063790 ) ) ;
#34746=CARTESIAN_POINT ( 'NONE',  ( 792.2312462859673587, -419.9073299311465348, -307.2067596250082602 ) ) ;
#34750=CARTESIAN_POINT ( 'NONE',  ( 757.8323909638827445, -410.6346026584191122, -352.1044303154654358 ) ) ;
#34756=CARTESIAN_POINT ( 'NONE',  ( 787.6308680596127942, -251.2601417444141134, -364.1105419155492768 ) ) ;
#34758=CARTESIAN_POINT ( 'NONE',  ( 801.9858362298568863, -243.0783235625959833, -312.7379699480935642 ) ) ;
#34763=CARTESIAN_POINT ( 'NONE',  ( 754.9735926884551418, -42.35105083532388193, -340.5236548041000333 ) ) ;
#34764=CARTESIAN_POINT ( 'NONE',  ( 804.6798772138708955, -159.7255117493291436, -334.6312213355107019 ) ) ;
#34765=CARTESIAN_POINT ( 'NONE',  ( 792.1044303154645831, -204.4527844766016926, -317.8323909638837677 ) ) ;
#34767=CARTESIAN_POINT ( 'NONE',  ( 777.4774526936600978, -130.2709662947837899, -304.7301800767027657 ) ) ;
#34768=CARTESIAN_POINT ( 'NONE',  ( 757.8323909638828582, -122.6346026584201496, -352.1044303154654358 ) ) ;
#34770=CARTESIAN_POINT ( 'NONE',  ( 793.9708237608222134, -46.91815448151694312, -319.2295555964448681 ) ) ;
#34771=CARTESIAN_POINT ( 'NONE',  ( 772.4468031744293057, -393.8272453906067199, -363.8651313633793620 ) ) ;
#34779=CARTESIAN_POINT ( 'NONE',  ( 755.3028492785439312, -351.2817908451523294, -335.9200461376539693 ) ) ;
#34780=CARTESIAN_POINT ( 'NONE',  ( 800.0135310231082713, -374.0891481129647786, -325.0180583372163028 ) ) ;
#34781=CARTESIAN_POINT ( 'NONE',  ( 757.7880784355613741, -138.0090635724257311, -312.4576283171834916 ) ) ;
#34783=CARTESIAN_POINT ( 'NONE',  ( 759.9999999999992042, -462.9681489794448339, -309.9999999999998863 ) ) ;
#34785=CARTESIAN_POINT ( 'NONE',  ( 763.2154366446407039, -285.6237781080502600, -321.4292242960311228 ) ) ;
#34786=CARTESIAN_POINT ( 'NONE',  ( 768.0187753319979720, -440.6346026584191122, -318.0580252608186242 ) ) ;
#34787=CARTESIAN_POINT ( 'NONE',  ( 805.6418435158337843, -149.4636090269711417, -363.8556311672236916 ) ) ;
#34792=CARTESIAN_POINT ( 'NONE',  ( 805.0032342141413437, -181.5436935675108430, -314.9967657858572352 ) ) ;
#34794=( BOUNDED_CURVE ( )  B_SPLINE_CURVE ( 3, ( #9733, #23799, #6500, #20352 ),
 .UNSPECIFIED., .F., .T. ) 
 B_SPLINE_CURVE_WITH_KNOTS ( ( 4, 4 ),
 ( 4.691336726374857768, 4.712707788662813257 ),
 .UNSPECIFIED. ) 
 CURVE ( )  GEOMETRIC_REPRESENTATION_ITEM ( )  RATIONAL_B_SPLINE_CURVE ( ( 1.000000000000000000, 0.9999619401702002364, 0.9999619401702002364, 1.000000000000000000 ) ) 
 REPRESENTATION_ITEM ( '' )  );
#34796=CARTESIAN_POINT ( 'NONE',  ( 763.0537975583475827, -288.4527844766014937, -371.0346526505627480 ) ) ;
#34804=CARTESIAN_POINT ( 'NONE',  ( 807.5423716828161105, -369.0783235625956422, -362.2119215644372048 ) ) ;
#34805=CARTESIAN_POINT ( 'NONE',  ( 767.7687537140311633, -119.9073299311474443, -372.7932403749916830 ) ) ;
#34806=CARTESIAN_POINT ( 'NONE',  ( 787.5162901302840055, -371.3618753856919739, -305.4481719005792684 ) ) ;
#34812=CARTESIAN_POINT ( 'NONE',  ( 791.1614460488616487, -155.2601417444144261, -373.5763878283158874 ) ) ;
#34818=CARTESIAN_POINT ( 'NONE',  ( 772.4837098697144029, 0.6381246143067236254, -374.5518280994205611 ) ) ;
#34822=CARTESIAN_POINT ( 'NONE',  ( 748.6759233522253680, -424.3726999360612808, -324.3348316497537098 ) ) ;
#34825=CARTESIAN_POINT ( 'NONE',  ( 755.0636971347428243, -268.2709662947833067, -341.7834795799807353 ) ) ;
#34828=CARTESIAN_POINT ( 'NONE',  ( 760.7433823573367135, -252.0090635724254184, -355.9930595647440441 ) ) ;
#34829=CARTESIAN_POINT ( 'NONE',  ( 805.1927285166397041, -256.8164208402379245, -341.8018195045277707 ) ) ;
#34830=AXIS2_PLACEMENT_3D ( 'NONE', #32006, #27630, #42406 ) ;
#34832=CARTESIAN_POINT ( 'NONE',  ( 781.8018195045266339, -94.27096629478386092, -365.1927285166406705 ) ) ;
#34836=CARTESIAN_POINT ( 'NONE',  ( 795.8262568251477660, -46.37269993606239638, -308.3538107759623585 ) ) ;
#34842=CARTESIAN_POINT ( 'NONE',  ( 773.4516893846965786, 4.354572791210176597, -315.8398074228977066 ) ) ;
#34843=CARTESIAN_POINT ( 'NONE',  ( 814.9108240113580450, -64.27096629478397460, -337.5031285880265273 ) ) ;
#34845=CARTESIAN_POINT ( 'NONE',  ( 755.0636971347428243, -436.2709662947827951, -341.7834795799807353 ) ) ;
#34848=CARTESIAN_POINT ( 'NONE',  ( 787.4397851343537695, -189.7255117493290300, -374.2001403089903988 ) ) ;
#34854=DIRECTION ( 'NONE',  ( 0.000000000000000000, 0.000000000000000000, -1.000000000000000000 ) ) ;
#34855=CARTESIAN_POINT ( 'NONE',  ( 758.0141637701419768, -255.0783235625958980, -367.2620300519063790 ) ) ;
#34857=CARTESIAN_POINT ( 'NONE',  ( 782.4968714119720516, -274.8164208402378108, -305.0891759886411023 ) ) ;
#34862=CARTESIAN_POINT ( 'NONE',  ( 801.9858362298568863, -27.07832356259665474, -312.7379699480935642 ) ) ;
#34863=CARTESIAN_POINT ( 'NONE',  ( 781.7834795799800531, -394.8164208402374697, -315.0636971347436202 ) ) ;
#34866=CARTESIAN_POINT ( 'NONE',  ( 791.1614460488616487, -59.26014174441473870, -373.5763878283158874 ) ) ;
#34867=CARTESIAN_POINT ( 'NONE',  ( 755.8398074228967971, -187.4419599262325278, -333.4516893846970333 ) ) ;
#34870=VERTEX_POINT ( 'NONE', #18081 ) ;
#34871=CARTESIAN_POINT ( 'NONE',  ( 756.5762568750052424, -51.18005720387493085, -348.7366044899774238 ) ) ;
#34872=CARTESIAN_POINT ( 'NONE',  ( 786.6156483768007774, -217.4419599262324141, -315.5913626894246136 ) ) ;
#34875=CARTESIAN_POINT ( 'NONE',  ( 808.7758568127978833, -4.169232653505813069, -320.0363995740631822 ) ) ;
#34880=CARTESIAN_POINT ( 'NONE',  ( 752.7379699480933368, -300.0090635724252479, -361.9858362298580232 ) ) ;
#34885=CARTESIAN_POINT ( 'NONE',  ( 796.9571628226829034, -143.4636090269711701, -321.2382568024804641 ) ) ;
#34886=CARTESIAN_POINT ( 'NONE',  ( 797.6776695296629214, -139.5436935675110135, -357.6776695296636603 ) ) ;
#34888=CARTESIAN_POINT ( 'NONE',  ( 794.9819416627830151, -324.9982390220559409, -319.9864689768909898 ) ) ;
#34896=CARTESIAN_POINT ( 'NONE',  ( 748.6759233522253680, -376.3726999360614514, -324.3348316497537098 ) ) ;
#34900=CARTESIAN_POINT ( 'NONE',  ( 758.0580252608178853, -318.4527844766014368, -328.0187753319985404 ) ) ;
#34904=CARTESIAN_POINT ( 'NONE',  ( 802.9823548866075953, -217.0999726633345972, -330.0799878456151077 ) ) ;
#34909=CARTESIAN_POINT ( 'NONE',  ( 747.2067596250078623, -411.1800572038738437, -352.2312462859687230 ) ) ;
#34914=CARTESIAN_POINT ( 'NONE',  ( 772.4837098697144029, -71.36187538569302546, -374.5518280994205611 ) ) ;
#34915=CARTESIAN_POINT ( 'NONE',  ( 759.9864689768902508, -290.0891481129650629, -354.9819416627836404 ) ) ;
#34921=CARTESIAN_POINT ( 'NONE',  ( 814.8207195650702488, -26.19088175424427334, -336.2433038121456548 ) ) ;
#34922=CARTESIAN_POINT ( 'NONE',  ( 795.9930595647434757, -75.07832356259649487, -320.7433823573372820 ) ) ;
#34928=ORIENTED_EDGE ( 'NONE', *, *, #18974, .T. ) ;
#34929=CARTESIAN_POINT ( 'NONE',  ( 755.0636971347428243, -52.27096629478401724, -341.7834795799807353 ) ) ;
#34930=CARTESIAN_POINT ( 'NONE',  ( 798.7617431975189675, -363.6237781080502032, -323.0428371773161871 ) ) ;
#34934=CARTESIAN_POINT ( 'NONE',  ( 764.3348316497523456, -382.7146871989591546, -308.6759233522265617 ) ) ;
#34940=CARTESIAN_POINT ( 'NONE',  ( 811.0346526505616112, -254.6346026584196238, -323.0537975583477532 ) ) ;
#34943=CARTESIAN_POINT ( 'NONE',  ( 774.6312213355098493, -215.3618753856925707, -364.6798772138717482 ) ) ;
#34945=CARTESIAN_POINT ( 'NONE',  ( 759.7806653035534055, -366.9982390220556567, -324.8639956371180801 ) ) ;
#34946=CARTESIAN_POINT ( 'NONE',  ( 803.6646147819161570, -17.90732993114776406, -348.8264449731210561 ) ) ;
#34951=CARTESIAN_POINT ( 'NONE',  ( 802.5472867521000353, -460.3726999360611103, -350.8726784830461156 ) ) ;
#34953=CARTESIAN_POINT ( 'NONE',  ( 787.4999999999992042, -462.9681489794447202, -270.0000000000000568 ) ) ;
#34956=CARTESIAN_POINT ( 'NONE',  ( 766.4474001241216001, -259.0999726633343698, -307.3154664389482491 ) ) ;
#34959=CARTESIAN_POINT ( 'NONE',  ( 800.0135310231082713, -206.0891481129653471, -325.0180583372163028 ) ) ;
#34960=CARTESIAN_POINT ( 'NONE',  ( 796.7845633553578182, -393.6237781080500326, -358.5707757039688204 ) ) ;
#34963=CARTESIAN_POINT ( 'NONE',  ( 761.4292242960306112, -113.4636090269712554, -323.2154366446414429 ) ) ;
#34966=CARTESIAN_POINT ( 'NONE',  ( 791.1614460488616487, 12.73985825558503926, -373.5763878283158874 ) ) ;
#34967=CARTESIAN_POINT ( 'NONE',  ( 811.0346526505617248, -302.6346026584195670, -323.0537975583478101 ) ) ;
#34970=CARTESIAN_POINT ( 'NONE',  ( 781.7834795799800531, -82.81642084023846451, -315.0636971347436202 ) ) ;
#34972=CARTESIAN_POINT ( 'NONE',  ( 783.7566961878529810, -216.8965053807778816, -305.1792804349288417 ) ) ;
#34974=CARTESIAN_POINT ( 'NONE',  ( 747.2067596250078623, -435.1800572038737869, -352.2312462859687230 ) ) ;
#34984=CARTESIAN_POINT ( 'NONE',  ( 800.7704444035546203, -268.1692326535049347, -326.0291762391768771 ) ) ;
#34988=CARTESIAN_POINT ( 'NONE',  ( 761.9338519418445230, -278.5328690171412518, -370.4231160770881957 ) ) ;
#34993=CARTESIAN_POINT ( 'NONE',  ( 765.8855110935204493, -46.16923265350568784, -319.0159684113471599 ) ) ;
#34994=CARTESIAN_POINT ( 'NONE',  ( 768.0187753319979720, -176.6346026584199933, -318.0580252608186242 ) ) ;
#34995=CARTESIAN_POINT ( 'NONE',  ( 762.3223304703356007, -199.5436935675108430, -322.3223304703362828 ) ) ;
#34997=CARTESIAN_POINT ( 'NONE',  ( 782.4968714119720516, -106.8164208402383935, -305.0891759886411023 ) ) ;
#34998=CARTESIAN_POINT ( 'NONE',  ( 781.7834795799800531, -106.8164208402383935, -315.0636971347436202 ) ) ;
#35000=CARTESIAN_POINT ( 'NONE',  ( 757.4527132478984868, -400.3726999360612808, -329.1273215169538844 ) ) ;
#35009=CARTESIAN_POINT ( 'NONE',  ( 761.4292242960306112, -353.4636090269705733, -323.2154366446414429 ) ) ;
#35010=CARTESIAN_POINT ( 'NONE',  ( 758.0580252608178853, -342.4527844766013231, -328.0187753319985404 ) ) ;
#35011=CARTESIAN_POINT ( 'NONE',  ( 776.2046728542105711, -164.1908817542438612, -304.8212110874238761 ) ) ;
#35015=CARTESIAN_POINT ( 'NONE',  ( 760.5453621957607311, -285.0783235625958127, -323.8424801807151425 ) ) ;
#35017=CARTESIAN_POINT ( 'NONE',  ( 791.0478386215596629, -141.8272453906075157, -306.7653713866226326 ) ) ;
#35023=CARTESIAN_POINT ( 'NONE',  ( 751.6929314249750860, -222.9982390220561683, -318.8095938919659034 ) ) ;
#35025=AXIS2_PLACEMENT_3D ( 'NONE', #9298, #23367, #37469 ) ;
#35027=CARTESIAN_POINT ( 'NONE',  ( 749.2812353651451076, -342.4527844766013231, -323.2262854647983090 ) ) ;
#35033=CARTESIAN_POINT ( 'NONE',  ( 808.7758568127978833, -388.1692326535045936, -320.0363995740631822 ) ) ;
#35034=CARTESIAN_POINT ( 'NONE',  ( 811.0346526505616112, -110.6346026584201638, -323.0537975583477532 ) ) ;
#35036=CARTESIAN_POINT ( 'NONE',  ( 755.2512626584698410, -415.5436935675102177, -315.2512626584710915 ) ) ;
#35041=CARTESIAN_POINT ( 'NONE',  ( 746.0683387631852383, -163.4419599262325846, -331.3260364891676204 ) ) ;
#35046=CARTESIAN_POINT ( 'NONE',  ( 771.2633955100217236, -143.9073299311473590, -363.4237431249939618 ) ) ;
#35049=CARTESIAN_POINT ( 'NONE',  ( 754.9967657858570647, -25.54369356751136877, -365.0032342141425374 ) ) ;
#35053=CARTESIAN_POINT ( 'NONE',  ( 814.2805881961230625, -409.6454272087884760, -331.2368401574024119 ) ) ;
#35054=VECTOR ( 'NONE', #20760, 1000.000000000000000 ) ;
#35055=VERTEX_POINT ( 'NONE', #28227 ) ;
#35056=CARTESIAN_POINT ( 'NONE',  ( 805.1927285166397041, -256.8164208402379245, -341.8018195045277707 ) ) ;
#35060=CARTESIAN_POINT ( 'NONE',  ( 755.1538015810308480, -254.1908817542435770, -343.0433043558613804 ) ) ;
#35061=CARTESIAN_POINT ( 'NONE',  ( 791.9812246680005501, -236.6346026584198228, -361.9419747391813189 ) ) ;
#35062=CARTESIAN_POINT ( 'NONE',  ( 755.5713283507202505, -437.3618753856919170, -334.6858677611754729 ) ) ;
#35063=CARTESIAN_POINT ( 'NONE',  ( 755.5713283507202505, -125.3618753856928834, -334.6858677611754729 ) ) ;
#35064=EDGE_CURVE ( 'NONE', #30163, #17451, #3760, .T. ) ;
#35068=CARTESIAN_POINT ( 'NONE',  ( 778.7629533639073998, -32.73633629969879877, -375.0009284576466371 ) ) ;
#35076=CARTESIAN_POINT ( 'NONE',  ( 763.8424801807145741, -18.00906357242611477, -320.5453621957614700 ) ) ;
#35077=CARTESIAN_POINT ( 'NONE',  ( 745.4481719005789273, -75.72551174932938522, -347.5162901302853697 ) ) ;
#35081=CARTESIAN_POINT ( 'NONE',  ( 815.2698199232961542, -184.8164208402380950, -342.5225473063383106 ) ) ;
#35086=CARTESIAN_POINT ( 'NONE',  ( 786.2056067578752163, -275.8055962898685038, -374.4686193811670023 ) ) ;
#35088=CARTESIAN_POINT ( 'NONE',  ( 763.2262854647970016, -296.6346026584195670, -309.2812353651462445 ) ) ;
#35092=CARTESIAN_POINT ( 'NONE',  ( 791.9812246680005501, -380.6346026584192828, -361.9419747391813189 ) ) ;
#35094=CARTESIAN_POINT ( 'NONE',  ( 756.5762568750052424, -195.1800572038744974, -348.7366044899774238 ) ) ;
#35095=CARTESIAN_POINT ( 'NONE',  ( 793.4146539503750546, -49.98741447168749374, -307.6481478633938877 ) ) ;
#35096=CARTESIAN_POINT ( 'NONE',  ( 802.7791456095903868, -196.7146871989598083, -329.0155153010375102 ) ) ;
#35100=CARTESIAN_POINT ( 'NONE',  ( 801.3366627262608972, -200.5328690171415644, -353.0897708529566899 ) ) ;
#35104=CARTESIAN_POINT ( 'NONE',  ( 764.3348316497523456, -46.71468719896022748, -308.6759233522265617 ) ) ;
#35109=CARTESIAN_POINT ( 'NONE',  ( 802.2119215644370342, -318.0090635724251911, -367.5423716828165084 ) ) ;
#35114=CARTESIAN_POINT ( 'NONE',  ( 799.2566176426618085, -144.0090635724257027, -324.0069404352559559 ) ) ;
#35115=CARTESIAN_POINT ( 'NONE',  ( 762.1405469898971887, -145.5436935675109851, -357.8594530101015607 ) ) ;
#35116=CARTESIAN_POINT ( 'NONE',  ( 785.3141322388236176, -357.7255117493285184, -364.4286716492789537 ) ) ;
#35126=CARTESIAN_POINT ( 'NONE',  ( 771.3260364891663130, -379.6454272087886466, -306.0683387631859773 ) ) ;
#35130=CARTESIAN_POINT ( 'NONE',  ( 792.1044303154645831, -348.4527844766012663, -317.8323909638837677 ) ) ;
#35132=CARTESIAN_POINT ( 'NONE',  ( 758.4439275373578084, -228.5545181178799794, -353.2243759319684386 ) ) ;
#35137=CARTESIAN_POINT ( 'NONE',  ( 813.1304606946831655, -401.9073299311464211, -352.3570229623691716 ) ) ;
#35142=CARTESIAN_POINT ( 'NONE',  ( 809.6099558218720631, -452.9681489794449476, -335.1781210895659342 ) ) ;
#35144=CARTESIAN_POINT ( 'NONE',  ( 748.9653473494363425, -50.63460265842036989, -356.9462024416521331 ) ) ;
#35145=CARTESIAN_POINT ( 'NONE',  ( 771.1735550268778070, -297.1800572038740711, -316.3353852180827630 ) ) ;
#35149=CARTESIAN_POINT ( 'NONE',  ( 762.1177392798416577, -18.55451811788065797, -309.8865473780659272 ) ) ;
#35150=CARTESIAN_POINT ( 'NONE',  ( 803.8651313633788504, -101.2601417444146250, -332.4468031744301015 ) ) ;
#35155=CARTESIAN_POINT ( 'NONE',  ( 755.0636971347428243, -4.270966294784170003, -341.7834795799807353 ) ) ;
#35156=CARTESIAN_POINT ( 'NONE',  ( 798.7617431975189675, -99.62377810805098477, -323.0428371773161871 ) ) ;
#35158=CARTESIAN_POINT ( 'NONE',  ( 804.9363028652555840, -64.27096629478397460, -338.2165204200192079 ) ) ;
#35160=CARTESIAN_POINT ( 'NONE',  ( 769.1273215169530886, -406.7146871989590409, -317.4527132478988847 ) ) ;
#35165=CARTESIAN_POINT ( 'NONE',  ( 749.8865473780648472, -404.5328690171409107, -322.1177392798429082 ) ) ;
#35175=CARTESIAN_POINT ( 'NONE',  ( 782.5225473063381969, -238.2709662947833920, -375.2698199232970637 ) ) ;
#35179=CARTESIAN_POINT ( 'NONE',  ( 759.9864689768902508, -242.0891481129652618, -354.9819416627836404 ) ) ;
#35181=CARTESIAN_POINT ( 'NONE',  ( 771.1735550268778070, -345.1800572038739006, -316.3353852180827630 ) ) ;
#35182=CARTESIAN_POINT ( 'NONE',  ( 755.5713283507202505, -5.361875385693257279, -334.6858677611754729 ) ) ;
#35187=CARTESIAN_POINT ( 'NONE',  ( 762.1405469898971887, -25.54369356751136877, -357.8594530101015607 ) ) ;
#35188=CARTESIAN_POINT ( 'NONE',  ( 755.2512626584698410, 16.45630643248849267, -315.2512626584710915 ) ) ;
#35191=CARTESIAN_POINT ( 'NONE',  ( 814.4686193811664907, -267.2817908451526137, -346.2056067578752732 ) ) ;
#35194=CARTESIAN_POINT ( 'NONE',  ( 785.3141322388236176, -213.7255117493289731, -364.4286716492789537 ) ) ;
#35195=CARTESIAN_POINT ( 'NONE',  ( 790.8726784830453198, -394.7146871989591546, -362.5472867521010585 ) ) ;
#35197=CARTESIAN_POINT ( 'NONE',  ( 759.0159684113467620, -112.9181544815167229, -325.8855110935213020 ) ) ;
#35201=CARTESIAN_POINT ( 'NONE',  ( 813.9316612368132837, 16.55804007376685050, -348.6739635108323228 ) ) ;
#35202=CARTESIAN_POINT ( 'NONE',  ( 749.2812353651451076, -318.4527844766014368, -323.2262854647983090 ) ) ;
#35204=CARTESIAN_POINT ( 'NONE',  ( 803.6646147819161570, -89.90732993114750116, -348.8264449731210561 ) ) ;
#35207=CARTESIAN_POINT ( 'NONE',  ( 786.2056067578752163, -203.8055962898688449, -374.4686193811670023 ) ) ;
#35209=CARTESIAN_POINT ( 'NONE',  ( 744.7301800767019131, -436.8164208402372992, -337.4774526936615757 ) ) ;
#35210=CIRCLE ( 'NONE', #43329, 30.00000000000008171 ) ;
#35214=CARTESIAN_POINT ( 'NONE',  ( 798.7617431975189675, 20.37622189194865285, -323.0428371773161871 ) ) ;
#35219=VERTEX_POINT ( 'NONE', #33748 ) ;
#35220=CARTESIAN_POINT ( 'NONE',  ( 803.2186876482843445, -247.9874144716867761, -350.0220218866286928 ) ) ;
#35222=CARTESIAN_POINT ( 'NONE',  ( 791.1614460488616487, -299.2601417444139997, -373.5763878283158874 ) ) ;
#35227=CARTESIAN_POINT ( 'NONE',  ( 801.3366627262608972, -32.53286901714208312, -353.0897708529566899 ) ) ;
#35228=CARTESIAN_POINT ( 'NONE',  ( 785.3141322388236176, -213.7255117493289731, -364.4286716492789537 ) ) ;
#35230=CARTESIAN_POINT ( 'NONE',  ( 787.5162901302840055, -155.3618753856927128, -305.4481719005792684 ) ) ;
#35231=CARTESIAN_POINT ( 'NONE',  ( 765.0180583372156207, -144.9982390220564525, -360.0135310231089534 ) ) ;
#35234=CARTESIAN_POINT ( 'NONE',  ( 761.4292242960306112, -377.4636090269704596, -323.2154366446414429 ) ) ;
#35241=ORIENTED_EDGE ( 'NONE', *, *, #17279, .T. ) ;
#35242=CARTESIAN_POINT ( 'NONE',  ( 763.8424801807145741, -378.0090635724250774, -320.5453621957614700 ) ) ;
#35243=CARTESIAN_POINT ( 'NONE',  ( 765.0180583372156207, -360.9982390220557704, -360.0135310231089534 ) ) ;
#35244=CARTESIAN_POINT ( 'NONE',  ( 754.3581564841646241, -161.4636090269711133, -316.1443688327762516 ) ) ;
#35248=CARTESIAN_POINT ( 'NONE',  ( 764.0069404352550464, -279.0783235625958127, -359.2566176426627180 ) ) ;
#35249=CARTESIAN_POINT ( 'NONE',  ( 756.3353852180819104, -437.9073299311463074, -331.1735550268788302 ) ) ;
#35250=CARTESIAN_POINT ( 'NONE',  ( 748.6759233522253680, -160.3726999360620482, -324.3348316497537098 ) ) ;
#35255=CARTESIAN_POINT ( 'NONE',  ( 792.3570229623691148, -213.1800572038743837, -373.1304606946836770 ) ) ;
#35259=CARTESIAN_POINT ( 'NONE',  ( 791.1614460488616487, -107.2601417444145824, -373.5763878283158874 ) ) ;
#35261=CARTESIAN_POINT ( 'NONE',  ( 772.4837098697144029, -335.3618753856920307, -374.5518280994205611 ) ) ;
#35266=CARTESIAN_POINT ( 'NONE',  ( 764.3348316497523456, -406.7146871989590409, -308.6759233522265617 ) ) ;
#35268=CARTESIAN_POINT ( 'NONE',  ( 754.9967657858570647, -145.5436935675109851, -365.0032342141425374 ) ) ;
#35269=CARTESIAN_POINT ( 'NONE',  ( 748.9653473494363425, -434.6346026584190554, -356.9462024416521331 ) ) ;
#35270=CARTESIAN_POINT ( 'NONE',  ( 799.9999999999993179, 205.0000000000000568, -339.9999999999999432 ) ) ;
#35272=ORIENTED_EDGE ( 'NONE', *, *, #15065, .T. ) ;
#35273=CARTESIAN_POINT ( 'NONE',  ( 807.5423716828161105, -201.0783235625961254, -362.2119215644372048 ) ) ;
#35279=CARTESIAN_POINT ( 'NONE',  ( 755.2512626584698410, -31.54369356751135456, -315.2512626584710915 ) ) ;
#35283=CARTESIAN_POINT ( 'NONE',  ( 764.1737431748507561, -442.3726999360611103, -371.6461892240376415 ) ) ;
#35287=CARTESIAN_POINT ( 'NONE',  ( 802.1676090361156639, -254.6346026584196238, -327.8955696845344505 ) ) ;
#35291=CARTESIAN_POINT ( 'NONE',  ( 783.0745993439762742, -248.1908817542435202, -365.1016975059196739 ) ) ;
#35292=CARTESIAN_POINT ( 'NONE',  ( 771.2633955100217236, -263.9073299311469327, -363.4237431249939618 ) ) ;
#35293=CARTESIAN_POINT ( 'NONE',  ( 790.0183182880230106, -452.9681489794449476, -362.9048749981275250 ) ) ;
#35294=CARTESIAN_POINT ( 'NONE',  ( 756.5762568750052424, -123.1800572038747106, -348.7366044899774238 ) ) ;
#35300=CARTESIAN_POINT ( 'NONE',  ( 755.8990559732751535, -59.46360902697142592, -365.9055244015606831 ) ) ;
#35306=CARTESIAN_POINT ( 'NONE',  ( 757.4527132478984868, -16.37269993606248519, -329.1273215169538844 ) ) ;
#35307=CARTESIAN_POINT ( 'NONE',  ( 746.8695393053151292, -101.9073299311474869, -327.6429770376306578 ) ) ;
#35309=CARTESIAN_POINT ( 'NONE',  ( 795.1360043628807261, -452.0891481129646650, -360.2193346964456282 ) ) ;
#35311=CARTESIAN_POINT ( 'NONE',  ( 763.2262854647970016, -224.6346026584198228, -309.2812353651462445 ) ) ;
#35314=CARTESIAN_POINT ( 'NONE',  ( 744.9990715423526808, -282.3510508353230080, -341.2370466360926002 ) ) ;
#35316=CARTESIAN_POINT ( 'NONE',  ( 813.1304606946830518, -305.9073299311467622, -352.3570229623690580 ) ) ;
#35320=CARTESIAN_POINT ( 'NONE',  ( 771.1735550268778070, -393.1800572038737300, -316.3353852180827630 ) ) ;
#35322=CARTESIAN_POINT ( 'NONE',  ( 807.5423716828161105, -81.07832356259649487, -362.2119215644372048 ) ) ;
#35328=CARTESIAN_POINT ( 'NONE',  ( 760.5453621957607311, -213.0783235625960401, -323.8424801807151425 ) ) ;
#35331=CARTESIAN_POINT ( 'NONE',  ( 747.3154664389472828, -19.98741447168758256, -326.4474001241230781 ) ) ;
#35336=CARTESIAN_POINT ( 'NONE',  ( 748.6759233522253680, -304.3726999360615082, -324.3348316497537098 ) ) ;
#35340=CARTESIAN_POINT ( 'NONE',  ( 761.4292242960306112, -161.4636090269711133, -323.2154366446414429 ) ) ;
#35341=CARTESIAN_POINT ( 'NONE',  ( 788.8264449731200330, -141.1800572038746395, -363.6646147819171233 ) ) ;
#35342=CARTESIAN_POINT ( 'NONE',  ( 755.5713283507202505, -341.3618753856922012, -334.6858677611754729 ) ) ;
#35343=ORIENTED_EDGE ( 'NONE', *, *, #17738, .F. ) ;
#35352=CARTESIAN_POINT ( 'NONE',  ( 768.9521613784389729, -393.8272453906067199, -373.2346286133773106 ) ) ;
#35353=CARTESIAN_POINT ( 'NONE',  ( 777.4774526936600978, -10.27096629478415046, -304.7301800767028226 ) ) ;
#35355=VECTOR ( 'NONE', #36104, 1000.000000000000000 ) ;
#35357=CARTESIAN_POINT ( 'NONE',  ( 759.7806653035534055, -366.9982390220556567, -324.8639956371180801 ) ) ;
#35359=CARTESIAN_POINT ( 'NONE',  ( 776.9254006560222479, -236.1908817542436338, -314.8983024940802125 ) ) ;
#35363=CARTESIAN_POINT ( 'NONE',  ( 745.4481719005789273, -411.7255117493282910, -347.5162901302853697 ) ) ;
#35368=CARTESIAN_POINT ( 'NONE',  ( 782.5225473063381969, -46.27096629478404566, -375.2698199232970637 ) ) ;
#35369=CARTESIAN_POINT ( 'NONE',  ( 764.8639956371174549, -272.0891481129651197, -319.7806653035542013 ) ) ;
#35374=CARTESIAN_POINT ( 'NONE',  ( 749.5768839229115201, -36.55451811788061178, -358.0661480581553064 ) ) ;
#35375=CARTESIAN_POINT ( 'NONE',  ( 764.0069404352550464, -87.07832356259646645, -359.2566176426627180 ) ) ;
#35380=CARTESIAN_POINT ( 'NONE',  ( 759.9864689768902508, -98.08914811296568814, -354.9819416627836404 ) ) ;
#35383=CARTESIAN_POINT ( 'NONE',  ( 793.2243759319678702, -410.5328690171408539, -318.4439275373583200 ) ) ;
#35386=CARTESIAN_POINT ( 'NONE',  ( 748.3538107759620743, -400.7146871989590977, -355.8262568251490165 ) ) ;
#35392=CARTESIAN_POINT ( 'NONE',  ( 796.7737145352015204, -236.6346026584198228, -370.7187646348536987 ) ) ;
#35396=CARTESIAN_POINT ( 'NONE',  ( 781.7834795799800531, -250.8164208402379245, -315.0636971347436202 ) ) ;
#35399=CARTESIAN_POINT ( 'NONE',  ( 754.8072714833581358, -364.8164208402374697, -338.1981804954720587 ) ) ;
#35400=CARTESIAN_POINT ( 'NONE',  ( 756.3353852180819104, -29.90732993114771787, -331.1735550268788302 ) ) ;
#35406=CARTESIAN_POINT ( 'NONE',  ( 762.3223304703356007, -7.543693567511430942, -322.3223304703362828 ) ) ;
#35411=CARTESIAN_POINT ( 'NONE',  ( 793.5525998758768083, -271.0999726633344267, -372.6845335610516941 ) ) ;
#35414=CARTESIAN_POINT ( 'NONE',  ( 778.1981804954714335, -274.2709662947833067, -314.8072714833589885 ) ) ;
#35415=CARTESIAN_POINT ( 'NONE',  ( 795.9930595647434757, -411.0783235625954717, -320.7433823573372820 ) ) ;
#35417=CARTESIAN_POINT ( 'NONE',  ( 757.0176451133909268, -133.0999726633348246, -349.9200121543848354 ) ) ;
#35419=CARTESIAN_POINT ( 'NONE',  ( 798.0661480581538854, -2.532869017142183932, -309.5768839229118043 ) ) ;
#35420=CARTESIAN_POINT ( 'NONE',  ( 746.8695393053151292, -317.9073299311467622, -327.6429770376306578 ) ) ;
#35425=CARTESIAN_POINT ( 'NONE',  ( 756.1443688327750579, -189.6237781080507148, -314.3581564841659315 ) ) ;
#35427=CARTESIAN_POINT ( 'NONE',  ( 762.1177392798416577, 5.445481882119263872, -309.8865473780659272 ) ) ;
#35433=CARTESIAN_POINT ( 'NONE',  ( 755.0488828828309806, 6.194403710130517382, -344.1219089521771934 ) ) ;
#35441=CARTESIAN_POINT ( 'NONE',  ( 754.9735926884551418, -306.3510508353230648, -340.5236548041000333 ) ) ;
#35443=CARTESIAN_POINT ( 'NONE',  ( 807.5423716828161105, -297.0783235625957559, -362.2119215644372048 ) ) ;
#35448=CARTESIAN_POINT ( 'NONE',  ( 787.6308680596127942, -59.26014174441473870, -364.1105419155492768 ) ) ;
#35449=CARTESIAN_POINT ( 'NONE',  ( 781.8018195045266339, -166.2709662947835909, -365.1927285166406705 ) ) ;
#35450=CARTESIAN_POINT ( 'NONE',  ( 764.8639956371174549, -224.0891481129653187, -319.7806653035542013 ) ) ;
#35452=CARTESIAN_POINT ( 'NONE',  ( 812.7932403749906598, -159.1800572038746111, -327.7687537140311633 ) ) ;
#35454=CARTESIAN_POINT ( 'NONE',  ( 771.2633955100217236, -143.9073299311473590, -363.4237431249939618 ) ) ;
#35456=CARTESIAN_POINT ( 'NONE',  ( 766.9102291470427417, -402.5545181178795247, -318.6633372737382501 ) ) ;
#35463=CARTESIAN_POINT ( 'NONE',  ( 805.2837595273609850, -410.7363362996976548, -340.5290396650784714 ) ) ;
#35465=CARTESIAN_POINT ( 'NONE',  ( 750.9282345327678740, -160.9181544815165807, -319.8311093483690115 ) ) ;
#35469=CARTESIAN_POINT ( 'NONE',  ( 756.7813123517142913, -283.9874144716867477, -329.9779781133712504 ) ) ;
#35471=CARTESIAN_POINT ( 'NONE',  ( 747.6481478633932056, -205.0999726633346256, -353.4146539503763620 ) ) ;
#35476=CARTESIAN_POINT ( 'NONE',  ( 812.7932403749906598, -207.1800572038744406, -327.7687537140311633 ) ) ;
#35481=CARTESIAN_POINT ( 'NONE',  ( 795.6651683502461765, -106.7146871989600498, -371.3240766477733814 ) ) ;
#35483=CARTESIAN_POINT ( 'NONE',  ( 777.4774526936600978, -322.2709662947830225, -304.7301800767027657 ) ) ;
#35489=CARTESIAN_POINT ( 'NONE',  ( 746.7653713866222915, -401.2601417444137155, -351.0478386215610271 ) ) ;
#35490=CARTESIAN_POINT ( 'NONE',  ( 746.8695393053150156, -437.9073299311463074, -327.6429770376306010 ) ) ;
#35495=CARTESIAN_POINT ( 'NONE',  ( 810.1134526219336749, -200.5328690171415644, -357.8822607201570349 ) ) ;
#35501=CARTESIAN_POINT ( 'NONE',  ( 813.1304606946830518, -41.90732993114767169, -352.3570229623690580 ) ) ;
#35503=VERTEX_POINT ( 'NONE', #41370 ) ;
#35504=CARTESIAN_POINT ( 'NONE',  ( 810.4231160770870019, -432.5545181178793541, -321.9338519418446936 ) ) ;
#35508=CARTESIAN_POINT ( 'NONE',  ( 759.9864689768902508, -290.0891481129650629, -354.9819416627836404 ) ) ;
#35512=CARTESIAN_POINT ( 'NONE',  ( 780.5236548040995785, -284.7363362996979390, -314.9735926884559944 ) ) ;
#35513=CARTESIAN_POINT ( 'NONE',  ( 803.6646147819161570, -257.9073299311469896, -348.8264449731210561 ) ) ;
#35515=CARTESIAN_POINT ( 'NONE',  ( 767.8955696845333705, -120.4527844766019484, -362.1676090361162323 ) ) ;
#35520=CARTESIAN_POINT ( 'NONE',  ( 754.3581564841646241, -65.46360902697142592, -316.1443688327762516 ) ) ;
#35526=CARTESIAN_POINT ( 'NONE',  ( 780.5236548040995785, -44.73633629969875614, -314.9735926884559944 ) ) ;
#35527=AXIS2_PLACEMENT_3D ( 'NONE', #27513, #3041, #13671 ) ;
#35528=CARTESIAN_POINT ( 'NONE',  ( 747.2067596250078623, -99.18005720387478164, -352.2312462859687230 ) ) ;
#35530=CARTESIAN_POINT ( 'NONE',  ( 799.9999999999993179, 205.0000000000000568, -339.9999999999999432 ) ) ;
#35533=CARTESIAN_POINT ( 'NONE',  ( 745.4481719005789273, -219.7255117493289447, -347.5162901302853129 ) ) ;
#35537=CARTESIAN_POINT ( 'NONE',  ( 793.4146539503750546, -313.9874144716866908, -307.6481478633938877 ) ) ;
#35539=CARTESIAN_POINT ( 'NONE',  ( 796.9462024416508257, -300.4527844766012663, -308.9653473494370246 ) ) ;
#35543=CARTESIAN_POINT ( 'NONE',  ( 795.1360043628807261, -380.0891481129646650, -360.2193346964456282 ) ) ;
#35545=CARTESIAN_POINT ( 'NONE',  ( 745.1769319972822814, -89.80559628986918597, -346.2694204179732083 ) ) ;
#35549=CARTESIAN_POINT ( 'NONE',  ( 755.8398074228967971, -187.4419599262325278, -333.4516893846970333 ) ) ;
#35551=CARTESIAN_POINT ( 'NONE',  ( 746.0683387631852383, -19.44195992623303937, -331.3260364891676204 ) ) ;
#35555=LINE ( 'NONE', #18272, #21257 ) ;
#35558=CARTESIAN_POINT ( 'NONE',  ( 745.7194118038753459, -349.6454272087887603, -348.7631598425976449 ) ) ;
#35561=CARTESIAN_POINT ( 'NONE',  ( 759.0159684113467620, -184.9181544815165239, -325.8855110935213020 ) ) ;
#35562=CARTESIAN_POINT ( 'NONE',  ( 768.0187753319979720, -152.6346026584200786, -318.0580252608186242 ) ) ;
#35563=CARTESIAN_POINT ( 'NONE',  ( 757.8323909638828582, -362.6346026584193964, -352.1044303154654358 ) ) ;
#35571=ORIENTED_EDGE ( 'NONE', *, *, #27299, .T. ) ;
#35572=CARTESIAN_POINT ( 'NONE',  ( 776.2046728542105711, -380.1908817542431507, -304.8212110874238761 ) ) ;
#35574=CARTESIAN_POINT ( 'NONE',  ( 758.8095938919644823, 15.91085188703394593, -311.6929314249762797 ) ) ;
#35577=CARTESIAN_POINT ( 'NONE',  ( 765.0180583372156207, -360.9982390220557704, -360.0135310231089534 ) ) ;
#35580=CARTESIAN_POINT ( 'NONE',  ( 804.1105419155481968, -219.8272453906073167, -347.6308680596136469 ) ) ;
#35583=AXIS2_PLACEMENT_3D ( 'NONE', #41909, #6786, #20862 ) ;
#35585=CARTESIAN_POINT ( 'NONE',  ( 767.7687537140311633, -431.9073299311464211, -372.7932403749916830 ) ) ;
#35591=CARTESIAN_POINT ( 'NONE',  ( 804.7487373415286811, -67.54369356751125508, -364.7487373415288516 ) ) ;
#35592=CARTESIAN_POINT ( 'NONE',  ( 757.8323909638827445, -290.6346026584195101, -352.1044303154654358 ) ) ;
#35596=CARTESIAN_POINT ( 'NONE',  ( 781.2370466360911223, -68.73633629969867798, -304.9990715423533629 ) ) ;
#35597=CARTESIAN_POINT ( 'NONE',  ( 775.9200461376533440, -71.80559628986922860, -315.3028492785443291 ) ) ;
#35601=CARTESIAN_POINT ( 'NONE',  ( 759.9864689768902508, -2.089148112965993231, -354.9819416627836404 ) ) ;
#35602=CARTESIAN_POINT ( 'NONE',  ( 786.6156483768007774, -97.44195992623281199, -315.5913626894246136 ) ) ;
#35604=CARTESIAN_POINT ( 'NONE',  ( 754.8072714833581358, -100.8164208402383792, -338.1981804954720587 ) ) ;
#35605=CARTESIAN_POINT ( 'NONE',  ( 790.8726784830453198, -394.7146871989591546, -362.5472867521010585 ) ) ;
#35610=CARTESIAN_POINT ( 'NONE',  ( 813.9316612368132837, -415.4419599262318457, -348.6739635108323228 ) ) ;
#35617=CARTESIAN_POINT ( 'NONE',  ( 763.0537975583475827, -240.4527844766015221, -371.0346526505627480 ) ) ;
#35621=CARTESIAN_POINT ( 'NONE',  ( 783.0745993439762742, -56.19088175424417386, -365.1016975059196739 ) ) ;
#35622=CARTESIAN_POINT ( 'NONE',  ( 771.2633955100217236, -263.9073299311469327, -363.4237431249939618 ) ) ;
#35624=CARTESIAN_POINT ( 'NONE',  ( 802.1676090361156639, -350.6346026584192828, -327.8955696845344505 ) ) ;
#35625=CARTESIAN_POINT ( 'NONE',  ( 757.8323909638827445, -2.634602658420536869, -352.1044303154654358 ) ) ;
#35631=CARTESIAN_POINT ( 'NONE',  ( 802.1676090361156639, -14.63460265842049424, -327.8955696845344505 ) ) ;
#35635=CARTESIAN_POINT ( 'NONE',  ( 781.2370466360911223, -284.7363362996979390, -304.9990715423533629 ) ) ;
#35638=CARTESIAN_POINT ( 'NONE',  ( 762.1405469898971887, -241.5436935675106156, -357.8594530101015607 ) ) ;
#35640=CARTESIAN_POINT ( 'NONE',  ( 793.0897708529556667, -102.5545181178804057, -361.3366627262616362 ) ) ;
#35644=FACE_OUTER_BOUND ( 'NONE', #40847, .T. ) ;
#35645=CARTESIAN_POINT ( 'NONE',  ( 811.6461892240364477, 19.28531280103956647, -324.1737431748509835 ) ) ;
#35646=CARTESIAN_POINT ( 'NONE',  ( 777.4774526936600978, -298.2709662947831930, -304.7301800767028226 ) ) ;
#35651=CARTESIAN_POINT ( 'NONE',  ( 751.2241431872005251, -208.1692326535051905, -359.9636004259367610 ) ) ;
#35653=CARTESIAN_POINT ( 'NONE',  ( 777.5031285880264704, -430.8164208402374129, -374.9108240113588408 ) ) ;
#35658=CARTESIAN_POINT ( 'NONE',  ( 769.1273215169530886, 25.28531280103955226, -317.4527132478988847 ) ) ;
#35665=CARTESIAN_POINT ( 'NONE',  ( 764.0069404352550464, -279.0783235625958127, -359.2566176426627180 ) ) ;
#35667=CARTESIAN_POINT ( 'NONE',  ( 786.2056067578752163, -299.8055962898685038, -374.4686193811670023 ) ) ;
#35672=CARTESIAN_POINT ( 'NONE',  ( 765.8855110935204493, -94.16923265350555994, -319.0159684113471599 ) ) ;
#35673=CARTESIAN_POINT ( 'NONE',  ( 774.6858677611749044, -153.7255117493291721, -315.5713283507209894 ) ) ;
#35674=CARTESIAN_POINT ( 'NONE',  ( 778.1981804954714335, -202.2709662947834772, -314.8072714833589885 ) ) ;
#35676=CARTESIAN_POINT ( 'NONE',  ( 792.3570229623688874, -141.1800572038746395, -373.1304606946836202 ) ) ;
#35678=CIRCLE ( 'NONE', #36444, 20.00000000000001776 ) ;
#35679=CARTESIAN_POINT ( 'NONE',  ( 764.8639956371174549, -152.0891481129655460, -319.7806653035542581 ) ) ;
#35682=CARTESIAN_POINT ( 'NONE',  ( 793.9708237608222134, -382.9181544815159555, -319.2295555964448681 ) ) ;
#35691=CARTESIAN_POINT ( 'NONE',  ( 798.5707757039680246, -389.4636090269704027, -356.7845633553585003 ) ) ;
#35693=CARTESIAN_POINT ( 'NONE',  ( 768.9521613784389729, -177.8272453906074304, -373.2346286133773106 ) ) ;
#35698=CARTESIAN_POINT ( 'NONE',  ( 755.8398074228967971, -283.4419599262321867, -333.4516893846970333 ) ) ;
#35700=CARTESIAN_POINT ( 'NONE',  ( 807.2620300519052989, -192.0090635724255606, -318.0141637701419768 ) ) ;
#35707=CARTESIAN_POINT ( 'NONE',  ( 758.8095938919644823, -224.0891481129652902, -311.6929314249762797 ) ) ;
#35708=DIRECTION ( 'NONE',  ( 0.000000000000000000, -1.000000000000000000, 0.000000000000000000 ) ) ;
#35709=CARTESIAN_POINT ( 'NONE',  ( 802.1676090361156639, 9.365397341579420498, -327.8955696845344505 ) ) ;
#35711=CARTESIAN_POINT ( 'NONE',  ( 786.2056067578752163, -83.80559628986920018, -374.4686193811670023 ) ) ;
#35713=CARTESIAN_POINT ( 'NONE',  ( 787.5162901302840055, -323.3618753856923149, -305.4481719005792684 ) ) ;
#35721=CARTESIAN_POINT ( 'NONE',  ( 773.7943932421234194, -407.8055962898681628, -305.5313806188329409 ) ) ;
#35722=CARTESIAN_POINT ( 'NONE',  ( 804.7487373415286811, -427.5436935675101040, -364.7487373415288516 ) ) ;
#35728=CARTESIAN_POINT ( 'NONE',  ( 808.7758568127978833, -196.1692326535052473, -320.0363995740631822 ) ) ;
#35735=AXIS2_PLACEMENT_3D ( 'NONE', #16980, #41694, #31285 ) ;
#35736=CARTESIAN_POINT ( 'NONE',  ( 801.1904061080336987, -44.08914811296584446, -368.3070685750235498 ) ) ;
#35738=VERTEX_POINT ( 'NONE', #21016 ) ;
#35739=CARTESIAN_POINT ( 'NONE',  ( 797.8822607201568644, -462.5545181178792973, -370.1134526219340160 ) ) ;
#35745=CARTESIAN_POINT ( 'NONE',  ( 804.6798772138708955, -303.7255117493287457, -334.6312213355107019 ) ) ;
#35751=CARTESIAN_POINT ( 'NONE',  ( 790.0220218866281812, -295.0999726633343698, -363.2186876482849129 ) ) ;
#35752=CARTESIAN_POINT ( 'NONE',  ( 758.0580252608178853, -294.4527844766013800, -328.0187753319985404 ) ) ;
#35753=CARTESIAN_POINT ( 'NONE',  ( 758.0580252608178853, -438.4527844766009821, -328.0187753319985404 ) ) ;
#35754=CARTESIAN_POINT ( 'NONE',  ( 764.8639956371174549, -104.0891481129656881, -319.7806653035542013 ) ) ;
#35755=CIRCLE ( 'NONE', #42411, 30.00000000000002842 ) ;
#35760=CARTESIAN_POINT ( 'NONE',  ( 755.8990559732751535, -83.46360902697136908, -365.9055244015606831 ) ) ;
#35767=CARTESIAN_POINT ( 'NONE',  ( 761.4292242960306112, -41.46360902697149697, -323.2154366446414429 ) ) ;
#35768=CARTESIAN_POINT ( 'NONE',  ( 815.2698199232962679, -88.81642084023843609, -342.5225473063383674 ) ) ;
#35770=CARTESIAN_POINT ( 'NONE',  ( 769.9999999999992042, 178.9475563372491251, -320.0000000000000000 ) ) ;
#35772=CARTESIAN_POINT ( 'NONE',  ( 745.7998596910086917, -221.3618753856925707, -332.5602148656461168 ) ) ;
#35778=CARTESIAN_POINT ( 'NONE',  ( 812.6845335610512393, -319.9874144716866340, -353.5525998758768651 ) ) ;
#35780=CARTESIAN_POINT ( 'NONE',  ( 792.2312462859673587, -299.9073299311468759, -307.2067596250082602 ) ) ;
#35784=CARTESIAN_POINT ( 'NONE',  ( 767.8955696845333705, -432.4527844766008684, -362.1676090361162323 ) ) ;
#35786=CARTESIAN_POINT ( 'NONE',  ( 774.6312213355099630, -191.3618753856925991, -364.6798772138717482 ) ) ;
#35788=CARTESIAN_POINT ( 'NONE',  ( 815.0009284576459549, -78.35105083532376113, -338.7629533639073429 ) ) ;
#35793=CARTESIAN_POINT ( 'NONE',  ( 796.7845633553578182, -201.6237781080506863, -358.5707757039688204 ) ) ;
#35795=CARTESIAN_POINT ( 'NONE',  ( 759.8311093483677041, -22.16923265350575889, -310.9282345327691814 ) ) ;
#35802=CARTESIAN_POINT ( 'NONE',  ( 744.6391490659812007, -350.7363362996978253, -338.7502325331110455 ) ) ;
#35807=CARTESIAN_POINT ( 'NONE',  ( 790.0220218866281812, -199.0999726633346825, -363.2186876482849129 ) ) ;
#35808=CARTESIAN_POINT ( 'NONE',  ( 795.1360043628807261, -188.0891481129653187, -360.2193346964456282 ) ) ;
#35809=CARTESIAN_POINT ( 'NONE',  ( 803.6646147819162707, -353.9073299311467053, -348.8264449731211130 ) ) ;
#35812=FACE_BOUND ( 'NONE', #44138, .T. ) ;
#35817=CARTESIAN_POINT ( 'NONE',  ( 762.1177392798416577, -426.5545181178794678, -309.8865473780659272 ) ) ;
#35819=CARTESIAN_POINT ( 'NONE',  ( 763.0537975583476964, -0.4527844766023629286, -371.0346526505628617 ) ) ;
#35823=CARTESIAN_POINT ( 'NONE',  ( 781.8018195045266339, -358.2709662947829088, -365.1927285166406705 ) ) ;
#35827=CARTESIAN_POINT ( 'NONE',  ( 796.1575198192839480, -270.0090635724253048, -359.4546378042384163 ) ) ;
#35831=DIRECTION ( 'NONE',  ( -0.000000000000000000, 1.000000000000000000, -0.000000000000000000 ) ) ;
#35838=CARTESIAN_POINT ( 'NONE',  ( 763.2262854647970016, -104.6346026584202207, -309.2812353651462445 ) ) ;
#35839=CARTESIAN_POINT ( 'NONE',  ( 757.8323909638827445, -266.6346026584197375, -352.1044303154654358 ) ) ;
#35844=CARTESIAN_POINT ( 'NONE',  ( 773.7305795820266212, -57.28179084515326736, -374.8230680027170365 ) ) ;
#35845=CARTESIAN_POINT ( 'NONE',  ( 772.3691319403857278, -95.26014174441461080, -315.8894580844506663 ) ) ;
#35848=CARTESIAN_POINT ( 'NONE',  ( 778.1981804954714335, 13.72903370521577138, -314.8072714833589885 ) ) ;
#35849=CARTESIAN_POINT ( 'NONE',  ( 773.3843516231979720, -109.4419599262327836, -364.4086373105754433 ) ) ;
#35851=CARTESIAN_POINT ( 'NONE',  ( 805.1927285166397041, -88.81642084023842187, -341.8018195045277707 ) ) ;
#35852=CARTESIAN_POINT ( 'NONE',  ( 772.3691319403857278, -407.2601417444137155, -315.8894580844506663 ) ) ;
#35855=CARTESIAN_POINT ( 'NONE',  ( 766.5853460496234675, -397.9874144716864066, -372.3518521366060554 ) ) ;
#35861=CARTESIAN_POINT ( 'NONE',  ( 751.6929314249748586, -246.9982390220560546, -318.8095938919659034 ) ) ;
#35865=CARTESIAN_POINT ( 'NONE',  ( 804.8461984189677878, -74.19088175424410281, -336.9566956441385628 ) ) ;
#35867=CARTESIAN_POINT ( 'NONE',  ( 803.4237431249931660, -231.1800572038743553, -331.2633955100225194 ) ) ;
#35869=CARTESIAN_POINT ( 'NONE',  ( 756.5762568750052424, -411.1800572038738437, -348.7366044899774238 ) ) ;
#35870=CARTESIAN_POINT ( 'NONE',  ( 797.8594530101008786, -37.54369356751132614, -322.1405469898980982 ) ) ;
#35876=CARTESIAN_POINT ( 'NONE',  ( 800.2193346964447755, -18.99823902205683979, -355.1360043628815788 ) ) ;
#35880=CARTESIAN_POINT ( 'NONE',  ( 812.3518521366052028, -313.0999726633342561, -326.5853460496235243 ) ) ;
#35883=CARTESIAN_POINT ( 'NONE',  ( 781.8018195045266339, -262.2709662947831930, -365.1927285166406705 ) ) ;
#35885=CARTESIAN_POINT ( 'NONE',  ( 799.2566176426618085, -120.0090635724258021, -324.0069404352559559 ) ) ;
#35888=CARTESIAN_POINT ( 'NONE',  ( 814.2001403089898304, -329.3618753856922581, -347.4397851343538264 ) ) ;
#35889=PLANE ( 'NONE',  #12116 ) ;
#35892=CARTESIAN_POINT ( 'NONE',  ( 752.4576283171824116, -189.0783235625961822, -317.7880784355627952 ) ) ;
#35894=CARTESIAN_POINT ( 'NONE',  ( 776.2046728542105711, 3.809118245755632959, -304.8212110874238761 ) ) ;
#35901=CARTESIAN_POINT ( 'NONE',  ( 805.1016975059191054, 17.10349461922139369, -343.0745993439771837 ) ) ;
#35902=DIRECTION ( 'NONE',  ( -0.000000000000000000, 1.000000000000000000, 0.000000000000000000 ) ) ;
#35906=EDGE_LOOP ( 'NONE', ( #29541, #29983 ) ) ;
#35908=CARTESIAN_POINT ( 'NONE',  ( 798.7617431975189675, -291.6237781080503169, -323.0428371773161871 ) ) ;
#35909=CARTESIAN_POINT ( 'NONE',  ( 754.0944755984390895, -303.6237781080503169, -364.1009440267246760 ) ) ;
#35915=CARTESIAN_POINT ( 'NONE',  ( 754.9735926884551418, -90.35105083532373271, -340.5236548041000333 ) ) ;
#35918=CARTESIAN_POINT ( 'NONE',  ( 812.7932403749906598, -135.1800572038746679, -327.7687537140311633 ) ) ;
#35920=CARTESIAN_POINT ( 'NONE',  ( 800.2193346964446619, -138.9982390220564241, -355.1360043628816925 ) ) ;
#35922=AXIS2_PLACEMENT_3D ( 'NONE', #35530, #24676, #32317 ) ;
#35923=CARTESIAN_POINT ( 'NONE',  ( 763.8424801807145741, -426.0090635724247932, -320.5453621957614700 ) ) ;
#35931=CARTESIAN_POINT ( 'NONE',  ( 773.4516893846965786, -379.6454272087886466, -315.8398074228977066 ) ) ;
#35933=CARTESIAN_POINT ( 'NONE',  ( 745.7194118038753459, -181.6454272087892434, -348.7631598425976449 ) ) ;
#35936=LINE ( 'NONE', #4305, #40373 ) ;
#35938=CARTESIAN_POINT ( 'NONE',  ( 780.5290396650775619, -324.3510508353229511, -365.2837595273619513 ) ) ;
#35940=CARTESIAN_POINT ( 'NONE',  ( 745.5313806188320314, -183.2817908451528695, -333.7943932421247268 ) ) ;
#35947=CARTESIAN_POINT ( 'NONE',  ( 745.4481719005789273, -195.7255117493290015, -347.5162901302853697 ) ) ;
#35949=CARTESIAN_POINT ( 'NONE',  ( 765.0180583372156207, -0.9982390220569063999, -360.0135310231089534 ) ) ;
#35951=CARTESIAN_POINT ( 'NONE',  ( 768.8385539511368734, -95.26014174441461080, -306.4236121716840557 ) ) ;
#35953=CARTESIAN_POINT ( 'NONE',  ( 808.0189434323515343, -350.0891481129648923, -319.0252816721025511 ) ) ;
#35954=LINE ( 'NONE', #21409, #29117 ) ;
#35958=CARTESIAN_POINT ( 'NONE',  ( 810.1134526219336749, -416.5328690171409107, -357.8822607201570349 ) ) ;
#35959=CARTESIAN_POINT ( 'NONE',  ( 808.0189434323515343, -422.0891481129647218, -319.0252816721025511 ) ) ;
#35963=AXIS2_PLACEMENT_3D ( 'NONE', #20697, #24854, #28308 ) ;
#35965=CARTESIAN_POINT ( 'NONE',  ( 800.7704444035546203, -196.1692326535052473, -326.0291762391768771 ) ) ;
#35967=CARTESIAN_POINT ( 'NONE',  ( 812.6845335610512393, -175.9874144716871172, -353.5525998758768651 ) ) ;
#35971=AXIS2_PLACEMENT_3D ( 'NONE', #43065, #32677, #21368 ) ;
#35973=CARTESIAN_POINT ( 'NONE',  ( 781.8018195045266339, -142.2709662947837330, -365.1927285166406705 ) ) ;
#35976=CARTESIAN_POINT ( 'NONE',  ( 745.4481719005789273, -51.72551174932946338, -347.5162901302853129 ) ) ;
#35978=CARTESIAN_POINT ( 'NONE',  ( 805.6418435158337843, -461.4636090269701754, -363.8556311672236916 ) ) ;
#35983=CARTESIAN_POINT ( 'NONE',  ( 768.0187753319979720, -296.6346026584195670, -318.0580252608186242 ) ) ;
#35987=CARTESIAN_POINT ( 'NONE',  ( 804.6971507214547046, -291.2817908451525000, -344.0799538623459739 ) ) ;
#35988=CARTESIAN_POINT ( 'NONE',  ( 762.3223304703356007, -271.5436935675106156, -322.3223304703362828 ) ) ;
#35990=CARTESIAN_POINT ( 'NONE',  ( 755.3201227861273992, -123.7255117493292147, -345.3687786644892981 ) ) ;
#35993=ORIENTED_EDGE ( 'NONE', *, *, #24982, .F. ) ;
#35998=CARTESIAN_POINT ( 'NONE',  ( 791.0478386215596629, -93.82724539060770041, -306.7653713866226326 ) ) ;
#35999=LINE ( 'NONE', #33001, #30747 ) ;
#36005=CARTESIAN_POINT ( 'NONE',  ( 782.5225473063383106, -118.2709662947838041, -375.2698199232970637 ) ) ;
#36008=CYLINDRICAL_SURFACE ( 'NONE', #3486, 30.00000000000008171 ) ;
#36010=CARTESIAN_POINT ( 'NONE',  ( 814.5518280994195948, -231.7255117493288310, -332.4837098697145734 ) ) ;
#36012=CARTESIAN_POINT ( 'NONE',  ( 759.9999999999992042, -512.9681489794448908, -370.0000000000000000 ) ) ;
#36013=CARTESIAN_POINT ( 'NONE',  ( 752.4576283171824116, -309.0783235625957559, -317.7880784355627952 ) ) ;
#36016=CARTESIAN_POINT ( 'NONE',  ( 812.7932403749906598, -327.1800572038741279, -327.7687537140311633 ) ) ;
#36021=CARTESIAN_POINT ( 'NONE',  ( 755.5713283507202505, -413.3618753856920307, -334.6858677611754729 ) ) ;
#36022=EDGE_CURVE ( 'NONE', #39264, #11556, #35555, .T. ) ;
#36024=CARTESIAN_POINT ( 'NONE',  ( 805.9055244015594326, -75.62377810805104161, -315.8990559732753240 ) ) ;
#36029=CARTESIAN_POINT ( 'NONE',  ( 794.1144889064781864, -250.1692326535050199, -360.9840315886528401 ) ) ;
#36033=CARTESIAN_POINT ( 'NONE',  ( 754.0944755984390895, -39.62377810805116951, -364.1009440267246760 ) ) ;
#36037=CARTESIAN_POINT ( 'NONE',  ( 762.1177392798416577, -330.5545181178796952, -309.8865473780659272 ) ) ;
#36041=CARTESIAN_POINT ( 'NONE',  ( 766.0291762391763086, -178.9181544815165239, -360.7704444035551319 ) ) ;
#36042=CARTESIAN_POINT ( 'NONE',  ( 765.0180583372156207, -192.9982390220562820, -360.0135310231089534 ) ) ;
#36043=CARTESIAN_POINT ( 'NONE',  ( 764.8639956371174549, -368.0891481129647786, -319.7806653035542581 ) ) ;
#36045=CARTESIAN_POINT ( 'NONE',  ( 790.8726784830453198, 13.28531280103958423, -362.5472867521010585 ) ) ;
#36054=CARTESIAN_POINT ( 'NONE',  ( 804.1009440267234822, -407.4636090269703459, -314.0944755984392600 ) ) ;
#36055=CARTESIAN_POINT ( 'NONE',  ( 772.4837098697145166, 0.6381246143067237364, -374.5518280994205611 ) ) ;
#36058=CARTESIAN_POINT ( 'NONE',  ( 792.1044303154645831, -372.4527844766010958, -317.8323909638837677 ) ) ;
#36061=CARTESIAN_POINT ( 'NONE',  ( 802.9823548866075953, -265.0999726633344267, -330.0799878456151077 ) ) ;
#36066=CIRCLE ( 'NONE', #5792, 10.00000000000000888 ) ;
#36071=CARTESIAN_POINT ( 'NONE',  ( 797.8594530101008786, -325.5436935675105019, -322.1405469898980982 ) ) ;
#36075=CARTESIAN_POINT ( 'NONE',  ( 813.5763878283155464, -51.82724539060782121, -351.1614460488615350 ) ) ;
#36076=CARTESIAN_POINT ( 'NONE',  ( 804.1601925771018387, -103.4419599262327836, -346.5483106153029098 ) ) ;
#36079=CARTESIAN_POINT ( 'NONE',  ( 762.3223304703356007, -7.543693567511430942, -322.3223304703362828 ) ) ;
#36080=CARTESIAN_POINT ( 'NONE',  ( 779.4709603349208464, -144.3510508353235764, -314.7162404726379918 ) ) ;
#36082=CARTESIAN_POINT ( 'NONE',  ( 781.8018195045266339, -94.27096629478386092, -365.1927285166406705 ) ) ;
#36084=CARTESIAN_POINT ( 'NONE',  ( 761.2382568024794409, -399.6237781080500326, -356.9571628226838129 ) ) ;
#36088=ORIENTED_EDGE ( 'NONE', *, *, #12264, .T. ) ;
#36090=ORIENTED_EDGE ( 'NONE', *, *, #20725, .T. ) ;
#36095=CARTESIAN_POINT ( 'NONE',  ( 760.7433823573367135, -84.00906357242590161, -355.9930595647440441 ) ) ;
#36097=CARTESIAN_POINT ( 'NONE',  ( 795.1360043628808398, -260.0891481129650629, -360.2193346964456282 ) ) ;
#36100=CARTESIAN_POINT ( 'NONE',  ( 792.1044303154645831, -396.4527844766010389, -317.8323909638837677 ) ) ;
#36101=CARTESIAN_POINT ( 'NONE',  ( 802.1676090361156639, -38.63460265842041252, -327.8955696845344505 ) ) ;
#36104=DIRECTION ( 'NONE',  ( -1.000000000000000000, -0.000000000000000000, -0.000000000000000000 ) ) ;
#36105=CARTESIAN_POINT ( 'NONE',  ( 804.4286716492782716, -17.36187538569322086, -345.3141322388244703 ) ) ;
#36108=CARTESIAN_POINT ( 'NONE',  ( 799.9636004259356241, -310.9181544815160123, -311.2241431872006956 ) ) ;
#36111=CARTESIAN_POINT ( 'NONE',  ( 768.0187753319979720, -272.6346026584196807, -318.0580252608186242 ) ) ;
#36112=CARTESIAN_POINT ( 'NONE',  ( 773.4516893846965786, -139.6454272087893571, -315.8398074228977066 ) ) ;
#36115=CARTESIAN_POINT ( 'NONE',  ( 752.4576283171824116, -21.07832356259667250, -317.7880784355627952 ) ) ;
#36116=CARTESIAN_POINT ( 'NONE',  ( 804.7487373415286811, -355.5436935675103882, -364.7487373415288516 ) ) ;
#36120=CARTESIAN_POINT ( 'NONE',  ( 812.6845335610512393, -223.9874144716869182, -353.5525998758768651 ) ) ;
#36122=CARTESIAN_POINT ( 'NONE',  ( 782.4968714119720516, 13.18357915976123174, -305.0891759886411023 ) ) ;
#36129=CARTESIAN_POINT ( 'NONE',  ( 800.0135310231082713, -446.0891481129646081, -325.0180583372163028 ) ) ;
#36136=CARTESIAN_POINT ( 'NONE',  ( 754.8983024940795303, -306.8965053807775689, -336.9254006560228163 ) ) ;
#36138=CARTESIAN_POINT ( 'NONE',  ( 810.1134526219336749, -344.5328690171410813, -357.8822607201570349 ) ) ;
#36143=CARTESIAN_POINT ( 'NONE',  ( 757.2208543904082489, -64.71468719896019195, -350.9844846989624330 ) ) ;
#36145=CARTESIAN_POINT ( 'NONE',  ( 782.4968714119720516, -130.8164208402383224, -305.0891759886411023 ) ) ;
#36147=CARTESIAN_POINT ( 'NONE',  ( 802.1676090361155502, -158.6346026584200217, -327.8955696845344505 ) ) ;
#36149=CARTESIAN_POINT ( 'NONE',  ( 801.5560724626406000, -432.5545181178793541, -326.7756240680316182 ) ) ;
#36157=CARTESIAN_POINT ( 'NONE',  ( 793.9708237608222134, -406.9181544815157849, -319.2295555964448681 ) ) ;
#36159=CARTESIAN_POINT ( 'NONE',  ( 748.6759233522253680, -208.3726999360619061, -324.3348316497537098 ) ) ;
#36163=CARTESIAN_POINT ( 'NONE',  ( 779.4709603349208464, -312.3510508353230080, -314.7162404726379918 ) ) ;
#36166=CARTESIAN_POINT ( 'NONE',  ( 809.0717654672305343, -196.9181544815164386, -360.1688906516309885 ) ) ;
#36171=CARTESIAN_POINT ( 'NONE',  ( 796.7737145352015204, -236.6346026584198228, -370.7187646348536987 ) ) ;
#36173=CARTESIAN_POINT ( 'NONE',  ( 755.0636971347428243, -4.270966294784170003, -341.7834795799807353 ) ) ;
#36175=CARTESIAN_POINT ( 'NONE',  ( 805.9055244015594326, -99.62377810805098477, -315.8990559732753240 ) ) ;
#36177=CARTESIAN_POINT ( 'NONE',  ( 755.2512626584698410, -391.5436935675101608, -315.2512626584710915 ) ) ;
#36182=CARTESIAN_POINT ( 'NONE',  ( 751.2241431872005251, -424.1692326535044799, -359.9636004259367610 ) ) ;
#36183=CARTESIAN_POINT ( 'NONE',  ( 805.6418435158337843, -5.463609026971610660, -363.8556311672236916 ) ) ;
#36187=CARTESIAN_POINT ( 'NONE',  ( 803.8651313633788504, -197.2601417444143124, -332.4468031744301015 ) ) ;
#36189=CARTESIAN_POINT ( 'NONE',  ( 773.7943932421234194, -191.8055962898689017, -305.5313806188329409 ) ) ;
#36193=CARTESIAN_POINT ( 'NONE',  ( 805.1927285166397041, -136.8164208402382371, -341.8018195045277707 ) ) ;
#36195=CARTESIAN_POINT ( 'NONE',  ( 758.8095938919642549, -32.08914811296588709, -311.6929314249763365 ) ) ;
#36198=CARTESIAN_POINT ( 'NONE',  ( 745.5313806188320314, -447.2817908451521021, -333.7943932421247268 ) ) ;
#36200=CARTESIAN_POINT ( 'NONE',  ( 757.4527132478984868, -304.3726999360615082, -329.1273215169538844 ) ) ;
#36205=CARTESIAN_POINT ( 'NONE',  ( 799.2566176426618085, -288.0090635724252479, -324.0069404352559559 ) ) ;
#36206=CARTESIAN_POINT ( 'NONE',  ( 759.7806653035534055, -270.9982390220561115, -324.8639956371180801 ) ) ;
#36208=CARTESIAN_POINT ( 'NONE',  ( 774.6858677611749044, -153.7255117493291721, -315.5713283507209894 ) ) ;
#36214=CARTESIAN_POINT ( 'NONE',  ( 812.3518521366052028, -97.09997266333496668, -326.5853460496235243 ) ) ;
#36221=CARTESIAN_POINT ( 'NONE',  ( 747.2067596250078623, -147.1800572038746395, -352.2312462859687230 ) ) ;
#36225=CARTESIAN_POINT ( 'NONE',  ( 772.5602148656447525, -249.7255117493288594, -305.7998596910095443 ) ) ;
#36230=CARTESIAN_POINT ( 'NONE',  ( 807.5423716828161105, -297.0783235625957559, -362.2119215644372048 ) ) ;
#36232=CARTESIAN_POINT ( 'NONE',  ( 796.7737145352015204, -356.6346026584193964, -370.7187646348536987 ) ) ;
#36235=VERTEX_POINT ( 'NONE', #2717 ) ;
#36236=CARTESIAN_POINT ( 'NONE',  ( 804.6798772138708955, -423.7255117493281205, -334.6312213355107019 ) ) ;
#36237=CARTESIAN_POINT ( 'NONE',  ( 774.6858677611749044, -225.7255117493289163, -315.5713283507209894 ) ) ;
#36238=CARTESIAN_POINT ( 'NONE',  ( 803.8556311672234642, -81.62377810805104161, -365.6418435158340117 ) ) ;
#36244=CARTESIAN_POINT ( 'NONE',  ( 772.3691319403857278, -239.2601417444141987, -315.8894580844506663 ) ) ;
#36247=CARTESIAN_POINT ( 'NONE',  ( 746.0683387631852383, -67.44195992623289726, -331.3260364891676204 ) ) ;
#36249=CARTESIAN_POINT ( 'NONE',  ( 809.0082352070306797, -452.9681489794448908, -335.5949598064873385 ) ) ;
#36251=CARTESIAN_POINT ( 'NONE',  ( 814.2805881961230625, -337.6454272087888171, -331.2368401574024119 ) ) ;
#36254=CARTESIAN_POINT ( 'NONE',  ( 804.4086373105744769, -169.6454272087892718, -333.3843516231986541 ) ) ;
#36255=CARTESIAN_POINT ( 'NONE',  ( 774.6858677611749044, -177.7255117493290868, -315.5713283507209894 ) ) ;
#36256=VECTOR ( 'NONE', #9972, 1000.000000000000000 ) ;
#36257=CARTESIAN_POINT ( 'NONE',  ( 797.8594530101009923, -373.5436935675102177, -322.1405469898982119 ) ) ;
#36259=CARTESIAN_POINT ( 'NONE',  ( 802.7791456095903868, 19.28531280103956647, -329.0155153010375102 ) ) ;
#36260=ORIENTED_EDGE ( 'NONE', *, *, #2706, .T. ) ;
#36272=CARTESIAN_POINT ( 'NONE',  ( 805.6418435158337843, -413.4636090269704027, -363.8556311672236916 ) ) ;
#36273=CARTESIAN_POINT ( 'NONE',  ( 777.5031285880264704, 1.183579159761269040, -374.9108240113588408 ) ) ;
#36276=CARTESIAN_POINT ( 'NONE',  ( 781.8018195045266339, -406.2709662947829088, -365.1927285166406705 ) ) ;
#36280=CARTESIAN_POINT ( 'NONE',  ( 786.5483106153019435, -247.6454272087890160, -364.1601925771022366 ) ) ;
#36289=CARTESIAN_POINT ( 'NONE',  ( 788.8264449731200330, -309.1800572038740711, -363.6646147819171233 ) ) ;
#36293=CARTESIAN_POINT ( 'NONE',  ( 814.8207195650702488, -74.19088175424410281, -336.2433038121456548 ) ) ;
#36294=CARTESIAN_POINT ( 'NONE',  ( 754.9735926884551418, -114.3510508353236617, -340.5236548041000333 ) ) ;
#36298=CARTESIAN_POINT ( 'NONE',  ( 767.8955696845333705, -24.45278447660229304, -362.1676090361162323 ) ) ;
#36299=CARTESIAN_POINT ( 'NONE',  ( 772.3691319403857278, -143.2601417444144829, -315.8894580844506663 ) ) ;
#36300=CARTESIAN_POINT ( 'NONE',  ( 785.3141322388236176, -93.72551174932934259, -364.4286716492789537 ) ) ;
#36301=CARTESIAN_POINT ( 'NONE',  ( 754.9735926884551418, -426.3510508353226669, -340.5236548041000333 ) ) ;
#36305=ORIENTED_EDGE ( 'NONE', *, *, #24982, .T. ) ;
#36311=CARTESIAN_POINT ( 'NONE',  ( 772.4468031744293057, -81.82724539060772884, -363.8651313633793620 ) ) ;
#36314=CARTESIAN_POINT ( 'NONE',  ( 805.1927285166399315, -280.8164208402378108, -341.8018195045277707 ) ) ;
#36316=CARTESIAN_POINT ( 'NONE',  ( 762.1405469898971887, -385.5436935675102745, -357.8594530101015607 ) ) ;
#36317=CARTESIAN_POINT ( 'NONE',  ( 804.6798772138708955, -63.72551174932939233, -334.6312213355107019 ) ) ;
#36320=DIRECTION ( 'NONE',  ( -0.000000000000000000, 1.000000000000000000, -0.000000000000000000 ) ) ;
#36323=CARTESIAN_POINT ( 'NONE',  ( 810.4231160770870019, -24.55451811788064020, -321.9338519418446936 ) ) ;
#36326=CARTESIAN_POINT ( 'NONE',  ( 776.2046728542105711, -308.1908817542434349, -304.8212110874238761 ) ) ;
#36330=CARTESIAN_POINT ( 'NONE',  ( 792.1044303154645831, -252.4527844766015789, -317.8323909638837677 ) ) ;
#36331=CARTESIAN_POINT ( 'NONE',  ( 772.4999999999993179, -462.9681489794448339, -370.0000000000000568 ) ) ;
#36332=CARTESIAN_POINT ( 'NONE',  ( 798.5707757039680246, -149.4636090269711417, -356.7845633553585003 ) ) ;
#36335=CARTESIAN_POINT ( 'NONE',  ( 788.7631598425961101, -25.44195992623301450, -305.7194118038759143 ) ) ;
#36336=CARTESIAN_POINT ( 'NONE',  ( 796.7737145352015204, -356.6346026584193964, -370.7187646348536987 ) ) ;
#36340=CARTESIAN_POINT ( 'NONE',  ( 756.1443688327750579, -237.6237781080505442, -314.3581564841659315 ) ) ;
#36342=CARTESIAN_POINT ( 'NONE',  ( 795.6651683502461765, -442.7146871989589840, -371.3240766477733814 ) ) ;
#36348=CARTESIAN_POINT ( 'NONE',  ( 796.7845633553578182, -9.623778108051251223, -358.5707757039688204 ) ) ;
#36349=FACE_BOUND ( 'NONE', #12842, .T. ) ;
#36355=CARTESIAN_POINT ( 'NONE',  ( 804.9511171171677688, -341.8055962898683333, -335.8780910478229202 ) ) ;
#36357=CARTESIAN_POINT ( 'NONE',  ( 776.2433038121456548, -324.8965053807775121, -374.8207195650711014 ) ) ;
#36362=CARTESIAN_POINT ( 'NONE',  ( 759.2295555964440155, -64.16923265350563099, -353.9708237608231229 ) ) ;
#36365=CARTESIAN_POINT ( 'NONE',  ( 747.2067596250078623, -195.1800572038744974, -352.2312462859687230 ) ) ;
#36367=CARTESIAN_POINT ( 'NONE',  ( 804.4286716492782716, -185.3618753856926844, -345.3141322388244703 ) ) ;
#36368=ORIENTED_EDGE ( 'NONE', *, *, #27299, .F. ) ;
#36369=CARTESIAN_POINT ( 'NONE',  ( 773.4516893846965786, -427.6454272087885897, -315.8398074228977066 ) ) ;
#36376=CARTESIAN_POINT ( 'NONE',  ( 790.0220218866281812, -415.0999726633340288, -363.2186876482849129 ) ) ;
#36379=CARTESIAN_POINT ( 'NONE',  ( 746.4236121716829757, -207.8272453906073451, -328.8385539511384650 ) ) ;
#36383=CARTESIAN_POINT ( 'NONE',  ( 805.1016975059191054, -318.8965053807775121, -343.0745993439771837 ) ) ;
#36385=CARTESIAN_POINT ( 'NONE',  ( 814.4686193811664907, -171.2817908451529263, -346.2056067578752732 ) ) ;
#36386=DIRECTION ( 'NONE',  ( 0.000000000000000000, 0.000000000000000000, 1.000000000000000000 ) ) ;
#36389=CARTESIAN_POINT ( 'NONE',  ( 814.9108240113580450, -256.2709662947834204, -337.5031285880265273 ) ) ;
#36392=CARTESIAN_POINT ( 'NONE',  ( 759.7806653035534055, -6.998239022056885972, -324.8639956371180801 ) ) ;
#36395=CARTESIAN_POINT ( 'NONE',  ( 756.1443688327750579, -117.6237781080509279, -314.3581564841659315 ) ) ;
#36397=CARTESIAN_POINT ( 'NONE',  ( 782.5225473063381969, -382.2709662947828519, -375.2698199232970637 ) ) ;
#36402=CARTESIAN_POINT ( 'NONE',  ( 778.2165204200184689, -382.8164208402374697, -364.9363028652563230 ) ) ;
#36403=CARTESIAN_POINT ( 'NONE',  ( 810.4231160770870019, -0.5545181178807169209, -321.9338519418446936 ) ) ;
#36408=CARTESIAN_POINT ( 'NONE',  ( 787.6308680596127942, -179.2601417444143692, -364.1105419155492768 ) ) ;
#36411=CARTESIAN_POINT ( 'NONE',  ( 749.8865473780648472, -212.5328690171415076, -322.1177392798429082 ) ) ;
#36418=CARTESIAN_POINT ( 'NONE',  ( 804.7487373415286811, -91.54369356751116982, -364.7487373415288516 ) ) ;
#36420=CARTESIAN_POINT ( 'NONE',  ( 755.8894580844503253, -15.82724539060794200, -332.3691319403863531 ) ) ;
#36422=CARTESIAN_POINT ( 'NONE',  ( 769.9779781133707957, -331.0999726633342561, -316.7813123517150871 ) ) ;
#36426=CARTESIAN_POINT ( 'NONE',  ( 802.1676090361156639, -302.6346026584196238, -327.8955696845344505 ) ) ;
#36429=CARTESIAN_POINT ( 'NONE',  ( 755.1538015810308480, -302.1908817542433781, -343.0433043558613804 ) ) ;
#36430=CARTESIAN_POINT ( 'NONE',  ( 778.1981804954714335, -298.2709662947830793, -314.8072714833589885 ) ) ;
#36432=CARTESIAN_POINT ( 'NONE',  ( 756.3353852180819104, -149.9073299311473875, -331.1735550268788302 ) ) ;
#36438=CARTESIAN_POINT ( 'NONE',  ( 795.8262568251477660, -94.37269993606224716, -308.3538107759623585 ) ) ;
#36444=AXIS2_PLACEMENT_3D ( 'NONE', #12812, #23429, #26893 ) ;
#36446=CARTESIAN_POINT ( 'NONE',  ( 746.8695393053151292, -125.9073299311474159, -327.6429770376306578 ) ) ;
#36449=CARTESIAN_POINT ( 'NONE',  ( 805.1016975059191054, -438.8965053807771710, -343.0745993439771837 ) ) ;
#36451=CARTESIAN_POINT ( 'NONE',  ( 782.4968714119720516, -274.8164208402378108, -305.0891759886411023 ) ) ;
#36455=CARTESIAN_POINT ( 'NONE',  ( 793.4146539503750546, -25.98741447168755769, -307.6481478633938877 ) ) ;
#36457=CARTESIAN_POINT ( 'NONE',  ( 786.2056067578752163, -299.8055962898685038, -374.4686193811670023 ) ) ;
#36460=CARTESIAN_POINT ( 'NONE',  ( 815.2698199232961542, -352.8164208402374129, -342.5225473063383106 ) ) ;
#36464=CARTESIAN_POINT ( 'NONE',  ( 797.8594530101008786, -421.5436935675101040, -322.1405469898980982 ) ) ;
#36466=CARTESIAN_POINT ( 'NONE',  ( 813.9316612368132837, -127.4419599262326983, -348.6739635108323228 ) ) ;
#36470=CARTESIAN_POINT ( 'NONE',  ( 790.8726784830453198, -226.7146871989596661, -362.5472867521010585 ) ) ;
#36472=CARTESIAN_POINT ( 'NONE',  ( 813.9316612368132837, -55.44195992623293989, -348.6739635108323228 ) ) ;
#36475=ORIENTED_EDGE ( 'NONE', *, *, #4371, .T. ) ;
#36477=CARTESIAN_POINT ( 'NONE',  ( 746.4236121716829757, -351.8272453906068336, -328.8385539511384650 ) ) ;
#36481=CARTESIAN_POINT ( 'NONE',  ( 801.5560724626406000, -192.5545181178801215, -326.7756240680316182 ) ) ;
#36482=CARTESIAN_POINT ( 'NONE',  ( 762.3223304703356007, -199.5436935675108430, -322.3223304703362828 ) ) ;
#36483=CARTESIAN_POINT ( 'NONE',  ( 768.0187753319979720, -392.6346026584193396, -318.0580252608186242 ) ) ;
#36488=PLANE ( 'NONE',  #7868 ) ;
#36491=AXIS2_PLACEMENT_3D ( 'NONE', #16526, #37074, #5212 ) ;
#36495=CARTESIAN_POINT ( 'NONE',  ( 814.2805881961230625, -409.6454272087884760, -331.2368401574024119 ) ) ;
#36496=CARTESIAN_POINT ( 'NONE',  ( 747.2067596250078623, -51.18005720387493085, -352.2312462859687230 ) ) ;
#36498=CARTESIAN_POINT ( 'NONE',  ( 762.1405469898971887, -385.5436935675102745, -357.8594530101015607 ) ) ;
#36499=CARTESIAN_POINT ( 'NONE',  ( 781.7834795799800531, -10.81642084023869543, -315.0636971347436202 ) ) ;
#36502=CARTESIAN_POINT ( 'NONE',  ( 800.9840315886518738, -244.9181544815162681, -354.1144889064786412 ) ) ;
#36503=CARTESIAN_POINT ( 'NONE',  ( 745.7998596910086917, -173.3618753856927128, -332.5602148656461168 ) ) ;
#36504=CLOSED_SHELL ( 'NONE', ( #39160, #5482, #24160, #19526, #16564, #38233, #5547, #5542, #14601, #15411, #20664, #31994, #21588, #38900, #28990, #24634, #29796, #45360, #1508, #6627, #4907, #105, #22445, #3109, #9067, #15961, #9149, #5720, #23807, #45578, #10783, #15618, #10901, #28070, #4610, #1831, #18431, #18765, #17403, #44942, #11095, #30957, #16541, #4782, #13693, #2382, #40701, #33390, #12597, #5963 ) ) ;
#36515=CARTESIAN_POINT ( 'NONE',  ( 800.0135310231082713, -302.0891481129650629, -325.0180583372163028 ) ) ;
#36518=CARTESIAN_POINT ( 'NONE',  ( 748.6759233522253680, -64.37269993606231822, -324.3348316497537098 ) ) ;
#36519=CARTESIAN_POINT ( 'NONE',  ( 755.0488828828309806, -113.8055962898691149, -344.1219089521771934 ) ) ;
#36524=CARTESIAN_POINT ( 'NONE',  ( 778.2165204200184689, -22.81642084023865280, -364.9363028652563230 ) ) ;
#36525=CARTESIAN_POINT ( 'NONE',  ( 795.9930595647434757, -123.0783235625963385, -320.7433823573372820 ) ) ;
#36526=CARTESIAN_POINT ( 'NONE',  ( 800.0135310231082713, -134.0891481129655745, -325.0180583372163028 ) ) ;
#36528=VECTOR ( 'NONE', #9992, 1000.000000000000000 ) ;
#36531=CARTESIAN_POINT ( 'NONE',  ( 769.1273215169530886, -430.7146871989590409, -317.4527132478988847 ) ) ;
#36542=ORIENTED_EDGE ( 'NONE', *, *, #2975, .F. ) ;
#36543=CARTESIAN_POINT ( 'NONE',  ( 786.5483106153019435, -79.64542720878957027, -364.1601925771022366 ) ) ;
#36545=CARTESIAN_POINT ( 'NONE',  ( 764.8639956371174549, -272.0891481129651197, -319.7806653035542581 ) ) ;
#36548=CARTESIAN_POINT ( 'NONE',  ( 803.4237431249931660, -399.1800572038738437, -331.2633955100225194 ) ) ;
#36549=CARTESIAN_POINT ( 'NONE',  ( 755.0636971347428243, -52.27096629478401724, -341.7834795799807353 ) ) ;
#36552=FACE_OUTER_BOUND ( 'NONE', #26433, .T. ) ;
#36554=CARTESIAN_POINT ( 'NONE',  ( 752.7379699480933368, -12.00906357242613609, -361.9858362298580232 ) ) ;
#36557=CARTESIAN_POINT ( 'NONE',  ( 811.3240766477731540, -292.3726999360616219, -355.6651683502462902 ) ) ;
#36562=CARTESIAN_POINT ( 'NONE',  ( 802.1676090361156639, -302.6346026584196238, -327.8955696845344505 ) ) ;
#36565=CARTESIAN_POINT ( 'NONE',  ( 757.4527132478984868, -160.3726999360620482, -329.1273215169538844 ) ) ;
#36569=CARTESIAN_POINT ( 'NONE',  ( 807.5423716828161105, -9.078323562596708030, -362.2119215644372048 ) ) ;
#36570=CARTESIAN_POINT ( 'NONE',  ( 814.2001403089898304, -353.3618753856922012, -347.4397851343538264 ) ) ;
#36574=CARTESIAN_POINT ( 'NONE',  ( 807.5423716828161105, -249.0783235625959549, -362.2119215644372048 ) ) ;
#36576=CARTESIAN_POINT ( 'NONE',  ( 788.7631598425961101, -433.4419599262316183, -305.7194118038759143 ) ) ;
#36581=CARTESIAN_POINT ( 'NONE',  ( 804.1601925771018387, -31.44195992623299674, -346.5483106153029098 ) ) ;
#36589=EDGE_CURVE ( 'NONE', #30631, #21713, #4359, .T. ) ;
#36590=CARTESIAN_POINT ( 'NONE',  ( 789.9200121543843807, -337.9874144716865771, -317.0176451133914384 ) ) ;
#36593=CARTESIAN_POINT ( 'NONE',  ( 788.7631598425961101, -337.4419599262319593, -305.7194118038759143 ) ) ;
#36599=CARTESIAN_POINT ( 'NONE',  ( 802.7791456095903868, -76.71468719896012090, -329.0155153010375102 ) ) ;
#36603=CARTESIAN_POINT ( 'NONE',  ( 787.4397851343537695, -165.7255117493291152, -374.2001403089903988 ) ) ;
#36606=CARTESIAN_POINT ( 'NONE',  ( 795.1360043628808398, -188.0891481129653755, -360.2193346964456282 ) ) ;
#36608=CARTESIAN_POINT ( 'NONE',  ( 780.5236548040995785, -428.7363362996975980, -314.9735926884559944 ) ) ;
#36615=CARTESIAN_POINT ( 'NONE',  ( 769.9779781133707957, -427.0999726633338582, -316.7813123517150871 ) ) ;
#36616=CARTESIAN_POINT ( 'NONE',  ( 759.9999999999992042, -512.9681489794448908, -339.9999999999999432 ) ) ;
#36617=CARTESIAN_POINT ( 'NONE',  ( 762.1177392798416577, -210.5545181178800647, -309.8865473780659272 ) ) ;
#36621=CARTESIAN_POINT ( 'NONE',  ( 788.7366044899766848, -203.9073299311471885, -316.5762568750059813 ) ) ;
#36622=CARTESIAN_POINT ( 'NONE',  ( 758.6633372737375112, -332.5328690171411381, -326.9102291470432533 ) ) ;
#36623=CARTESIAN_POINT ( 'NONE',  ( 779.9999999999992042, 166.4563064324884465, -339.9999999999999432 ) ) ;
#36624=CARTESIAN_POINT ( 'NONE',  ( 748.6759233522253680, -208.3726999360619061, -324.3348316497537098 ) ) ;
#36627=CARTESIAN_POINT ( 'NONE',  ( 779.4763451958990572, -32.73633629969879877, -365.0264073115438919 ) ) ;
#36628=AXIS2_PLACEMENT_3D ( 'NONE', #13728, #3565, #16732 ) ;
#36630=CARTESIAN_POINT ( 'NONE',  ( 787.5162901302840055, -227.3618753856925423, -305.4481719005793252 ) ) ;
#36633=CARTESIAN_POINT ( 'NONE',  ( 794.9819416627830151, -12.99823902205686821, -319.9864689768909898 ) ) ;
#36635=CARTESIAN_POINT ( 'NONE',  ( 771.2368401574024119, -133.4419599262326699, -374.2805881961240857 ) ) ;
#36637=CARTESIAN_POINT ( 'NONE',  ( 767.7687537140311633, -383.9073299311466485, -372.7932403749916830 ) ) ;
#36643=CARTESIAN_POINT ( 'NONE',  ( 771.1735550268778070, -393.1800572038737300, -316.3353852180827630 ) ) ;
#36644=CARTESIAN_POINT ( 'NONE',  ( 799.9636004259356241, 1.081845518482914104, -311.2241431872006956 ) ) ;
#36648=CARTESIAN_POINT ( 'NONE',  ( 775.9200461376533440, -215.8055962898687881, -315.3028492785443291 ) ) ;
#36650=CARTESIAN_POINT ( 'NONE',  ( 771.2368401574024119, -229.4419599262323572, -374.2805881961240857 ) ) ;
#36656=CARTESIAN_POINT ( 'NONE',  ( 815.2698199232961542, -64.81642084023852135, -342.5225473063383106 ) ) ;
#36657=CARTESIAN_POINT ( 'NONE',  ( 800.0135310231082713, -86.08914811296573077, -325.0180583372163028 ) ) ;
#36658=ORIENTED_EDGE ( 'NONE', *, *, #18785, .F. ) ;
#36659=CARTESIAN_POINT ( 'NONE',  ( 804.6971507214547046, -3.281790845153435221, -344.0799538623459739 ) ) ;
#36660=ORIENTED_EDGE ( 'NONE', *, *, #32638, .F. ) ;
#36661=CARTESIAN_POINT ( 'NONE',  ( 761.4292242960306112, -329.4636090269706870, -323.2154366446414429 ) ) ;
#36669=CARTESIAN_POINT ( 'NONE',  ( 805.2837595273609850, -314.7363362996979959, -340.5290396650784714 ) ) ;
#36670=CARTESIAN_POINT ( 'NONE',  ( 768.0187753319979720, -272.6346026584196807, -318.0580252608186242 ) ) ;
#36671=CARTESIAN_POINT ( 'NONE',  ( 754.8072714833581358, -148.8164208402382656, -338.1981804954720587 ) ) ;
#36675=CARTESIAN_POINT ( 'NONE',  ( 783.7953271457878373, -128.1908817542439465, -375.1787889125761239 ) ) ;
#36676=DIRECTION ( 'NONE',  ( 0.000000000000000000, 0.000000000000000000, 1.000000000000000000 ) ) ;
#36681=CARTESIAN_POINT ( 'NONE',  ( 811.0346526505617248, -134.6346026584201070, -323.0537975583478101 ) ) ;
#36684=CARTESIAN_POINT ( 'NONE',  ( 763.2262854647970016, -272.6346026584196807, -309.2812353651462445 ) ) ;
#36685=CARTESIAN_POINT ( 'NONE',  ( 745.4481719005789273, -435.7255117493282341, -347.5162901302853697 ) ) ;
#36688=CARTESIAN_POINT ( 'NONE',  ( 754.0944755984390895, -327.6237781080502600, -364.1009440267246760 ) ) ;
#36690=CARTESIAN_POINT ( 'NONE',  ( 804.7487373415286811, -91.54369356751116982, -364.7487373415288516 ) ) ;
#36692=CARTESIAN_POINT ( 'NONE',  ( 782.5225473063381969, -358.2709662947829088, -375.2698199232970637 ) ) ;
#36697=CARTESIAN_POINT ( 'NONE',  ( 776.2433038121456548, -108.8965053807782084, -374.8207195650711014 ) ) ;
#36702=CARTESIAN_POINT ( 'NONE',  ( 796.7845633553578182, -249.6237781080505158, -358.5707757039688204 ) ) ;
#36704=CARTESIAN_POINT ( 'NONE',  ( 800.9747183278959710, 11.00176097794305541, -311.9810565676471583 ) ) ;
#36705=CARTESIAN_POINT ( 'NONE',  ( 788.7631598425961101, -73.44195992623286884, -305.7194118038759143 ) ) ;
#36707=EDGE_LOOP ( 'NONE', ( #39637, #43203, #28103, #20412 ) ) ;
#36709=CARTESIAN_POINT ( 'NONE',  ( 788.6739635108323228, -391.6454272087885897, -373.9316612368139090 ) ) ;
#36712=CARTESIAN_POINT ( 'NONE',  ( 776.9254006560222479, -212.1908817542436623, -314.8983024940802125 ) ) ;
#36713=CARTESIAN_POINT ( 'NONE',  ( 788.7366044899766848, -179.9073299311472454, -316.5762568750059813 ) ) ;
#36714=CARTESIAN_POINT ( 'NONE',  ( 802.1676090361155502, -398.6346026584193396, -327.8955696845344505 ) ) ;
#36717=CARTESIAN_POINT ( 'NONE',  ( 776.9566956441375396, 11.10349461922141145, -364.8461984189686405 ) ) ;
#36728=CARTESIAN_POINT ( 'NONE',  ( 809.0717654672305343, -412.9181544815157281, -360.1688906516309885 ) ) ;
#36729=CARTESIAN_POINT ( 'NONE',  ( 808.3070685750232087, -18.99823902205684689, -361.1904061080339829 ) ) ;
#36731=CARTESIAN_POINT ( 'NONE',  ( 756.5762568750052424, -411.1800572038738437, -348.7366044899774238 ) ) ;
#36732=CARTESIAN_POINT ( 'NONE',  ( 781.8018195045267476, 1.729033705215812233, -365.1927285166407273 ) ) ;
#36735=CARTESIAN_POINT ( 'NONE',  ( 801.5560724626406000, -264.5545181178798657, -326.7756240680316182 ) ) ;
#36736=CARTESIAN_POINT ( 'NONE',  ( 755.2512626584698410, -151.5436935675109851, -315.2512626584710915 ) ) ;
#36739=CARTESIAN_POINT ( 'NONE',  ( 770.1068079863199500, 16.45630643248850333, -316.7980005127122922 ) ) ;
#36745=CARTESIAN_POINT ( 'NONE',  ( 804.4286716492782716, -329.3618753856922581, -345.3141322388244703 ) ) ;
#36747=CARTESIAN_POINT ( 'NONE',  ( 781.2370466360911223, -92.73633629969860692, -304.9990715423533629 ) ) ;
#36748=CARTESIAN_POINT ( 'NONE',  ( 795.9930595647434757, -123.0783235625963385, -320.7433823573372820 ) ) ;
#36753=CARTESIAN_POINT ( 'NONE',  ( 755.3201227861273992, -27.72551174932954510, -345.3687786644892981 ) ) ;
#36754=CARTESIAN_POINT ( 'NONE',  ( 761.2382568024794409, -135.6237781080508853, -356.9571628226838129 ) ) ;
#36755=CARTESIAN_POINT ( 'NONE',  ( 771.1735550268778070, -129.1800572038746111, -316.3353852180827630 ) ) ;
#36757=CARTESIAN_POINT ( 'NONE',  ( 794.1144889064781864, -442.1692326535044231, -360.9840315886528401 ) ) ;
#36763=CARTESIAN_POINT ( 'NONE',  ( 793.5525998758768083, -271.0999726633344267, -372.6845335610516941 ) ) ;
#36771=CARTESIAN_POINT ( 'NONE',  ( 790.9844846989617508, -70.37269993606230400, -317.2208543904092721 ) ) ;
#36772=CARTESIAN_POINT ( 'NONE',  ( 756.3353852180820240, -293.9073299311468759, -331.1735550268787733 ) ) ;
#36774=CARTESIAN_POINT ( 'NONE',  ( 759.7806653035534055, -390.9982390220557136, -324.8639956371180801 ) ) ;
#36775=CARTESIAN_POINT ( 'NONE',  ( 768.0187753319979720, -56.63460265842036279, -318.0580252608186242 ) ) ;
#36779=CARTESIAN_POINT ( 'NONE',  ( 764.1737431748507561, -10.37269993606250473, -371.6461892240376415 ) ) ;
#36782=CARTESIAN_POINT ( 'NONE',  ( 804.1009440267234822, -311.4636090269706870, -314.0944755984392600 ) ) ;
#36786=CARTESIAN_POINT ( 'NONE',  ( 759.7806653035534055, -294.9982390220560546, -324.8639956371180801 ) ) ;
#36788=CARTESIAN_POINT ( 'NONE',  ( 796.9571628226829034, -167.4636090269711133, -321.2382568024804641 ) ) ;
#36789=EDGE_CURVE ( 'NONE', #29612, #37323, #36066, .T. ) ;
#36791=CARTESIAN_POINT ( 'NONE',  ( 814.8230680027162407, -5.805596289869448867, -333.7305795820267917 ) ) ;
#36792=CARTESIAN_POINT ( 'NONE',  ( 811.0346526505617248, -350.6346026584193396, -323.0537975583478101 ) ) ;
#36797=CARTESIAN_POINT ( 'NONE',  ( 759.8311093483677041, -430.1692326535043094, -310.9282345327691814 ) ) ;
#36803=CARTESIAN_POINT ( 'NONE',  ( 779.4709603349208464, -0.3510508353240099355, -314.7162404726379918 ) ) ;
#36808=CARTESIAN_POINT ( 'NONE',  ( 797.6776695296629214, -43.54369356751131903, -357.6776695296636603 ) ) ;
#36809=CARTESIAN_POINT ( 'NONE',  ( 805.0264073115434940, -342.3510508353228943, -339.4763451958999099 ) ) ;
#36811=CARTESIAN_POINT ( 'NONE',  ( 795.6651683502461765, -346.7146871989592682, -371.3240766477733814 ) ) ;
#36819=CARTESIAN_POINT ( 'NONE',  ( 767.7687537140311633, -191.9073299311471885, -372.7932403749916830 ) ) ;
#36822=ORIENTED_EDGE ( 'NONE', *, *, #29910, .F. ) ;
#36823=CARTESIAN_POINT ( 'NONE',  ( 800.0135310231082713, -182.0891481129654323, -325.0180583372163028 ) ) ;
#36825=CARTESIAN_POINT ( 'NONE',  ( 779.4763451958990572, -440.7363362996975980, -365.0264073115438919 ) ) ;
#36826=( BOUNDED_SURFACE ( )  B_SPLINE_SURFACE ( 3, 2, ( 
 ( #25445, #32614, #39318, #3753, #28218, #35848, #3535, #39099, #39566, #32154, #7449, #24989, #28458, #24519, #24760, #21302, #42775, #10443, #17842, #32397, #7920, #42313, #747, #4224, #28697, #42557, #28921, #11136, #10677, #31909, #14379, #31687, #17619, #21524, #35601, #25207, #3977, #7673, #35155, #517, #18534, #21753, #42999, #11365, #36079, #4446, #956, #15061, #42092, #6988, #21073, #40003, #8808, #29597, #36968, #22419, #32841, #1414, #15517, #26118, #43675, #25892, #26351, #43455, #1192, #5322, #22655, #43898, #25682, #12491, #19649, #40455, #36524, #15299, #22876, #36298, #40232, #26568, #5109, #8589, #12046, #36753, #11603, #11822, #8353, #29817, #43232, #4883, #19416, #40666, #29384, #33507, #1855, #15728, #19197, #15963, #12276, #18986, #33077, #33284, #18753, #4655, #1629, #30045, #44126, #9020, #23090, #22205, #37190, #5556, #33742, #2092, #29148, #39794, #8142, #30737, #41824, #9492, #34656, #27041, #33958, #38131, #41582, #9937, #34871, #2310, #31183, #20099, #16651, #30489, #3015, #44594, #16181, #30262, #12711, #44831, #24009, #24246, #6700, #6482, #19881, #45278, #23555, #9263, #44354, #37657, #6006, #38355, #13191, #5795, #12954, #26790, #13637, #20778, #34174, #2546, #27272, #20561, #40895, #41363, #41139, #9711, #23774, #27484, #17102, #10169, #30964, #37888, #6239, #13415, #20328, #34422, #2790, #16882, #45058, #27720, #37435, #8475, #4554, #3476, #39906, #15193, #15416, #14323, #31857, #43355, #22546, #4775, #38820, #17324, #32971, #7174, #3235, #10391, #21011, #15923, #30007, #40636, #8776, #33704, #23057, #2054, #19384, #16148, #8989, #27002, #9223, #1815, #2275, #37617, #30231, #29781, #44322, #23297, #44555, #26757, #33470, #30451, #16374, #19611, #36937, #33924, #12914, #41098, #44094, #37157, #23516, #40423, #9453, #12459, #15696, #5970, #12677, #37399, #19842, #20060, #19168, #40862, #26318, #5753, #26538, #22844, #5515, #33252, #43856, #1598, #12239, #5291, #28808, #42887, #39444, #37318, #44473, #41471, #16533, #6369, #13074, #19767, #2672, #16767, #33626, #30848, #12609, #1977, #44944, #44249, #5676, #9378, #26685, #2207, #23444, #13300, #20451, #27376, #9824, #23893, #18428, #11937, #39908, #32508, #5014, #36193, #26004, #43128, #22315, #15196, #32974, #8038, #40576, #29281, #29939, #35973, #1317, #33398, #14957, #15419, #22549, #29043, #8714, #1744, #19105, #4557, #11496, #43359, #8249, #39691, #25576, #33192, #43785, #22104, #12166, #26249, #36875, #18647, #32737, #1082, #20460, #20224, #16306, #41480, #45173, #41256, #1984, #9612, #34311, #6379, #37785, #33860, #38023, #9833, #16542, #37325, #13308, #23902, #34548, #19776, #34076, #13533, #26693, #2907, #26919, #19536, #16998, #23673, #2681, #44952, #31074, #27608, #6133, #30166, #16777, #12838, #12615, #41024, #30857, #5441, #44721, #2213, #41715, #30625, #13084, #22992, #30389, #37551, #37085, #27385, #33632, #27168, #9384, #16082, #44256, #9147, #40789, #44481, #23216, #5685, #23451, #5909, #2439, #19999, #38251, #21146, #17216, #28765, #14455, #24142, #28064, #6596, #31755, #31544, #20674, #24829, #10288, #3607, #31303, #42158, #34995, #10510, #27850, #14689, #3371, #35674, #587, #7063, #39170, #34765, #38703, #124, #10071, #28533, #21594, #24586, #24363, #7520, #17462, #45647, #13772, #4050, #41947, #31979, #17694, #18148, #35228, #14214, #28283, #32227, #42383, #38466, #3127, #42628, #13996, #45410, #6819, #20897, #10752, #10990, #3821, #38949, #7299, #350, #21374, #35450, #17911, #25058, #1588, #19160, #5283, #15688, #12668, #19602, #9213, #5069, #8768, #8543, #29770, #22835, #19833, #2044, #1808, #12451, #23509, #36929, #16364, #33460, #43848, #33915, #23288, #37390, #22609, #26309, #15914, #29998, #26530, #8980, #44545, #23049, #37147, #16138, #2267, #45230, #10348, #38770, #21206, #24422, #34375, #45705, #23963, #23731, #30691, #38084, #20519, #7127, #31133, #20283, #2745, #13144, #14056, #35287, #34611, #6440, #2968, #35056, #27225, #27673, #16840, #41778, #30918, #42005, #6881, #10576, #45474, #17056, #24202, #27908, #13367, #3189, #13591, #45014, #10128, #3429, #31367, #3665, #34825, #9889, #38527, #38311, #20957, #6657, #27439, #20731, #17276, #13831, #17527, #31600, #28127, #42222, #24653, #41317, #9666, #6191, #14277, #1093, #8259, #14968, #25113, #21432, #11505, #24891, #14750, #15206, #39461, #28823, #648, #4124, #186, #418, #14522, #18439, #31816, #39227, #39701, #29294, #35508, #43370, #39917, #25804, #11048, #7580, #32293, #3883, #25346, #42903, #7819, #28599, #35983, #11270, #11734, #29053, #21657, #4566, #22325, #4348, #42450, #32517, #43139, #36426, #25590, #35745, #17752, #18657, #8049, #32046, #22113, #28348, #10818, #39005, #7356, #17976, #8489, #45126, #9332, #1326, #34497, #23622, #2622, #27337, #13484, #2857, #37731, #11948, #44900, #40970, #40126, #23401, #34250, #32987, #27115, #30333, #41661, #13025, #41206, #10016, #12780, #19952, #27556, #6083, #24085, #9562, #37504, #41430, #9781, #37269, #16722, #16255, #23161, #30806, #5629, #44426, #30564, #19723, #15430, #16483, #26015, #4789, #23848, #18892, #5863, #29507, #13259, #26862, #43580, #37962, #33811, #44664, #2164, #34027, #2383, #20401, #16949, #42799, #31491, #18096, #28719, #35181, #21542, #31255, #21095, #28236, #11159, #42581, #3996, #24537, #6771, #35624, #45594, #13942, #41892, #32177, #24316, #14401, #31706, #540, #3557, #38650, #17644, #14644, #7008, #38420, #6547, #10939, #28016, #73, #10237, #3771, #28480, #38199, #7252, #14165, #42331, #35399, #20847, #10698, #42110, #34945, #10461, #25012, #38898, #20626, #24780, #3313, #17861, #21323, #300, #31929, #17409, #39121, #7471, #34719, #3078, #45357, #13717, #27796, #43020, #1434, #18775, #40022, #21775, #8612, #15750, #22442, #32635, #28942, #19004, #32417, #22222, #22677, #1211, #36316, #8159, #11623, #7694, #7942, #22009, #25912, #39341, #978, #15535, #36774, #11384, #29616, #33096, #11841, #25701, #43694, #8373, #25467, #39586, #36100, #14866, #765, #15082, #4464, #36548, #32863, #4905, #18336, #18553, #1649, #29169, #43252, #12066, #15319, #39813, #4677, #5130, #29401, #26140, #43473, #40256, #19217, #33304, #29838, #43920, #25230, #35869, #4246, #12732, #12514, #30757, #30068, #30980, #26374, #8829, #26811, #37680, #20348, #2808, #6029, #15986, #27289, #5578, #5342, #12299, #19669, #2114, #34443, #40918, #1877, #44149, #40476, #41382, #16899, #16203, #33763, #30283, #16671, #22896, #9284, #26589, #40687, #9042, #23111, #37213, #33529, #44376, #23354, #27065, #19903, #41160, #19436, #37456, #36988, #5816, #33980, #34196, #2331, #16431, #30511, #37907, #44614, #44850, #12977, #9511, #2566, #20121, #13212, #23575, #9730, #23796, #6261, #45537, #6718, #24950, #10408, #31653, #38838, #39065, #15024, #11790, #40189, #22616, #25861, #18282 ),
 ( #12011, #1156, #32577, #25646, #29350, #14807, #4616, #39528, #42961, #21959, #4850, #15261, #8554, #36259, #11329, #8316, #43195, #33045, #25406, #7883, #11564, #39760, #18715, #43423, #36045, #15486, #43642, #26076, #36717, #32116, #481, #11102, #14586, #39282, #7638, #21714, #37139, #27215, #8973, #44538, #45003, #37603, #12897, #26983, #19825, #15905, #16130, #30217, #34124, #1796, #9204, #23723, #13358, #5497, #37836, #41309, #2491, #33908, #6185, #30682, #29990, #41082, #13137, #38074, #6433, #20275, #19591, #2737, #26741, #26523, #44077, #23278, #5738, #12443, #5956, #23041, #33688, #2037, #16831, #44307, #44781, #34367, #27432, #12661, #27663, #38517, #19535, #5684, #23215, #13083, #27167, #34310, #41255, #19775, #12837, #9611, #23672, #2680, #16776, #30856, #13307, #40361, #22780, #5225, #19315, #38250, #7061, #27848, #35227, #20672, #31073, #45408, #13770, #24361, #41945, #24141, #24584, #41714, #27607, #3606, #20895, #42157, #23901, #10750, #17909, #38701, #34763, #10070, #21144, #34547, #6817, #24827, #3369, #34993, #10287, #17460, #9832, #6594, #3125, #10508, #41479, #17214, #17692, #38947, #31301, #31753, #122, #13994, #31543, #14212, #28281, #45645, #42381, #7297, #16997, #2906, #21372, #35448, #3819, #31977, #27384, #20459, #38022, #6378, #32225, #11207, #36362, #36143, #18378, #28988, #40060, #7744, #32917, #25279, #585, #4723, #39857, #8198, #33137, #14687, #29442, #32458, #14907, #28763, #1262, #42843, #14453, #28531, #25518, #36599, #39391, #8420, #806, #10988, #11882, #32682, #11667, #18826, #22490, #25953, #15132, #21592, #22265, #4287, #4048, #43069, #43300, #42626, #4505, #21821, #4954, #22053, #18597, #25056, #35915, #11434, #39168, #29223, #7518, #25744, #39631, #35672, #7986, #12773, #38079, #31128, #42093, #35602, #38630, #55, #14380, #35156, #45574, #28459, #27998, #25446, #11137, #20827, #42558, #10444, #10921, #14625, #24520, #42776, #6989, #39319, #17620, #7674, #31688, #35849, #14148, #6754, #4225, #32398, #43000, #18318, #748, #28922, #22420, #29598, #30046, #43899, #5323, #25893, #8143, #36969, #32842, #1193, #43233, #19417, #25683, #15729, #33078, #33508, #36525, #40004, #4884, #1856, #8354, #39795, #7921, #12277, #15300, #22877, #15964, #44127, #29385, #43456, #18987, #11604, #1415, #15518, #43676, #22206, #12047, #26119, #12492, #36754, #11823, #26352, #39567, #40233, #18535, #8590, #5110, #21992, #22656, #4656, #8809, #40456, #19198, #36299, #29818, #36080, #4447, #18754, #33285, #1630, #32615, #957, #15062, #29149, #37436, #6240, #27042, #34423, #19882, #30263, #44595, #12955, #23556, #41140, #23332, #23775, #40896, #44355, #2791, #20100, #41364, #23091, #9938, #17103, #37889, #33959, #12712, #20329, #33743, #37658, #24010, #2547, #6007, #9493, #34175, #9021, #9264, #5796, #27273, #40667, #2311, #16883, #38132, #26791, #30965, #45059, #13192, #16652, #13416, #9712, #16410, #30490, #30738, #16182, #2093, #44832, #27485, #41583, #6483, #20562, #19650, #34657, #3016, #31184, #45279, #26569, #37191, #5557, #28171, #39265, #6929, #32097, #24468, #31413, #35549, #39048, #7397, #32339, #45519, #28644, #17567, #14097, #13873, #464, #27949, #13638, #27721, #10170, #42264, #21471, #21697, #4171, #3925, #17325, #42722, #21012, #6701, #41825, #35100, #3477, #35793, #10624, #3236, #42045, #24247, #11085, #18265, #31639, #7, #24701, #18020, #38356, #38821, #10392, #7175, #38574, #24933, #14568, #7621, #28400, #21248, #35328, #10867, #3706, #31858, #17792, #20779, #229, #14324, #34872, #42499, #25155, #8302, #7866, #32788, #25633, #1139, #18484, #5275, #39744, #26299, #36921, #43409, #29760, #25390, #29337, #36470, #19368, #5060, #12221, #15248, #15009, #43837, #8093, #22155, #4393, #8760, #32561, #22599, #22366, #22827, #25846, #4832, #18935, #695, #33030, #905, #14791, #19152, #36244, #28864, #42945, #11313, #4603, #18698, #1368, #29096, #15472, #29550, #43625, #43182, #11993, #26059, #39510, #40170, #8534, #33238, #21944, #36702, #36029, #1579, #15678, #11551, #44746, #40812, #44973, #2702, #23472, #44277, #20243, #30876, #27404, #26713, #41045, #6401, #33655, #9852, #2232, #26495, #41501, #2461, #41277, #6155, #23922, #20483, #16565, #37107, #23694, #16327, #19560, #30409, #13104, #8944, #20018, #44504, #34570, #37572, #9630, #2929, #12863, #26946, #29962, #37806, #44046, #34334, #5464, #2006, #16103, #30187, #12634, #27872, #6620, #35248, #3148, #10311, #42181, #31325, #45193, #28085, #24166, #35698, #35469, #31094, #35015, #34785, #10531, #20694, #28305, #38969, #11009, #31776, #17486, #24607, #14236, #45432, #3626, #24383, #13795, #6839, #3843, #146, #25076, #21167, #41969, #10774, #31565, #24851, #38487, #17239, #45665, #14017, #38724, #7086, #20919, #7319, #17934, #32003, #374, #14476, #28556, #13555, #39190, #7540, #21616, #17017, #27628, #41737, #38273, #10090, #1495, #25765, #15156, #32704, #36163, #32249, #32478, #828, #4745, #18173, #11459, #25974, #15593, #21845, #8442, #43536, #36383, #4525, #40082, #18849, #4306, #18398, #7767, #39415, #25303, #25542, #35938, #32939, #11692, #1285, #42863, #14927, #26213, #29010, #43093, #22512, #39877, #8007, #18617, #29675, #39655, #36622, #22073, #1050, #4977, #29463, #11903, #22745, #29247, #19070, #43324, #8218, #22287, #33158, #15384, #4074, #608, #14709, #43753, #12131, #40328, #8681, #28785, #11230, #6098, #30131, #29903, #36839, #44219, #26654, #13273, #37286, #26441, #40540, #19277, #20188, #44915, #40750, #12577, #9109, #41221, #5190, #33827, #9578, #30582, #23419, #23178, #27132, #5879, #37051, #5403, #8890, #22955, #12365, #5646, #19499, #19969, #44443, #34044, #43988, #1947, #27351, #33596, #16049, #13042, #12799, #19740, #2180, #16738, #16272, #23638, #30351, #26881, #37748, #16502, #44684, #9796, #40989, #34268, #9349, #37520, #2401, #2641, #30821, #33364, #1709, #15813, #41445, #3572, #31943, #14418, #17659, #27573, #38914, #17182, #16963, #23864, #31270, #13734, #314, #24330, #13497, #41677, #6336, #7267, #28497, #27811, #45372, #41908, #28248, #37981, #20861, #10034, #34960, #24101, #35195, #87, #3785, #38666, #10252, #17427, #21112, #6562, #42125, #38434, #38214, #6785, #42347, #24551, #42595, #28031, #34733, #31720, #3332, #14180, #31505, #20639, #45610, #13957, #10476, #7023, #3093, #10714, #24796, #21337, #35415, #17877, #20418, #34513, #2872, #31040, #45139, #19748, #15453, #34276, #33010, #23426, #9804, #34051, #37527, #5886, #44453, #39937, #40760, #9118, #13052, #25825, #2188, #44922, #37991, #30139, #19975, #26663, #13280, #27357, #41452, #16280, #2409, #34521, #44227, #6344, #30359, #22346, #20428, #30592, #9586, #2879, #16971, #31047, #44692, #1350, #11758, #12809, #12584, #26890, #23646, #36449, #16510, #27140, #37757, #7031, #21117, #4017, #6791, #13964, #39140 ),
 ( #20868, #41686, #14185, #45379, #38672, #6568, #31513, #24336, #45616, #17189, #18118, #38440, #25030, #35645, #42131, #28502, #24109, #28038, #35201, #45146, #3792, #10961, #10482, #13741, #42600, #34966, #3340, #3098, #7490, #31276, #21343, #3577, #21562, #24556, #17663, #31726, #13507, #93, #27818, #27580, #17882, #17433, #10040, #38221, #20646, #28253, #42352, #10721, #41915, #24801, #38920, #7272, #10259, #35419, #31949, #34738, #319, #14423, #4923, #36791, #1229, #25249, #15335, #25929, #15550, #36569, #43040, #1449, #19021, #18572, #14661, #11402, #25490, #33112, #42818, #39602, #29630, #43709, #32434, #26161, #40276, #5148, #32655, #32196, #21794, #7958, #22026, #36115, #4480, #997, #15100, #43269, #25718, #39830, #22238, #36335, #36455, #34413, #34862, #13864, #20551, #3005, #24458, #3467, #17093, #42036, #31172, #10382, #38565, #13868, #17318, #31408, #10619, #9706, #6923, #41577, #38126, #37882, #10386, #23769, #37652, #6000, #34168, #6477, #45515, #1, #28166, #27943, #41355, #21003, #30959, #30732, #20093, #45053, #27479, #14092, #20554, #27267, #6232, #2541, #35095, #42259, #9931, #13407, #24004, #42040, #16645, #34650, #20322, #3009, #34417, #3228, #24461, #17562, #6694, #17097, #31176, #34866, #2784, #10164, #45272, #16876, #13631, #38569, #38349, #44826, #41819, #27714, #3471, #24240, #31634, #20773, #13185, #42717, #11081, #21693, #25150, #21467, #21939, #39043, #42494, #900, #18261, #39505, #21243, #8088, #15244, #36024, #32089, #28394, #18477, #31853, #35788, #22150, #688, #4165, #7617, #35322, #36238, #29333, #4387, #459, #10861, #32556, #225, #32335, #4599, #14787, #28860, #42941, #39261, #7169, #7392, #35545, #25386, #38813, #14564, #15002, #18693, #24929, #29091, #43176, #11309, #7861, #11545, #25628, #3921, #18016, #28638, #14318, #39738, #32782, #1133, #43405, #24696, #3701, #17788, #22594, #33903, #15467, #8530, #33681, #33447, #15674, #26294, #37375, #5055, #30210, #36697, #29545, #2031, #37132, #5491, #30433, #43621, #26736, #29754, #12215, #11988, #44301, #26054, #11771, #25841, #8296, #40406, #19586, #19820, #2256, #16125, #40165, #40838, #19147, #4828, #39953, #33233, #1574, #16353, #8755, #1363, #43831, #22361, #9198, #36466, #22821, #36915, #5269, #12656, #18931, #19362, #1791, #15898, #29985, #23037, #23272, #5733, #26517, #44071, #12437, #8968, #40617, #33026, #6180, #13132, #34361, #3173, #45216, #6864, #2954, #9655, #24191, #44998, #6644, #37830, #2485, #16825, #30904, #41525, #13353, #41304, #41764, #27210, #16594, #20718, #38069, #13578, #10115, #27896, #27657, #23718, #13818, #17263, #6427, #20270, #34812, #45457, #31352, #2732, #9877, #20944, #30676, #24408, #27428, #41076, #41992, #17042, #38298, #10335, #38512, #35041, #31120, #5951, #3416, #23950, #34119, #20508, #17510, #26976, #34596, #44532, #12892, #9432, #23497, #37598, #20041, #44774, #25571, #32277, #22099, #21642, #3869, #21877, #35967, #17739, #28810, #42433, #21194, #4106, #31802, #24877, #11033, #172, #14044, #42671, #38756, #4550, #4334, #45691, #17961, #28114, #7566, #7342, #42208, #634, #14263, #25099, #7113, #32030, #10802, #403, #3651, #36189, #38992, #11491, #31588, #28584, #14952, #10558, #14506, #35728, #24635, #18423, #43122, #39214, #28331, #29036, #21419, #35495, #35273, #39684, #18201, #7802, #14736, #8032, #42889, #11256, #25331, #39446, #32503, #852, #32730, #22987, #11932, #1979, #40784, #26688, #25999, #40109, #19099, #36411, #26245, #1524, #40356, #1313, #8708, #33188, #16076, #15843, #8472, #37081, #9141, #36869, #43352, #5220, #22543, #5436, #18642, #15622, #4772, #29705, #22312, #29935, #40571, #44251, #33394, #5008, #12161, #44018, #15413, #19309, #36650, #32968, #43781, #19529, #1740, #23209, #22775, #29491, #12391, #26470, #8918, #33628, #18877, #30160, #12611, #37320, #1077, #43563, #15189, #29275, #11718, #25790, #39904, #8244, #2209, #34758, #41937, #2901, #13076, #9380, #45168, #12833, #2674, #3120, #27378, #16769, #34302, #37779, #33855, #34072, #2433, #6371, #19769, #27161, #27602, #17209, #23446, #10065, #13528, #38016, #6127, #41709, #20453, #5905, #19994, #37547, #41020, #26912, #41249, #16535, #34541, #13302, #16992, #44475, #30618, #27843, #44715, #9605, #24133, #41474, #23666, #20218, #31296, #30850, #38244, #44946, #9826, #6589, #31068, #20667, #24356, #23896, #45402, #13766, #10282, #5678, #16300, #30384, #11426, #6812, #34988, #7292, #18140, #801, #28983, #32220, #42152, #7738, #31746, #31538, #38460, #117, #28275, #14901, #38942, #28059, #10503, #20890, #21816, #43064, #42376, #14207, #7055, #10744, #42838, #39163, #3363, #42621, #3600, #580, #21367, #14681, #24822, #24579, #35443, #3812, #17904, #31972, #35222, #35667, #21139, #38696, #28758, #343, #7513, #17455, #35909, #45639, #4042, #14446, #17687, #11202, #13987, #28526, #4282, #10982, #25051, #21585, #25274, #39384, #18373, #32453, #26185, #39626, #32912, #1684, #22931, #43295, #29877, #19251, #12106, #11877, #15788, #40299, #25738, #39852, #29215, #15126, #1023, #1255, #11662, #8653, #33132, #22717, #18592, #36357, #1919, #8193, #22260, #43962, #1469, #29436, #40055, #5379, #18820, #12339, #4716, #15358, #26413, #5167, #33339, #44190, #43510, #40514, #25948, #8415, #22483, #8865, #36593, #25512, #7980, #22047, #4950, #37025, #33568, #16025, #19473, #19041, #30105, #15568, #32676, #36138, #29651, #43728, #4500, #36811, #2151, #16243, #40724, #41647, #20614, #16469, #5852, #30552, #16938, #12552, #9549, #30322, #23612, #44414, #23835, #34486, #38189, #27326, #44653, #6070, #9769, #40958, #30795, #19940, #13473, #45116, #9321, #37719, #34709, #12768, #6534, #13014, #9081, #10003, #44888, #37950, #2845, #3067, #24072, #13248, #19713, #6305, #2372, #26849, #27104, #41419, #23147, #34235, #37492, #17158, #20159, #2610, #31244, #34016, #41195, #26626, #20389, #37256, #16710, #31018, #27543, #5617, #23391, #33799, #10450, #34934, #17849, #31478, #38637, #24767, #13930, #27782, #10684, #6761, #18324, #3983, #13703, #17629, #41881, #21310, #21081, #10225, #14387, #45582, #38883, #20835, #31694, #24527, #62, #17394, #4232, #6996, #25214, #35855, #42319, #28703, #24303, #28225, #35386, #45340, #18080, #11144, #14154, #28005, #42782, #35165, #3543, #3300, #39326, #42100, #21530, #7238, #7681, #3759, #31916, #287, #21761, #28466, #42567, #38410, #32160, #10928, #24996, #39107, #7457, #35610, #525, #14631, #5062, #40624, #15907, #8975, #15682, #23043, #1799, #30439, #30219, #26302, #5740, #9438, #5500, #11995, #19594, #44309, #16359, #2039, #43839, #2262, #19827, #26525, #1582, #23282, #37142, #29762, #33691, #29993, #44540, #12663, #40412, #33910, #23503, #16132, #26061, #26743, #40845, #12900, #9207, #12223, #26986, #41086, #37383, #8762, #37605, #5958, #32404, #22829, #44079, #1370 ),
 ( #36923, #12445, #15474, #29553, #43628, #40172, #5277, #8536, #22602, #19154, #36704, #19371, #33240, #33455, #6187, #13360, #45223, #34369, #2493, #31126, #27217, #38762, #24416, #34126, #38076, #16601, #41772, #41532, #30684, #34818, #20277, #13585, #41311, #6435, #45005, #20514, #37838, #24644, #27434, #45697, #10567, #17047, #3423, #44785, #2961, #10122, #20047, #38520, #31594, #34604, #2739, #17519, #9884, #23956, #23725, #14050, #16834, #41998, #27666, #28120, #24197, #38304, #6652, #42216, #20726, #30912, #13140, #6871, #3180, #9661, #17270, #31359, #45465, #13825, #27902, #10341, #20952, #35049, #22106, #410, #177, #7120, #14514, #42676, #29284, #7572, #42440, #10810, #35279, #36195, #15198, #11039, #28591, #25105, #11498, #21199, #4115, #24884, #18209, #38998, #18430, #29045, #32739, #21887, #39220, #639, #4340, #35501, #25337, #21649, #21425, #35736, #25579, #7808, #43361, #11261, #17968, #32510, #32284, #14959, #14741, #7348, #28815, #42895, #39453, #35976, #3875, #859, #32040, #43131, #39694, #8041, #4559, #3657, #18649, #11727, #1085, #25796, #17745, #31809, #14271, #28340, #37327, #15851, #5227, #22782, #26251, #22317, #22551, #36656, #40578, #8251, #1531, #16084, #5688, #11939, #44259, #33634, #26476, #40364, #30168, #8924, #40116, #8481, #43571, #29499, #15421, #15627, #26006, #22994, #1746, #37088, #32977, #5016, #16309, #19107, #33194, #12617, #29941, #43787, #8716, #19778, #29710, #26695, #12169, #36877, #40791, #19539, #1987, #12840, #19318, #9150, #33401, #44025, #12397, #23220, #5444, #39910, #36418, #4781, #33862, #2215, #30391, #44483, #18883, #1319, #6821, #17464, #23905, #10290, #5911, #9835, #17000, #31547, #31305, #38469, #13310, #41258, #24366, #20226, #34314, #30628, #20899, #13087, #3129, #20462, #34997, #38026, #27387, #6381, #3374, #41482, #27170, #41027, #45413, #2683, #45649, #26923, #9387, #16780, #30860, #34551, #44724, #2910, #31076, #45175, #9614, #13535, #27610, #23453, #24144, #44954, #13774, #37553, #41719, #20001, #10073, #38253, #34078, #6599, #37787, #41949, #27852, #20677, #23675, #17218, #2441, #16544, #6135, #34767, #36145, #17696, #39634, #17913, #10513, #43071, #32229, #11211, #35918, #7989, #11436, #589, #21148, #7746, #3823, #3609, #31982, #42846, #42161, #35676, #38951, #4507, #21596, #4053, #18599, #21376, #28535, #22055, #14691, #32685, #18152, #353, #4289, #18380, #126, #25282, #24831, #31757, #28767, #14217, #7301, #39173, #28286, #24588, #25060, #35230, #13998, #32460, #28066, #14458, #38705, #39393, #35452, #7066, #21825, #42385, #7522, #10755, #42630, #10992, #808, #14909, #28991, #25521, #36603, #5385, #1689, #9087, #5172, #11885, #26421, #1476, #8872, #40063, #4726, #19049, #33140, #43734, #15576, #43519, #43970, #15365, #18829, #22936, #40308, #15793, #43303, #30111, #37263, #12345, #8423, #32921, #40521, #8201, #12112, #44200, #22723, #26192, #29657, #8661, #29227, #29446, #25956, #29883, #15135, #22493, #37032, #12558, #1265, #19478, #33575, #33346, #36819, #1927, #16030, #4957, #19258, #26634, #36365, #22268, #40730, #23154, #5624, #19718, #1031, #39860, #11671, #25748, #37498, #30557, #10010, #9774, #37725, #2617, #13711, #27110, #6540, #44659, #5858, #24080, #13479, #27550, #6766, #19946, #3072, #6077, #34242, #34022, #20620, #2377, #33805, #2158, #30327, #16717, #41654, #41887, #24310, #38194, #16478, #17163, #41200, #26854, #16250, #9557, #23617, #10230, #30801, #23396, #13020, #44421, #31250, #38415, #20165, #44894, #13254, #34714, #12775, #27332, #41425, #23843, #37955, #45121, #45349, #27789, #2851, #6314, #20396, #31023, #34491, #16944, #40965, #9327, #42105, #28473, #35392, #42574, #45587, #35175, #7687, #10455, #21090, #35617, #17855, #28231, #24775, #11151, #17636, #18086, #3551, #24532, #21535, #39113, #7462, #35861, #38645, #14636, #42326, #10690, #7002, #32169, #31700, #20841, #3306, #17402, #38891, #3989, #21766, #34940, #532, #67, #25220, #7245, #14160, #31486, #21317, #3765, #13935, #31921, #293, #14392, #10933, #28010, #25002, #28709, #42789, #39332, #20766, #16398, #13401, #34162, #27473, #20087, #27708, #38343, #42032, #31168, #2778, #9923, #13624, #44820, #34644, #23763, #30726, #6224, #34857, #17089, #24454, #20547, #27259, #41812, #16870, #24234, #9699, #2533, #34409, #30952, #41571, #45046, #13178, #10158, #41349, #16638, #6688, #23996, #45265, #12942, #45507, #6915, #3221, #37876, #20316, #17311, #23542, #38118, #13860, #6471, #3001, #31402, #27936, #44581, #10378, #38561, #20995, #30478, #35088, #27028, #41127, #9479, #37645, #5994, #35780, #35539, #39496, #18253, #3694, #17781, #7162, #38806, #24687, #10853, #14997, #35316, #25379, #42711, #29084, #451, #3915, #32081, #43171, #18009, #31846, #17556, #7853, #42486, #32548, #25621, #11539, #24922, #39036, #14555, #21236, #11075, #28633, #25143, #218, #39256, #7610, #894, #681, #7385, #21931, #39732, #21687, #28160, #4158, #14781, #8081, #32327, #14312, #18469, #36016, #28853, #28384, #4379, #22143, #3463, #21461, #42934, #31628, #11301, #11299, #14085, #42253, #10611, #8751, #33441, #12432, #30206, #19581, #22817, #43400, #29980, #26047, #25834, #8523, #19355, #18688, #12209, #15460, #26731, #43825, #26288, #40834, #43613, #5051, #44296, #36909, #9192, #40401, #22588, #26511, #40612, #22355, #1784, #1357, #39946, #5263, #36460, #29538, #15667, #4822, #32777, #1569, #11766, #36232, #8963, #4593, #36692, #1124, #15894, #11979, #15237, #44067, #18924, #29747, #8291, #19142, #40158, #33229, #33019, #29326, #23032, #16120, #37127, #5484, #33676, #2026, #12651, #13349, #13813, #27651, #34806, #9649, #37592, #20713, #16589, #30671, #26970, #9425, #44768, #2725, #5946, #5729, #34356, #30427, #41988, #41760, #37367, #41299, #19815, #44993, #13127, #33898, #38064, #23492, #16821, #44527, #23714, #2481, #37825, #41067, #27891, #27205, #3168, #23267, #20265, #6640, #2252, #6176, #27424, #16347, #10110, #17259, #30899, #20037, #31346, #41521, #9873, #34114, #45453, #23944, #45211, #6421, #12885, #20503, #34592, #2949, #17037, #31115, #13574, #24187, #38293, #3647, #39439, #32496, #18417, #17734, #31797, #10798, #28107, #17955, #38988, #32026, #38751, #397, #24872, #7794, #7561, #167, #28804, #846, #28579, #35036, #42667, #21636, #21871, #25095, #21189, #25324, #42882, #3865, #24630, #629, #11250, #35959, #7109, #21414, #14946, #14039, #4327, #14258, #6858, #29029, #11029, #35722, #32271, #10330, #24404, #39209, #17506, #4100, #28326, #45686, #42427, #18195, #38507, #14501, #35269, #20940, #14731, #3412, #31584, #7338, #35490, #42204, #10552, #33621, #33181, #15405, #33386, #1731, #29269, #40350, #8237, #32723, #15613, #26463, #29698, #8702, #19301, #37075, #40564, #43773, #4543, #36862, #32961, #1071, #29485, #26238, #25564, #19093, #22306, #1972 ),
 ( #16070, #15836, #11485, #43556, #39677, #1518, #18870, #8025, #12155, #43345, #36644, #18637, #11922, #36403, #25993, #15180, #43116, #4766, #22979, #22093, #40101, #8912, #36183, #8465, #22768, #11712, #29928, #5427, #22535, #25783, #19522, #1307, #5000, #39895, #5213, #44012, #12385, #24290, #42307, #27767, #31230, #13688, #10671, #45326, #31005, #44244, #35149, #24057, #14142, #7225, #38870, #38175, #20602, #41869, #2833, #38396, #10213, #6746, #13460, #20820, #34921, #28213, #27991, #34697, #3526, #21296, #3285, #9133, #17380, #42086, #24755, #45567, #41629, #48, #17612, #13919, #45103, #21066, #31681, #35374, #27529, #10437, #3749, #34473, #30154, #3056, #26680, #24512, #38621, #12602, #6981, #9988, #40776, #23200, #37309, #17145, #5671, #19762, #16925, #14620, #28914, #39999, #21519, #43451, #21747, #14373, #1187, #36075, #15057, #39789, #11818, #15295, #4442, #24984, #11598, #7669, #7444, #35844, #951, #276, #39561, #42771, #8347, #25440, #7916, #22415, #25203, #32391, #25886, #18528, #36518, #21986, #4219, #8137, #22201, #3973, #29143, #28692, #35596, #32610, #18067, #11131, #42995, #32149, #28454, #11361, #39094, #17837, #36293, #31904, #18312, #42553, #43227, #39313, #10915, #25676, #512, #4651, #742, #14841, #18748, #32836, #29379, #9486, #43891, #30484, #41134, #1850, #33954, #29593, #33502, #40662, #23548, #9259, #16404, #36963, #19193, #2305, #12271, #26346, #8585, #44589, #36747, #26786, #44121, #12949, #15956, #5317, #30040, #27035, #19412, #5105, #18981, #23328, #40450, #4879, #33071, #1410, #8804, #22871, #12487, #22649, #26564, #9016, #23086, #33280, #37186, #5550, #15513, #2086, #19644, #37431, #43671, #33736, #12042, #16177, #26111, #30258, #1625, #40226, #5787, #44350, #15724, #29812, #12707, #40891, #19877, #27184, #44497, #34327, #9627, #2698, #9401, #16795, #41272, #24159, #23918, #20014, #45189, #3144, #44968, #5705, #13324, #38039, #10086, #41496, #37567, #41732, #13550, #20240, #41040, #17013, #27624, #38269, #23468, #37802, #17234, #30405, #6615, #30644, #23237, #20690, #27400, #6396, #2924, #34781, #31321, #20479, #33875, #34566, #16559, #16323, #44742, #31090, #9164, #30872, #5924, #45427, #26708, #40807, #37343, #34091, #23690, #19792, #2228, #12859, #26940, #13100, #2456, #6150, #45661, #11005, #24602, #3387, #31998, #14011, #7080, #38965, #28081, #41963, #24846, #20914, #32474, #18168, #27868, #31771, #10306, #35465, #35244, #24379, #28551, #42177, #7315, #35011, #142, #38720, #14232, #31561, #18394, #21161, #39409, #4303, #10769, #42859, #38483, #42400, #3838, #13790, #32244, #25298, #28300, #10527, #11226, #3622, #17710, #17481, #7763, #21392, #35693, #17929, #21840, #370, #14471, #604, #42644, #35933, #6835, #25072, #39186, #7536, #21611, #4070, #14705, #28781, #8438, #29241, #22508, #15380, #43983, #43748, #39873, #19272, #22951, #19065, #25537, #33154, #12126, #29899, #15589, #11688, #15808, #33360, #40077, #15152, #36834, #1704, #12360, #43319, #11898, #37047, #4521, #26437, #4741, #43088, #40536, #1491, #26209, #22741, #8885, #5399, #29671, #8003, #40323, #36379, #36159, #18845, #8676, #29005, #36617, #25761, #19494, #4972, #5186, #823, #8214, #29459, #14923, #11454, #39650, #22069, #32935, #18613, #32699, #1045, #22283, #1280, #43532, #25970, #19735, #26875, #13037, #2176, #16044, #44680, #40746, #6558, #37976, #1942, #5875, #30127, #9574, #9344, #44215, #2637, #33823, #27127, #9104, #19965, #12794, #34039, #5641, #38209, #40985, #13494, #24095, #30577, #16959, #12573, #16496, #23634, #33592, #6331, #45135, #2397, #16268, #31036, #23414, #37516, #37282, #27568, #30346, #9792, #41217, #41672, #37743, #6094, #20184, #10030, #34261, #44438, #26648, #20413, #23173, #16734, #30816, #44911, #13269, #27347, #23859, #41441, #34509, #2868, #14176, #17872, #3326, #38909, #28027, #34956, #10471, #25023, #21333, #28730, #24792, #31501, #310, #21108, #28493, #13952, #24326, #38661, #7017, #17655, #35191, #17423, #31939, #45605, #38430, #42591, #28245, #35411, #17178, #4008, #11169, #14412, #42121, #6780, #10951, #27807, #31716, #18107, #42342, #83, #3567, #10708, #3088, #24547, #7262, #3781, #34729, #39131, #7483, #32189, #20857, #21552, #35635, #550, #14653, #42810, #25241, #39351, #20635, #31265, #10248, #41902, #45367, #13730, #22453, #15327, #36557, #775, #18563, #29847, #11393, #4472, #29623, #29409, #11631, #22230, #33312, #987, #26151, #32645, #25477, #43702, #33104, #1442, #26382, #39595, #22686, #25709, #8167, #7950, #40267, #22017, #7706, #21785, #4255, #36326, #15543, #15759, #43931, #12075, #36108, #36782, #15092, #14875, #35880, #29178, #43261, #12310, #4687, #43030, #39821, #18345, #5138, #32426, #18783, #32874, #1220, #43481, #11849, #25920, #40030, #8384, #19225, #4915, #19012, #8621, #28949, #1657, #19443, #12986, #6036, #23803, #9518, #5586, #9738, #13219, #33986, #9049, #30766, #41390, #27296, #37221, #5824, #16906, #44156, #20356, #44383, #36995, #37915, #27074, #37689, #16679, #34452, #6269, #41167, #1885, #34204, #30291, #30077, #12739, #23584, #22904, #16438, #19678, #30987, #2338, #30519, #45084, #2123, #9291, #2815, #20128, #13440, #44621, #26819, #44857, #40484, #26596, #2574, #33772, #12522, #8836, #40694, #16210, #19910, #23118, #5349, #33537, #15996, #40924, #23361, #37462, #45545, #9966, #3504, #3262, #24035, #42286, #27746, #21039, #34679, #13896, #6724, #27970, #45304, #32124, #20799, #7422, #18044, #24491, #10892, #6504, #10415, #17590, #489, #31881, #39073, #42066, #41848, #24959, #34896, #17354, #31209, #21495, #13663, #3727, #35126, #35572, #38598, #6955, #31661, #3949, #28, #10192, #41608, #253, #31439, #27510, #38155, #20583, #14120, #28193, #10648, #24268, #24727, #3036, #14350, #17124, #38848, #38376, #7201, #21272, #35352, #17815, #28427, #42526, #21724, #929, #39536, #15033, #32363, #19177, #7893, #40202, #5086, #11575, #43651, #39290, #43204, #4628, #33262, #18958, #26088, #29121, #28890, #12020, #21968, #36054, #18289, #8563, #719, #36495, #8117, #22628, #25656, #39769, #22177, #36728, #36272, #14817, #28669, #33054, #4416, #14596, #42747, #11109, #18508, #32587, #18725, #42971, #32813, #1165, #15273, #11337, #29359, #43431, #25179, #11799, #25868, #1391, #7645, #39978, #35817, #8327, #22391, #4196, #4858, #25416, #29575, #15495, #40871, #15934, #37628, #2516, #34145, #44104, #12686, #23747, #5299, #27241, #5525, #43870, #30708, #19853, #44564, #23526, #41333, #44805, #33933, #8785, #41110, #37166, #36946, #19620, #30460, #29790, #23306, #26547, #37860, #9235, #37407, #6208, #8998, #16157, #9683, #2284, #20301, #5765, #33716, #5979, #20071, #33480, #12925, #12468, #19393, #16383, #1826, #40645, #26765, #30018, #12249, #27011, #22853, #9463, #16622, #2065, #13162, #1608, #23066, #30239, #44331 ),
 ( #15705, #26328, #40433, #31387, #34842, #17297, #206, #3206, #34630, #2763, #38792, #27693, #17770, #10838, #42472, #41796, #10146, #45492, #6457, #42021, #13848, #10367, #17074, #24442, #27926, #31835, #31618, #24221, #7147, #24910, #6899, #13385, #20979, #45721, #14298, #3448, #45249, #3683, #21225, #38547, #2987, #24673, #35306, #28370, #31152, #35076, #39024, #38101, #7374, #38329, #30937, #34392, #17545, #14074, #10597, #16857, #45030, #28148, #41555, #42241, #6675, #23981, #20751, #27458, #9909, #20536, #13609, #12582, #29680, #43758, #26659, #28842, #36627, #16054, #22750, #40755, #12136, #39482, #12370, #26446, #7598, #19282, #32313, #11065, #40333, #21674, #14770, #1500, #35767, #3902, #33163, #28619, #21450, #40545, #35526, #8447, #17995, #22517, #25132, #39245, #32067, #5408, #30136, #25365, #42922, #4982, #8895, #439, #19075, #4145, #15598, #18239, #33369, #43993, #1952, #36845, #26218, #8686, #1714, #669, #5196, #11288, #15818, #29908, #22961, #37056, #44224, #19504, #33601, #14541, #42701, #16967, #2405, #12804, #27136, #41225, #6102, #9582, #5883, #6340, #23423, #26886, #31044, #2645, #23868, #5651, #38217, #45375, #20422, #16506, #40993, #2876, #16277, #20192, #6565, #30825, #34272, #37753, #23642, #37291, #37524, #19972, #9800, #23183, #30586, #45143, #20642, #9353, #13501, #27576, #41449, #16742, #41681, #37985, #34048, #44688, #13046, #44448, #30356, #44919, #13277, #34517, #27354, #10037, #2185, #24104, #31273, #34736, #3096, #17185, #13738, #27814, #9114, #19745, #33832, #14658, #7026, #13960, #18114, #21558, #35640, #14880, #28034, #11176, #89, #42349, #42128, #28734, #10479, #41911, #10255, #38437, #10716, #4014, #4260, #32431, #32194, #45613, #25246, #35197, #34963, #24333, #3575, #31722, #18351, #21791, #14182, #6788, #39355, #14420, #39138, #556, #35885, #7711, #28499, #3335, #42815, #28250, #31509, #24798, #25027, #20864, #17879, #21114, #780, #3788, #31945, #17430, #17661, #38916, #24554, #42597, #38669, #316, #7269, #21340, #35417, #10957, #7488, #39827, #18567, #1446, #15098, #22235, #8389, #43266, #11399, #40034, #36112, #1892, #33316, #43036, #1225, #25484, #4920, #4692, #39600, #43707, #29185, #22459, #4477, #15332, #8172, #29416, #994, #33543, #36332, #8841, #19448, #25925, #12315, #7955, #11854, #19017, #28957, #1662, #40490, #43486, #11637, #26389, #18791, #32880, #32651, #22909, #25715, #5144, #36565, #37000, #33109, #15548, #29627, #5355, #12081, #26158, #22023, #15764, #40272, #8628, #22691, #36788, #19230, #29853, #43936, #33776, #23588, #44625, #37693, #44387, #6041, #30523, #13444, #13224, #9296, #34458, #38162, #34207, #40700, #2581, #27301, #45089, #30770, #26823, #30991, #2820, #9524, #30294, #6275, #16912, #27514, #12743, #27077, #6511, #19684, #12527, #41615, #20589, #41394, #23365, #2128, #9742, #23122, #12989, #9973, #20132, #41170, #16684, #2342, #44164, #40930, #37467, #44861, #30082, #5828, #37919, #24042, #16216, #20362, #23809, #34684, #16442, #16000, #26601, #19914, #33991, #9056, #5592, #37227, #10421, #38383, #17822, #10656, #31889, #41854, #13903, #25186, #6731, #45552, #24967, #24738, #6963, #17596, #28675, #42072, #21502, #27977, #20805, #39081, #28437, #42535, #21731, #34904, #18051, #21047, #3512, #3267, #35580, #17362, #3042, #17131, #45310, #31667, #10899, #11117, #39298, #7429, #31447, #32133, #24498, #10199, #31215, #38606, #35132, #7653, #34, #14127, #28199, #13672, #498, #27752, #42293, #38856, #7208, #3958, #24277, #21281, #35359, #3734, #261, #14357, #14604, #42754, #4866, #22187, #29368, #33061, #18515, #8335, #43212, #4427, #25664, #40209, #36502, #43877, #39987, #938, #15502, #36280, #43658, #29127, #39546, #8125, #4637, #32821, #18735, #32595, #1398, #15042, #7903, #12029, #43438, #18967, #25424, #29582, #11806, #26096, #28899, #11585, #12256, #21975, #39777, #8572, #25875, #1173, #15282, #15714, #22399, #22637, #36735, #36061, #5093, #19183, #33269, #8792, #1615, #29799, #26336, #40440, #35827, #4205, #18297, #32374, #727, #14825, #42980, #11346, #27249, #9690, #41118, #44111, #2524, #5532, #1834, #22860, #33723, #16164, #41340, #26773, #12475, #26554, #19402, #16629, #23754, #30246, #19629, #44338, #5986, #36953, #23313, #40652, #37416, #9005, #9471, #20078, #5306, #23533, #40879, #2292, #37635, #2072, #44572, #12693, #9242, #5772, #30716, #27019, #33488, #34153, #19860, #44812, #33940, #13169, #16390, #37174, #30469, #12932, #15943, #30026, #23075, #15633, #32743, #36200, #40370, #11944, #33199, #14965, #1750, #8929, #29716, #25801, #22110, #12175, #25585, #15426, #15858, #40121, #29504, #1323, #4786, #862, #1089, #15203, #19112, #32514, #39914, #8721, #29947, #4563, #22787, #26257, #5021, #18889, #36882, #1536, #18654, #29290, #43366, #8045, #39698, #8256, #32984, #11731, #26012, #43576, #8486, #22322, #22557, #36661, #44031, #43793, #36422, #5232, #40583, #19322, #43135, #33407, #12402, #26481, #22999, #37094, #18436, #29049, #11502, #19782, #41486, #6386, #38030, #2220, #16548, #27614, #9155, #31081, #9390, #1993, #34555, #23680, #2687, #27391, #45179, #2914, #37791, #12622, #44958, #41031, #40797, #23459, #34318, #33640, #27174, #30396, #41723, #13092, #41262, #10077, #12845, #20006, #13541, #6141, #24149, #9618, #37558, #9841, #23909, #37333, #16785, #16314, #23227, #20230, #5695, #44489, #30633, #33867, #16089, #44729, #26700, #5449, #20467, #19544, #5916, #30173, #30864, #26928, #44264, #13315, #34082, #17004, #2447, #24591, #17469, #38708, #10294, #42850, #31551, #18158, #28771, #35234, #21601, #17224, #21151, #28290, #11217, #42635, #4057, #7070, #6824, #35682, #45652, #14001, #41953, #32233, #24369, #14462, #31761, #594, #3613, #17700, #131, #14695, #14220, #38473, #6603, #10996, #28069, #38257, #20681, #34771, #42165, #10516, #42388, #27858, #7305, #10759, #21382, #31309, #3377, #3134, #20904, #35000, #28540, #24836, #38955, #35456, #45417, #3828, #25064, #17917, #31988, #39177, #358, #7527, #13779, #43077, #40313, #29232, #25752, #25525, #43739, #11441, #43975, #39399, #21829, #39864, #4963, #33352, #15799, #19055, #28995, #8667, #18604, #18384, #25286, #32689, #15139, #1694, #8205, #14914, #39639, #7750, #22730, #29888, #43307, #1037, #11676, #29663, #35923, #22273, #7993, #36369, #22059, #36608, #1481, #5177, #40067, #4732, #18833, #22497, #36149, #43523, #32925, #4511, #1271, #12118, #25961, #4294, #29450, #15370, #33145, #11889, #15581, #8429, #26198, #36825, #19263, #32464, #812, #9092, #9563, #26640, #30118, #34251, #5864, #27116, #8877, #41431, #2858, #23623, #19724, #16035, #6084, #19485, #9333, #9782, #34028, #23402, #40971, #44427, #40527, #40736, #23162, #13026, #26427, #33812, #2623, #23849, #44205, #16723, #20171, #44665, #12781, #30807, #41207, #12564, #37270, #5630 ),
 ( #2384, #30334, #44901, #13260, #2165, #37732, #16256, #1932, #30565, #26863, #37505, #19953, #16484, #22941, #27338, #33581, #31028, #37963, #37038, #6319, #5390, #20402, #34498, #16950, #12350, #45358, #38651, #6548, #31492, #24317, #45595, #17170, #3997, #38421, #25013, #35625, #42111, #28481, #24086, #28017, #35182, #18097, #3772, #10940, #13943, #13718, #42582, #6772, #20848, #3079, #39122, #31256, #21324, #7009, #7472, #10462, #24538, #21096, #21543, #3558, #27797, #13485, #17862, #34946, #45127, #27557, #41662, #3314, #17410, #17645, #41893, #31707, #74, #14166, #10238, #28237, #42332, #10017, #10699, #24781, #31930, #38200, #38899, #20627, #7253, #35400, #34720, #301, #14402, #1435, #4906, #25702, #766, #22443, #33097, #19005, #28943, #43253, #8613, #35870, #12067, #36101, #28720, #15536, #4678, #29402, #43021, #4247, #8374, #11842, #25913, #5131, #18337, #29617, #4465, #32636, #32418, #43695, #14867, #32178, #541, #42800, #979, #40023, #40257, #22678, #36549, #11385, #26141, #25468, #25231, #14645, #39587, #22010, #36775, #15083, #21776, #7943, #11160, #39342, #7695, #18554, #29170, #11624, #39814, #8160, #22223, #36317, #18776, #32864, #43474, #1212, #15320, #34619, #5579, #12733, #17063, #1878, #38091, #26590, #33530, #9043, #24208, #20525, #27914, #23969, #30069, #45237, #19670, #27680, #12515, #22897, #37214, #33764, #16204, #2115, #15987, #31140, #44150, #36989, #41785, #26812, #2974, #15751, #3195, #10355, #13597, #40688, #5343, #10135, #26375, #30284, #17284, #41544, #44377, #9896, #6446, #1650, #23112, #38318, #6665, #33305, #20738, #34832, #31373, #19437, #45481, #13837, #42011, #24431, #38535, #19218, #29839, #43921, #12300, #8830, #40477, #14286, #42230, #21664, #14530, #35754, #45711, #17759, #29060, #10583, #3672, #28830, #28606, #10826, #21439, #32524, #194, #25353, #39467, #31823, #24661, #42910, #32301, #655, #25598, #38777, #21905, #24898, #7363, #7135, #7827, #21213, #6888, #20966, #3437, #35515, #14756, #14975, #43146, #11277, #35294, #35990, #28355, #28135, #35063, #42459, #39012, #11512, #3890, #17984, #32054, #17534, #4356, #31607, #425, #11055, #25120, #18446, #39234, #7587, #4133, #18225, #872, #5243, #15868, #19554, #8731, #26023, #33210, #36890, #22331, #12185, #1333, #8266, #29515, #44041, #40380, #2002, #43803, #4796, #19333, #40133, #1760, #32995, #43376, #11955, #8496, #36671, #22567, #36432, #33416, #18899, #11743, #29957, #1547, #22796, #36208, #23009, #30182, #12411, #15437, #25810, #26491, #1100, #5031, #37103, #15642, #19121, #29725, #26266, #22120, #43587, #40592, #8938, #8055, #5459, #33650, #16098, #39923, #44273, #12630, #39708, #4572, #18663, #32753, #15214, #29302, #12130, #43752, #29674, #15812, #26212, #23177, #16048, #37285, #1494, #19276, #30581, #40327, #5189, #30350, #30130, #12364, #22954, #34043, #1708, #44683, #16500, #29902, #43987, #8888, #8680, #44218, #37050, #12576, #36837, #26652, #5402, #5878, #5645, #26440, #26880, #13041, #40749, #33157, #9108, #19739, #37519, #33826, #33363, #23418, #40988, #1946, #22744, #44441, #9348, #19968, #40539, #19498, #27131, #33595, #2400, #2179, #4976, #8441, #16271, #12798, #22511, #36621, #19068, #15592, #2640, #34959, #31039, #30820, #13496, #24329, #23637, #17181, #20417, #31719, #3092, #31269, #86, #2871, #10033, #35194, #41906, #14179, #45371, #27572, #31504, #45609, #27350, #38433, #6334, #44914, #13733, #41444, #34512, #20638, #9795, #37747, #6561, #16737, #41220, #13955, #9577, #41676, #6097, #27810, #16962, #20187, #10251, #23863, #34732, #13272, #24099, #45138, #38213, #37980, #34266, #6784, #21111, #20860, #3331, #24550, #17426, #28030, #42124, #10475, #38665, #7022, #3571, #17658, #25713, #21556, #35638, #31942, #39824, #14417, #4475, #21789, #8170, #25245, #28733, #11173, #22233, #42813, #28496, #42346, #32649, #4012, #11635, #24795, #39354, #7953, #36330, #18788, #22021, #313, #43264, #18112, #21336, #28247, #32192, #554, #4690, #7709, #17876, #42594, #10713, #32878, #1223, #14657, #35883, #4258, #991, #38913, #18349, #10955, #32429, #25026, #39598, #18566, #7266, #43033, #778, #14878, #25482, #39135, #28954, #11397, #7486, #36111, #15096, #29183, #35414, #3784, #26156, #40698, #15762, #23120, #8625, #19015, #33314, #1660, #12313, #29851, #12078, #12525, #29625, #33108, #37225, #8839, #30080, #11852, #44385, #5827, #26599, #22689, #1445, #9054, #22457, #26386, #12741, #36998, #40488, #43934, #22907, #43484, #43705, #40271, #15999, #29414, #36786, #5590, #26821, #15546, #19681, #33774, #1889, #5353, #2126, #44161, #5142, #19228, #19446, #4918, #36562, #33541, #16213, #30292, #40928, #9294, #8387, #23363, #37464, #19912, #33988, #15330, #25923, #40033, #16910, #27975, #41392, #20803, #13222, #20130, #24275, #27750, #41852, #21045, #34206, #17361, #6273, #2818, #2579, #34900, #16682, #2340, #16440, #41169, #27298, #24496, #6039, #44859, #38381, #24040, #20359, #30989, #42070, #9740, #3266, #23806, #30768, #6729, #10197, #31445, #30521, #37917, #45550, #34456, #45086, #13442, #13901, #27512, #44624, #12988, #27075, #41612, #10420, #38603, #6960, #9521, #9971, #23586, #38160, #37691, #6510, #20588, #34682, #3040, #17128, #31213, #45308, #13669, #18511, #43209, #39077, #28434, #7426, #39542, #35130, #32130, #7205, #495, #38853, #723, #11341, #15037, #4201, #21499, #28673, #32369, #17819, #7649, #42531, #3731, #24964, #7899, #35823, #11581, #39295, #257, #14821, #35577, #42976, #10896, #21277, #3955, #18048, #14600, #42752, #31887, #28894, #14354, #35357, #25420, #11113, #18293, #31665, #32591, #25660, #21972, #25183, #21728, #36058, #42290, #4422, #934, #29125, #39773, #8121, #3509, #17594, #32, #14125, #28197, #10653, #24734, #44107, #19624, #39982, #26550, #15938, #8788, #8567, #12471, #36949, #22394, #36498, #25871, #11802, #43434, #29578, #8331, #5302, #29793, #19398, #33483, #15498, #40648, #44334, #40436, #1169, #22856, #1829, #5528, #30022, #33057, #37169, #9001, #15710, #4862, #23071, #33719, #2068, #18963, #33265, #12689, #1394, #16160, #26091, #18729, #30242, #26769, #40874, #22182, #36276, #4633, #32817, #29364, #15278, #12024, #43654, #40205, #22633, #36731, #43873, #5089, #19180, #12252, #26332, #1611, #16625, #23750, #3210, #9912, #45495, #45033, #27244, #45253, #13612, #41114, #6461, #20074, #44567, #27461, #9466, #2519, #34396, #23529, #37411, #20304, #16386, #27929, #27696, #23309, #41336, #5768, #30940, #30712, #19856, #23984, #37631, #2767, #30465, #9686, #34149, #37865, #27015, #13852, #44808, #34845, #9238, #6211, #38332, #33936, #16860, #13389, #2287, #41800, #20755, #41559, #5982, #6678, #13165, #38105, #12928, #17300, #20539, #31155, #34633, #31390, #2990, #17077, #10149, #24224, #10841, #42244, #10370, #672, #35309, #25370, #18460, #4370 ) ),
 .UNSPECIFIED., .T., .F., .T. ) 
 B_SPLINE_SURFACE_WITH_KNOTS ( ( 4, 3, 4 ),
 ( 3, 2, 2, 2, 2, 2, 2, 2, 2, 2, 2, 2, 2, 2, 2, 2, 2, 2, 2, 2, 2, 2, 2, 2, 2, 2, 2, 2, 2, 2, 2, 2, 2, 2, 2, 2, 2, 2, 2, 2, 2, 2, 2, 2, 2, 2, 2, 2, 2, 2, 2, 2, 2, 2, 2, 2, 2, 2, 2, 2, 2, 2, 2, 2, 2, 2, 2, 2, 2, 2, 2, 2, 2, 2, 2, 2, 2, 2, 2, 2, 2, 2, 2, 2, 2, 2, 2, 2, 2, 2, 2, 2, 2, 2, 2, 2, 2, 2, 2, 2, 2, 2, 2, 2, 2, 2, 2, 2, 2, 2, 2, 2, 2, 2, 2, 2, 2, 2, 2, 2, 2, 2, 2, 2, 2, 2, 2, 2, 2, 2, 2, 2, 2, 2, 2, 2, 2, 2, 2, 2, 2, 2, 2, 2, 2, 2, 2, 2, 2, 2, 2, 2, 2, 2, 2, 2, 2, 2, 2, 2, 2, 2, 2, 2, 2, 2, 2, 2, 2, 2, 2, 2, 2, 2, 2, 2, 2, 2, 2, 2, 2, 2, 2, 2, 2, 2, 2, 2, 2, 2, 2, 2, 2, 2, 2, 2, 2, 2, 2, 2, 2, 2, 2, 2, 2, 2, 2, 2, 2, 2, 2, 2, 2, 2, 2, 2, 2, 2, 2, 2, 2, 2, 2, 2, 2, 2, 2, 2, 2, 2, 2, 2, 2, 2, 2, 2, 2, 2, 2, 2, 2, 2, 2, 2, 2, 2, 2, 2, 2, 2, 2, 2, 2, 2, 2, 2, 2, 2, 2, 2, 2, 2, 2, 2, 2, 2, 2, 2, 2, 2, 2, 2, 2, 2, 2, 2, 2, 2, 2, 2, 2, 2, 2, 2, 2, 2, 2, 2, 2, 2, 2, 2, 2, 2, 2, 2, 2, 2, 2, 2, 2, 2, 2, 2, 2, 2, 2, 2, 2, 2, 2, 2, 2, 2, 2, 2, 2, 2, 2, 2, 2, 2, 2, 2, 2, 2, 2, 2, 2, 2, 2, 2, 2, 2, 2, 2, 2, 2, 2, 2, 2, 2, 2, 2, 2, 2, 2, 2, 2, 2, 2, 2, 2, 2, 2, 2, 2, 2, 2, 2, 2, 2, 2, 2, 2, 2, 2, 2, 2, 2, 2, 2, 2, 2, 2, 2, 2, 2, 2, 2, 2, 2, 2, 2, 2, 2, 2, 2, 2, 2, 2, 2, 2, 2, 2, 2, 2, 2, 2, 2, 2, 2, 2, 2, 2, 2, 2, 2, 2, 2, 2, 2, 2, 2, 2, 2, 2, 2, 2, 2, 2, 2, 2, 2, 2, 2, 2, 2, 2, 2, 2, 3 ),
 ( 0.000000000000000000, 0.5000000000000000000, 1.000000000000000000 ),
 ( 0.000000000000000000, 0.002272727272727272617, 0.004545454545454545234, 0.006818181818181817851, 0.009090909090909090468, 0.01136363636363636395, 0.01363636363636363570, 0.01590909090909090745, 0.01818181818181818094, 0.02045454545454545442, 0.02272727272727272790, 0.02500000000000000139, 0.02727272727272727140, 0.02954545454545454489, 0.03181818181818181490, 0.03409090909090908839, 0.03636363636363636187, 0.03863636363636363535, 0.04090909090909090884, 0.04318181818181818232, 0.04545454545454545581, 0.04772727272727272929, 0.05000000000000000278, 0.05227272727272726932, 0.05454545454545454281, 0.05681818181818181629, 0.05909090909090908977, 0.06136363636363636326, 0.06363636363636362980, 0.06590909090909090329, 0.06818181818181817677, 0.07045454545454545026, 0.07272727272727272374, 0.07499999999999999722, 0.07727272727272727071, 0.07954545454545454419, 0.08181818181818181768, 0.08409090909090909116, 0.08636363636363636465, 0.08863636363636363813, 0.09090909090909091161, 0.09318181818181818510, 0.09545454545454545858, 0.09772727272727273207, 0.1000000000000000056, 0.1022727272727272790, 0.1045454545454545386, 0.1068181818181818121, 0.1090909090909090856, 0.1113636363636363591, 0.1136363636363636326, 0.1159090909090909061, 0.1181818181818181795, 0.1204545454545454530, 0.1227272727272727265, 0.1250000000000000000, 0.1272727272727272596, 0.1295454545454545470, 0.1318181818181818066, 0.1340909090909090939, 0.1363636363636363535, 0.1386363636363636409, 0.1409090909090909005, 0.1431818181818181879, 0.1454545454545454475, 0.1477272727272727348, 0.1499999999999999944, 0.1522727272727272818, 0.1545454545454545414, 0.1568181818181818288, 0.1590909090909090884, 0.1613636363636363757, 0.1636363636363636354, 0.1659090909090909227, 0.1681818181818181823, 0.1704545454545454419, 0.1727272727272727293, 0.1749999999999999889, 0.1772727272727272763, 0.1795454545454545359, 0.1818181818181818232, 0.1840909090909090828, 0.1863636363636363702, 0.1886363636363636298, 0.1909090909090909172, 0.1931818181818181768, 0.1954545454545454641, 0.1977272727272727237, 0.2000000000000000111, 0.2022727272727272707, 0.2045454545454545581, 0.2068181818181818177, 0.2090909090909090773, 0.2113636363636363646, 0.2136363636363636243, 0.2159090909090909116, 0.2181818181818181712, 0.2204545454545454586, 0.2227272727272727182, 0.2250000000000000056, 0.2272727272727272652, 0.2295454545454545525, 0.2318181818181818121, 0.2340909090909090995, 0.2363636363636363591, 0.2386363636363636465, 0.2409090909090909061, 0.2431818181818181934, 0.2454545454545454530, 0.2477272727272727404, 0.2500000000000000000, 0.2522727272727272596, 0.2545454545454545192, 0.2568181818181818343, 0.2590909090909090939, 0.2613636363636363535, 0.2636363636363636131, 0.2659090909090909283, 0.2681818181818181879, 0.2704545454545454475, 0.2727272727272727071, 0.2750000000000000222, 0.2772727272727272818, 0.2795454545454545414, 0.2818181818181818010, 0.2840909090909091161, 0.2863636363636363757, 0.2886363636363636354, 0.2909090909090908950, 0.2931818181818181546, 0.2954545454545454697, 0.2977272727272727293, 0.2999999999999999889, 0.3022727272727272485, 0.3045454545454545636, 0.3068181818181818232, 0.3090909090909090828, 0.3113636363636363424, 0.3136363636363636576, 0.3159090909090909172, 0.3181818181818181768, 0.3204545454545454364, 0.3227272727272727515, 0.3250000000000000111, 0.3272727272727272707, 0.3295454545454545303, 0.3318181818181818454, 0.3340909090909091050, 0.3363636363636363646, 0.3386363636363636243, 0.3409090909090908839, 0.3431818181818181990, 0.3454545454545454586, 0.3477272727272727182, 0.3499999999999999778, 0.3522727272727272929, 0.3545454545454545525, 0.3568181818181818121, 0.3590909090909090717, 0.3613636363636363869, 0.3636363636363636465, 0.3659090909090909061, 0.3681818181818181657, 0.3704545454545454808, 0.3727272727272727404, 0.3750000000000000000, 0.3772727272727272596, 0.3795454545454545192, 0.3818181818181818343, 0.3840909090909090939, 0.3863636363636363535, 0.3886363636363636131, 0.3909090909090909283, 0.3931818181818181879, 0.3954545454545454475, 0.3977272727272727071, 0.4000000000000000222, 0.4022727272727272818, 0.4045454545454545414, 0.4068181818181818010, 0.4090909090909091161, 0.4113636363636363757, 0.4136363636363636354, 0.4159090909090908950, 0.4181818181818181546, 0.4204545454545454697, 0.4227272727272727293, 0.4249999999999999889, 0.4272727272727272485, 0.4295454545454545636, 0.4318181818181818232, 0.4340909090909090828, 0.4363636363636363424, 0.4386363636363636576, 0.4409090909090909172, 0.4431818181818181768, 0.4454545454545454364, 0.4477272727272727515, 0.4500000000000000111, 0.4522727272727272707, 0.4545454545454545303, 0.4568181818181818454, 0.4590909090909091050, 0.4613636363636363646, 0.4636363636363636243, 0.4659090909090908839, 0.4681818181818181990, 0.4704545454545454586, 0.4727272727272727182, 0.4749999999999999778, 0.4772727272727272929, 0.4795454545454545525, 0.4818181818181818121, 0.4840909090909090717, 0.4863636363636363869, 0.4886363636363636465, 0.4909090909090909061, 0.4931818181818181657, 0.4954545454545454808, 0.4977272727272727404, 0.5000000000000000000, 0.5022727272727273151, 0.5045454545454545192, 0.5068181818181818343, 0.5090909090909090384, 0.5113636363636363535, 0.5136363636363636687, 0.5159090909090908728, 0.5181818181818181879, 0.5204545454545455030, 0.5227272727272727071, 0.5250000000000000222, 0.5272727272727272263, 0.5295454545454545414, 0.5318181818181818565, 0.5340909090909090606, 0.5363636363636363757, 0.5386363636363636909, 0.5409090909090908950, 0.5431818181818182101, 0.5454545454545454142, 0.5477272727272727293, 0.5500000000000000444, 0.5522727272727272485, 0.5545454545454545636, 0.5568181818181817677, 0.5590909090909090828, 0.5613636363636363980, 0.5636363636363636020, 0.5659090909090909172, 0.5681818181818182323, 0.5704545454545454364, 0.5727272727272727515, 0.5749999999999999556, 0.5772727272727272707, 0.5795454545454545858, 0.5818181818181817899, 0.5840909090909091050, 0.5863636363636363091, 0.5886363636363636243, 0.5909090909090909394, 0.5931818181818181435, 0.5954545454545454586, 0.5977272727272727737, 0.5999999999999999778, 0.6022727272727272929, 0.6045454545454544970, 0.6068181818181818121, 0.6090909090909091272, 0.6113636363636363313, 0.6136363636363636465, 0.6159090909090909616, 0.6181818181818181657, 0.6204545454545454808, 0.6227272727272726849, 0.6250000000000000000, 0.6272727272727273151, 0.6295454545454545192, 0.6318181818181818343, 0.6340909090909090384, 0.6363636363636363535, 0.6386363636363636687, 0.6409090909090908728, 0.6431818181818181879, 0.6454545454545455030, 0.6477272727272727071, 0.6500000000000000222, 0.6522727272727272263, 0.6545454545454545414, 0.6568181818181818565, 0.6590909090909090606, 0.6613636363636363757, 0.6636363636363636909, 0.6659090909090908950, 0.6681818181818182101, 0.6704545454545454142, 0.6727272727272727293, 0.6750000000000000444, 0.6772727272727272485, 0.6795454545454545636, 0.6818181818181817677, 0.6840909090909090828, 0.6863636363636363980, 0.6886363636363636020, 0.6909090909090909172, 0.6931818181818182323, 0.6954545454545454364, 0.6977272727272727515, 0.6999999999999999556, 0.7022727272727272707, 0.7045454545454545858, 0.7068181818181817899, 0.7090909090909091050, 0.7113636363636363091, 0.7136363636363636243, 0.7159090909090909394, 0.7181818181818181435, 0.7204545454545454586, 0.7227272727272727737, 0.7249999999999999778, 0.7272727272727272929, 0.7295454545454544970, 0.7318181818181818121, 0.7340909090909091272, 0.7363636363636363313, 0.7386363636363636465, 0.7409090909090909616, 0.7431818181818181657, 0.7454545454545454808, 0.7477272727272726849, 0.7500000000000000000, 0.7522727272727273151, 0.7545454545454545192, 0.7568181818181818343, 0.7590909090909090384, 0.7613636363636363535, 0.7636363636363636687, 0.7659090909090908728, 0.7681818181818181879, 0.7704545454545455030, 0.7727272727272727071, 0.7750000000000000222, 0.7772727272727272263, 0.7795454545454545414, 0.7818181818181818565, 0.7840909090909090606, 0.7863636363636363757, 0.7886363636363636909, 0.7909090909090908950, 0.7931818181818182101, 0.7954545454545454142, 0.7977272727272727293, 0.8000000000000000444, 0.8022727272727272485, 0.8045454545454545636, 0.8068181818181817677, 0.8090909090909090828, 0.8113636363636363980, 0.8136363636363636020, 0.8159090909090909172, 0.8181818181818182323, 0.8204545454545454364, 0.8227272727272727515, 0.8249999999999999556, 0.8272727272727272707, 0.8295454545454545858, 0.8318181818181817899, 0.8340909090909091050, 0.8363636363636363091, 0.8386363636363636243, 0.8409090909090909394, 0.8431818181818181435, 0.8454545454545454586, 0.8477272727272727737, 0.8499999999999999778, 0.8522727272727272929, 0.8545454545454544970, 0.8568181818181818121, 0.8590909090909091272, 0.8613636363636363313, 0.8636363636363636465, 0.8659090909090909616, 0.8681818181818181657, 0.8704545454545454808, 0.8727272727272726849, 0.8750000000000000000, 0.8772727272727273151, 0.8795454545454545192, 0.8818181818181818343, 0.8840909090909090384, 0.8863636363636363535, 0.8886363636363636687, 0.8909090909090908728, 0.8931818181818181879, 0.8954545454545455030, 0.8977272727272727071, 0.9000000000000000222, 0.9022727272727272263, 0.9045454545454545414, 0.9068181818181818565, 0.9090909090909090606, 0.9113636363636363757, 0.9136363636363636909, 0.9159090909090908950, 0.9181818181818182101, 0.9204545454545454142, 0.9227272727272727293, 0.9250000000000000444, 0.9272727272727272485, 0.9295454545454545636, 0.9318181818181817677, 0.9340909090909090828, 0.9363636363636363980, 0.9386363636363636020, 0.9409090909090909172, 0.9431818181818182323, 0.9454545454545454364, 0.9477272727272727515, 0.9499999999999999556, 0.9522727272727272707, 0.9545454545454545858, 0.9568181818181817899, 0.9590909090909091050, 0.9613636363636363091, 0.9636363636363636243, 0.9659090909090909394, 0.9681818181818181435, 0.9704545454545454586, 0.9727272727272727737, 0.9749999999999999778, 0.9772727272727272929, 0.9781254700864303597 ),
 .UNSPECIFIED. ) 
 GEOMETRIC_REPRESENTATION_ITEM ( )  RATIONAL_B_SPLINE_SURFACE ( (
 ( 1.000000000000000000, 0.9898214418809326842, 1.000000000000000000, 0.9898214418809326842, 1.000000000000000000, 0.9898214418809326842, 1.000000000000000000, 0.9898214418809326842, 1.000000000000000000, 0.9898214418809326842, 1.000000000000000000, 0.9898214418809326842, 1.000000000000000000, 0.9898214418809326842, 1.000000000000000000, 0.9898214418809326842, 1.000000000000000000, 0.9898214418809326842, 1.000000000000000000, 0.9898214418809326842, 1.000000000000000000, 0.9898214418809326842, 1.000000000000000000, 0.9898214418809326842, 1.000000000000000000, 0.9898214418809326842, 1.000000000000000000, 0.9898214418809326842, 1.000000000000000000, 0.9898214418809326842, 1.000000000000000000, 0.9898214418809326842, 1.000000000000000000, 0.9898214418809326842, 1.000000000000000000, 0.9898214418809326842, 1.000000000000000000, 0.9898214418809326842, 1.000000000000000000, 0.9898214418809326842, 1.000000000000000000, 0.9898214418809326842, 1.000000000000000000, 0.9898214418809326842, 1.000000000000000000, 0.9898214418809326842, 1.000000000000000000, 0.9898214418809326842, 1.000000000000000000, 0.9898214418809326842, 1.000000000000000000, 0.9898214418809326842, 1.000000000000000000, 0.9898214418809326842, 1.000000000000000000, 0.9898214418809326842, 1.000000000000000000, 0.9898214418809326842, 1.000000000000000000, 0.9898214418809326842, 1.000000000000000000, 0.9898214418809326842, 1.000000000000000000, 0.9898214418809326842, 1.000000000000000000, 0.9898214418809326842, 1.000000000000000000, 0.9898214418809326842, 1.000000000000000000, 0.9898214418809326842, 1.000000000000000000, 0.9898214418809326842, 1.000000000000000000, 0.9898214418809326842, 1.000000000000000000, 0.9898214418809326842, 1.000000000000000000, 0.9898214418809326842, 1.000000000000000000, 0.9898214418809326842, 1.000000000000000000, 0.9898214418809326842, 1.000000000000000000, 0.9898214418809326842, 1.000000000000000000, 0.9898214418809326842, 1.000000000000000000, 0.9898214418809326842, 1.000000000000000000, 0.9898214418809326842, 1.000000000000000000, 0.9898214418809326842, 1.000000000000000000, 0.9898214418809326842, 1.000000000000000000, 0.9898214418809326842, 1.000000000000000000, 0.9898214418809326842, 1.000000000000000000, 0.9898214418809326842, 1.000000000000000000, 0.9898214418809326842, 1.000000000000000000, 0.9898214418809326842, 1.000000000000000000, 0.9898214418809326842, 1.000000000000000000, 0.9898214418809326842, 1.000000000000000000, 0.9898214418809326842, 1.000000000000000000, 0.9898214418809326842, 1.000000000000000000, 0.9898214418809326842, 1.000000000000000000, 0.9898214418809326842, 1.000000000000000000, 0.9898214418809326842, 1.000000000000000000, 0.9898214418809326842, 1.000000000000000000, 0.9898214418809326842, 1.000000000000000000, 0.9898214418809326842, 1.000000000000000000, 0.9898214418809326842, 1.000000000000000000, 0.9898214418809326842, 1.000000000000000000, 0.9898214418809326842, 1.000000000000000000, 0.9898214418809326842, 1.000000000000000000, 0.9898214418809326842, 1.000000000000000000, 0.9898214418809326842, 1.000000000000000000, 0.9898214418809326842, 1.000000000000000000, 0.9898214418809326842, 1.000000000000000000, 0.9898214418809326842, 1.000000000000000000, 0.9898214418809326842, 1.000000000000000000, 0.9898214418809326842, 1.000000000000000000, 0.9898214418809326842, 1.000000000000000000, 0.9898214418809326842, 1.000000000000000000, 0.9898214418809326842, 1.000000000000000000, 0.9898214418809326842, 1.000000000000000000, 0.9898214418809326842, 1.000000000000000000, 0.9898214418809326842, 1.000000000000000000, 0.9898214418809326842, 1.000000000000000000, 0.9898214418809326842, 1.000000000000000000, 0.9898214418809326842, 1.000000000000000000, 0.9898214418809326842, 1.000000000000000000, 0.9898214418809326842, 1.000000000000000000, 0.9898214418809326842, 1.000000000000000000, 0.9898214418809326842, 1.000000000000000000, 0.9898214418809326842, 1.000000000000000000, 0.9898214418809326842, 1.000000000000000000, 0.9898214418809326842, 1.000000000000000000, 0.9898214418809326842, 1.000000000000000000, 0.9898214418809326842, 1.000000000000000000, 0.9898214418809326842, 1.000000000000000000, 0.9898214418809326842, 1.000000000000000000, 0.9898214418809326842, 1.000000000000000000, 0.9898214418809326842, 1.000000000000000000, 0.9898214418809326842, 1.000000000000000000, 0.9898214418809326842, 1.000000000000000000, 0.9898214418809326842, 1.000000000000000000, 0.9898214418809326842, 1.000000000000000000, 0.9898214418809326842, 1.000000000000000000, 0.9898214418809326842, 1.000000000000000000, 0.9898214418809326842, 1.000000000000000000, 0.9898214418809326842, 1.000000000000000000, 0.9898214418809326842, 1.000000000000000000, 0.9898214418809326842, 1.000000000000000000, 0.9898214418809326842, 1.000000000000000000, 0.9898214418809326842, 1.000000000000000000, 0.9898214418809326842, 1.000000000000000000, 0.9898214418809326842, 1.000000000000000000, 0.9898214418809326842, 1.000000000000000000, 0.9898214418809326842, 1.000000000000000000, 0.9898214418809326842, 1.000000000000000000, 0.9898214418809326842, 1.000000000000000000, 0.9898214418809326842, 1.000000000000000000, 0.9898214418809326842, 1.000000000000000000, 0.9898214418809326842, 1.000000000000000000, 0.9898214418809326842, 1.000000000000000000, 0.9898214418809326842, 1.000000000000000000, 0.9898214418809326842, 1.000000000000000000, 0.9898214418809326842, 1.000000000000000000, 0.9898214418809326842, 1.000000000000000000, 0.9898214418809326842, 1.000000000000000000, 0.9898214418809326842, 1.000000000000000000, 0.9898214418809326842, 1.000000000000000000, 0.9898214418809326842, 1.000000000000000000, 0.9898214418809326842, 1.000000000000000000, 0.9898214418809326842, 1.000000000000000000, 0.9898214418809326842, 1.000000000000000000, 0.9898214418809326842, 1.000000000000000000, 0.9898214418809326842, 1.000000000000000000, 0.9898214418809326842, 1.000000000000000000, 0.9898214418809326842, 1.000000000000000000, 0.9898214418809326842, 1.000000000000000000, 0.9898214418809326842, 1.000000000000000000, 0.9898214418809326842, 1.000000000000000000, 0.9898214418809326842, 1.000000000000000000, 0.9898214418809326842, 1.000000000000000000, 0.9898214418809326842, 1.000000000000000000, 0.9898214418809326842, 1.000000000000000000, 0.9898214418809326842, 1.000000000000000000, 0.9898214418809326842, 1.000000000000000000, 0.9898214418809326842, 1.000000000000000000, 0.9898214418809326842, 1.000000000000000000, 0.9898214418809326842, 1.000000000000000000, 0.9898214418809326842, 1.000000000000000000, 0.9898214418809326842, 1.000000000000000000, 0.9898214418809326842, 1.000000000000000000, 0.9898214418809326842, 1.000000000000000000, 0.9898214418809326842, 1.000000000000000000, 0.9898214418809326842, 1.000000000000000000, 0.9898214418809326842, 1.000000000000000000, 0.9898214418809326842, 1.000000000000000000, 0.9898214418809326842, 1.000000000000000000, 0.9898214418809326842, 1.000000000000000000, 0.9898214418809326842, 1.000000000000000000, 0.9898214418809326842, 1.000000000000000000, 0.9898214418809326842, 1.000000000000000000, 0.9898214418809326842, 1.000000000000000000, 0.9898214418809326842, 1.000000000000000000, 0.9898214418809326842, 1.000000000000000000, 0.9898214418809326842, 1.000000000000000000, 0.9898214418809326842, 1.000000000000000000, 0.9898214418809326842, 1.000000000000000000, 0.9898214418809326842, 1.000000000000000000, 0.9898214418809326842, 1.000000000000000000, 0.9898214418809326842, 1.000000000000000000, 0.9898214418809326842, 1.000000000000000000, 0.9898214418809326842, 1.000000000000000000, 0.9898214418809326842, 1.000000000000000000, 0.9898214418809326842, 1.000000000000000000, 0.9898214418809326842, 1.000000000000000000, 0.9898214418809326842, 1.000000000000000000, 0.9898214418809326842, 1.000000000000000000, 0.9898214418809326842, 1.000000000000000000, 0.9898214418809326842, 1.000000000000000000, 0.9898214418809326842, 1.000000000000000000, 0.9898214418809326842, 1.000000000000000000, 0.9898214418809326842, 1.000000000000000000, 0.9898214418809326842, 1.000000000000000000, 0.9898214418809326842, 1.000000000000000000, 0.9898214418809326842, 1.000000000000000000, 0.9898214418809326842, 1.000000000000000000, 0.9898214418809326842, 1.000000000000000000, 0.9898214418809326842, 1.000000000000000000, 0.9898214418809326842, 1.000000000000000000, 0.9898214418809326842, 1.000000000000000000, 0.9898214418809326842, 1.000000000000000000, 0.9898214418809326842, 1.000000000000000000, 0.9898214418809326842, 1.000000000000000000, 0.9898214418809326842, 1.000000000000000000, 0.9898214418809326842, 1.000000000000000000, 0.9898214418809326842, 1.000000000000000000, 0.9898214418809326842, 1.000000000000000000, 0.9898214418809326842, 1.000000000000000000, 0.9898214418809326842, 1.000000000000000000, 0.9898214418809326842, 1.000000000000000000, 0.9898214418809326842, 1.000000000000000000, 0.9898214418809326842, 1.000000000000000000, 0.9898214418809326842, 1.000000000000000000, 0.9898214418809326842, 1.000000000000000000, 0.9898214418809326842, 1.000000000000000000, 0.9898214418809326842, 1.000000000000000000, 0.9898214418809326842, 1.000000000000000000, 0.9898214418809326842, 1.000000000000000000, 0.9898214418809326842, 1.000000000000000000, 0.9898214418809326842, 1.000000000000000000, 0.9898214418809326842, 1.000000000000000000, 0.9898214418809326842, 1.000000000000000000, 0.9898214418809326842, 1.000000000000000000, 0.9898214418809326842, 1.000000000000000000, 0.9898214418809326842, 1.000000000000000000, 0.9898214418809326842, 1.000000000000000000, 0.9898214418809326842, 1.000000000000000000, 0.9898214418809326842, 1.000000000000000000, 0.9898214418809326842, 1.000000000000000000, 0.9898214418809326842, 1.000000000000000000, 0.9898214418809326842, 1.000000000000000000, 0.9898214418809326842, 1.000000000000000000, 0.9898214418809326842, 1.000000000000000000, 0.9898214418809326842, 1.000000000000000000, 0.9898214418809326842, 1.000000000000000000, 0.9898214418809326842, 1.000000000000000000, 0.9898214418809326842, 1.000000000000000000, 0.9898214418809326842, 1.000000000000000000, 0.9898214418809326842, 1.000000000000000000, 0.9898214418809326842, 1.000000000000000000, 0.9898214418809326842, 1.000000000000000000, 0.9898214418809326842, 1.000000000000000000, 0.9898214418809326842, 1.000000000000000000, 0.9898214418809326842, 1.000000000000000000, 0.9898214418809326842, 1.000000000000000000, 0.9898214418809326842, 1.000000000000000000, 0.9898214418809326842, 1.000000000000000000, 0.9898214418809326842, 1.000000000000000000, 0.9898214418809326842, 1.000000000000000000, 0.9898214418809326842, 1.000000000000000000, 0.9898214418809326842, 1.000000000000000000, 0.9898214418809326842, 1.000000000000000000, 0.9898214418809326842, 1.000000000000000000, 0.9898214418809326842, 1.000000000000000000, 0.9898214418809326842, 1.000000000000000000, 0.9898214418809326842, 1.000000000000000000, 0.9898214418809326842, 1.000000000000000000, 0.9898214418809326842, 1.000000000000000000, 0.9898214418809326842, 1.000000000000000000, 0.9898214418809326842, 1.000000000000000000, 0.9898214418809326842, 1.000000000000000000, 0.9898214418809326842, 1.000000000000000000, 0.9898214418809326842, 1.000000000000000000, 0.9898214418809326842, 1.000000000000000000, 0.9898214418809326842, 1.000000000000000000, 0.9898214418809326842, 1.000000000000000000, 0.9898214418809326842, 1.000000000000000000, 0.9898214418809326842, 1.000000000000000000, 0.9898214418809326842, 1.000000000000000000, 0.9898214418809326842, 1.000000000000000000, 0.9898214418809326842, 1.000000000000000000, 0.9898214418809326842, 1.000000000000000000, 0.9898214418809326842, 1.000000000000000000, 0.9898214418809326842, 1.000000000000000000, 0.9898214418809326842, 1.000000000000000000, 0.9898214418809326842, 1.000000000000000000, 0.9898214418809326842, 1.000000000000000000, 0.9898214418809326842, 1.000000000000000000, 0.9898214418809326842, 1.000000000000000000, 0.9898214418809326842, 1.000000000000000000, 0.9898214418809326842, 1.000000000000000000, 0.9898214418809326842, 1.000000000000000000, 0.9898214418809326842, 1.000000000000000000, 0.9898214418809326842, 1.000000000000000000, 0.9898214418809326842, 1.000000000000000000, 0.9898214418809326842, 1.000000000000000000, 0.9898214418809326842, 1.000000000000000000, 0.9898214418809326842, 1.000000000000000000, 0.9898214418809326842, 1.000000000000000000, 0.9898214418809326842, 1.000000000000000000, 0.9898214418809326842, 1.000000000000000000, 0.9898214418809326842, 1.000000000000000000, 0.9898214418809326842, 1.000000000000000000, 0.9898214418809326842, 1.000000000000000000, 0.9898214418809326842, 1.000000000000000000, 0.9898214418809326842, 1.000000000000000000, 0.9898214418809326842, 1.000000000000000000, 0.9898214418809326842, 1.000000000000000000, 0.9898214418809326842, 1.000000000000000000, 0.9898214418809326842, 1.000000000000000000, 0.9898214418809326842, 1.000000000000000000, 0.9898214418809326842, 1.000000000000000000, 0.9898214418809326842, 1.000000000000000000, 0.9898214418809326842, 1.000000000000000000, 0.9898214418809326842, 1.000000000000000000, 0.9898214418809326842, 1.000000000000000000, 0.9898214418809326842, 1.000000000000000000, 0.9898214418809326842, 1.000000000000000000, 0.9898214418809326842, 1.000000000000000000, 0.9898214418809326842, 1.000000000000000000, 0.9898214418809326842, 1.000000000000000000, 0.9898214418809326842, 1.000000000000000000, 0.9898214418809326842, 1.000000000000000000, 0.9898214418809326842, 1.000000000000000000, 0.9898214418809326842, 1.000000000000000000, 0.9898214418809326842, 1.000000000000000000, 0.9898214418809326842, 1.000000000000000000, 0.9898214418809326842, 1.000000000000000000, 0.9898214418809326842, 1.000000000000000000, 0.9898214418809326842, 1.000000000000000000, 0.9898214418809326842, 1.000000000000000000, 0.9898214418809326842, 1.000000000000000000, 0.9898214418809326842, 1.000000000000000000, 0.9898214418809326842, 1.000000000000000000, 0.9898214418809326842, 1.000000000000000000, 0.9898214418809326842, 1.000000000000000000, 0.9898214418809326842, 1.000000000000000000, 0.9898214418809326842, 1.000000000000000000, 0.9898214418809326842, 1.000000000000000000, 0.9898214418809326842, 1.000000000000000000, 0.9898214418809326842, 1.000000000000000000, 0.9898214418809326842, 1.000000000000000000, 0.9898214418809326842, 1.000000000000000000, 0.9898214418809326842, 1.000000000000000000, 0.9898214418809326842, 1.000000000000000000, 0.9898214418809326842, 1.000000000000000000, 0.9898214418809326842, 1.000000000000000000, 0.9898214418809326842, 1.000000000000000000, 0.9898214418809326842, 1.000000000000000000, 0.9898214418809326842, 1.000000000000000000, 0.9898214418809326842, 1.000000000000000000, 0.9898214418809326842, 1.000000000000000000, 0.9898214418809326842, 1.000000000000000000, 0.9898214418809326842, 1.000000000000000000, 0.9898214418809326842, 1.000000000000000000, 0.9898214418809326842, 1.000000000000000000, 0.9898214418809326842, 1.000000000000000000, 0.9898214418809326842, 1.000000000000000000, 0.9898214418809326842, 1.000000000000000000, 0.9898214418809326842, 1.000000000000000000, 0.9898214418809326842, 1.000000000000000000, 0.9898214418809326842, 1.000000000000000000, 0.9898214418809326842, 1.000000000000000000, 0.9898214418809326842, 1.000000000000000000, 0.9898214418809326842, 1.000000000000000000, 0.9898214418809326842, 1.000000000000000000, 0.9898214418809326842, 1.000000000000000000, 0.9898214418809326842, 1.000000000000000000, 0.9898214418809326842, 1.000000000000000000, 0.9898214418809326842, 1.000000000000000000, 0.9898214418809326842, 1.000000000000000000, 0.9898214418809326842, 1.000000000000000000, 0.9898214418809326842, 1.000000000000000000, 0.9898214418809326842, 1.000000000000000000, 0.9898214418809326842, 1.000000000000000000, 0.9898214418809326842, 1.000000000000000000, 0.9898214418809326842, 1.000000000000000000, 0.9898214418809326842, 1.000000000000000000, 0.9898214418809326842, 1.000000000000000000, 0.9898214418809326842, 1.000000000000000000, 0.9898214418809326842, 1.000000000000000000, 0.9898214418809326842, 1.000000000000000000, 0.9898214418809326842, 1.000000000000000000, 0.9898214418809326842, 1.000000000000000000, 0.9898214418809326842, 1.000000000000000000, 0.9898214418809326842, 1.000000000000000000, 0.9898214418809326842, 1.000000000000000000, 0.9898214418809326842, 1.000000000000000000, 0.9898214418809326842, 1.000000000000000000, 0.9898214418809326842, 1.000000000000000000, 0.9898214418809326842, 1.000000000000000000, 0.9898214418809326842, 1.000000000000000000, 0.9898214418809326842, 1.000000000000000000, 0.9898214418809326842, 1.000000000000000000, 0.9898214418809326842, 1.000000000000000000, 0.9898214418809326842, 1.000000000000000000, 0.9898214418809326842, 1.000000000000000000, 0.9898214418809326842, 1.000000000000000000, 0.9898214418809326842, 1.000000000000000000, 0.9898214418809326842, 1.000000000000000000, 0.9898214418809326842, 1.000000000000000000, 0.9898214418809326842, 1.000000000000000000, 0.9898214418809326842, 1.000000000000000000, 0.9898214418809326842, 1.000000000000000000, 0.9898214418809326842, 1.000000000000000000, 0.9898214418809326842, 1.000000000000000000, 0.9898214418809326842, 1.000000000000000000, 0.9898214418809326842, 1.000000000000000000, 0.9898214418809326842, 1.000000000000000000, 0.9898214418809326842, 1.000000000000000000, 0.9898214418809326842, 1.000000000000000000, 0.9898214418809326842, 1.000000000000000000, 0.9898214418809326842, 1.000000000000000000, 0.9898214418809326842, 1.000000000000000000, 0.9898214418809326842, 1.000000000000000000, 0.9898214418809326842, 1.000000000000000000, 0.9898214418809326842, 1.000000000000000000, 0.9898214418809326842, 1.000000000000000000, 0.9898214418809326842, 1.000000000000000000, 0.9898214418809326842, 1.000000000000000000, 0.9898214418809326842, 1.000000000000000000, 0.9898214418809326842, 1.000000000000000000, 0.9898214418809326842, 1.000000000000000000, 0.9898214418809326842, 1.000000000000000000, 0.9898214418809326842, 1.000000000000000000, 0.9898214418809326842, 1.000000000000000000, 0.9898214418809326842, 1.000000000000000000, 0.9898214418809326842, 1.000000000000000000, 0.9898214418809326842, 1.000000000000000000, 0.9898214418809326842, 1.000000000000000000, 0.9898214418809326842, 1.000000000000000000, 0.9898214418809326842, 1.000000000000000000, 0.9898214418809326842, 1.000000000000000000, 0.9898214418809326842, 1.000000000000000000, 0.9898214418809326842, 1.000000000000000000, 0.9898214418809326842, 1.000000000000000000, 0.9898214418809326842, 1.000000000000000000, 0.9898214418809326842, 1.000000000000000000, 0.9898214418809326842, 1.000000000000000000, 0.9898214418809326842, 1.000000000000000000, 0.9898214418809326842, 1.000000000000000000, 0.9898214418809326842, 1.000000000000000000, 0.9898214418809326842, 1.000000000000000000, 0.9898214418809326842, 1.000000000000000000, 0.9898214418809326842, 1.000000000000000000, 0.9898214418809326842, 1.000000000000000000, 0.9898214418809326842, 1.000000000000000000, 0.9898214418809326842, 1.000000000000000000, 0.9898214418809326842, 1.000000000000000000, 0.9898214418809326842, 1.000000000000000000, 0.9898214418809326842, 1.000000000000000000, 0.9898214418809326842, 1.000000000000000000, 0.9898214418809326842, 1.000000000000000000, 0.9898214418809326842, 1.000000000000000000, 0.9961809353924466759, 0.9952277490961531914),
 ( 0.3333333333333333703, 0.3299404806269776169, 0.3333333333333333703, 0.3299404806269776169, 0.3333333333333333703, 0.3299404806269776169, 0.3333333333333333703, 0.3299404806269776169, 0.3333333333333333703, 0.3299404806269776169, 0.3333333333333333703, 0.3299404806269776169, 0.3333333333333333703, 0.3299404806269776169, 0.3333333333333333703, 0.3299404806269776169, 0.3333333333333333703, 0.3299404806269776169, 0.3333333333333333703, 0.3299404806269776169, 0.3333333333333333703, 0.3299404806269776169, 0.3333333333333333703, 0.3299404806269776169, 0.3333333333333333703, 0.3299404806269776169, 0.3333333333333333703, 0.3299404806269776169, 0.3333333333333333703, 0.3299404806269776169, 0.3333333333333333703, 0.3299404806269776169, 0.3333333333333333703, 0.3299404806269776169, 0.3333333333333333703, 0.3299404806269776169, 0.3333333333333333703, 0.3299404806269776169, 0.3333333333333333703, 0.3299404806269776169, 0.3333333333333333703, 0.3299404806269776169, 0.3333333333333333703, 0.3299404806269776169, 0.3333333333333333703, 0.3299404806269776169, 0.3333333333333333703, 0.3299404806269776169, 0.3333333333333333703, 0.3299404806269776169, 0.3333333333333333703, 0.3299404806269776169, 0.3333333333333333703, 0.3299404806269776169, 0.3333333333333333703, 0.3299404806269776169, 0.3333333333333333703, 0.3299404806269776169, 0.3333333333333333703, 0.3299404806269776169, 0.3333333333333333703, 0.3299404806269776169, 0.3333333333333333703, 0.3299404806269776169, 0.3333333333333333703, 0.3299404806269776169, 0.3333333333333333703, 0.3299404806269776169, 0.3333333333333333703, 0.3299404806269776169, 0.3333333333333333703, 0.3299404806269776169, 0.3333333333333333703, 0.3299404806269776169, 0.3333333333333333703, 0.3299404806269776169, 0.3333333333333333703, 0.3299404806269776169, 0.3333333333333333703, 0.3299404806269776169, 0.3333333333333333703, 0.3299404806269776169, 0.3333333333333333703, 0.3299404806269776169, 0.3333333333333333703, 0.3299404806269776169, 0.3333333333333333703, 0.3299404806269776169, 0.3333333333333333703, 0.3299404806269776169, 0.3333333333333333703, 0.3299404806269776169, 0.3333333333333333703, 0.3299404806269776169, 0.3333333333333333703, 0.3299404806269776169, 0.3333333333333333703, 0.3299404806269776169, 0.3333333333333333703, 0.3299404806269776169, 0.3333333333333333703, 0.3299404806269776169, 0.3333333333333333703, 0.3299404806269776169, 0.3333333333333333703, 0.3299404806269776169, 0.3333333333333333703, 0.3299404806269776169, 0.3333333333333333703, 0.3299404806269776169, 0.3333333333333333703, 0.3299404806269776169, 0.3333333333333333703, 0.3299404806269776169, 0.3333333333333333703, 0.3299404806269776169, 0.3333333333333333703, 0.3299404806269776169, 0.3333333333333333703, 0.3299404806269776169, 0.3333333333333333703, 0.3299404806269776169, 0.3333333333333333703, 0.3299404806269776169, 0.3333333333333333703, 0.3299404806269776169, 0.3333333333333333703, 0.3299404806269776169, 0.3333333333333333703, 0.3299404806269776169, 0.3333333333333333703, 0.3299404806269776169, 0.3333333333333333703, 0.3299404806269776169, 0.3333333333333333703, 0.3299404806269776169, 0.3333333333333333703, 0.3299404806269776169, 0.3333333333333333703, 0.3299404806269776169, 0.3333333333333333703, 0.3299404806269776169, 0.3333333333333333703, 0.3299404806269776169, 0.3333333333333333703, 0.3299404806269776169, 0.3333333333333333703, 0.3299404806269776169, 0.3333333333333333703, 0.3299404806269776169, 0.3333333333333333703, 0.3299404806269776169, 0.3333333333333333703, 0.3299404806269776169, 0.3333333333333333703, 0.3299404806269776169, 0.3333333333333333703, 0.3299404806269776169, 0.3333333333333333703, 0.3299404806269776169, 0.3333333333333333703, 0.3299404806269776169, 0.3333333333333333703, 0.3299404806269776169, 0.3333333333333333703, 0.3299404806269776169, 0.3333333333333333703, 0.3299404806269776169, 0.3333333333333333703, 0.3299404806269776169, 0.3333333333333333703, 0.3299404806269776169, 0.3333333333333333703, 0.3299404806269776169, 0.3333333333333333703, 0.3299404806269776169, 0.3333333333333333703, 0.3299404806269776169, 0.3333333333333333703, 0.3299404806269776169, 0.3333333333333333703, 0.3299404806269776169, 0.3333333333333333703, 0.3299404806269776169, 0.3333333333333333703, 0.3299404806269776169, 0.3333333333333333703, 0.3299404806269776169, 0.3333333333333333703, 0.3299404806269776169, 0.3333333333333333703, 0.3299404806269776169, 0.3333333333333333703, 0.3299404806269776169, 0.3333333333333333703, 0.3299404806269776169, 0.3333333333333333703, 0.3299404806269776169, 0.3333333333333333703, 0.3299404806269776169, 0.3333333333333333703, 0.3299404806269776169, 0.3333333333333333703, 0.3299404806269776169, 0.3333333333333333703, 0.3299404806269776169, 0.3333333333333333703, 0.3299404806269776169, 0.3333333333333333703, 0.3299404806269776169, 0.3333333333333333703, 0.3299404806269776169, 0.3333333333333333703, 0.3299404806269776169, 0.3333333333333333703, 0.3299404806269776169, 0.3333333333333333703, 0.3299404806269776169, 0.3333333333333333703, 0.3299404806269776169, 0.3333333333333333703, 0.3299404806269776169, 0.3333333333333333703, 0.3299404806269776169, 0.3333333333333333703, 0.3299404806269776169, 0.3333333333333333703, 0.3299404806269776169, 0.3333333333333333703, 0.3299404806269776169, 0.3333333333333333703, 0.3299404806269776169, 0.3333333333333333703, 0.3299404806269776169, 0.3333333333333333703, 0.3299404806269776169, 0.3333333333333333703, 0.3299404806269776169, 0.3333333333333333703, 0.3299404806269776169, 0.3333333333333333703, 0.3299404806269776169, 0.3333333333333333703, 0.3299404806269776169, 0.3333333333333333703, 0.3299404806269776169, 0.3333333333333333703, 0.3299404806269776169, 0.3333333333333333703, 0.3299404806269776169, 0.3333333333333333703, 0.3299404806269776169, 0.3333333333333333703, 0.3299404806269776169, 0.3333333333333333703, 0.3299404806269776169, 0.3333333333333333703, 0.3299404806269776169, 0.3333333333333333703, 0.3299404806269776169, 0.3333333333333333703, 0.3299404806269776169, 0.3333333333333333703, 0.3299404806269776169, 0.3333333333333333703, 0.3299404806269776169, 0.3333333333333333703, 0.3299404806269776169, 0.3333333333333333703, 0.3299404806269776169, 0.3333333333333333703, 0.3299404806269776169, 0.3333333333333333703, 0.3299404806269776169, 0.3333333333333333703, 0.3299404806269776169, 0.3333333333333333703, 0.3299404806269776169, 0.3333333333333333703, 0.3299404806269776169, 0.3333333333333333703, 0.3299404806269776169, 0.3333333333333333703, 0.3299404806269776169, 0.3333333333333333703, 0.3299404806269776169, 0.3333333333333333703, 0.3299404806269776169, 0.3333333333333333703, 0.3299404806269776169, 0.3333333333333333703, 0.3299404806269776169, 0.3333333333333333703, 0.3299404806269776169, 0.3333333333333333703, 0.3299404806269776169, 0.3333333333333333703, 0.3299404806269776169, 0.3333333333333333703, 0.3299404806269776169, 0.3333333333333333703, 0.3299404806269776169, 0.3333333333333333703, 0.3299404806269776169, 0.3333333333333333703, 0.3299404806269776169, 0.3333333333333333703, 0.3299404806269776169, 0.3333333333333333703, 0.3299404806269776169, 0.3333333333333333703, 0.3299404806269776169, 0.3333333333333333703, 0.3299404806269776169, 0.3333333333333333703, 0.3299404806269776169, 0.3333333333333333703, 0.3299404806269776169, 0.3333333333333333703, 0.3299404806269776169, 0.3333333333333333703, 0.3299404806269776169, 0.3333333333333333703, 0.3299404806269776169, 0.3333333333333333703, 0.3299404806269776169, 0.3333333333333333703, 0.3299404806269776169, 0.3333333333333333703, 0.3299404806269776169, 0.3333333333333333703, 0.3299404806269776169, 0.3333333333333333703, 0.3299404806269776169, 0.3333333333333333703, 0.3299404806269776169, 0.3333333333333333703, 0.3299404806269776169, 0.3333333333333333703, 0.3299404806269776169, 0.3333333333333333703, 0.3299404806269776169, 0.3333333333333333703, 0.3299404806269776169, 0.3333333333333333703, 0.3299404806269776169, 0.3333333333333333703, 0.3299404806269776169, 0.3333333333333333703, 0.3299404806269776169, 0.3333333333333333703, 0.3299404806269776169, 0.3333333333333333703, 0.3299404806269776169, 0.3333333333333333703, 0.3299404806269776169, 0.3333333333333333703, 0.3299404806269776169, 0.3333333333333333703, 0.3299404806269776169, 0.3333333333333333703, 0.3299404806269776169, 0.3333333333333333703, 0.3299404806269776169, 0.3333333333333333703, 0.3299404806269776169, 0.3333333333333333703, 0.3299404806269776169, 0.3333333333333333703, 0.3299404806269776169, 0.3333333333333333703, 0.3299404806269776169, 0.3333333333333333703, 0.3299404806269776169, 0.3333333333333333703, 0.3299404806269776169, 0.3333333333333333703, 0.3299404806269776169, 0.3333333333333333703, 0.3299404806269776169, 0.3333333333333333703, 0.3299404806269776169, 0.3333333333333333703, 0.3299404806269776169, 0.3333333333333333703, 0.3299404806269776169, 0.3333333333333333703, 0.3299404806269776169, 0.3333333333333333703, 0.3299404806269776169, 0.3333333333333333703, 0.3299404806269776169, 0.3333333333333333703, 0.3299404806269776169, 0.3333333333333333703, 0.3299404806269776169, 0.3333333333333333703, 0.3299404806269776169, 0.3333333333333333703, 0.3299404806269776169, 0.3333333333333333703, 0.3299404806269776169, 0.3333333333333333703, 0.3299404806269776169, 0.3333333333333333703, 0.3299404806269776169, 0.3333333333333333703, 0.3299404806269776169, 0.3333333333333333703, 0.3299404806269776169, 0.3333333333333333703, 0.3299404806269776169, 0.3333333333333333703, 0.3299404806269776169, 0.3333333333333333703, 0.3299404806269776169, 0.3333333333333333703, 0.3299404806269776169, 0.3333333333333333703, 0.3299404806269776169, 0.3333333333333333703, 0.3299404806269776169, 0.3333333333333333703, 0.3299404806269776169, 0.3333333333333333703, 0.3299404806269776169, 0.3333333333333333703, 0.3299404806269776169, 0.3333333333333333703, 0.3299404806269776169, 0.3333333333333333703, 0.3299404806269776169, 0.3333333333333333703, 0.3299404806269776169, 0.3333333333333333703, 0.3299404806269776169, 0.3333333333333333703, 0.3299404806269776169, 0.3333333333333333703, 0.3299404806269776169, 0.3333333333333333703, 0.3299404806269776169, 0.3333333333333333703, 0.3299404806269776169, 0.3333333333333333703, 0.3299404806269776169, 0.3333333333333333703, 0.3299404806269776169, 0.3333333333333333703, 0.3299404806269776169, 0.3333333333333333703, 0.3299404806269776169, 0.3333333333333333703, 0.3299404806269776169, 0.3333333333333333703, 0.3299404806269776169, 0.3333333333333333703, 0.3299404806269776169, 0.3333333333333333703, 0.3299404806269776169, 0.3333333333333333703, 0.3299404806269776169, 0.3333333333333333703, 0.3299404806269776169, 0.3333333333333333703, 0.3299404806269776169, 0.3333333333333333703, 0.3299404806269776169, 0.3333333333333333703, 0.3299404806269776169, 0.3333333333333333703, 0.3299404806269776169, 0.3333333333333333703, 0.3299404806269776169, 0.3333333333333333703, 0.3299404806269776169, 0.3333333333333333703, 0.3299404806269776169, 0.3333333333333333703, 0.3299404806269776169, 0.3333333333333333703, 0.3299404806269776169, 0.3333333333333333703, 0.3299404806269776169, 0.3333333333333333703, 0.3299404806269776169, 0.3333333333333333703, 0.3299404806269776169, 0.3333333333333333703, 0.3299404806269776169, 0.3333333333333333703, 0.3299404806269776169, 0.3333333333333333703, 0.3299404806269776169, 0.3333333333333333703, 0.3299404806269776169, 0.3333333333333333703, 0.3299404806269776169, 0.3333333333333333703, 0.3299404806269776169, 0.3333333333333333703, 0.3299404806269776169, 0.3333333333333333703, 0.3299404806269776169, 0.3333333333333333703, 0.3299404806269776169, 0.3333333333333333703, 0.3299404806269776169, 0.3333333333333333703, 0.3299404806269776169, 0.3333333333333333703, 0.3299404806269776169, 0.3333333333333333703, 0.3299404806269776169, 0.3333333333333333703, 0.3299404806269776169, 0.3333333333333333703, 0.3299404806269776169, 0.3333333333333333703, 0.3299404806269776169, 0.3333333333333333703, 0.3299404806269776169, 0.3333333333333333703, 0.3299404806269776169, 0.3333333333333333703, 0.3299404806269776169, 0.3333333333333333703, 0.3299404806269776169, 0.3333333333333333703, 0.3299404806269776169, 0.3333333333333333703, 0.3299404806269776169, 0.3333333333333333703, 0.3299404806269776169, 0.3333333333333333703, 0.3299404806269776169, 0.3333333333333333703, 0.3299404806269776169, 0.3333333333333333703, 0.3299404806269776169, 0.3333333333333333703, 0.3299404806269776169, 0.3333333333333333703, 0.3299404806269776169, 0.3333333333333333703, 0.3299404806269776169, 0.3333333333333333703, 0.3299404806269776169, 0.3333333333333333703, 0.3299404806269776169, 0.3333333333333333703, 0.3299404806269776169, 0.3333333333333333703, 0.3299404806269776169, 0.3333333333333333703, 0.3299404806269776169, 0.3333333333333333703, 0.3299404806269776169, 0.3333333333333333703, 0.3299404806269776169, 0.3333333333333333703, 0.3299404806269776169, 0.3333333333333333703, 0.3299404806269776169, 0.3333333333333333703, 0.3299404806269776169, 0.3333333333333333703, 0.3299404806269776169, 0.3333333333333333703, 0.3299404806269776169, 0.3333333333333333703, 0.3299404806269776169, 0.3333333333333333703, 0.3299404806269776169, 0.3333333333333333703, 0.3299404806269776169, 0.3333333333333333703, 0.3299404806269776169, 0.3333333333333333703, 0.3299404806269776169, 0.3333333333333333703, 0.3299404806269776169, 0.3333333333333333703, 0.3299404806269776169, 0.3333333333333333703, 0.3299404806269776169, 0.3333333333333333703, 0.3299404806269776169, 0.3333333333333333703, 0.3299404806269776169, 0.3333333333333333703, 0.3299404806269776169, 0.3333333333333333703, 0.3299404806269776169, 0.3333333333333333703, 0.3299404806269776169, 0.3333333333333333703, 0.3299404806269776169, 0.3333333333333333703, 0.3299404806269776169, 0.3333333333333333703, 0.3299404806269776169, 0.3333333333333333703, 0.3299404806269776169, 0.3333333333333333703, 0.3299404806269776169, 0.3333333333333333703, 0.3299404806269776169, 0.3333333333333333703, 0.3299404806269776169, 0.3333333333333333703, 0.3299404806269776169, 0.3333333333333333703, 0.3299404806269776169, 0.3333333333333333703, 0.3299404806269776169, 0.3333333333333333703, 0.3299404806269776169, 0.3333333333333333703, 0.3299404806269776169, 0.3333333333333333703, 0.3299404806269776169, 0.3333333333333333703, 0.3299404806269776169, 0.3333333333333333703, 0.3299404806269776169, 0.3333333333333333703, 0.3299404806269776169, 0.3333333333333333703, 0.3299404806269776169, 0.3333333333333333703, 0.3299404806269776169, 0.3333333333333333703, 0.3299404806269776169, 0.3333333333333333703, 0.3299404806269776169, 0.3333333333333333703, 0.3299404806269776169, 0.3333333333333333703, 0.3299404806269776169, 0.3333333333333333703, 0.3299404806269776169, 0.3333333333333333703, 0.3299404806269776169, 0.3333333333333333703, 0.3299404806269776169, 0.3333333333333333703, 0.3299404806269776169, 0.3333333333333333703, 0.3299404806269776169, 0.3333333333333333703, 0.3299404806269776169, 0.3333333333333333703, 0.3299404806269776169, 0.3333333333333333703, 0.3299404806269776169, 0.3333333333333333703, 0.3299404806269776169, 0.3333333333333333703, 0.3299404806269776169, 0.3333333333333333703, 0.3299404806269776169, 0.3333333333333333703, 0.3299404806269776169, 0.3333333333333333703, 0.3299404806269776169, 0.3333333333333333703, 0.3299404806269776169, 0.3333333333333333703, 0.3299404806269776169, 0.3333333333333333703, 0.3299404806269776169, 0.3333333333333333703, 0.3299404806269776169, 0.3333333333333333703, 0.3299404806269776169, 0.3333333333333333703, 0.3299404806269776169, 0.3333333333333333703, 0.3299404806269776169, 0.3333333333333333703, 0.3299404806269776169, 0.3333333333333333703, 0.3299404806269776169, 0.3333333333333333703, 0.3299404806269776169, 0.3333333333333333703, 0.3299404806269776169, 0.3333333333333333703, 0.3299404806269776169, 0.3333333333333333703, 0.3299404806269776169, 0.3333333333333333703, 0.3299404806269776169, 0.3333333333333333703, 0.3299404806269776169, 0.3333333333333333703, 0.3299404806269776169, 0.3333333333333333703, 0.3299404806269776169, 0.3333333333333333703, 0.3299404806269776169, 0.3333333333333333703, 0.3299404806269776169, 0.3333333333333333703, 0.3299404806269776169, 0.3333333333333333703, 0.3299404806269776169, 0.3333333333333333703, 0.3299404806269776169, 0.3333333333333333703, 0.3299404806269776169, 0.3333333333333333703, 0.3299404806269776169, 0.3333333333333333703, 0.3299404806269776169, 0.3333333333333333703, 0.3299404806269776169, 0.3333333333333333703, 0.3299404806269776169, 0.3333333333333333703, 0.3299404806269776169, 0.3333333333333333703, 0.3299404806269776169, 0.3333333333333333703, 0.3299404806269776169, 0.3333333333333333703, 0.3299404806269776169, 0.3333333333333333703, 0.3299404806269776169, 0.3333333333333333703, 0.3299404806269776169, 0.3333333333333333703, 0.3299404806269776169, 0.3333333333333333703, 0.3299404806269776169, 0.3333333333333333703, 0.3299404806269776169, 0.3333333333333333703, 0.3299404806269776169, 0.3333333333333333703, 0.3299404806269776169, 0.3333333333333333703, 0.3299404806269776169, 0.3333333333333333703, 0.3299404806269776169, 0.3333333333333333703, 0.3299404806269776169, 0.3333333333333333703, 0.3299404806269776169, 0.3333333333333333703, 0.3299404806269776169, 0.3333333333333333703, 0.3299404806269776169, 0.3333333333333333703, 0.3299404806269776169, 0.3333333333333333703, 0.3299404806269776169, 0.3333333333333333703, 0.3299404806269776169, 0.3333333333333333703, 0.3299404806269776169, 0.3333333333333333703, 0.3299404806269776169, 0.3333333333333333703, 0.3299404806269776169, 0.3333333333333333703, 0.3299404806269776169, 0.3333333333333333703, 0.3299404806269776169, 0.3333333333333333703, 0.3299404806269776169, 0.3333333333333333703, 0.3299404806269776169, 0.3333333333333333703, 0.3299404806269776169, 0.3333333333333333703, 0.3299404806269776169, 0.3333333333333333703, 0.3299404806269776169, 0.3333333333333333703, 0.3299404806269776169, 0.3333333333333333703, 0.3299404806269776169, 0.3333333333333333703, 0.3299404806269776169, 0.3333333333333333703, 0.3299404806269776169, 0.3333333333333333703, 0.3299404806269776169, 0.3333333333333333703, 0.3299404806269776169, 0.3333333333333333703, 0.3299404806269776169, 0.3333333333333333703, 0.3299404806269776169, 0.3333333333333333703, 0.3299404806269776169, 0.3333333333333333703, 0.3299404806269776169, 0.3333333333333333703, 0.3299404806269776169, 0.3333333333333333703, 0.3299404806269776169, 0.3333333333333333703, 0.3299404806269776169, 0.3333333333333333703, 0.3299404806269776169, 0.3333333333333333703, 0.3299404806269776169, 0.3333333333333333703, 0.3299404806269776169, 0.3333333333333333703, 0.3299404806269776169, 0.3333333333333333703, 0.3299404806269776169, 0.3333333333333333703, 0.3299404806269776169, 0.3333333333333333703, 0.3299404806269776169, 0.3333333333333333703, 0.3299404806269776169, 0.3333333333333333703, 0.3299404806269776169, 0.3333333333333333703, 0.3299404806269776169, 0.3333333333333333703, 0.3299404806269776169, 0.3333333333333333703, 0.3299404806269776169, 0.3333333333333333703, 0.3299404806269776169, 0.3333333333333333703, 0.3299404806269776169, 0.3333333333333333703, 0.3299404806269776169, 0.3333333333333333703, 0.3299404806269776169, 0.3333333333333333703, 0.3299404806269776169, 0.3333333333333333703, 0.3299404806269776169, 0.3333333333333333703, 0.3299404806269776169, 0.3333333333333333703, 0.3299404806269776169, 0.3333333333333333703, 0.3299404806269776169, 0.3333333333333333703, 0.3299404806269776169, 0.3333333333333333703, 0.3299404806269776169, 0.3333333333333333703, 0.3299404806269776169, 0.3333333333333333703, 0.3299404806269776169, 0.3333333333333333703, 0.3299404806269776169, 0.3333333333333333703, 0.3299404806269776169, 0.3333333333333333703, 0.3320603117974822438, 0.3317425830320511193),
 ( 0.3333333333333333703, 0.3299404806269776169, 0.3333333333333333703, 0.3299404806269776169, 0.3333333333333333703, 0.3299404806269776169, 0.3333333333333333703, 0.3299404806269776169, 0.3333333333333333703, 0.3299404806269776169, 0.3333333333333333703, 0.3299404806269776169, 0.3333333333333333703, 0.3299404806269776169, 0.3333333333333333703, 0.3299404806269776169, 0.3333333333333333703, 0.3299404806269776169, 0.3333333333333333703, 0.3299404806269776169, 0.3333333333333333703, 0.3299404806269776169, 0.3333333333333333703, 0.3299404806269776169, 0.3333333333333333703, 0.3299404806269776169, 0.3333333333333333703, 0.3299404806269776169, 0.3333333333333333703, 0.3299404806269776169, 0.3333333333333333703, 0.3299404806269776169, 0.3333333333333333703, 0.3299404806269776169, 0.3333333333333333703, 0.3299404806269776169, 0.3333333333333333703, 0.3299404806269776169, 0.3333333333333333703, 0.3299404806269776169, 0.3333333333333333703, 0.3299404806269776169, 0.3333333333333333703, 0.3299404806269776169, 0.3333333333333333703, 0.3299404806269776169, 0.3333333333333333703, 0.3299404806269776169, 0.3333333333333333703, 0.3299404806269776169, 0.3333333333333333703, 0.3299404806269776169, 0.3333333333333333703, 0.3299404806269776169, 0.3333333333333333703, 0.3299404806269776169, 0.3333333333333333703, 0.3299404806269776169, 0.3333333333333333703, 0.3299404806269776169, 0.3333333333333333703, 0.3299404806269776169, 0.3333333333333333703, 0.3299404806269776169, 0.3333333333333333703, 0.3299404806269776169, 0.3333333333333333703, 0.3299404806269776169, 0.3333333333333333703, 0.3299404806269776169, 0.3333333333333333703, 0.3299404806269776169, 0.3333333333333333703, 0.3299404806269776169, 0.3333333333333333703, 0.3299404806269776169, 0.3333333333333333703, 0.3299404806269776169, 0.3333333333333333703, 0.3299404806269776169, 0.3333333333333333703, 0.3299404806269776169, 0.3333333333333333703, 0.3299404806269776169, 0.3333333333333333703, 0.3299404806269776169, 0.3333333333333333703, 0.3299404806269776169, 0.3333333333333333703, 0.3299404806269776169, 0.3333333333333333703, 0.3299404806269776169, 0.3333333333333333703, 0.3299404806269776169, 0.3333333333333333703, 0.3299404806269776169, 0.3333333333333333703, 0.3299404806269776169, 0.3333333333333333703, 0.3299404806269776169, 0.3333333333333333703, 0.3299404806269776169, 0.3333333333333333703, 0.3299404806269776169, 0.3333333333333333703, 0.3299404806269776169, 0.3333333333333333703, 0.3299404806269776169, 0.3333333333333333703, 0.3299404806269776169, 0.3333333333333333703, 0.3299404806269776169, 0.3333333333333333703, 0.3299404806269776169, 0.3333333333333333703, 0.3299404806269776169, 0.3333333333333333703, 0.3299404806269776169, 0.3333333333333333703, 0.3299404806269776169, 0.3333333333333333703, 0.3299404806269776169, 0.3333333333333333703, 0.3299404806269776169, 0.3333333333333333703, 0.3299404806269776169, 0.3333333333333333703, 0.3299404806269776169, 0.3333333333333333703, 0.3299404806269776169, 0.3333333333333333703, 0.3299404806269776169, 0.3333333333333333703, 0.3299404806269776169, 0.3333333333333333703, 0.3299404806269776169, 0.3333333333333333703, 0.3299404806269776169, 0.3333333333333333703, 0.3299404806269776169, 0.3333333333333333703, 0.3299404806269776169, 0.3333333333333333703, 0.3299404806269776169, 0.3333333333333333703, 0.3299404806269776169, 0.3333333333333333703, 0.3299404806269776169, 0.3333333333333333703, 0.3299404806269776169, 0.3333333333333333703, 0.3299404806269776169, 0.3333333333333333703, 0.3299404806269776169, 0.3333333333333333703, 0.3299404806269776169, 0.3333333333333333703, 0.3299404806269776169, 0.3333333333333333703, 0.3299404806269776169, 0.3333333333333333703, 0.3299404806269776169, 0.3333333333333333703, 0.3299404806269776169, 0.3333333333333333703, 0.3299404806269776169, 0.3333333333333333703, 0.3299404806269776169, 0.3333333333333333703, 0.3299404806269776169, 0.3333333333333333703, 0.3299404806269776169, 0.3333333333333333703, 0.3299404806269776169, 0.3333333333333333703, 0.3299404806269776169, 0.3333333333333333703, 0.3299404806269776169, 0.3333333333333333703, 0.3299404806269776169, 0.3333333333333333703, 0.3299404806269776169, 0.3333333333333333703, 0.3299404806269776169, 0.3333333333333333703, 0.3299404806269776169, 0.3333333333333333703, 0.3299404806269776169, 0.3333333333333333703, 0.3299404806269776169, 0.3333333333333333703, 0.3299404806269776169, 0.3333333333333333703, 0.3299404806269776169, 0.3333333333333333703, 0.3299404806269776169, 0.3333333333333333703, 0.3299404806269776169, 0.3333333333333333703, 0.3299404806269776169, 0.3333333333333333703, 0.3299404806269776169, 0.3333333333333333703, 0.3299404806269776169, 0.3333333333333333703, 0.3299404806269776169, 0.3333333333333333703, 0.3299404806269776169, 0.3333333333333333703, 0.3299404806269776169, 0.3333333333333333703, 0.3299404806269776169, 0.3333333333333333703, 0.3299404806269776169, 0.3333333333333333703, 0.3299404806269776169, 0.3333333333333333703, 0.3299404806269776169, 0.3333333333333333703, 0.3299404806269776169, 0.3333333333333333703, 0.3299404806269776169, 0.3333333333333333703, 0.3299404806269776169, 0.3333333333333333703, 0.3299404806269776169, 0.3333333333333333703, 0.3299404806269776169, 0.3333333333333333703, 0.3299404806269776169, 0.3333333333333333703, 0.3299404806269776169, 0.3333333333333333703, 0.3299404806269776169, 0.3333333333333333703, 0.3299404806269776169, 0.3333333333333333703, 0.3299404806269776169, 0.3333333333333333703, 0.3299404806269776169, 0.3333333333333333703, 0.3299404806269776169, 0.3333333333333333703, 0.3299404806269776169, 0.3333333333333333703, 0.3299404806269776169, 0.3333333333333333703, 0.3299404806269776169, 0.3333333333333333703, 0.3299404806269776169, 0.3333333333333333703, 0.3299404806269776169, 0.3333333333333333703, 0.3299404806269776169, 0.3333333333333333703, 0.3299404806269776169, 0.3333333333333333703, 0.3299404806269776169, 0.3333333333333333703, 0.3299404806269776169, 0.3333333333333333703, 0.3299404806269776169, 0.3333333333333333703, 0.3299404806269776169, 0.3333333333333333703, 0.3299404806269776169, 0.3333333333333333703, 0.3299404806269776169, 0.3333333333333333703, 0.3299404806269776169, 0.3333333333333333703, 0.3299404806269776169, 0.3333333333333333703, 0.3299404806269776169, 0.3333333333333333703, 0.3299404806269776169, 0.3333333333333333703, 0.3299404806269776169, 0.3333333333333333703, 0.3299404806269776169, 0.3333333333333333703, 0.3299404806269776169, 0.3333333333333333703, 0.3299404806269776169, 0.3333333333333333703, 0.3299404806269776169, 0.3333333333333333703, 0.3299404806269776169, 0.3333333333333333703, 0.3299404806269776169, 0.3333333333333333703, 0.3299404806269776169, 0.3333333333333333703, 0.3299404806269776169, 0.3333333333333333703, 0.3299404806269776169, 0.3333333333333333703, 0.3299404806269776169, 0.3333333333333333703, 0.3299404806269776169, 0.3333333333333333703, 0.3299404806269776169, 0.3333333333333333703, 0.3299404806269776169, 0.3333333333333333703, 0.3299404806269776169, 0.3333333333333333703, 0.3299404806269776169, 0.3333333333333333703, 0.3299404806269776169, 0.3333333333333333703, 0.3299404806269776169, 0.3333333333333333703, 0.3299404806269776169, 0.3333333333333333703, 0.3299404806269776169, 0.3333333333333333703, 0.3299404806269776169, 0.3333333333333333703, 0.3299404806269776169, 0.3333333333333333703, 0.3299404806269776169, 0.3333333333333333703, 0.3299404806269776169, 0.3333333333333333703, 0.3299404806269776169, 0.3333333333333333703, 0.3299404806269776169, 0.3333333333333333703, 0.3299404806269776169, 0.3333333333333333703, 0.3299404806269776169, 0.3333333333333333703, 0.3299404806269776169, 0.3333333333333333703, 0.3299404806269776169, 0.3333333333333333703, 0.3299404806269776169, 0.3333333333333333703, 0.3299404806269776169, 0.3333333333333333703, 0.3299404806269776169, 0.3333333333333333703, 0.3299404806269776169, 0.3333333333333333703, 0.3299404806269776169, 0.3333333333333333703, 0.3299404806269776169, 0.3333333333333333703, 0.3299404806269776169, 0.3333333333333333703, 0.3299404806269776169, 0.3333333333333333703, 0.3299404806269776169, 0.3333333333333333703, 0.3299404806269776169, 0.3333333333333333703, 0.3299404806269776169, 0.3333333333333333703, 0.3299404806269776169, 0.3333333333333333703, 0.3299404806269776169, 0.3333333333333333703, 0.3299404806269776169, 0.3333333333333333703, 0.3299404806269776169, 0.3333333333333333703, 0.3299404806269776169, 0.3333333333333333703, 0.3299404806269776169, 0.3333333333333333703, 0.3299404806269776169, 0.3333333333333333703, 0.3299404806269776169, 0.3333333333333333703, 0.3299404806269776169, 0.3333333333333333703, 0.3299404806269776169, 0.3333333333333333703, 0.3299404806269776169, 0.3333333333333333703, 0.3299404806269776169, 0.3333333333333333703, 0.3299404806269776169, 0.3333333333333333703, 0.3299404806269776169, 0.3333333333333333703, 0.3299404806269776169, 0.3333333333333333703, 0.3299404806269776169, 0.3333333333333333703, 0.3299404806269776169, 0.3333333333333333703, 0.3299404806269776169, 0.3333333333333333703, 0.3299404806269776169, 0.3333333333333333703, 0.3299404806269776169, 0.3333333333333333703, 0.3299404806269776169, 0.3333333333333333703, 0.3299404806269776169, 0.3333333333333333703, 0.3299404806269776169, 0.3333333333333333703, 0.3299404806269776169, 0.3333333333333333703, 0.3299404806269776169, 0.3333333333333333703, 0.3299404806269776169, 0.3333333333333333703, 0.3299404806269776169, 0.3333333333333333703, 0.3299404806269776169, 0.3333333333333333703, 0.3299404806269776169, 0.3333333333333333703, 0.3299404806269776169, 0.3333333333333333703, 0.3299404806269776169, 0.3333333333333333703, 0.3299404806269776169, 0.3333333333333333703, 0.3299404806269776169, 0.3333333333333333703, 0.3299404806269776169, 0.3333333333333333703, 0.3299404806269776169, 0.3333333333333333703, 0.3299404806269776169, 0.3333333333333333703, 0.3299404806269776169, 0.3333333333333333703, 0.3299404806269776169, 0.3333333333333333703, 0.3299404806269776169, 0.3333333333333333703, 0.3299404806269776169, 0.3333333333333333703, 0.3299404806269776169, 0.3333333333333333703, 0.3299404806269776169, 0.3333333333333333703, 0.3299404806269776169, 0.3333333333333333703, 0.3299404806269776169, 0.3333333333333333703, 0.3299404806269776169, 0.3333333333333333703, 0.3299404806269776169, 0.3333333333333333703, 0.3299404806269776169, 0.3333333333333333703, 0.3299404806269776169, 0.3333333333333333703, 0.3299404806269776169, 0.3333333333333333703, 0.3299404806269776169, 0.3333333333333333703, 0.3299404806269776169, 0.3333333333333333703, 0.3299404806269776169, 0.3333333333333333703, 0.3299404806269776169, 0.3333333333333333703, 0.3299404806269776169, 0.3333333333333333703, 0.3299404806269776169, 0.3333333333333333703, 0.3299404806269776169, 0.3333333333333333703, 0.3299404806269776169, 0.3333333333333333703, 0.3299404806269776169, 0.3333333333333333703, 0.3299404806269776169, 0.3333333333333333703, 0.3299404806269776169, 0.3333333333333333703, 0.3299404806269776169, 0.3333333333333333703, 0.3299404806269776169, 0.3333333333333333703, 0.3299404806269776169, 0.3333333333333333703, 0.3299404806269776169, 0.3333333333333333703, 0.3299404806269776169, 0.3333333333333333703, 0.3299404806269776169, 0.3333333333333333703, 0.3299404806269776169, 0.3333333333333333703, 0.3299404806269776169, 0.3333333333333333703, 0.3299404806269776169, 0.3333333333333333703, 0.3299404806269776169, 0.3333333333333333703, 0.3299404806269776169, 0.3333333333333333703, 0.3299404806269776169, 0.3333333333333333703, 0.3299404806269776169, 0.3333333333333333703, 0.3299404806269776169, 0.3333333333333333703, 0.3299404806269776169, 0.3333333333333333703, 0.3299404806269776169, 0.3333333333333333703, 0.3299404806269776169, 0.3333333333333333703, 0.3299404806269776169, 0.3333333333333333703, 0.3299404806269776169, 0.3333333333333333703, 0.3299404806269776169, 0.3333333333333333703, 0.3299404806269776169, 0.3333333333333333703, 0.3299404806269776169, 0.3333333333333333703, 0.3299404806269776169, 0.3333333333333333703, 0.3299404806269776169, 0.3333333333333333703, 0.3299404806269776169, 0.3333333333333333703, 0.3299404806269776169, 0.3333333333333333703, 0.3299404806269776169, 0.3333333333333333703, 0.3299404806269776169, 0.3333333333333333703, 0.3299404806269776169, 0.3333333333333333703, 0.3299404806269776169, 0.3333333333333333703, 0.3299404806269776169, 0.3333333333333333703, 0.3299404806269776169, 0.3333333333333333703, 0.3299404806269776169, 0.3333333333333333703, 0.3299404806269776169, 0.3333333333333333703, 0.3299404806269776169, 0.3333333333333333703, 0.3299404806269776169, 0.3333333333333333703, 0.3299404806269776169, 0.3333333333333333703, 0.3299404806269776169, 0.3333333333333333703, 0.3299404806269776169, 0.3333333333333333703, 0.3299404806269776169, 0.3333333333333333703, 0.3299404806269776169, 0.3333333333333333703, 0.3299404806269776169, 0.3333333333333333703, 0.3299404806269776169, 0.3333333333333333703, 0.3299404806269776169, 0.3333333333333333703, 0.3299404806269776169, 0.3333333333333333703, 0.3299404806269776169, 0.3333333333333333703, 0.3299404806269776169, 0.3333333333333333703, 0.3299404806269776169, 0.3333333333333333703, 0.3299404806269776169, 0.3333333333333333703, 0.3299404806269776169, 0.3333333333333333703, 0.3299404806269776169, 0.3333333333333333703, 0.3299404806269776169, 0.3333333333333333703, 0.3299404806269776169, 0.3333333333333333703, 0.3299404806269776169, 0.3333333333333333703, 0.3299404806269776169, 0.3333333333333333703, 0.3299404806269776169, 0.3333333333333333703, 0.3299404806269776169, 0.3333333333333333703, 0.3299404806269776169, 0.3333333333333333703, 0.3299404806269776169, 0.3333333333333333703, 0.3299404806269776169, 0.3333333333333333703, 0.3299404806269776169, 0.3333333333333333703, 0.3299404806269776169, 0.3333333333333333703, 0.3299404806269776169, 0.3333333333333333703, 0.3299404806269776169, 0.3333333333333333703, 0.3299404806269776169, 0.3333333333333333703, 0.3299404806269776169, 0.3333333333333333703, 0.3299404806269776169, 0.3333333333333333703, 0.3299404806269776169, 0.3333333333333333703, 0.3299404806269776169, 0.3333333333333333703, 0.3299404806269776169, 0.3333333333333333703, 0.3299404806269776169, 0.3333333333333333703, 0.3299404806269776169, 0.3333333333333333703, 0.3299404806269776169, 0.3333333333333333703, 0.3299404806269776169, 0.3333333333333333703, 0.3299404806269776169, 0.3333333333333333703, 0.3299404806269776169, 0.3333333333333333703, 0.3299404806269776169, 0.3333333333333333703, 0.3299404806269776169, 0.3333333333333333703, 0.3299404806269776169, 0.3333333333333333703, 0.3299404806269776169, 0.3333333333333333703, 0.3299404806269776169, 0.3333333333333333703, 0.3299404806269776169, 0.3333333333333333703, 0.3299404806269776169, 0.3333333333333333703, 0.3299404806269776169, 0.3333333333333333703, 0.3299404806269776169, 0.3333333333333333703, 0.3299404806269776169, 0.3333333333333333703, 0.3299404806269776169, 0.3333333333333333703, 0.3299404806269776169, 0.3333333333333333703, 0.3299404806269776169, 0.3333333333333333703, 0.3299404806269776169, 0.3333333333333333703, 0.3299404806269776169, 0.3333333333333333703, 0.3299404806269776169, 0.3333333333333333703, 0.3299404806269776169, 0.3333333333333333703, 0.3299404806269776169, 0.3333333333333333703, 0.3299404806269776169, 0.3333333333333333703, 0.3299404806269776169, 0.3333333333333333703, 0.3299404806269776169, 0.3333333333333333703, 0.3299404806269776169, 0.3333333333333333703, 0.3299404806269776169, 0.3333333333333333703, 0.3299404806269776169, 0.3333333333333333703, 0.3299404806269776169, 0.3333333333333333703, 0.3299404806269776169, 0.3333333333333333703, 0.3299404806269776169, 0.3333333333333333703, 0.3299404806269776169, 0.3333333333333333703, 0.3299404806269776169, 0.3333333333333333703, 0.3299404806269776169, 0.3333333333333333703, 0.3299404806269776169, 0.3333333333333333703, 0.3299404806269776169, 0.3333333333333333703, 0.3299404806269776169, 0.3333333333333333703, 0.3299404806269776169, 0.3333333333333333703, 0.3299404806269776169, 0.3333333333333333703, 0.3299404806269776169, 0.3333333333333333703, 0.3299404806269776169, 0.3333333333333333703, 0.3299404806269776169, 0.3333333333333333703, 0.3299404806269776169, 0.3333333333333333703, 0.3299404806269776169, 0.3333333333333333703, 0.3299404806269776169, 0.3333333333333333703, 0.3299404806269776169, 0.3333333333333333703, 0.3299404806269776169, 0.3333333333333333703, 0.3299404806269776169, 0.3333333333333333703, 0.3299404806269776169, 0.3333333333333333703, 0.3299404806269776169, 0.3333333333333333703, 0.3299404806269776169, 0.3333333333333333703, 0.3299404806269776169, 0.3333333333333333703, 0.3299404806269776169, 0.3333333333333333703, 0.3299404806269776169, 0.3333333333333333703, 0.3299404806269776169, 0.3333333333333333703, 0.3299404806269776169, 0.3333333333333333703, 0.3299404806269776169, 0.3333333333333333703, 0.3299404806269776169, 0.3333333333333333703, 0.3299404806269776169, 0.3333333333333333703, 0.3299404806269776169, 0.3333333333333333703, 0.3299404806269776169, 0.3333333333333333703, 0.3299404806269776169, 0.3333333333333333703, 0.3299404806269776169, 0.3333333333333333703, 0.3299404806269776169, 0.3333333333333333703, 0.3299404806269776169, 0.3333333333333333703, 0.3299404806269776169, 0.3333333333333333703, 0.3299404806269776169, 0.3333333333333333703, 0.3299404806269776169, 0.3333333333333333703, 0.3299404806269776169, 0.3333333333333333703, 0.3299404806269776169, 0.3333333333333333703, 0.3299404806269776169, 0.3333333333333333703, 0.3299404806269776169, 0.3333333333333333703, 0.3299404806269776169, 0.3333333333333333703, 0.3299404806269776169, 0.3333333333333333703, 0.3299404806269776169, 0.3333333333333333703, 0.3299404806269776169, 0.3333333333333333703, 0.3299404806269776169, 0.3333333333333333703, 0.3299404806269776169, 0.3333333333333333703, 0.3299404806269776169, 0.3333333333333333703, 0.3299404806269776169, 0.3333333333333333703, 0.3299404806269776169, 0.3333333333333333703, 0.3299404806269776169, 0.3333333333333333703, 0.3299404806269776169, 0.3333333333333333703, 0.3299404806269776169, 0.3333333333333333703, 0.3299404806269776169, 0.3333333333333333703, 0.3299404806269776169, 0.3333333333333333703, 0.3299404806269776169, 0.3333333333333333703, 0.3299404806269776169, 0.3333333333333333703, 0.3299404806269776169, 0.3333333333333333703, 0.3299404806269776169, 0.3333333333333333703, 0.3299404806269776169, 0.3333333333333333703, 0.3299404806269776169, 0.3333333333333333703, 0.3299404806269776169, 0.3333333333333333703, 0.3299404806269776169, 0.3333333333333333703, 0.3299404806269776169, 0.3333333333333333703, 0.3299404806269776169, 0.3333333333333333703, 0.3299404806269776169, 0.3333333333333333703, 0.3299404806269776169, 0.3333333333333333703, 0.3299404806269776169, 0.3333333333333333703, 0.3299404806269776169, 0.3333333333333333703, 0.3299404806269776169, 0.3333333333333333703, 0.3299404806269776169, 0.3333333333333333703, 0.3299404806269776169, 0.3333333333333333703, 0.3299404806269776169, 0.3333333333333333703, 0.3299404806269776169, 0.3333333333333333703, 0.3299404806269776169, 0.3333333333333333703, 0.3299404806269776169, 0.3333333333333333703, 0.3299404806269776169, 0.3333333333333333703, 0.3299404806269776169, 0.3333333333333333703, 0.3299404806269776169, 0.3333333333333333703, 0.3299404806269776169, 0.3333333333333333703, 0.3299404806269776169, 0.3333333333333333703, 0.3299404806269776169, 0.3333333333333333703, 0.3299404806269776169, 0.3333333333333333703, 0.3299404806269776169, 0.3333333333333333703, 0.3299404806269776169, 0.3333333333333333703, 0.3299404806269776169, 0.3333333333333333703, 0.3299404806269776169, 0.3333333333333333703, 0.3299404806269776169, 0.3333333333333333703, 0.3320603117974822438, 0.3317425830320511193),
 ( 1.000000000000000000, 0.9898214418809326842, 1.000000000000000000, 0.9898214418809326842, 1.000000000000000000, 0.9898214418809326842, 1.000000000000000000, 0.9898214418809326842, 1.000000000000000000, 0.9898214418809326842, 1.000000000000000000, 0.9898214418809326842, 1.000000000000000000, 0.9898214418809326842, 1.000000000000000000, 0.9898214418809326842, 1.000000000000000000, 0.9898214418809326842, 1.000000000000000000, 0.9898214418809326842, 1.000000000000000000, 0.9898214418809326842, 1.000000000000000000, 0.9898214418809326842, 1.000000000000000000, 0.9898214418809326842, 1.000000000000000000, 0.9898214418809326842, 1.000000000000000000, 0.9898214418809326842, 1.000000000000000000, 0.9898214418809326842, 1.000000000000000000, 0.9898214418809326842, 1.000000000000000000, 0.9898214418809326842, 1.000000000000000000, 0.9898214418809326842, 1.000000000000000000, 0.9898214418809326842, 1.000000000000000000, 0.9898214418809326842, 1.000000000000000000, 0.9898214418809326842, 1.000000000000000000, 0.9898214418809326842, 1.000000000000000000, 0.9898214418809326842, 1.000000000000000000, 0.9898214418809326842, 1.000000000000000000, 0.9898214418809326842, 1.000000000000000000, 0.9898214418809326842, 1.000000000000000000, 0.9898214418809326842, 1.000000000000000000, 0.9898214418809326842, 1.000000000000000000, 0.9898214418809326842, 1.000000000000000000, 0.9898214418809326842, 1.000000000000000000, 0.9898214418809326842, 1.000000000000000000, 0.9898214418809326842, 1.000000000000000000, 0.9898214418809326842, 1.000000000000000000, 0.9898214418809326842, 1.000000000000000000, 0.9898214418809326842, 1.000000000000000000, 0.9898214418809326842, 1.000000000000000000, 0.9898214418809326842, 1.000000000000000000, 0.9898214418809326842, 1.000000000000000000, 0.9898214418809326842, 1.000000000000000000, 0.9898214418809326842, 1.000000000000000000, 0.9898214418809326842, 1.000000000000000000, 0.9898214418809326842, 1.000000000000000000, 0.9898214418809326842, 1.000000000000000000, 0.9898214418809326842, 1.000000000000000000, 0.9898214418809326842, 1.000000000000000000, 0.9898214418809326842, 1.000000000000000000, 0.9898214418809326842, 1.000000000000000000, 0.9898214418809326842, 1.000000000000000000, 0.9898214418809326842, 1.000000000000000000, 0.9898214418809326842, 1.000000000000000000, 0.9898214418809326842, 1.000000000000000000, 0.9898214418809326842, 1.000000000000000000, 0.9898214418809326842, 1.000000000000000000, 0.9898214418809326842, 1.000000000000000000, 0.9898214418809326842, 1.000000000000000000, 0.9898214418809326842, 1.000000000000000000, 0.9898214418809326842, 1.000000000000000000, 0.9898214418809326842, 1.000000000000000000, 0.9898214418809326842, 1.000000000000000000, 0.9898214418809326842, 1.000000000000000000, 0.9898214418809326842, 1.000000000000000000, 0.9898214418809326842, 1.000000000000000000, 0.9898214418809326842, 1.000000000000000000, 0.9898214418809326842, 1.000000000000000000, 0.9898214418809326842, 1.000000000000000000, 0.9898214418809326842, 1.000000000000000000, 0.9898214418809326842, 1.000000000000000000, 0.9898214418809326842, 1.000000000000000000, 0.9898214418809326842, 1.000000000000000000, 0.9898214418809326842, 1.000000000000000000, 0.9898214418809326842, 1.000000000000000000, 0.9898214418809326842, 1.000000000000000000, 0.9898214418809326842, 1.000000000000000000, 0.9898214418809326842, 1.000000000000000000, 0.9898214418809326842, 1.000000000000000000, 0.9898214418809326842, 1.000000000000000000, 0.9898214418809326842, 1.000000000000000000, 0.9898214418809326842, 1.000000000000000000, 0.9898214418809326842, 1.000000000000000000, 0.9898214418809326842, 1.000000000000000000, 0.9898214418809326842, 1.000000000000000000, 0.9898214418809326842, 1.000000000000000000, 0.9898214418809326842, 1.000000000000000000, 0.9898214418809326842, 1.000000000000000000, 0.9898214418809326842, 1.000000000000000000, 0.9898214418809326842, 1.000000000000000000, 0.9898214418809326842, 1.000000000000000000, 0.9898214418809326842, 1.000000000000000000, 0.9898214418809326842, 1.000000000000000000, 0.9898214418809326842, 1.000000000000000000, 0.9898214418809326842, 1.000000000000000000, 0.9898214418809326842, 1.000000000000000000, 0.9898214418809326842, 1.000000000000000000, 0.9898214418809326842, 1.000000000000000000, 0.9898214418809326842, 1.000000000000000000, 0.9898214418809326842, 1.000000000000000000, 0.9898214418809326842, 1.000000000000000000, 0.9898214418809326842, 1.000000000000000000, 0.9898214418809326842, 1.000000000000000000, 0.9898214418809326842, 1.000000000000000000, 0.9898214418809326842, 1.000000000000000000, 0.9898214418809326842, 1.000000000000000000, 0.9898214418809326842, 1.000000000000000000, 0.9898214418809326842, 1.000000000000000000, 0.9898214418809326842, 1.000000000000000000, 0.9898214418809326842, 1.000000000000000000, 0.9898214418809326842, 1.000000000000000000, 0.9898214418809326842, 1.000000000000000000, 0.9898214418809326842, 1.000000000000000000, 0.9898214418809326842, 1.000000000000000000, 0.9898214418809326842, 1.000000000000000000, 0.9898214418809326842, 1.000000000000000000, 0.9898214418809326842, 1.000000000000000000, 0.9898214418809326842, 1.000000000000000000, 0.9898214418809326842, 1.000000000000000000, 0.9898214418809326842, 1.000000000000000000, 0.9898214418809326842, 1.000000000000000000, 0.9898214418809326842, 1.000000000000000000, 0.9898214418809326842, 1.000000000000000000, 0.9898214418809326842, 1.000000000000000000, 0.9898214418809326842, 1.000000000000000000, 0.9898214418809326842, 1.000000000000000000, 0.9898214418809326842, 1.000000000000000000, 0.9898214418809326842, 1.000000000000000000, 0.9898214418809326842, 1.000000000000000000, 0.9898214418809326842, 1.000000000000000000, 0.9898214418809326842, 1.000000000000000000, 0.9898214418809326842, 1.000000000000000000, 0.9898214418809326842, 1.000000000000000000, 0.9898214418809326842, 1.000000000000000000, 0.9898214418809326842, 1.000000000000000000, 0.9898214418809326842, 1.000000000000000000, 0.9898214418809326842, 1.000000000000000000, 0.9898214418809326842, 1.000000000000000000, 0.9898214418809326842, 1.000000000000000000, 0.9898214418809326842, 1.000000000000000000, 0.9898214418809326842, 1.000000000000000000, 0.9898214418809326842, 1.000000000000000000, 0.9898214418809326842, 1.000000000000000000, 0.9898214418809326842, 1.000000000000000000, 0.9898214418809326842, 1.000000000000000000, 0.9898214418809326842, 1.000000000000000000, 0.9898214418809326842, 1.000000000000000000, 0.9898214418809326842, 1.000000000000000000, 0.9898214418809326842, 1.000000000000000000, 0.9898214418809326842, 1.000000000000000000, 0.9898214418809326842, 1.000000000000000000, 0.9898214418809326842, 1.000000000000000000, 0.9898214418809326842, 1.000000000000000000, 0.9898214418809326842, 1.000000000000000000, 0.9898214418809326842, 1.000000000000000000, 0.9898214418809326842, 1.000000000000000000, 0.9898214418809326842, 1.000000000000000000, 0.9898214418809326842, 1.000000000000000000, 0.9898214418809326842, 1.000000000000000000, 0.9898214418809326842, 1.000000000000000000, 0.9898214418809326842, 1.000000000000000000, 0.9898214418809326842, 1.000000000000000000, 0.9898214418809326842, 1.000000000000000000, 0.9898214418809326842, 1.000000000000000000, 0.9898214418809326842, 1.000000000000000000, 0.9898214418809326842, 1.000000000000000000, 0.9898214418809326842, 1.000000000000000000, 0.9898214418809326842, 1.000000000000000000, 0.9898214418809326842, 1.000000000000000000, 0.9898214418809326842, 1.000000000000000000, 0.9898214418809326842, 1.000000000000000000, 0.9898214418809326842, 1.000000000000000000, 0.9898214418809326842, 1.000000000000000000, 0.9898214418809326842, 1.000000000000000000, 0.9898214418809326842, 1.000000000000000000, 0.9898214418809326842, 1.000000000000000000, 0.9898214418809326842, 1.000000000000000000, 0.9898214418809326842, 1.000000000000000000, 0.9898214418809326842, 1.000000000000000000, 0.9898214418809326842, 1.000000000000000000, 0.9898214418809326842, 1.000000000000000000, 0.9898214418809326842, 1.000000000000000000, 0.9898214418809326842, 1.000000000000000000, 0.9898214418809326842, 1.000000000000000000, 0.9898214418809326842, 1.000000000000000000, 0.9898214418809326842, 1.000000000000000000, 0.9898214418809326842, 1.000000000000000000, 0.9898214418809326842, 1.000000000000000000, 0.9898214418809326842, 1.000000000000000000, 0.9898214418809326842, 1.000000000000000000, 0.9898214418809326842, 1.000000000000000000, 0.9898214418809326842, 1.000000000000000000, 0.9898214418809326842, 1.000000000000000000, 0.9898214418809326842, 1.000000000000000000, 0.9898214418809326842, 1.000000000000000000, 0.9898214418809326842, 1.000000000000000000, 0.9898214418809326842, 1.000000000000000000, 0.9898214418809326842, 1.000000000000000000, 0.9898214418809326842, 1.000000000000000000, 0.9898214418809326842, 1.000000000000000000, 0.9898214418809326842, 1.000000000000000000, 0.9898214418809326842, 1.000000000000000000, 0.9898214418809326842, 1.000000000000000000, 0.9898214418809326842, 1.000000000000000000, 0.9898214418809326842, 1.000000000000000000, 0.9898214418809326842, 1.000000000000000000, 0.9898214418809326842, 1.000000000000000000, 0.9898214418809326842, 1.000000000000000000, 0.9898214418809326842, 1.000000000000000000, 0.9898214418809326842, 1.000000000000000000, 0.9898214418809326842, 1.000000000000000000, 0.9898214418809326842, 1.000000000000000000, 0.9898214418809326842, 1.000000000000000000, 0.9898214418809326842, 1.000000000000000000, 0.9898214418809326842, 1.000000000000000000, 0.9898214418809326842, 1.000000000000000000, 0.9898214418809326842, 1.000000000000000000, 0.9898214418809326842, 1.000000000000000000, 0.9898214418809326842, 1.000000000000000000, 0.9898214418809326842, 1.000000000000000000, 0.9898214418809326842, 1.000000000000000000, 0.9898214418809326842, 1.000000000000000000, 0.9898214418809326842, 1.000000000000000000, 0.9898214418809326842, 1.000000000000000000, 0.9898214418809326842, 1.000000000000000000, 0.9898214418809326842, 1.000000000000000000, 0.9898214418809326842, 1.000000000000000000, 0.9898214418809326842, 1.000000000000000000, 0.9898214418809326842, 1.000000000000000000, 0.9898214418809326842, 1.000000000000000000, 0.9898214418809326842, 1.000000000000000000, 0.9898214418809326842, 1.000000000000000000, 0.9898214418809326842, 1.000000000000000000, 0.9898214418809326842, 1.000000000000000000, 0.9898214418809326842, 1.000000000000000000, 0.9898214418809326842, 1.000000000000000000, 0.9898214418809326842, 1.000000000000000000, 0.9898214418809326842, 1.000000000000000000, 0.9898214418809326842, 1.000000000000000000, 0.9898214418809326842, 1.000000000000000000, 0.9898214418809326842, 1.000000000000000000, 0.9898214418809326842, 1.000000000000000000, 0.9898214418809326842, 1.000000000000000000, 0.9898214418809326842, 1.000000000000000000, 0.9898214418809326842, 1.000000000000000000, 0.9898214418809326842, 1.000000000000000000, 0.9898214418809326842, 1.000000000000000000, 0.9898214418809326842, 1.000000000000000000, 0.9898214418809326842, 1.000000000000000000, 0.9898214418809326842, 1.000000000000000000, 0.9898214418809326842, 1.000000000000000000, 0.9898214418809326842, 1.000000000000000000, 0.9898214418809326842, 1.000000000000000000, 0.9898214418809326842, 1.000000000000000000, 0.9898214418809326842, 1.000000000000000000, 0.9898214418809326842, 1.000000000000000000, 0.9898214418809326842, 1.000000000000000000, 0.9898214418809326842, 1.000000000000000000, 0.9898214418809326842, 1.000000000000000000, 0.9898214418809326842, 1.000000000000000000, 0.9898214418809326842, 1.000000000000000000, 0.9898214418809326842, 1.000000000000000000, 0.9898214418809326842, 1.000000000000000000, 0.9898214418809326842, 1.000000000000000000, 0.9898214418809326842, 1.000000000000000000, 0.9898214418809326842, 1.000000000000000000, 0.9898214418809326842, 1.000000000000000000, 0.9898214418809326842, 1.000000000000000000, 0.9898214418809326842, 1.000000000000000000, 0.9898214418809326842, 1.000000000000000000, 0.9898214418809326842, 1.000000000000000000, 0.9898214418809326842, 1.000000000000000000, 0.9898214418809326842, 1.000000000000000000, 0.9898214418809326842, 1.000000000000000000, 0.9898214418809326842, 1.000000000000000000, 0.9898214418809326842, 1.000000000000000000, 0.9898214418809326842, 1.000000000000000000, 0.9898214418809326842, 1.000000000000000000, 0.9898214418809326842, 1.000000000000000000, 0.9898214418809326842, 1.000000000000000000, 0.9898214418809326842, 1.000000000000000000, 0.9898214418809326842, 1.000000000000000000, 0.9898214418809326842, 1.000000000000000000, 0.9898214418809326842, 1.000000000000000000, 0.9898214418809326842, 1.000000000000000000, 0.9898214418809326842, 1.000000000000000000, 0.9898214418809326842, 1.000000000000000000, 0.9898214418809326842, 1.000000000000000000, 0.9898214418809326842, 1.000000000000000000, 0.9898214418809326842, 1.000000000000000000, 0.9898214418809326842, 1.000000000000000000, 0.9898214418809326842, 1.000000000000000000, 0.9898214418809326842, 1.000000000000000000, 0.9898214418809326842, 1.000000000000000000, 0.9898214418809326842, 1.000000000000000000, 0.9898214418809326842, 1.000000000000000000, 0.9898214418809326842, 1.000000000000000000, 0.9898214418809326842, 1.000000000000000000, 0.9898214418809326842, 1.000000000000000000, 0.9898214418809326842, 1.000000000000000000, 0.9898214418809326842, 1.000000000000000000, 0.9898214418809326842, 1.000000000000000000, 0.9898214418809326842, 1.000000000000000000, 0.9898214418809326842, 1.000000000000000000, 0.9898214418809326842, 1.000000000000000000, 0.9898214418809326842, 1.000000000000000000, 0.9898214418809326842, 1.000000000000000000, 0.9898214418809326842, 1.000000000000000000, 0.9898214418809326842, 1.000000000000000000, 0.9898214418809326842, 1.000000000000000000, 0.9898214418809326842, 1.000000000000000000, 0.9898214418809326842, 1.000000000000000000, 0.9898214418809326842, 1.000000000000000000, 0.9898214418809326842, 1.000000000000000000, 0.9898214418809326842, 1.000000000000000000, 0.9898214418809326842, 1.000000000000000000, 0.9898214418809326842, 1.000000000000000000, 0.9898214418809326842, 1.000000000000000000, 0.9898214418809326842, 1.000000000000000000, 0.9898214418809326842, 1.000000000000000000, 0.9898214418809326842, 1.000000000000000000, 0.9898214418809326842, 1.000000000000000000, 0.9898214418809326842, 1.000000000000000000, 0.9898214418809326842, 1.000000000000000000, 0.9898214418809326842, 1.000000000000000000, 0.9898214418809326842, 1.000000000000000000, 0.9898214418809326842, 1.000000000000000000, 0.9898214418809326842, 1.000000000000000000, 0.9898214418809326842, 1.000000000000000000, 0.9898214418809326842, 1.000000000000000000, 0.9898214418809326842, 1.000000000000000000, 0.9898214418809326842, 1.000000000000000000, 0.9898214418809326842, 1.000000000000000000, 0.9898214418809326842, 1.000000000000000000, 0.9898214418809326842, 1.000000000000000000, 0.9898214418809326842, 1.000000000000000000, 0.9898214418809326842, 1.000000000000000000, 0.9898214418809326842, 1.000000000000000000, 0.9898214418809326842, 1.000000000000000000, 0.9898214418809326842, 1.000000000000000000, 0.9898214418809326842, 1.000000000000000000, 0.9898214418809326842, 1.000000000000000000, 0.9898214418809326842, 1.000000000000000000, 0.9898214418809326842, 1.000000000000000000, 0.9898214418809326842, 1.000000000000000000, 0.9898214418809326842, 1.000000000000000000, 0.9898214418809326842, 1.000000000000000000, 0.9898214418809326842, 1.000000000000000000, 0.9898214418809326842, 1.000000000000000000, 0.9898214418809326842, 1.000000000000000000, 0.9898214418809326842, 1.000000000000000000, 0.9898214418809326842, 1.000000000000000000, 0.9898214418809326842, 1.000000000000000000, 0.9898214418809326842, 1.000000000000000000, 0.9898214418809326842, 1.000000000000000000, 0.9898214418809326842, 1.000000000000000000, 0.9898214418809326842, 1.000000000000000000, 0.9898214418809326842, 1.000000000000000000, 0.9898214418809326842, 1.000000000000000000, 0.9898214418809326842, 1.000000000000000000, 0.9898214418809326842, 1.000000000000000000, 0.9898214418809326842, 1.000000000000000000, 0.9898214418809326842, 1.000000000000000000, 0.9898214418809326842, 1.000000000000000000, 0.9898214418809326842, 1.000000000000000000, 0.9898214418809326842, 1.000000000000000000, 0.9898214418809326842, 1.000000000000000000, 0.9898214418809326842, 1.000000000000000000, 0.9898214418809326842, 1.000000000000000000, 0.9898214418809326842, 1.000000000000000000, 0.9898214418809326842, 1.000000000000000000, 0.9898214418809326842, 1.000000000000000000, 0.9898214418809326842, 1.000000000000000000, 0.9898214418809326842, 1.000000000000000000, 0.9898214418809326842, 1.000000000000000000, 0.9898214418809326842, 1.000000000000000000, 0.9898214418809326842, 1.000000000000000000, 0.9898214418809326842, 1.000000000000000000, 0.9898214418809326842, 1.000000000000000000, 0.9898214418809326842, 1.000000000000000000, 0.9898214418809326842, 1.000000000000000000, 0.9898214418809326842, 1.000000000000000000, 0.9898214418809326842, 1.000000000000000000, 0.9898214418809326842, 1.000000000000000000, 0.9898214418809326842, 1.000000000000000000, 0.9898214418809326842, 1.000000000000000000, 0.9898214418809326842, 1.000000000000000000, 0.9898214418809326842, 1.000000000000000000, 0.9898214418809326842, 1.000000000000000000, 0.9898214418809326842, 1.000000000000000000, 0.9898214418809326842, 1.000000000000000000, 0.9898214418809326842, 1.000000000000000000, 0.9898214418809326842, 1.000000000000000000, 0.9898214418809326842, 1.000000000000000000, 0.9898214418809326842, 1.000000000000000000, 0.9898214418809326842, 1.000000000000000000, 0.9898214418809326842, 1.000000000000000000, 0.9898214418809326842, 1.000000000000000000, 0.9898214418809326842, 1.000000000000000000, 0.9898214418809326842, 1.000000000000000000, 0.9898214418809326842, 1.000000000000000000, 0.9898214418809326842, 1.000000000000000000, 0.9898214418809326842, 1.000000000000000000, 0.9898214418809326842, 1.000000000000000000, 0.9898214418809326842, 1.000000000000000000, 0.9898214418809326842, 1.000000000000000000, 0.9898214418809326842, 1.000000000000000000, 0.9898214418809326842, 1.000000000000000000, 0.9898214418809326842, 1.000000000000000000, 0.9898214418809326842, 1.000000000000000000, 0.9898214418809326842, 1.000000000000000000, 0.9898214418809326842, 1.000000000000000000, 0.9898214418809326842, 1.000000000000000000, 0.9898214418809326842, 1.000000000000000000, 0.9898214418809326842, 1.000000000000000000, 0.9898214418809326842, 1.000000000000000000, 0.9898214418809326842, 1.000000000000000000, 0.9898214418809326842, 1.000000000000000000, 0.9898214418809326842, 1.000000000000000000, 0.9898214418809326842, 1.000000000000000000, 0.9898214418809326842, 1.000000000000000000, 0.9898214418809326842, 1.000000000000000000, 0.9898214418809326842, 1.000000000000000000, 0.9898214418809326842, 1.000000000000000000, 0.9898214418809326842, 1.000000000000000000, 0.9898214418809326842, 1.000000000000000000, 0.9898214418809326842, 1.000000000000000000, 0.9898214418809326842, 1.000000000000000000, 0.9898214418809326842, 1.000000000000000000, 0.9898214418809326842, 1.000000000000000000, 0.9898214418809326842, 1.000000000000000000, 0.9898214418809326842, 1.000000000000000000, 0.9898214418809326842, 1.000000000000000000, 0.9961809353924466759, 0.9952277490961531914),
 ( 0.3333333333333333703, 0.3299404806269776169, 0.3333333333333333703, 0.3299404806269776169, 0.3333333333333333703, 0.3299404806269776169, 0.3333333333333333703, 0.3299404806269776169, 0.3333333333333333703, 0.3299404806269776169, 0.3333333333333333703, 0.3299404806269776169, 0.3333333333333333703, 0.3299404806269776169, 0.3333333333333333703, 0.3299404806269776169, 0.3333333333333333703, 0.3299404806269776169, 0.3333333333333333703, 0.3299404806269776169, 0.3333333333333333703, 0.3299404806269776169, 0.3333333333333333703, 0.3299404806269776169, 0.3333333333333333703, 0.3299404806269776169, 0.3333333333333333703, 0.3299404806269776169, 0.3333333333333333703, 0.3299404806269776169, 0.3333333333333333703, 0.3299404806269776169, 0.3333333333333333703, 0.3299404806269776169, 0.3333333333333333703, 0.3299404806269776169, 0.3333333333333333703, 0.3299404806269776169, 0.3333333333333333703, 0.3299404806269776169, 0.3333333333333333703, 0.3299404806269776169, 0.3333333333333333703, 0.3299404806269776169, 0.3333333333333333703, 0.3299404806269776169, 0.3333333333333333703, 0.3299404806269776169, 0.3333333333333333703, 0.3299404806269776169, 0.3333333333333333703, 0.3299404806269776169, 0.3333333333333333703, 0.3299404806269776169, 0.3333333333333333703, 0.3299404806269776169, 0.3333333333333333703, 0.3299404806269776169, 0.3333333333333333703, 0.3299404806269776169, 0.3333333333333333703, 0.3299404806269776169, 0.3333333333333333703, 0.3299404806269776169, 0.3333333333333333703, 0.3299404806269776169, 0.3333333333333333703, 0.3299404806269776169, 0.3333333333333333703, 0.3299404806269776169, 0.3333333333333333703, 0.3299404806269776169, 0.3333333333333333703, 0.3299404806269776169, 0.3333333333333333703, 0.3299404806269776169, 0.3333333333333333703, 0.3299404806269776169, 0.3333333333333333703, 0.3299404806269776169, 0.3333333333333333703, 0.3299404806269776169, 0.3333333333333333703, 0.3299404806269776169, 0.3333333333333333703, 0.3299404806269776169, 0.3333333333333333703, 0.3299404806269776169, 0.3333333333333333703, 0.3299404806269776169, 0.3333333333333333703, 0.3299404806269776169, 0.3333333333333333703, 0.3299404806269776169, 0.3333333333333333703, 0.3299404806269776169, 0.3333333333333333703, 0.3299404806269776169, 0.3333333333333333703, 0.3299404806269776169, 0.3333333333333333703, 0.3299404806269776169, 0.3333333333333333703, 0.3299404806269776169, 0.3333333333333333703, 0.3299404806269776169, 0.3333333333333333703, 0.3299404806269776169, 0.3333333333333333703, 0.3299404806269776169, 0.3333333333333333703, 0.3299404806269776169, 0.3333333333333333703, 0.3299404806269776169, 0.3333333333333333703, 0.3299404806269776169, 0.3333333333333333703, 0.3299404806269776169, 0.3333333333333333703, 0.3299404806269776169, 0.3333333333333333703, 0.3299404806269776169, 0.3333333333333333703, 0.3299404806269776169, 0.3333333333333333703, 0.3299404806269776169, 0.3333333333333333703, 0.3299404806269776169, 0.3333333333333333703, 0.3299404806269776169, 0.3333333333333333703, 0.3299404806269776169, 0.3333333333333333703, 0.3299404806269776169, 0.3333333333333333703, 0.3299404806269776169, 0.3333333333333333703, 0.3299404806269776169, 0.3333333333333333703, 0.3299404806269776169, 0.3333333333333333703, 0.3299404806269776169, 0.3333333333333333703, 0.3299404806269776169, 0.3333333333333333703, 0.3299404806269776169, 0.3333333333333333703, 0.3299404806269776169, 0.3333333333333333703, 0.3299404806269776169, 0.3333333333333333703, 0.3299404806269776169, 0.3333333333333333703, 0.3299404806269776169, 0.3333333333333333703, 0.3299404806269776169, 0.3333333333333333703, 0.3299404806269776169, 0.3333333333333333703, 0.3299404806269776169, 0.3333333333333333703, 0.3299404806269776169, 0.3333333333333333703, 0.3299404806269776169, 0.3333333333333333703, 0.3299404806269776169, 0.3333333333333333703, 0.3299404806269776169, 0.3333333333333333703, 0.3299404806269776169, 0.3333333333333333703, 0.3299404806269776169, 0.3333333333333333703, 0.3299404806269776169, 0.3333333333333333703, 0.3299404806269776169, 0.3333333333333333703, 0.3299404806269776169, 0.3333333333333333703, 0.3299404806269776169, 0.3333333333333333703, 0.3299404806269776169, 0.3333333333333333703, 0.3299404806269776169, 0.3333333333333333703, 0.3299404806269776169, 0.3333333333333333703, 0.3299404806269776169, 0.3333333333333333703, 0.3299404806269776169, 0.3333333333333333703, 0.3299404806269776169, 0.3333333333333333703, 0.3299404806269776169, 0.3333333333333333703, 0.3299404806269776169, 0.3333333333333333703, 0.3299404806269776169, 0.3333333333333333703, 0.3299404806269776169, 0.3333333333333333703, 0.3299404806269776169, 0.3333333333333333703, 0.3299404806269776169, 0.3333333333333333703, 0.3299404806269776169, 0.3333333333333333703, 0.3299404806269776169, 0.3333333333333333703, 0.3299404806269776169, 0.3333333333333333703, 0.3299404806269776169, 0.3333333333333333703, 0.3299404806269776169, 0.3333333333333333703, 0.3299404806269776169, 0.3333333333333333703, 0.3299404806269776169, 0.3333333333333333703, 0.3299404806269776169, 0.3333333333333333703, 0.3299404806269776169, 0.3333333333333333703, 0.3299404806269776169, 0.3333333333333333703, 0.3299404806269776169, 0.3333333333333333703, 0.3299404806269776169, 0.3333333333333333703, 0.3299404806269776169, 0.3333333333333333703, 0.3299404806269776169, 0.3333333333333333703, 0.3299404806269776169, 0.3333333333333333703, 0.3299404806269776169, 0.3333333333333333703, 0.3299404806269776169, 0.3333333333333333703, 0.3299404806269776169, 0.3333333333333333703, 0.3299404806269776169, 0.3333333333333333703, 0.3299404806269776169, 0.3333333333333333703, 0.3299404806269776169, 0.3333333333333333703, 0.3299404806269776169, 0.3333333333333333703, 0.3299404806269776169, 0.3333333333333333703, 0.3299404806269776169, 0.3333333333333333703, 0.3299404806269776169, 0.3333333333333333703, 0.3299404806269776169, 0.3333333333333333703, 0.3299404806269776169, 0.3333333333333333703, 0.3299404806269776169, 0.3333333333333333703, 0.3299404806269776169, 0.3333333333333333703, 0.3299404806269776169, 0.3333333333333333703, 0.3299404806269776169, 0.3333333333333333703, 0.3299404806269776169, 0.3333333333333333703, 0.3299404806269776169, 0.3333333333333333703, 0.3299404806269776169, 0.3333333333333333703, 0.3299404806269776169, 0.3333333333333333703, 0.3299404806269776169, 0.3333333333333333703, 0.3299404806269776169, 0.3333333333333333703, 0.3299404806269776169, 0.3333333333333333703, 0.3299404806269776169, 0.3333333333333333703, 0.3299404806269776169, 0.3333333333333333703, 0.3299404806269776169, 0.3333333333333333703, 0.3299404806269776169, 0.3333333333333333703, 0.3299404806269776169, 0.3333333333333333703, 0.3299404806269776169, 0.3333333333333333703, 0.3299404806269776169, 0.3333333333333333703, 0.3299404806269776169, 0.3333333333333333703, 0.3299404806269776169, 0.3333333333333333703, 0.3299404806269776169, 0.3333333333333333703, 0.3299404806269776169, 0.3333333333333333703, 0.3299404806269776169, 0.3333333333333333703, 0.3299404806269776169, 0.3333333333333333703, 0.3299404806269776169, 0.3333333333333333703, 0.3299404806269776169, 0.3333333333333333703, 0.3299404806269776169, 0.3333333333333333703, 0.3299404806269776169, 0.3333333333333333703, 0.3299404806269776169, 0.3333333333333333703, 0.3299404806269776169, 0.3333333333333333703, 0.3299404806269776169, 0.3333333333333333703, 0.3299404806269776169, 0.3333333333333333703, 0.3299404806269776169, 0.3333333333333333703, 0.3299404806269776169, 0.3333333333333333703, 0.3299404806269776169, 0.3333333333333333703, 0.3299404806269776169, 0.3333333333333333703, 0.3299404806269776169, 0.3333333333333333703, 0.3299404806269776169, 0.3333333333333333703, 0.3299404806269776169, 0.3333333333333333703, 0.3299404806269776169, 0.3333333333333333703, 0.3299404806269776169, 0.3333333333333333703, 0.3299404806269776169, 0.3333333333333333703, 0.3299404806269776169, 0.3333333333333333703, 0.3299404806269776169, 0.3333333333333333703, 0.3299404806269776169, 0.3333333333333333703, 0.3299404806269776169, 0.3333333333333333703, 0.3299404806269776169, 0.3333333333333333703, 0.3299404806269776169, 0.3333333333333333703, 0.3299404806269776169, 0.3333333333333333703, 0.3299404806269776169, 0.3333333333333333703, 0.3299404806269776169, 0.3333333333333333703, 0.3299404806269776169, 0.3333333333333333703, 0.3299404806269776169, 0.3333333333333333703, 0.3299404806269776169, 0.3333333333333333703, 0.3299404806269776169, 0.3333333333333333703, 0.3299404806269776169, 0.3333333333333333703, 0.3299404806269776169, 0.3333333333333333703, 0.3299404806269776169, 0.3333333333333333703, 0.3299404806269776169, 0.3333333333333333703, 0.3299404806269776169, 0.3333333333333333703, 0.3299404806269776169, 0.3333333333333333703, 0.3299404806269776169, 0.3333333333333333703, 0.3299404806269776169, 0.3333333333333333703, 0.3299404806269776169, 0.3333333333333333703, 0.3299404806269776169, 0.3333333333333333703, 0.3299404806269776169, 0.3333333333333333703, 0.3299404806269776169, 0.3333333333333333703, 0.3299404806269776169, 0.3333333333333333703, 0.3299404806269776169, 0.3333333333333333703, 0.3299404806269776169, 0.3333333333333333703, 0.3299404806269776169, 0.3333333333333333703, 0.3299404806269776169, 0.3333333333333333703, 0.3299404806269776169, 0.3333333333333333703, 0.3299404806269776169, 0.3333333333333333703, 0.3299404806269776169, 0.3333333333333333703, 0.3299404806269776169, 0.3333333333333333703, 0.3299404806269776169, 0.3333333333333333703, 0.3299404806269776169, 0.3333333333333333703, 0.3299404806269776169, 0.3333333333333333703, 0.3299404806269776169, 0.3333333333333333703, 0.3299404806269776169, 0.3333333333333333703, 0.3299404806269776169, 0.3333333333333333703, 0.3299404806269776169, 0.3333333333333333703, 0.3299404806269776169, 0.3333333333333333703, 0.3299404806269776169, 0.3333333333333333703, 0.3299404806269776169, 0.3333333333333333703, 0.3299404806269776169, 0.3333333333333333703, 0.3299404806269776169, 0.3333333333333333703, 0.3299404806269776169, 0.3333333333333333703, 0.3299404806269776169, 0.3333333333333333703, 0.3299404806269776169, 0.3333333333333333703, 0.3299404806269776169, 0.3333333333333333703, 0.3299404806269776169, 0.3333333333333333703, 0.3299404806269776169, 0.3333333333333333703, 0.3299404806269776169, 0.3333333333333333703, 0.3299404806269776169, 0.3333333333333333703, 0.3299404806269776169, 0.3333333333333333703, 0.3299404806269776169, 0.3333333333333333703, 0.3299404806269776169, 0.3333333333333333703, 0.3299404806269776169, 0.3333333333333333703, 0.3299404806269776169, 0.3333333333333333703, 0.3299404806269776169, 0.3333333333333333703, 0.3299404806269776169, 0.3333333333333333703, 0.3299404806269776169, 0.3333333333333333703, 0.3299404806269776169, 0.3333333333333333703, 0.3299404806269776169, 0.3333333333333333703, 0.3299404806269776169, 0.3333333333333333703, 0.3299404806269776169, 0.3333333333333333703, 0.3299404806269776169, 0.3333333333333333703, 0.3299404806269776169, 0.3333333333333333703, 0.3299404806269776169, 0.3333333333333333703, 0.3299404806269776169, 0.3333333333333333703, 0.3299404806269776169, 0.3333333333333333703, 0.3299404806269776169, 0.3333333333333333703, 0.3299404806269776169, 0.3333333333333333703, 0.3299404806269776169, 0.3333333333333333703, 0.3299404806269776169, 0.3333333333333333703, 0.3299404806269776169, 0.3333333333333333703, 0.3299404806269776169, 0.3333333333333333703, 0.3299404806269776169, 0.3333333333333333703, 0.3299404806269776169, 0.3333333333333333703, 0.3299404806269776169, 0.3333333333333333703, 0.3299404806269776169, 0.3333333333333333703, 0.3299404806269776169, 0.3333333333333333703, 0.3299404806269776169, 0.3333333333333333703, 0.3299404806269776169, 0.3333333333333333703, 0.3299404806269776169, 0.3333333333333333703, 0.3299404806269776169, 0.3333333333333333703, 0.3299404806269776169, 0.3333333333333333703, 0.3299404806269776169, 0.3333333333333333703, 0.3299404806269776169, 0.3333333333333333703, 0.3299404806269776169, 0.3333333333333333703, 0.3299404806269776169, 0.3333333333333333703, 0.3299404806269776169, 0.3333333333333333703, 0.3299404806269776169, 0.3333333333333333703, 0.3299404806269776169, 0.3333333333333333703, 0.3299404806269776169, 0.3333333333333333703, 0.3299404806269776169, 0.3333333333333333703, 0.3299404806269776169, 0.3333333333333333703, 0.3299404806269776169, 0.3333333333333333703, 0.3299404806269776169, 0.3333333333333333703, 0.3299404806269776169, 0.3333333333333333703, 0.3299404806269776169, 0.3333333333333333703, 0.3299404806269776169, 0.3333333333333333703, 0.3299404806269776169, 0.3333333333333333703, 0.3299404806269776169, 0.3333333333333333703, 0.3299404806269776169, 0.3333333333333333703, 0.3299404806269776169, 0.3333333333333333703, 0.3299404806269776169, 0.3333333333333333703, 0.3299404806269776169, 0.3333333333333333703, 0.3299404806269776169, 0.3333333333333333703, 0.3299404806269776169, 0.3333333333333333703, 0.3299404806269776169, 0.3333333333333333703, 0.3299404806269776169, 0.3333333333333333703, 0.3299404806269776169, 0.3333333333333333703, 0.3299404806269776169, 0.3333333333333333703, 0.3299404806269776169, 0.3333333333333333703, 0.3299404806269776169, 0.3333333333333333703, 0.3299404806269776169, 0.3333333333333333703, 0.3299404806269776169, 0.3333333333333333703, 0.3299404806269776169, 0.3333333333333333703, 0.3299404806269776169, 0.3333333333333333703, 0.3299404806269776169, 0.3333333333333333703, 0.3299404806269776169, 0.3333333333333333703, 0.3299404806269776169, 0.3333333333333333703, 0.3299404806269776169, 0.3333333333333333703, 0.3299404806269776169, 0.3333333333333333703, 0.3299404806269776169, 0.3333333333333333703, 0.3299404806269776169, 0.3333333333333333703, 0.3299404806269776169, 0.3333333333333333703, 0.3299404806269776169, 0.3333333333333333703, 0.3299404806269776169, 0.3333333333333333703, 0.3299404806269776169, 0.3333333333333333703, 0.3299404806269776169, 0.3333333333333333703, 0.3299404806269776169, 0.3333333333333333703, 0.3299404806269776169, 0.3333333333333333703, 0.3299404806269776169, 0.3333333333333333703, 0.3299404806269776169, 0.3333333333333333703, 0.3299404806269776169, 0.3333333333333333703, 0.3299404806269776169, 0.3333333333333333703, 0.3299404806269776169, 0.3333333333333333703, 0.3299404806269776169, 0.3333333333333333703, 0.3299404806269776169, 0.3333333333333333703, 0.3299404806269776169, 0.3333333333333333703, 0.3299404806269776169, 0.3333333333333333703, 0.3299404806269776169, 0.3333333333333333703, 0.3299404806269776169, 0.3333333333333333703, 0.3299404806269776169, 0.3333333333333333703, 0.3299404806269776169, 0.3333333333333333703, 0.3299404806269776169, 0.3333333333333333703, 0.3299404806269776169, 0.3333333333333333703, 0.3299404806269776169, 0.3333333333333333703, 0.3299404806269776169, 0.3333333333333333703, 0.3299404806269776169, 0.3333333333333333703, 0.3299404806269776169, 0.3333333333333333703, 0.3299404806269776169, 0.3333333333333333703, 0.3299404806269776169, 0.3333333333333333703, 0.3299404806269776169, 0.3333333333333333703, 0.3299404806269776169, 0.3333333333333333703, 0.3299404806269776169, 0.3333333333333333703, 0.3299404806269776169, 0.3333333333333333703, 0.3299404806269776169, 0.3333333333333333703, 0.3299404806269776169, 0.3333333333333333703, 0.3299404806269776169, 0.3333333333333333703, 0.3299404806269776169, 0.3333333333333333703, 0.3299404806269776169, 0.3333333333333333703, 0.3299404806269776169, 0.3333333333333333703, 0.3299404806269776169, 0.3333333333333333703, 0.3299404806269776169, 0.3333333333333333703, 0.3299404806269776169, 0.3333333333333333703, 0.3299404806269776169, 0.3333333333333333703, 0.3299404806269776169, 0.3333333333333333703, 0.3299404806269776169, 0.3333333333333333703, 0.3299404806269776169, 0.3333333333333333703, 0.3299404806269776169, 0.3333333333333333703, 0.3299404806269776169, 0.3333333333333333703, 0.3299404806269776169, 0.3333333333333333703, 0.3299404806269776169, 0.3333333333333333703, 0.3299404806269776169, 0.3333333333333333703, 0.3299404806269776169, 0.3333333333333333703, 0.3299404806269776169, 0.3333333333333333703, 0.3299404806269776169, 0.3333333333333333703, 0.3299404806269776169, 0.3333333333333333703, 0.3299404806269776169, 0.3333333333333333703, 0.3299404806269776169, 0.3333333333333333703, 0.3299404806269776169, 0.3333333333333333703, 0.3299404806269776169, 0.3333333333333333703, 0.3299404806269776169, 0.3333333333333333703, 0.3299404806269776169, 0.3333333333333333703, 0.3299404806269776169, 0.3333333333333333703, 0.3299404806269776169, 0.3333333333333333703, 0.3299404806269776169, 0.3333333333333333703, 0.3299404806269776169, 0.3333333333333333703, 0.3299404806269776169, 0.3333333333333333703, 0.3299404806269776169, 0.3333333333333333703, 0.3299404806269776169, 0.3333333333333333703, 0.3299404806269776169, 0.3333333333333333703, 0.3299404806269776169, 0.3333333333333333703, 0.3299404806269776169, 0.3333333333333333703, 0.3299404806269776169, 0.3333333333333333703, 0.3299404806269776169, 0.3333333333333333703, 0.3299404806269776169, 0.3333333333333333703, 0.3299404806269776169, 0.3333333333333333703, 0.3299404806269776169, 0.3333333333333333703, 0.3299404806269776169, 0.3333333333333333703, 0.3299404806269776169, 0.3333333333333333703, 0.3299404806269776169, 0.3333333333333333703, 0.3299404806269776169, 0.3333333333333333703, 0.3299404806269776169, 0.3333333333333333703, 0.3299404806269776169, 0.3333333333333333703, 0.3299404806269776169, 0.3333333333333333703, 0.3299404806269776169, 0.3333333333333333703, 0.3299404806269776169, 0.3333333333333333703, 0.3299404806269776169, 0.3333333333333333703, 0.3299404806269776169, 0.3333333333333333703, 0.3299404806269776169, 0.3333333333333333703, 0.3299404806269776169, 0.3333333333333333703, 0.3299404806269776169, 0.3333333333333333703, 0.3299404806269776169, 0.3333333333333333703, 0.3299404806269776169, 0.3333333333333333703, 0.3299404806269776169, 0.3333333333333333703, 0.3299404806269776169, 0.3333333333333333703, 0.3299404806269776169, 0.3333333333333333703, 0.3299404806269776169, 0.3333333333333333703, 0.3299404806269776169, 0.3333333333333333703, 0.3299404806269776169, 0.3333333333333333703, 0.3299404806269776169, 0.3333333333333333703, 0.3299404806269776169, 0.3333333333333333703, 0.3299404806269776169, 0.3333333333333333703, 0.3299404806269776169, 0.3333333333333333703, 0.3299404806269776169, 0.3333333333333333703, 0.3299404806269776169, 0.3333333333333333703, 0.3299404806269776169, 0.3333333333333333703, 0.3299404806269776169, 0.3333333333333333703, 0.3299404806269776169, 0.3333333333333333703, 0.3299404806269776169, 0.3333333333333333703, 0.3299404806269776169, 0.3333333333333333703, 0.3299404806269776169, 0.3333333333333333703, 0.3299404806269776169, 0.3333333333333333703, 0.3299404806269776169, 0.3333333333333333703, 0.3299404806269776169, 0.3333333333333333703, 0.3299404806269776169, 0.3333333333333333703, 0.3299404806269776169, 0.3333333333333333703, 0.3299404806269776169, 0.3333333333333333703, 0.3299404806269776169, 0.3333333333333333703, 0.3299404806269776169, 0.3333333333333333703, 0.3299404806269776169, 0.3333333333333333703, 0.3299404806269776169, 0.3333333333333333703, 0.3299404806269776169, 0.3333333333333333703, 0.3299404806269776169, 0.3333333333333333703, 0.3299404806269776169, 0.3333333333333333703, 0.3299404806269776169, 0.3333333333333333703, 0.3299404806269776169, 0.3333333333333333703, 0.3299404806269776169, 0.3333333333333333703, 0.3299404806269776169, 0.3333333333333333703, 0.3299404806269776169, 0.3333333333333333703, 0.3299404806269776169, 0.3333333333333333703, 0.3299404806269776169, 0.3333333333333333703, 0.3299404806269776169, 0.3333333333333333703, 0.3299404806269776169, 0.3333333333333333703, 0.3299404806269776169, 0.3333333333333333703, 0.3320603117974822438, 0.3317425830320511193),
 ( 0.3333333333333333703, 0.3299404806269776169, 0.3333333333333333703, 0.3299404806269776169, 0.3333333333333333703, 0.3299404806269776169, 0.3333333333333333703, 0.3299404806269776169, 0.3333333333333333703, 0.3299404806269776169, 0.3333333333333333703, 0.3299404806269776169, 0.3333333333333333703, 0.3299404806269776169, 0.3333333333333333703, 0.3299404806269776169, 0.3333333333333333703, 0.3299404806269776169, 0.3333333333333333703, 0.3299404806269776169, 0.3333333333333333703, 0.3299404806269776169, 0.3333333333333333703, 0.3299404806269776169, 0.3333333333333333703, 0.3299404806269776169, 0.3333333333333333703, 0.3299404806269776169, 0.3333333333333333703, 0.3299404806269776169, 0.3333333333333333703, 0.3299404806269776169, 0.3333333333333333703, 0.3299404806269776169, 0.3333333333333333703, 0.3299404806269776169, 0.3333333333333333703, 0.3299404806269776169, 0.3333333333333333703, 0.3299404806269776169, 0.3333333333333333703, 0.3299404806269776169, 0.3333333333333333703, 0.3299404806269776169, 0.3333333333333333703, 0.3299404806269776169, 0.3333333333333333703, 0.3299404806269776169, 0.3333333333333333703, 0.3299404806269776169, 0.3333333333333333703, 0.3299404806269776169, 0.3333333333333333703, 0.3299404806269776169, 0.3333333333333333703, 0.3299404806269776169, 0.3333333333333333703, 0.3299404806269776169, 0.3333333333333333703, 0.3299404806269776169, 0.3333333333333333703, 0.3299404806269776169, 0.3333333333333333703, 0.3299404806269776169, 0.3333333333333333703, 0.3299404806269776169, 0.3333333333333333703, 0.3299404806269776169, 0.3333333333333333703, 0.3299404806269776169, 0.3333333333333333703, 0.3299404806269776169, 0.3333333333333333703, 0.3299404806269776169, 0.3333333333333333703, 0.3299404806269776169, 0.3333333333333333703, 0.3299404806269776169, 0.3333333333333333703, 0.3299404806269776169, 0.3333333333333333703, 0.3299404806269776169, 0.3333333333333333703, 0.3299404806269776169, 0.3333333333333333703, 0.3299404806269776169, 0.3333333333333333703, 0.3299404806269776169, 0.3333333333333333703, 0.3299404806269776169, 0.3333333333333333703, 0.3299404806269776169, 0.3333333333333333703, 0.3299404806269776169, 0.3333333333333333703, 0.3299404806269776169, 0.3333333333333333703, 0.3299404806269776169, 0.3333333333333333703, 0.3299404806269776169, 0.3333333333333333703, 0.3299404806269776169, 0.3333333333333333703, 0.3299404806269776169, 0.3333333333333333703, 0.3299404806269776169, 0.3333333333333333703, 0.3299404806269776169, 0.3333333333333333703, 0.3299404806269776169, 0.3333333333333333703, 0.3299404806269776169, 0.3333333333333333703, 0.3299404806269776169, 0.3333333333333333703, 0.3299404806269776169, 0.3333333333333333703, 0.3299404806269776169, 0.3333333333333333703, 0.3299404806269776169, 0.3333333333333333703, 0.3299404806269776169, 0.3333333333333333703, 0.3299404806269776169, 0.3333333333333333703, 0.3299404806269776169, 0.3333333333333333703, 0.3299404806269776169, 0.3333333333333333703, 0.3299404806269776169, 0.3333333333333333703, 0.3299404806269776169, 0.3333333333333333703, 0.3299404806269776169, 0.3333333333333333703, 0.3299404806269776169, 0.3333333333333333703, 0.3299404806269776169, 0.3333333333333333703, 0.3299404806269776169, 0.3333333333333333703, 0.3299404806269776169, 0.3333333333333333703, 0.3299404806269776169, 0.3333333333333333703, 0.3299404806269776169, 0.3333333333333333703, 0.3299404806269776169, 0.3333333333333333703, 0.3299404806269776169, 0.3333333333333333703, 0.3299404806269776169, 0.3333333333333333703, 0.3299404806269776169, 0.3333333333333333703, 0.3299404806269776169, 0.3333333333333333703, 0.3299404806269776169, 0.3333333333333333703, 0.3299404806269776169, 0.3333333333333333703, 0.3299404806269776169, 0.3333333333333333703, 0.3299404806269776169, 0.3333333333333333703, 0.3299404806269776169, 0.3333333333333333703, 0.3299404806269776169, 0.3333333333333333703, 0.3299404806269776169, 0.3333333333333333703, 0.3299404806269776169, 0.3333333333333333703, 0.3299404806269776169, 0.3333333333333333703, 0.3299404806269776169, 0.3333333333333333703, 0.3299404806269776169, 0.3333333333333333703, 0.3299404806269776169, 0.3333333333333333703, 0.3299404806269776169, 0.3333333333333333703, 0.3299404806269776169, 0.3333333333333333703, 0.3299404806269776169, 0.3333333333333333703, 0.3299404806269776169, 0.3333333333333333703, 0.3299404806269776169, 0.3333333333333333703, 0.3299404806269776169, 0.3333333333333333703, 0.3299404806269776169, 0.3333333333333333703, 0.3299404806269776169, 0.3333333333333333703, 0.3299404806269776169, 0.3333333333333333703, 0.3299404806269776169, 0.3333333333333333703, 0.3299404806269776169, 0.3333333333333333703, 0.3299404806269776169, 0.3333333333333333703, 0.3299404806269776169, 0.3333333333333333703, 0.3299404806269776169, 0.3333333333333333703, 0.3299404806269776169, 0.3333333333333333703, 0.3299404806269776169, 0.3333333333333333703, 0.3299404806269776169, 0.3333333333333333703, 0.3299404806269776169, 0.3333333333333333703, 0.3299404806269776169, 0.3333333333333333703, 0.3299404806269776169, 0.3333333333333333703, 0.3299404806269776169, 0.3333333333333333703, 0.3299404806269776169, 0.3333333333333333703, 0.3299404806269776169, 0.3333333333333333703, 0.3299404806269776169, 0.3333333333333333703, 0.3299404806269776169, 0.3333333333333333703, 0.3299404806269776169, 0.3333333333333333703, 0.3299404806269776169, 0.3333333333333333703, 0.3299404806269776169, 0.3333333333333333703, 0.3299404806269776169, 0.3333333333333333703, 0.3299404806269776169, 0.3333333333333333703, 0.3299404806269776169, 0.3333333333333333703, 0.3299404806269776169, 0.3333333333333333703, 0.3299404806269776169, 0.3333333333333333703, 0.3299404806269776169, 0.3333333333333333703, 0.3299404806269776169, 0.3333333333333333703, 0.3299404806269776169, 0.3333333333333333703, 0.3299404806269776169, 0.3333333333333333703, 0.3299404806269776169, 0.3333333333333333703, 0.3299404806269776169, 0.3333333333333333703, 0.3299404806269776169, 0.3333333333333333703, 0.3299404806269776169, 0.3333333333333333703, 0.3299404806269776169, 0.3333333333333333703, 0.3299404806269776169, 0.3333333333333333703, 0.3299404806269776169, 0.3333333333333333703, 0.3299404806269776169, 0.3333333333333333703, 0.3299404806269776169, 0.3333333333333333703, 0.3299404806269776169, 0.3333333333333333703, 0.3299404806269776169, 0.3333333333333333703, 0.3299404806269776169, 0.3333333333333333703, 0.3299404806269776169, 0.3333333333333333703, 0.3299404806269776169, 0.3333333333333333703, 0.3299404806269776169, 0.3333333333333333703, 0.3299404806269776169, 0.3333333333333333703, 0.3299404806269776169, 0.3333333333333333703, 0.3299404806269776169, 0.3333333333333333703, 0.3299404806269776169, 0.3333333333333333703, 0.3299404806269776169, 0.3333333333333333703, 0.3299404806269776169, 0.3333333333333333703, 0.3299404806269776169, 0.3333333333333333703, 0.3299404806269776169, 0.3333333333333333703, 0.3299404806269776169, 0.3333333333333333703, 0.3299404806269776169, 0.3333333333333333703, 0.3299404806269776169, 0.3333333333333333703, 0.3299404806269776169, 0.3333333333333333703, 0.3299404806269776169, 0.3333333333333333703, 0.3299404806269776169, 0.3333333333333333703, 0.3299404806269776169, 0.3333333333333333703, 0.3299404806269776169, 0.3333333333333333703, 0.3299404806269776169, 0.3333333333333333703, 0.3299404806269776169, 0.3333333333333333703, 0.3299404806269776169, 0.3333333333333333703, 0.3299404806269776169, 0.3333333333333333703, 0.3299404806269776169, 0.3333333333333333703, 0.3299404806269776169, 0.3333333333333333703, 0.3299404806269776169, 0.3333333333333333703, 0.3299404806269776169, 0.3333333333333333703, 0.3299404806269776169, 0.3333333333333333703, 0.3299404806269776169, 0.3333333333333333703, 0.3299404806269776169, 0.3333333333333333703, 0.3299404806269776169, 0.3333333333333333703, 0.3299404806269776169, 0.3333333333333333703, 0.3299404806269776169, 0.3333333333333333703, 0.3299404806269776169, 0.3333333333333333703, 0.3299404806269776169, 0.3333333333333333703, 0.3299404806269776169, 0.3333333333333333703, 0.3299404806269776169, 0.3333333333333333703, 0.3299404806269776169, 0.3333333333333333703, 0.3299404806269776169, 0.3333333333333333703, 0.3299404806269776169, 0.3333333333333333703, 0.3299404806269776169, 0.3333333333333333703, 0.3299404806269776169, 0.3333333333333333703, 0.3299404806269776169, 0.3333333333333333703, 0.3299404806269776169, 0.3333333333333333703, 0.3299404806269776169, 0.3333333333333333703, 0.3299404806269776169, 0.3333333333333333703, 0.3299404806269776169, 0.3333333333333333703, 0.3299404806269776169, 0.3333333333333333703, 0.3299404806269776169, 0.3333333333333333703, 0.3299404806269776169, 0.3333333333333333703, 0.3299404806269776169, 0.3333333333333333703, 0.3299404806269776169, 0.3333333333333333703, 0.3299404806269776169, 0.3333333333333333703, 0.3299404806269776169, 0.3333333333333333703, 0.3299404806269776169, 0.3333333333333333703, 0.3299404806269776169, 0.3333333333333333703, 0.3299404806269776169, 0.3333333333333333703, 0.3299404806269776169, 0.3333333333333333703, 0.3299404806269776169, 0.3333333333333333703, 0.3299404806269776169, 0.3333333333333333703, 0.3299404806269776169, 0.3333333333333333703, 0.3299404806269776169, 0.3333333333333333703, 0.3299404806269776169, 0.3333333333333333703, 0.3299404806269776169, 0.3333333333333333703, 0.3299404806269776169, 0.3333333333333333703, 0.3299404806269776169, 0.3333333333333333703, 0.3299404806269776169, 0.3333333333333333703, 0.3299404806269776169, 0.3333333333333333703, 0.3299404806269776169, 0.3333333333333333703, 0.3299404806269776169, 0.3333333333333333703, 0.3299404806269776169, 0.3333333333333333703, 0.3299404806269776169, 0.3333333333333333703, 0.3299404806269776169, 0.3333333333333333703, 0.3299404806269776169, 0.3333333333333333703, 0.3299404806269776169, 0.3333333333333333703, 0.3299404806269776169, 0.3333333333333333703, 0.3299404806269776169, 0.3333333333333333703, 0.3299404806269776169, 0.3333333333333333703, 0.3299404806269776169, 0.3333333333333333703, 0.3299404806269776169, 0.3333333333333333703, 0.3299404806269776169, 0.3333333333333333703, 0.3299404806269776169, 0.3333333333333333703, 0.3299404806269776169, 0.3333333333333333703, 0.3299404806269776169, 0.3333333333333333703, 0.3299404806269776169, 0.3333333333333333703, 0.3299404806269776169, 0.3333333333333333703, 0.3299404806269776169, 0.3333333333333333703, 0.3299404806269776169, 0.3333333333333333703, 0.3299404806269776169, 0.3333333333333333703, 0.3299404806269776169, 0.3333333333333333703, 0.3299404806269776169, 0.3333333333333333703, 0.3299404806269776169, 0.3333333333333333703, 0.3299404806269776169, 0.3333333333333333703, 0.3299404806269776169, 0.3333333333333333703, 0.3299404806269776169, 0.3333333333333333703, 0.3299404806269776169, 0.3333333333333333703, 0.3299404806269776169, 0.3333333333333333703, 0.3299404806269776169, 0.3333333333333333703, 0.3299404806269776169, 0.3333333333333333703, 0.3299404806269776169, 0.3333333333333333703, 0.3299404806269776169, 0.3333333333333333703, 0.3299404806269776169, 0.3333333333333333703, 0.3299404806269776169, 0.3333333333333333703, 0.3299404806269776169, 0.3333333333333333703, 0.3299404806269776169, 0.3333333333333333703, 0.3299404806269776169, 0.3333333333333333703, 0.3299404806269776169, 0.3333333333333333703, 0.3299404806269776169, 0.3333333333333333703, 0.3299404806269776169, 0.3333333333333333703, 0.3299404806269776169, 0.3333333333333333703, 0.3299404806269776169, 0.3333333333333333703, 0.3299404806269776169, 0.3333333333333333703, 0.3299404806269776169, 0.3333333333333333703, 0.3299404806269776169, 0.3333333333333333703, 0.3299404806269776169, 0.3333333333333333703, 0.3299404806269776169, 0.3333333333333333703, 0.3299404806269776169, 0.3333333333333333703, 0.3299404806269776169, 0.3333333333333333703, 0.3299404806269776169, 0.3333333333333333703, 0.3299404806269776169, 0.3333333333333333703, 0.3299404806269776169, 0.3333333333333333703, 0.3299404806269776169, 0.3333333333333333703, 0.3299404806269776169, 0.3333333333333333703, 0.3299404806269776169, 0.3333333333333333703, 0.3299404806269776169, 0.3333333333333333703, 0.3299404806269776169, 0.3333333333333333703, 0.3299404806269776169, 0.3333333333333333703, 0.3299404806269776169, 0.3333333333333333703, 0.3299404806269776169, 0.3333333333333333703, 0.3299404806269776169, 0.3333333333333333703, 0.3299404806269776169, 0.3333333333333333703, 0.3299404806269776169, 0.3333333333333333703, 0.3299404806269776169, 0.3333333333333333703, 0.3299404806269776169, 0.3333333333333333703, 0.3299404806269776169, 0.3333333333333333703, 0.3299404806269776169, 0.3333333333333333703, 0.3299404806269776169, 0.3333333333333333703, 0.3299404806269776169, 0.3333333333333333703, 0.3299404806269776169, 0.3333333333333333703, 0.3299404806269776169, 0.3333333333333333703, 0.3299404806269776169, 0.3333333333333333703, 0.3299404806269776169, 0.3333333333333333703, 0.3299404806269776169, 0.3333333333333333703, 0.3299404806269776169, 0.3333333333333333703, 0.3299404806269776169, 0.3333333333333333703, 0.3299404806269776169, 0.3333333333333333703, 0.3299404806269776169, 0.3333333333333333703, 0.3299404806269776169, 0.3333333333333333703, 0.3299404806269776169, 0.3333333333333333703, 0.3299404806269776169, 0.3333333333333333703, 0.3299404806269776169, 0.3333333333333333703, 0.3299404806269776169, 0.3333333333333333703, 0.3299404806269776169, 0.3333333333333333703, 0.3299404806269776169, 0.3333333333333333703, 0.3299404806269776169, 0.3333333333333333703, 0.3299404806269776169, 0.3333333333333333703, 0.3299404806269776169, 0.3333333333333333703, 0.3299404806269776169, 0.3333333333333333703, 0.3299404806269776169, 0.3333333333333333703, 0.3299404806269776169, 0.3333333333333333703, 0.3299404806269776169, 0.3333333333333333703, 0.3299404806269776169, 0.3333333333333333703, 0.3299404806269776169, 0.3333333333333333703, 0.3299404806269776169, 0.3333333333333333703, 0.3299404806269776169, 0.3333333333333333703, 0.3299404806269776169, 0.3333333333333333703, 0.3299404806269776169, 0.3333333333333333703, 0.3299404806269776169, 0.3333333333333333703, 0.3299404806269776169, 0.3333333333333333703, 0.3299404806269776169, 0.3333333333333333703, 0.3299404806269776169, 0.3333333333333333703, 0.3299404806269776169, 0.3333333333333333703, 0.3299404806269776169, 0.3333333333333333703, 0.3299404806269776169, 0.3333333333333333703, 0.3299404806269776169, 0.3333333333333333703, 0.3299404806269776169, 0.3333333333333333703, 0.3299404806269776169, 0.3333333333333333703, 0.3299404806269776169, 0.3333333333333333703, 0.3299404806269776169, 0.3333333333333333703, 0.3299404806269776169, 0.3333333333333333703, 0.3299404806269776169, 0.3333333333333333703, 0.3299404806269776169, 0.3333333333333333703, 0.3299404806269776169, 0.3333333333333333703, 0.3299404806269776169, 0.3333333333333333703, 0.3299404806269776169, 0.3333333333333333703, 0.3299404806269776169, 0.3333333333333333703, 0.3299404806269776169, 0.3333333333333333703, 0.3299404806269776169, 0.3333333333333333703, 0.3299404806269776169, 0.3333333333333333703, 0.3299404806269776169, 0.3333333333333333703, 0.3299404806269776169, 0.3333333333333333703, 0.3299404806269776169, 0.3333333333333333703, 0.3299404806269776169, 0.3333333333333333703, 0.3299404806269776169, 0.3333333333333333703, 0.3299404806269776169, 0.3333333333333333703, 0.3299404806269776169, 0.3333333333333333703, 0.3299404806269776169, 0.3333333333333333703, 0.3299404806269776169, 0.3333333333333333703, 0.3299404806269776169, 0.3333333333333333703, 0.3299404806269776169, 0.3333333333333333703, 0.3299404806269776169, 0.3333333333333333703, 0.3299404806269776169, 0.3333333333333333703, 0.3299404806269776169, 0.3333333333333333703, 0.3299404806269776169, 0.3333333333333333703, 0.3299404806269776169, 0.3333333333333333703, 0.3299404806269776169, 0.3333333333333333703, 0.3299404806269776169, 0.3333333333333333703, 0.3299404806269776169, 0.3333333333333333703, 0.3299404806269776169, 0.3333333333333333703, 0.3299404806269776169, 0.3333333333333333703, 0.3299404806269776169, 0.3333333333333333703, 0.3299404806269776169, 0.3333333333333333703, 0.3299404806269776169, 0.3333333333333333703, 0.3299404806269776169, 0.3333333333333333703, 0.3299404806269776169, 0.3333333333333333703, 0.3299404806269776169, 0.3333333333333333703, 0.3299404806269776169, 0.3333333333333333703, 0.3299404806269776169, 0.3333333333333333703, 0.3299404806269776169, 0.3333333333333333703, 0.3299404806269776169, 0.3333333333333333703, 0.3299404806269776169, 0.3333333333333333703, 0.3299404806269776169, 0.3333333333333333703, 0.3299404806269776169, 0.3333333333333333703, 0.3299404806269776169, 0.3333333333333333703, 0.3299404806269776169, 0.3333333333333333703, 0.3299404806269776169, 0.3333333333333333703, 0.3299404806269776169, 0.3333333333333333703, 0.3299404806269776169, 0.3333333333333333703, 0.3299404806269776169, 0.3333333333333333703, 0.3299404806269776169, 0.3333333333333333703, 0.3299404806269776169, 0.3333333333333333703, 0.3299404806269776169, 0.3333333333333333703, 0.3299404806269776169, 0.3333333333333333703, 0.3299404806269776169, 0.3333333333333333703, 0.3299404806269776169, 0.3333333333333333703, 0.3299404806269776169, 0.3333333333333333703, 0.3299404806269776169, 0.3333333333333333703, 0.3299404806269776169, 0.3333333333333333703, 0.3299404806269776169, 0.3333333333333333703, 0.3299404806269776169, 0.3333333333333333703, 0.3299404806269776169, 0.3333333333333333703, 0.3299404806269776169, 0.3333333333333333703, 0.3299404806269776169, 0.3333333333333333703, 0.3299404806269776169, 0.3333333333333333703, 0.3299404806269776169, 0.3333333333333333703, 0.3299404806269776169, 0.3333333333333333703, 0.3299404806269776169, 0.3333333333333333703, 0.3299404806269776169, 0.3333333333333333703, 0.3299404806269776169, 0.3333333333333333703, 0.3299404806269776169, 0.3333333333333333703, 0.3299404806269776169, 0.3333333333333333703, 0.3299404806269776169, 0.3333333333333333703, 0.3299404806269776169, 0.3333333333333333703, 0.3299404806269776169, 0.3333333333333333703, 0.3299404806269776169, 0.3333333333333333703, 0.3299404806269776169, 0.3333333333333333703, 0.3299404806269776169, 0.3333333333333333703, 0.3299404806269776169, 0.3333333333333333703, 0.3299404806269776169, 0.3333333333333333703, 0.3299404806269776169, 0.3333333333333333703, 0.3299404806269776169, 0.3333333333333333703, 0.3299404806269776169, 0.3333333333333333703, 0.3299404806269776169, 0.3333333333333333703, 0.3299404806269776169, 0.3333333333333333703, 0.3299404806269776169, 0.3333333333333333703, 0.3299404806269776169, 0.3333333333333333703, 0.3299404806269776169, 0.3333333333333333703, 0.3299404806269776169, 0.3333333333333333703, 0.3299404806269776169, 0.3333333333333333703, 0.3299404806269776169, 0.3333333333333333703, 0.3299404806269776169, 0.3333333333333333703, 0.3299404806269776169, 0.3333333333333333703, 0.3299404806269776169, 0.3333333333333333703, 0.3299404806269776169, 0.3333333333333333703, 0.3299404806269776169, 0.3333333333333333703, 0.3299404806269776169, 0.3333333333333333703, 0.3299404806269776169, 0.3333333333333333703, 0.3299404806269776169, 0.3333333333333333703, 0.3299404806269776169, 0.3333333333333333703, 0.3299404806269776169, 0.3333333333333333703, 0.3299404806269776169, 0.3333333333333333703, 0.3299404806269776169, 0.3333333333333333703, 0.3299404806269776169, 0.3333333333333333703, 0.3299404806269776169, 0.3333333333333333703, 0.3299404806269776169, 0.3333333333333333703, 0.3299404806269776169, 0.3333333333333333703, 0.3299404806269776169, 0.3333333333333333703, 0.3299404806269776169, 0.3333333333333333703, 0.3299404806269776169, 0.3333333333333333703, 0.3299404806269776169, 0.3333333333333333703, 0.3299404806269776169, 0.3333333333333333703, 0.3320603117974822438, 0.3317425830320511193),
 ( 1.000000000000000000, 0.9898214418809326842, 1.000000000000000000, 0.9898214418809326842, 1.000000000000000000, 0.9898214418809326842, 1.000000000000000000, 0.9898214418809326842, 1.000000000000000000, 0.9898214418809326842, 1.000000000000000000, 0.9898214418809326842, 1.000000000000000000, 0.9898214418809326842, 1.000000000000000000, 0.9898214418809326842, 1.000000000000000000, 0.9898214418809326842, 1.000000000000000000, 0.9898214418809326842, 1.000000000000000000, 0.9898214418809326842, 1.000000000000000000, 0.9898214418809326842, 1.000000000000000000, 0.9898214418809326842, 1.000000000000000000, 0.9898214418809326842, 1.000000000000000000, 0.9898214418809326842, 1.000000000000000000, 0.9898214418809326842, 1.000000000000000000, 0.9898214418809326842, 1.000000000000000000, 0.9898214418809326842, 1.000000000000000000, 0.9898214418809326842, 1.000000000000000000, 0.9898214418809326842, 1.000000000000000000, 0.9898214418809326842, 1.000000000000000000, 0.9898214418809326842, 1.000000000000000000, 0.9898214418809326842, 1.000000000000000000, 0.9898214418809326842, 1.000000000000000000, 0.9898214418809326842, 1.000000000000000000, 0.9898214418809326842, 1.000000000000000000, 0.9898214418809326842, 1.000000000000000000, 0.9898214418809326842, 1.000000000000000000, 0.9898214418809326842, 1.000000000000000000, 0.9898214418809326842, 1.000000000000000000, 0.9898214418809326842, 1.000000000000000000, 0.9898214418809326842, 1.000000000000000000, 0.9898214418809326842, 1.000000000000000000, 0.9898214418809326842, 1.000000000000000000, 0.9898214418809326842, 1.000000000000000000, 0.9898214418809326842, 1.000000000000000000, 0.9898214418809326842, 1.000000000000000000, 0.9898214418809326842, 1.000000000000000000, 0.9898214418809326842, 1.000000000000000000, 0.9898214418809326842, 1.000000000000000000, 0.9898214418809326842, 1.000000000000000000, 0.9898214418809326842, 1.000000000000000000, 0.9898214418809326842, 1.000000000000000000, 0.9898214418809326842, 1.000000000000000000, 0.9898214418809326842, 1.000000000000000000, 0.9898214418809326842, 1.000000000000000000, 0.9898214418809326842, 1.000000000000000000, 0.9898214418809326842, 1.000000000000000000, 0.9898214418809326842, 1.000000000000000000, 0.9898214418809326842, 1.000000000000000000, 0.9898214418809326842, 1.000000000000000000, 0.9898214418809326842, 1.000000000000000000, 0.9898214418809326842, 1.000000000000000000, 0.9898214418809326842, 1.000000000000000000, 0.9898214418809326842, 1.000000000000000000, 0.9898214418809326842, 1.000000000000000000, 0.9898214418809326842, 1.000000000000000000, 0.9898214418809326842, 1.000000000000000000, 0.9898214418809326842, 1.000000000000000000, 0.9898214418809326842, 1.000000000000000000, 0.9898214418809326842, 1.000000000000000000, 0.9898214418809326842, 1.000000000000000000, 0.9898214418809326842, 1.000000000000000000, 0.9898214418809326842, 1.000000000000000000, 0.9898214418809326842, 1.000000000000000000, 0.9898214418809326842, 1.000000000000000000, 0.9898214418809326842, 1.000000000000000000, 0.9898214418809326842, 1.000000000000000000, 0.9898214418809326842, 1.000000000000000000, 0.9898214418809326842, 1.000000000000000000, 0.9898214418809326842, 1.000000000000000000, 0.9898214418809326842, 1.000000000000000000, 0.9898214418809326842, 1.000000000000000000, 0.9898214418809326842, 1.000000000000000000, 0.9898214418809326842, 1.000000000000000000, 0.9898214418809326842, 1.000000000000000000, 0.9898214418809326842, 1.000000000000000000, 0.9898214418809326842, 1.000000000000000000, 0.9898214418809326842, 1.000000000000000000, 0.9898214418809326842, 1.000000000000000000, 0.9898214418809326842, 1.000000000000000000, 0.9898214418809326842, 1.000000000000000000, 0.9898214418809326842, 1.000000000000000000, 0.9898214418809326842, 1.000000000000000000, 0.9898214418809326842, 1.000000000000000000, 0.9898214418809326842, 1.000000000000000000, 0.9898214418809326842, 1.000000000000000000, 0.9898214418809326842, 1.000000000000000000, 0.9898214418809326842, 1.000000000000000000, 0.9898214418809326842, 1.000000000000000000, 0.9898214418809326842, 1.000000000000000000, 0.9898214418809326842, 1.000000000000000000, 0.9898214418809326842, 1.000000000000000000, 0.9898214418809326842, 1.000000000000000000, 0.9898214418809326842, 1.000000000000000000, 0.9898214418809326842, 1.000000000000000000, 0.9898214418809326842, 1.000000000000000000, 0.9898214418809326842, 1.000000000000000000, 0.9898214418809326842, 1.000000000000000000, 0.9898214418809326842, 1.000000000000000000, 0.9898214418809326842, 1.000000000000000000, 0.9898214418809326842, 1.000000000000000000, 0.9898214418809326842, 1.000000000000000000, 0.9898214418809326842, 1.000000000000000000, 0.9898214418809326842, 1.000000000000000000, 0.9898214418809326842, 1.000000000000000000, 0.9898214418809326842, 1.000000000000000000, 0.9898214418809326842, 1.000000000000000000, 0.9898214418809326842, 1.000000000000000000, 0.9898214418809326842, 1.000000000000000000, 0.9898214418809326842, 1.000000000000000000, 0.9898214418809326842, 1.000000000000000000, 0.9898214418809326842, 1.000000000000000000, 0.9898214418809326842, 1.000000000000000000, 0.9898214418809326842, 1.000000000000000000, 0.9898214418809326842, 1.000000000000000000, 0.9898214418809326842, 1.000000000000000000, 0.9898214418809326842, 1.000000000000000000, 0.9898214418809326842, 1.000000000000000000, 0.9898214418809326842, 1.000000000000000000, 0.9898214418809326842, 1.000000000000000000, 0.9898214418809326842, 1.000000000000000000, 0.9898214418809326842, 1.000000000000000000, 0.9898214418809326842, 1.000000000000000000, 0.9898214418809326842, 1.000000000000000000, 0.9898214418809326842, 1.000000000000000000, 0.9898214418809326842, 1.000000000000000000, 0.9898214418809326842, 1.000000000000000000, 0.9898214418809326842, 1.000000000000000000, 0.9898214418809326842, 1.000000000000000000, 0.9898214418809326842, 1.000000000000000000, 0.9898214418809326842, 1.000000000000000000, 0.9898214418809326842, 1.000000000000000000, 0.9898214418809326842, 1.000000000000000000, 0.9898214418809326842, 1.000000000000000000, 0.9898214418809326842, 1.000000000000000000, 0.9898214418809326842, 1.000000000000000000, 0.9898214418809326842, 1.000000000000000000, 0.9898214418809326842, 1.000000000000000000, 0.9898214418809326842, 1.000000000000000000, 0.9898214418809326842, 1.000000000000000000, 0.9898214418809326842, 1.000000000000000000, 0.9898214418809326842, 1.000000000000000000, 0.9898214418809326842, 1.000000000000000000, 0.9898214418809326842, 1.000000000000000000, 0.9898214418809326842, 1.000000000000000000, 0.9898214418809326842, 1.000000000000000000, 0.9898214418809326842, 1.000000000000000000, 0.9898214418809326842, 1.000000000000000000, 0.9898214418809326842, 1.000000000000000000, 0.9898214418809326842, 1.000000000000000000, 0.9898214418809326842, 1.000000000000000000, 0.9898214418809326842, 1.000000000000000000, 0.9898214418809326842, 1.000000000000000000, 0.9898214418809326842, 1.000000000000000000, 0.9898214418809326842, 1.000000000000000000, 0.9898214418809326842, 1.000000000000000000, 0.9898214418809326842, 1.000000000000000000, 0.9898214418809326842, 1.000000000000000000, 0.9898214418809326842, 1.000000000000000000, 0.9898214418809326842, 1.000000000000000000, 0.9898214418809326842, 1.000000000000000000, 0.9898214418809326842, 1.000000000000000000, 0.9898214418809326842, 1.000000000000000000, 0.9898214418809326842, 1.000000000000000000, 0.9898214418809326842, 1.000000000000000000, 0.9898214418809326842, 1.000000000000000000, 0.9898214418809326842, 1.000000000000000000, 0.9898214418809326842, 1.000000000000000000, 0.9898214418809326842, 1.000000000000000000, 0.9898214418809326842, 1.000000000000000000, 0.9898214418809326842, 1.000000000000000000, 0.9898214418809326842, 1.000000000000000000, 0.9898214418809326842, 1.000000000000000000, 0.9898214418809326842, 1.000000000000000000, 0.9898214418809326842, 1.000000000000000000, 0.9898214418809326842, 1.000000000000000000, 0.9898214418809326842, 1.000000000000000000, 0.9898214418809326842, 1.000000000000000000, 0.9898214418809326842, 1.000000000000000000, 0.9898214418809326842, 1.000000000000000000, 0.9898214418809326842, 1.000000000000000000, 0.9898214418809326842, 1.000000000000000000, 0.9898214418809326842, 1.000000000000000000, 0.9898214418809326842, 1.000000000000000000, 0.9898214418809326842, 1.000000000000000000, 0.9898214418809326842, 1.000000000000000000, 0.9898214418809326842, 1.000000000000000000, 0.9898214418809326842, 1.000000000000000000, 0.9898214418809326842, 1.000000000000000000, 0.9898214418809326842, 1.000000000000000000, 0.9898214418809326842, 1.000000000000000000, 0.9898214418809326842, 1.000000000000000000, 0.9898214418809326842, 1.000000000000000000, 0.9898214418809326842, 1.000000000000000000, 0.9898214418809326842, 1.000000000000000000, 0.9898214418809326842, 1.000000000000000000, 0.9898214418809326842, 1.000000000000000000, 0.9898214418809326842, 1.000000000000000000, 0.9898214418809326842, 1.000000000000000000, 0.9898214418809326842, 1.000000000000000000, 0.9898214418809326842, 1.000000000000000000, 0.9898214418809326842, 1.000000000000000000, 0.9898214418809326842, 1.000000000000000000, 0.9898214418809326842, 1.000000000000000000, 0.9898214418809326842, 1.000000000000000000, 0.9898214418809326842, 1.000000000000000000, 0.9898214418809326842, 1.000000000000000000, 0.9898214418809326842, 1.000000000000000000, 0.9898214418809326842, 1.000000000000000000, 0.9898214418809326842, 1.000000000000000000, 0.9898214418809326842, 1.000000000000000000, 0.9898214418809326842, 1.000000000000000000, 0.9898214418809326842, 1.000000000000000000, 0.9898214418809326842, 1.000000000000000000, 0.9898214418809326842, 1.000000000000000000, 0.9898214418809326842, 1.000000000000000000, 0.9898214418809326842, 1.000000000000000000, 0.9898214418809326842, 1.000000000000000000, 0.9898214418809326842, 1.000000000000000000, 0.9898214418809326842, 1.000000000000000000, 0.9898214418809326842, 1.000000000000000000, 0.9898214418809326842, 1.000000000000000000, 0.9898214418809326842, 1.000000000000000000, 0.9898214418809326842, 1.000000000000000000, 0.9898214418809326842, 1.000000000000000000, 0.9898214418809326842, 1.000000000000000000, 0.9898214418809326842, 1.000000000000000000, 0.9898214418809326842, 1.000000000000000000, 0.9898214418809326842, 1.000000000000000000, 0.9898214418809326842, 1.000000000000000000, 0.9898214418809326842, 1.000000000000000000, 0.9898214418809326842, 1.000000000000000000, 0.9898214418809326842, 1.000000000000000000, 0.9898214418809326842, 1.000000000000000000, 0.9898214418809326842, 1.000000000000000000, 0.9898214418809326842, 1.000000000000000000, 0.9898214418809326842, 1.000000000000000000, 0.9898214418809326842, 1.000000000000000000, 0.9898214418809326842, 1.000000000000000000, 0.9898214418809326842, 1.000000000000000000, 0.9898214418809326842, 1.000000000000000000, 0.9898214418809326842, 1.000000000000000000, 0.9898214418809326842, 1.000000000000000000, 0.9898214418809326842, 1.000000000000000000, 0.9898214418809326842, 1.000000000000000000, 0.9898214418809326842, 1.000000000000000000, 0.9898214418809326842, 1.000000000000000000, 0.9898214418809326842, 1.000000000000000000, 0.9898214418809326842, 1.000000000000000000, 0.9898214418809326842, 1.000000000000000000, 0.9898214418809326842, 1.000000000000000000, 0.9898214418809326842, 1.000000000000000000, 0.9898214418809326842, 1.000000000000000000, 0.9898214418809326842, 1.000000000000000000, 0.9898214418809326842, 1.000000000000000000, 0.9898214418809326842, 1.000000000000000000, 0.9898214418809326842, 1.000000000000000000, 0.9898214418809326842, 1.000000000000000000, 0.9898214418809326842, 1.000000000000000000, 0.9898214418809326842, 1.000000000000000000, 0.9898214418809326842, 1.000000000000000000, 0.9898214418809326842, 1.000000000000000000, 0.9898214418809326842, 1.000000000000000000, 0.9898214418809326842, 1.000000000000000000, 0.9898214418809326842, 1.000000000000000000, 0.9898214418809326842, 1.000000000000000000, 0.9898214418809326842, 1.000000000000000000, 0.9898214418809326842, 1.000000000000000000, 0.9898214418809326842, 1.000000000000000000, 0.9898214418809326842, 1.000000000000000000, 0.9898214418809326842, 1.000000000000000000, 0.9898214418809326842, 1.000000000000000000, 0.9898214418809326842, 1.000000000000000000, 0.9898214418809326842, 1.000000000000000000, 0.9898214418809326842, 1.000000000000000000, 0.9898214418809326842, 1.000000000000000000, 0.9898214418809326842, 1.000000000000000000, 0.9898214418809326842, 1.000000000000000000, 0.9898214418809326842, 1.000000000000000000, 0.9898214418809326842, 1.000000000000000000, 0.9898214418809326842, 1.000000000000000000, 0.9898214418809326842, 1.000000000000000000, 0.9898214418809326842, 1.000000000000000000, 0.9898214418809326842, 1.000000000000000000, 0.9898214418809326842, 1.000000000000000000, 0.9898214418809326842, 1.000000000000000000, 0.9898214418809326842, 1.000000000000000000, 0.9898214418809326842, 1.000000000000000000, 0.9898214418809326842, 1.000000000000000000, 0.9898214418809326842, 1.000000000000000000, 0.9898214418809326842, 1.000000000000000000, 0.9898214418809326842, 1.000000000000000000, 0.9898214418809326842, 1.000000000000000000, 0.9898214418809326842, 1.000000000000000000, 0.9898214418809326842, 1.000000000000000000, 0.9898214418809326842, 1.000000000000000000, 0.9898214418809326842, 1.000000000000000000, 0.9898214418809326842, 1.000000000000000000, 0.9898214418809326842, 1.000000000000000000, 0.9898214418809326842, 1.000000000000000000, 0.9898214418809326842, 1.000000000000000000, 0.9898214418809326842, 1.000000000000000000, 0.9898214418809326842, 1.000000000000000000, 0.9898214418809326842, 1.000000000000000000, 0.9898214418809326842, 1.000000000000000000, 0.9898214418809326842, 1.000000000000000000, 0.9898214418809326842, 1.000000000000000000, 0.9898214418809326842, 1.000000000000000000, 0.9898214418809326842, 1.000000000000000000, 0.9898214418809326842, 1.000000000000000000, 0.9898214418809326842, 1.000000000000000000, 0.9898214418809326842, 1.000000000000000000, 0.9898214418809326842, 1.000000000000000000, 0.9898214418809326842, 1.000000000000000000, 0.9898214418809326842, 1.000000000000000000, 0.9898214418809326842, 1.000000000000000000, 0.9898214418809326842, 1.000000000000000000, 0.9898214418809326842, 1.000000000000000000, 0.9898214418809326842, 1.000000000000000000, 0.9898214418809326842, 1.000000000000000000, 0.9898214418809326842, 1.000000000000000000, 0.9898214418809326842, 1.000000000000000000, 0.9898214418809326842, 1.000000000000000000, 0.9898214418809326842, 1.000000000000000000, 0.9898214418809326842, 1.000000000000000000, 0.9898214418809326842, 1.000000000000000000, 0.9898214418809326842, 1.000000000000000000, 0.9898214418809326842, 1.000000000000000000, 0.9898214418809326842, 1.000000000000000000, 0.9898214418809326842, 1.000000000000000000, 0.9898214418809326842, 1.000000000000000000, 0.9898214418809326842, 1.000000000000000000, 0.9898214418809326842, 1.000000000000000000, 0.9898214418809326842, 1.000000000000000000, 0.9898214418809326842, 1.000000000000000000, 0.9898214418809326842, 1.000000000000000000, 0.9898214418809326842, 1.000000000000000000, 0.9898214418809326842, 1.000000000000000000, 0.9898214418809326842, 1.000000000000000000, 0.9898214418809326842, 1.000000000000000000, 0.9898214418809326842, 1.000000000000000000, 0.9898214418809326842, 1.000000000000000000, 0.9898214418809326842, 1.000000000000000000, 0.9898214418809326842, 1.000000000000000000, 0.9898214418809326842, 1.000000000000000000, 0.9898214418809326842, 1.000000000000000000, 0.9898214418809326842, 1.000000000000000000, 0.9898214418809326842, 1.000000000000000000, 0.9898214418809326842, 1.000000000000000000, 0.9898214418809326842, 1.000000000000000000, 0.9898214418809326842, 1.000000000000000000, 0.9898214418809326842, 1.000000000000000000, 0.9898214418809326842, 1.000000000000000000, 0.9898214418809326842, 1.000000000000000000, 0.9898214418809326842, 1.000000000000000000, 0.9898214418809326842, 1.000000000000000000, 0.9898214418809326842, 1.000000000000000000, 0.9898214418809326842, 1.000000000000000000, 0.9898214418809326842, 1.000000000000000000, 0.9898214418809326842, 1.000000000000000000, 0.9898214418809326842, 1.000000000000000000, 0.9898214418809326842, 1.000000000000000000, 0.9898214418809326842, 1.000000000000000000, 0.9898214418809326842, 1.000000000000000000, 0.9898214418809326842, 1.000000000000000000, 0.9898214418809326842, 1.000000000000000000, 0.9898214418809326842, 1.000000000000000000, 0.9898214418809326842, 1.000000000000000000, 0.9898214418809326842, 1.000000000000000000, 0.9898214418809326842, 1.000000000000000000, 0.9898214418809326842, 1.000000000000000000, 0.9898214418809326842, 1.000000000000000000, 0.9898214418809326842, 1.000000000000000000, 0.9898214418809326842, 1.000000000000000000, 0.9898214418809326842, 1.000000000000000000, 0.9898214418809326842, 1.000000000000000000, 0.9898214418809326842, 1.000000000000000000, 0.9898214418809326842, 1.000000000000000000, 0.9898214418809326842, 1.000000000000000000, 0.9898214418809326842, 1.000000000000000000, 0.9898214418809326842, 1.000000000000000000, 0.9898214418809326842, 1.000000000000000000, 0.9898214418809326842, 1.000000000000000000, 0.9898214418809326842, 1.000000000000000000, 0.9898214418809326842, 1.000000000000000000, 0.9898214418809326842, 1.000000000000000000, 0.9898214418809326842, 1.000000000000000000, 0.9898214418809326842, 1.000000000000000000, 0.9898214418809326842, 1.000000000000000000, 0.9898214418809326842, 1.000000000000000000, 0.9898214418809326842, 1.000000000000000000, 0.9898214418809326842, 1.000000000000000000, 0.9898214418809326842, 1.000000000000000000, 0.9898214418809326842, 1.000000000000000000, 0.9898214418809326842, 1.000000000000000000, 0.9898214418809326842, 1.000000000000000000, 0.9898214418809326842, 1.000000000000000000, 0.9898214418809326842, 1.000000000000000000, 0.9898214418809326842, 1.000000000000000000, 0.9898214418809326842, 1.000000000000000000, 0.9898214418809326842, 1.000000000000000000, 0.9898214418809326842, 1.000000000000000000, 0.9898214418809326842, 1.000000000000000000, 0.9898214418809326842, 1.000000000000000000, 0.9898214418809326842, 1.000000000000000000, 0.9898214418809326842, 1.000000000000000000, 0.9898214418809326842, 1.000000000000000000, 0.9898214418809326842, 1.000000000000000000, 0.9898214418809326842, 1.000000000000000000, 0.9898214418809326842, 1.000000000000000000, 0.9898214418809326842, 1.000000000000000000, 0.9898214418809326842, 1.000000000000000000, 0.9898214418809326842, 1.000000000000000000, 0.9898214418809326842, 1.000000000000000000, 0.9898214418809326842, 1.000000000000000000, 0.9898214418809326842, 1.000000000000000000, 0.9898214418809326842, 1.000000000000000000, 0.9898214418809326842, 1.000000000000000000, 0.9898214418809326842, 1.000000000000000000, 0.9898214418809326842, 1.000000000000000000, 0.9898214418809326842, 1.000000000000000000, 0.9898214418809326842, 1.000000000000000000, 0.9898214418809326842, 1.000000000000000000, 0.9898214418809326842, 1.000000000000000000, 0.9898214418809326842, 1.000000000000000000, 0.9898214418809326842, 1.000000000000000000, 0.9898214418809326842, 1.000000000000000000, 0.9898214418809326842, 1.000000000000000000, 0.9898214418809326842, 1.000000000000000000, 0.9961809353924466759, 0.9952277490961531914) ) ) 
 REPRESENTATION_ITEM ( '' )  SURFACE ( )  );
#36829=CARTESIAN_POINT ( 'NONE',  ( 762.3223304703356007, 16.45630643248849267, -322.3223304703362828 ) ) ;
#36832=CARTESIAN_POINT ( 'NONE',  ( 802.9823548866075953, -433.0999726633339151, -330.0799878456151077 ) ) ;
#36834=CARTESIAN_POINT ( 'NONE',  ( 805.6418435158337843, -197.4636090269709996, -363.8556311672236916 ) ) ;
#36837=CARTESIAN_POINT ( 'NONE',  ( 803.6646147819161570, -185.9073299311472454, -348.8264449731210561 ) ) ;
#36839=CARTESIAN_POINT ( 'NONE',  ( 790.8726784830453198, -346.7146871989592682, -362.5472867521010585 ) ) ;
#36840=CARTESIAN_POINT ( 'NONE',  ( 799.9999999999993179, -462.9681489794448339, -309.9999999999998863 ) ) ;
#36842=CARTESIAN_POINT ( 'NONE',  ( 781.2370466360911223, -212.7363362996982232, -304.9990715423533629 ) ) ;
#36845=CARTESIAN_POINT ( 'NONE',  ( 783.0745993439762742, -56.19088175424417386, -365.1016975059196739 ) ) ;
#36848=CARTESIAN_POINT ( 'NONE',  ( 814.5518280994195948, -231.7255117493288594, -332.4837098697145166 ) ) ;
#36849=CARTESIAN_POINT ( 'NONE',  ( 779.9999999999997726, 16.45630643248849267, -339.9999999999994884 ) ) ;
#36850=CARTESIAN_POINT ( 'NONE',  ( 755.5713283507202505, -29.36187538569318178, -334.6858677611754729 ) ) ;
#36853=CARTESIAN_POINT ( 'NONE',  ( 798.0661480581538854, -146.5328690171417350, -309.5768839229118043 ) ) ;
#36855=CARTESIAN_POINT ( 'NONE',  ( 745.7998596910086917, -389.3618753856919739, -332.5602148656461168 ) ) ;
#36860=CARTESIAN_POINT ( 'NONE',  ( 804.6798772138708955, -375.7255117493283478, -334.6312213355107019 ) ) ;
#36862=CARTESIAN_POINT ( 'NONE',  ( 814.2001403089898304, -449.3618753856918602, -347.4397851343538264 ) ) ;
#36867=CARTESIAN_POINT ( 'NONE',  ( 754.9735926884551418, -210.3510508353233490, -340.5236548041000333 ) ) ;
#36869=CARTESIAN_POINT ( 'NONE',  ( 801.9858362298568863, -219.0783235625960401, -312.7379699480935642 ) ) ;
#36875=CARTESIAN_POINT ( 'NONE',  ( 774.6858677611749044, -153.7255117493291721, -315.5713283507209894 ) ) ;
#36877=CARTESIAN_POINT ( 'NONE',  ( 796.9462024416508257, -84.45278447660206211, -308.9653473494370246 ) ) ;
#36878=CARTESIAN_POINT ( 'NONE',  ( 794.9819416627830151, -60.99823902205671544, -319.9864689768909898 ) ) ;
#36880=CARTESIAN_POINT ( 'NONE',  ( 773.4516893846965786, 4.354572791210176597, -315.8398074228977066 ) ) ;
#36882=CARTESIAN_POINT ( 'NONE',  ( 775.8780910478218402, -321.2817908451525000, -364.9511171171680530 ) ) ;
#36889=CARTESIAN_POINT ( 'NONE',  ( 766.0291762391763086, -322.9181544815161260, -360.7704444035551319 ) ) ;
#36890=CARTESIAN_POINT ( 'NONE',  ( 800.2193346964447755, -138.9982390220563957, -355.1360043628815788 ) ) ;
#36893=CARTESIAN_POINT ( 'NONE',  ( 772.4999999999993179, -512.9681489794448908, -309.9999999999998863 ) ) ;
#36900=CARTESIAN_POINT ( 'NONE',  ( 792.2312462859673587, -131.9073299311473875, -307.2067596250082602 ) ) ;
#36903=CARTESIAN_POINT ( 'NONE',  ( 754.9967657858570647, -265.5436935675106156, -365.0032342141425374 ) ) ;
#36906=CARTESIAN_POINT ( 'NONE',  ( 751.2241431872005251, -352.1692326535046504, -359.9636004259367610 ) ) ;
#36907=CARTESIAN_POINT ( 'NONE',  ( 772.5602148656447525, -81.72551174932937101, -305.7998596910095443 ) ) ;
#36909=CARTESIAN_POINT ( 'NONE',  ( 782.4968714119720516, -346.8164208402376971, -305.0891759886411023 ) ) ;
#36914=CARTESIAN_POINT ( 'NONE',  ( 785.3141322388236176, -213.7255117493289731, -364.4286716492789537 ) ) ;
#36915=CARTESIAN_POINT ( 'NONE',  ( 810.1134526219336749, -128.5328690171417634, -357.8822607201570349 ) ) ;
#36921=CARTESIAN_POINT ( 'NONE',  ( 803.2186876482843445, -223.9874144716869182, -350.0220218866286928 ) ) ;
#36923=CARTESIAN_POINT ( 'NONE',  ( 755.2512626584698410, 16.45630643248849267, -315.2512626584710915 ) ) ;
#36924=CARTESIAN_POINT ( 'NONE',  ( 746.7653713866222915, -65.26014174441471027, -351.0478386215610271 ) ) ;
#36928=CARTESIAN_POINT ( 'NONE',  ( 744.6391490659812007, -374.7363362996978253, -338.7502325331110455 ) ) ;
#36929=CARTESIAN_POINT ( 'NONE',  ( 800.2193346964447755, -234.9982390220561683, -355.1360043628815788 ) ) ;
#36932=CARTESIAN_POINT ( 'NONE',  ( 780.5236548040995785, -236.7363362996981380, -314.9735926884559944 ) ) ;
#36933=CARTESIAN_POINT ( 'NONE',  ( 791.9812246680005501, -212.6346026584198796, -361.9419747391813189 ) ) ;
#36934=CARTESIAN_POINT ( 'NONE',  ( 771.2633955100217236, -383.9073299311466485, -363.4237431249939618 ) ) ;
#36937=CARTESIAN_POINT ( 'NONE',  ( 762.3223304703356007, -103.5436935675111272, -322.3223304703362828 ) ) ;
#36941=CARTESIAN_POINT ( 'NONE',  ( 759.9999999999992042, 205.0000000000000568, -319.9999999999999432 ) ) ;
#36946=CARTESIAN_POINT ( 'NONE',  ( 760.0363995740630116, -442.9181544815157849, -368.7758568127991907 ) ) ;
#36947=CARTESIAN_POINT ( 'NONE',  ( 813.1304606946831655, -17.90732993114776406, -352.3570229623691716 ) ) ;
#36949=CARTESIAN_POINT ( 'NONE',  ( 767.8955696845333705, -384.4527844766011526, -362.1676090361162323 ) ) ;
#36950=CARTESIAN_POINT ( 'NONE',  ( 803.6646147819162707, -17.90732993114776406, -348.8264449731211130 ) ) ;
#36953=CARTESIAN_POINT ( 'NONE',  ( 787.5531968255692163, -285.8272453906071178, -316.1348686366205811 ) ) ;
#36954=CARTESIAN_POINT ( 'NONE',  ( 754.9967657858570647, -169.5436935675108430, -365.0032342141425374 ) ) ;
#36957=CARTESIAN_POINT ( 'NONE',  ( 788.0874520139973356, 16.45630643248838609, -314.0623709945898554 ) ) ;
#36961=CARTESIAN_POINT ( 'NONE',  ( 800.2193346964447755, -330.9982390220558273, -355.1360043628815788 ) ) ;
#36963=CARTESIAN_POINT ( 'NONE',  ( 750.9282345327678740, -88.91815448151682233, -319.8311093483690115 ) ) ;
#36964=CARTESIAN_POINT ( 'NONE',  ( 766.7756240680305382, -134.5328690171417350, -361.5560724626415663 ) ) ;
#36968=CARTESIAN_POINT ( 'NONE',  ( 794.9819416627830151, -12.99823902205686821, -319.9864689768909898 ) ) ;
#36969=CARTESIAN_POINT ( 'NONE',  ( 765.8855110935204493, -118.1692326535054463, -319.0159684113471599 ) ) ;
#36970=CARTESIAN_POINT ( 'NONE',  ( 795.1360043628807261, -116.0891481129656029, -360.2193346964456282 ) ) ;
#36972=CARTESIAN_POINT ( 'NONE',  ( 784.0799538623451781, -419.8055962898681059, -364.6971507214555572 ) ) ;
#36978=CARTESIAN_POINT ( 'NONE',  ( 804.1009440267234822, -263.4636090269708006, -314.0944755984392600 ) ) ;
#36985=CARTESIAN_POINT ( 'NONE',  ( 766.9102291470427417, -114.5545181178803631, -318.6633372737382501 ) ) ;
#36986=CARTESIAN_POINT ( 'NONE',  ( 794.9819416627830151, -276.9982390220559978, -319.9864689768909898 ) ) ;
#36988=CARTESIAN_POINT ( 'NONE',  ( 754.8072714833581358, -436.8164208402372992, -338.1981804954720587 ) ) ;
#36989=CARTESIAN_POINT ( 'NONE',  ( 771.1735550268778070, -81.18005720387481006, -316.3353852180827630 ) ) ;
#36995=CARTESIAN_POINT ( 'NONE',  ( 810.4231160770870019, -336.5545181178796952, -321.9338519418446936 ) ) ;
#36998=CARTESIAN_POINT ( 'NONE',  ( 759.9864689768902508, -290.0891481129650629, -354.9819416627836404 ) ) ;
#37000=CARTESIAN_POINT ( 'NONE',  ( 759.0159684113467620, -160.9181544815165807, -325.8855110935213020 ) ) ;
#37004=CARTESIAN_POINT ( 'NONE',  ( 763.2262854647970016, -368.6346026584193964, -309.2812353651462445 ) ) ;
#37009=CARTESIAN_POINT ( 'NONE',  ( 767.7687537140311633, 0.09267006885218045942, -372.7932403749916830 ) ) ;
#37012=EDGE_CURVE ( 'NONE', #29607, #29231, #14686, .T. ) ;
#37015=CARTESIAN_POINT ( 'NONE',  ( 775.9200461376533440, 0.1944037101305369775, -315.3028492785443291 ) ) ;
#37021=CARTESIAN_POINT ( 'NONE',  ( 795.9930595647434757, -315.0783235625957559, -320.7433823573372820 ) ) ;
#37025=CARTESIAN_POINT ( 'NONE',  ( 808.7758568127978833, -340.1692326535047641, -320.0363995740631822 ) ) ;
#37032=CARTESIAN_POINT ( 'NONE',  ( 796.7737145352015204, -188.6346026584199365, -370.7187646348536987 ) ) ;
#37036=CARTESIAN_POINT ( 'NONE',  ( 778.1981804954715471, -178.2709662947835909, -314.8072714833591021 ) ) ;
#37037=ORIENTED_EDGE ( 'NONE', *, *, #4371, .F. ) ;
#37038=CARTESIAN_POINT ( 'NONE',  ( 804.4286716492782716, 6.638124614306706306, -345.3141322388244703 ) ) ;
#37045=CARTESIAN_POINT ( 'NONE',  ( 780.5236548040995785, -428.7363362996975980, -314.9735926884559944 ) ) ;
#37047=CARTESIAN_POINT ( 'NONE',  ( 783.7953271457878373, -200.1908817542436907, -375.1787889125761239 ) ) ;
#37050=CARTESIAN_POINT ( 'NONE',  ( 805.1927285166397041, -184.8164208402380950, -341.8018195045277707 ) ) ;
#37051=CARTESIAN_POINT ( 'NONE',  ( 769.1273215169530886, -358.7146871989592114, -317.4527132478988847 ) ) ;
#37052=CARTESIAN_POINT ( 'NONE',  ( 767.9999999999992042, 205.0000000000000568, -339.9999999999999432 ) ) ;
#37053=CARTESIAN_POINT ( 'NONE',  ( 771.3260364891663130, -211.6454272087891582, -306.0683387631859773 ) ) ;
#37056=CARTESIAN_POINT ( 'NONE',  ( 755.5913626894240451, -61.64542720878961291, -346.6156483768012890 ) ) ;
#37059=CARTESIAN_POINT ( 'NONE',  ( 812.7932403749906598, -231.1800572038743553, -327.7687537140311633 ) ) ;
#37063=CARTESIAN_POINT ( 'NONE',  ( 774.6312213355099630, -47.36187538569312494, -364.6798772138717482 ) ) ;
#37066=CARTESIAN_POINT ( 'NONE',  ( 811.6461892240364477, -124.7146871989599930, -324.1737431748509835 ) ) ;
#37068=CARTESIAN_POINT ( 'NONE',  ( 755.2512626584698410, -367.5436935675102745, -315.2512626584710915 ) ) ;
#37073=CARTESIAN_POINT ( 'NONE',  ( 788.8264449731200330, -405.1800572038737300, -363.6646147819171233 ) ) ;
#37074=DIRECTION ( 'NONE',  ( -1.000000000000000000, -0.000000000000000000, -0.000000000000000000 ) ) ;
#37075=CARTESIAN_POINT ( 'NONE',  ( 812.7932403749906598, -447.1800572038736732, -327.7687537140311633 ) ) ;
#37079=CARTESIAN_POINT ( 'NONE',  ( 798.7617431975189675, -219.6237781080506295, -323.0428371773161871 ) ) ;
#37081=CARTESIAN_POINT ( 'NONE',  ( 793.4146539503750546, -217.9874144716870035, -307.6481478633938877 ) ) ;
#37085=CARTESIAN_POINT ( 'NONE',  ( 800.0135310231082713, -182.0891481129654323, -325.0180583372163028 ) ) ;
#37088=CARTESIAN_POINT ( 'NONE',  ( 744.7301800767019131, -76.81642084023845030, -337.4774526936615757 ) ) ;
#37090=CARTESIAN_POINT ( 'NONE',  ( 805.1927285166399315, -88.81642084023843609, -341.8018195045277707 ) ) ;
#37092=CARTESIAN_POINT ( 'NONE',  ( 758.4439275373578084, -12.55451811788067751, -353.2243759319684386 ) ) ;
#37094=CARTESIAN_POINT ( 'NONE',  ( 799.2566176426618085, -336.0090635724251911, -324.0069404352559559 ) ) ;
#37101=CARTESIAN_POINT ( 'NONE',  ( 757.4527132478984868, -328.3726999360615650, -329.1273215169538844 ) ) ;
#37102=CARTESIAN_POINT ( 'NONE',  ( 771.2633955100217236, -335.9073299311468190, -363.4237431249939618 ) ) ;
#37103=CARTESIAN_POINT ( 'NONE',  ( 802.1676090361156639, -158.6346026584199933, -327.8955696845344505 ) ) ;
#37107=CARTESIAN_POINT ( 'NONE',  ( 783.0433043558608688, -264.8965053807776826, -315.1538015810313027 ) ) ;
#37108=CARTESIAN_POINT ( 'NONE',  ( 745.1792804349281596, -134.1908817542439181, -343.7566961878542884 ) ) ;
#37113=CARTESIAN_POINT ( 'NONE',  ( 767.6429770376291799, -153.1800572038746111, -306.8695393053162093 ) ) ;
#37118=CARTESIAN_POINT ( 'NONE',  ( 812.7932403749906598, -279.1800572038741848, -327.7687537140311633 ) ) ;
#37123=CARTESIAN_POINT ( 'NONE',  ( 747.3154664389472828, -331.9874144716865203, -326.4474001241230781 ) ) ;
#37125=CARTESIAN_POINT ( 'NONE',  ( 808.3070685750230950, -90.99823902205663728, -361.1904061080339261 ) ) ;
#37127=CARTESIAN_POINT ( 'NONE',  ( 751.6929314249748586, -366.9982390220556567, -318.8095938919659034 ) ) ;
#37132=CARTESIAN_POINT ( 'NONE',  ( 761.9338519418445230, -110.5328690171418629, -370.4231160770881957 ) ) ;
#37139=CARTESIAN_POINT ( 'NONE',  ( 756.1348686366196716, 6.739858255585061464, -347.5531968255698416 ) ) ;
#37142=CARTESIAN_POINT ( 'NONE',  ( 759.8311093483677041, -430.1692326535043094, -310.9282345327691814 ) ) ;
#37146=CARTESIAN_POINT ( 'NONE',  ( 764.1737431748507561, -394.3726999360613377, -371.6461892240376415 ) ) ;
#37147=CARTESIAN_POINT ( 'NONE',  ( 756.5762568750052424, -243.1800572038743269, -348.7366044899774238 ) ) ;
#37150=CARTESIAN_POINT ( 'NONE',  ( 805.2837595273609850, -218.7363362996982232, -340.5290396650784714 ) ) ;
#37151=CARTESIAN_POINT ( 'NONE',  ( 804.6798772138708955, -207.7255117493289447, -334.6312213355107019 ) ) ;
#37153=CARTESIAN_POINT ( 'NONE',  ( 781.8018195045267476, -406.2709662947828519, -365.1927285166407273 ) ) ;
#37157=CARTESIAN_POINT ( 'NONE',  ( 778.1981804954714335, -106.2709662947838467, -314.8072714833589885 ) ) ;
#37158=EDGE_LOOP ( 'NONE', ( #40634, #43085, #36822, #21087, #986, #22154, #28608, #8084 ) ) ;
#37166=CARTESIAN_POINT ( 'NONE',  ( 764.1737431748507561, -442.3726999360611103, -371.6461892240376415 ) ) ;
#37167=CARTESIAN_POINT ( 'NONE',  ( 744.7301800767020268, -28.81642084023863504, -337.4774526936615189 ) ) ;
#37169=CARTESIAN_POINT ( 'NONE',  ( 792.1044303154645831, -396.4527844766010389, -317.8323909638837677 ) ) ;
#37170=CARTESIAN_POINT ( 'NONE',  ( 762.1405469898973024, -1.543693567511449594, -357.8594530101016176 ) ) ;
#37174=CARTESIAN_POINT ( 'NONE',  ( 760.7433823573367135, -300.0090635724252479, -355.9930595647440441 ) ) ;
#37175=CARTESIAN_POINT ( 'NONE',  ( 749.2812353651451076, -150.4527844766018916, -323.2262854647983090 ) ) ;
#37178=CARTESIAN_POINT ( 'NONE',  ( 795.0120564873543572, 16.45630643248849267, -314.4408280072604498 ) ) ;
#37182=CARTESIAN_POINT ( 'NONE',  ( 755.5713283507202505, -365.3618753856920875, -334.6858677611754729 ) ) ;
#37186=CARTESIAN_POINT ( 'NONE',  ( 768.9521613784389729, -105.8272453906076578, -373.2346286133773106 ) ) ;
#37187=CARTESIAN_POINT ( 'NONE',  ( 803.2186876482843445, -151.9874144716871740, -350.0220218866286928 ) ) ;
#37190=CARTESIAN_POINT ( 'NONE',  ( 801.9419747391806368, -42.45278447660223264, -351.9812246680014027 ) ) ;
#37191=CARTESIAN_POINT ( 'NONE',  ( 764.0069404352550464, -183.0783235625961538, -359.2566176426627180 ) ) ;
#37192=CARTESIAN_POINT ( 'NONE',  ( 795.1360043628807261, -140.0891481129654892, -360.2193346964456282 ) ) ;
#37194=CARTESIAN_POINT ( 'NONE',  ( 787.6308680596127942, -419.2601417444136587, -364.1105419155492768 ) ) ;
#37200=CARTESIAN_POINT ( 'NONE',  ( 778.7629533639073998, -272.7363362996981095, -375.0009284576466371 ) ) ;
#37209=CARTESIAN_POINT ( 'NONE',  ( 758.4439275373578084, -108.5545181178803915, -353.2243759319684386 ) ) ;
#37210=CARTESIAN_POINT ( 'NONE',  ( 755.5713283507202505, -101.3618753856929544, -334.6858677611754729 ) ) ;
#37211=CARTESIAN_POINT ( 'NONE',  ( 788.7366044899766848, -275.9073299311469896, -316.5762568750059813 ) ) ;
#37213=CARTESIAN_POINT ( 'NONE',  ( 771.2633955100217236, -431.9073299311464211, -363.4237431249939618 ) ) ;
#37214=CARTESIAN_POINT ( 'NONE',  ( 755.5713283507202505, -77.36187538569302546, -334.6858677611754729 ) ) ;
#37221=CARTESIAN_POINT ( 'NONE',  ( 786.2694204179717872, -333.2817908451523863, -305.1769319972829067 ) ) ;
#37225=CARTESIAN_POINT ( 'NONE',  ( 800.2193346964447755, -282.9982390220558841, -355.1360043628815788 ) ) ;
#37227=CARTESIAN_POINT ( 'NONE',  ( 760.7433823573367135, -204.0090635724255606, -355.9930595647440441 ) ) ;
#37230=CARTESIAN_POINT ( 'NONE',  ( 787.5162901302840055, -395.3618753856919739, -305.4481719005793252 ) ) ;
#37236=CARTESIAN_POINT ( 'NONE',  ( 796.9462024416508257, -12.45278447660232146, -308.9653473494370246 ) ) ;
#37237=CARTESIAN_POINT ( 'NONE',  ( 778.1981804954714335, -250.2709662947832783, -314.8072714833589885 ) ) ;
#37243=CARTESIAN_POINT ( 'NONE',  ( 799.4546378042377910, -9.078323562596708030, -356.1575198192848006 ) ) ;
#37248=ORIENTED_EDGE ( 'NONE', *, *, #37727, .F. ) ;
#37249=CARTESIAN_POINT ( 'NONE',  ( 788.8264449731200330, -45.18005720387493085, -363.6646147819171233 ) ) ;
#37251=CARTESIAN_POINT ( 'NONE',  ( 783.0433043558608688, -336.8965053807774552, -315.1538015810313027 ) ) ;
#37256=CARTESIAN_POINT ( 'NONE',  ( 744.9990715423526808, -378.3510508353227806, -341.2370466360926002 ) ) ;
#37263=CARTESIAN_POINT ( 'NONE',  ( 782.4968714119720516, -178.8164208402381519, -305.0891759886411023 ) ) ;
#37267=CARTESIAN_POINT ( 'NONE',  ( 791.9812246680005501, -164.6346026584200217, -361.9419747391813189 ) ) ;
#37269=CARTESIAN_POINT ( 'NONE',  ( 804.6798772138708955, -327.7255117493285184, -334.6312213355107019 ) ) ;
#37270=CARTESIAN_POINT ( 'NONE',  ( 791.9460785601769430, -462.7578698805381237, -362.0383033825738721 ) ) ;
#37279=CARTESIAN_POINT ( 'NONE',  ( 793.0897708529556667, -438.5545181178793541, -361.3366627262616362 ) ) ;
#37282=CARTESIAN_POINT ( 'NONE',  ( 814.4686193811664907, -243.2817908451526705, -346.2056067578752732 ) ) ;
#37285=CARTESIAN_POINT ( 'NONE',  ( 758.0580252608178853, -174.4527844766018063, -328.0187753319985404 ) ) ;
#37286=CARTESIAN_POINT ( 'NONE',  ( 776.9566956441375396, -348.8965053807774552, -364.8461984189686405 ) ) ;
#37288=CARTESIAN_POINT ( 'NONE',  ( 750.9282345327678740, -232.9181544815163249, -319.8311093483690115 ) ) ;
#37291=CARTESIAN_POINT ( 'NONE',  ( 783.0745993439762742, -80.19088175424411702, -365.1016975059196739 ) ) ;
#37295=CARTESIAN_POINT ( 'NONE',  ( 792.2312462859673587, -275.9073299311469896, -307.2067596250082602 ) ) ;
#37298=CARTESIAN_POINT ( 'NONE',  ( 764.8639956371174549, -56.08914811296580893, -319.7806653035542013 ) ) ;
#37299=AXIS2_PLACEMENT_3D ( 'NONE', #4516, #818, #8210 ) ;
#37301=CARTESIAN_POINT ( 'NONE',  ( 788.7631598425961101, -145.4419599262326699, -305.7194118038759143 ) ) ;
#37303=CARTESIAN_POINT ( 'NONE',  ( 787.5162901302840055, -395.3618753856918602, -305.4481719005792684 ) ) ;
#37307=CARTESIAN_POINT ( 'NONE',  ( 774.6312213355099630, -383.3618753856921444, -364.6798772138717482 ) ) ;
#37309=CARTESIAN_POINT ( 'NONE',  ( 781.2370466360911223, -44.73633629969875614, -304.9990715423533629 ) ) ;
#37315=EDGE_CURVE ( 'NONE', #14073, #43845, #41286, .T. ) ;
#37317=CARTESIAN_POINT ( 'NONE',  ( 776.9566956441375396, -228.8965053807778816, -364.8461984189686405 ) ) ;
#37318=CARTESIAN_POINT ( 'NONE',  ( 767.8955696845333705, -120.4527844766019484, -362.1676090361162323 ) ) ;
#37320=CARTESIAN_POINT ( 'NONE',  ( 756.1443688327750579, -237.6237781080505442, -314.3581564841659315 ) ) ;
#37323=VERTEX_POINT ( 'NONE', #7436 ) ;
#37325=CARTESIAN_POINT ( 'NONE',  ( 795.1360043628807261, -164.0891481129655176, -360.2193346964456282 ) ) ;
#37327=CARTESIAN_POINT ( 'NONE',  ( 800.9747183278959710, -60.99823902205671544, -311.9810565676471583 ) ) ;
#37328=CARTESIAN_POINT ( 'NONE',  ( 785.3687786644885591, -83.36187538569299704, -315.3201227861280813 ) ) ;
#37330=CARTESIAN_POINT ( 'NONE',  ( 780.5236548040995785, -20.73633629969883430, -314.9735926884559944 ) ) ;
#37333=CARTESIAN_POINT ( 'NONE',  ( 799.2566176426618085, -360.0090635724250774, -324.0069404352559559 ) ) ;
#37341=CARTESIAN_POINT ( 'NONE',  ( 787.5531968255692163, -309.8272453906070041, -316.1348686366205811 ) ) ;
#37342=CARTESIAN_POINT ( 'NONE',  ( 755.3201227861273992, -315.7255117493286320, -345.3687786644892981 ) ) ;
#37343=CARTESIAN_POINT ( 'NONE',  ( 814.8207195650702488, -146.1908817542438896, -336.2433038121456548 ) ) ;
#37347=CARTESIAN_POINT ( 'NONE',  ( 759.9999999999992042, -462.9681489794448339, -309.9999999999998863 ) ) ;
#37348=CARTESIAN_POINT ( 'NONE',  ( 786.2694204179717872, -117.2817908451530684, -305.1769319972829067 ) ) ;
#37349=DIRECTION ( 'NONE',  ( 0.000000000000000000, -1.000000000000000000, 0.000000000000000000 ) ) ;
#37355=CARTESIAN_POINT ( 'NONE',  ( 754.9967657858570647, -169.5436935675108998, -365.0032342141425943 ) ) ;
#37358=CARTESIAN_POINT ( 'NONE',  ( 745.7998596910086917, -293.3618753856923718, -332.5602148656461168 ) ) ;
#37360=CARTESIAN_POINT ( 'NONE',  ( 772.5602148656447525, -441.7255117493282910, -305.7998596910095443 ) ) ;
#37364=CARTESIAN_POINT ( 'NONE',  ( 801.9858362298568863, -339.0783235625956422, -312.7379699480935642 ) ) ;
#37365=CARTESIAN_POINT ( 'NONE',  ( 745.4481719005789273, -99.72551174932928575, -347.5162901302853129 ) ) ;
#37367=CARTESIAN_POINT ( 'NONE',  ( 801.1904061080336987, -380.0891481129646650, -368.3070685750235498 ) ) ;
#37375=CARTESIAN_POINT ( 'NONE',  ( 791.1614460488616487, -107.2601417444145824, -373.5763878283158874 ) ) ;
#37383=CARTESIAN_POINT ( 'NONE',  ( 812.6845335610512393, -439.9874144716862929, -353.5525998758768651 ) ) ;
#37386=ORIENTED_EDGE ( 'NONE', *, *, #7500, .F. ) ;
#37388=CARTESIAN_POINT ( 'NONE',  ( 793.5525998758768083, -367.0999726633342561, -372.6845335610516941 ) ) ;
#37390=CARTESIAN_POINT ( 'NONE',  ( 781.8018195045266339, -238.2709662947833920, -365.1927285166406705 ) ) ;
#37393=EDGE_CURVE ( 'NONE', #14073, #30422, #39781, .T. ) ;
#37394=CARTESIAN_POINT ( 'NONE',  ( 802.5472867521000353, -220.3726999360618208, -350.8726784830461156 ) ) ;
#37395=CARTESIAN_POINT ( 'NONE',  ( 765.0180583372156207, -216.9982390220562252, -360.0135310231089534 ) ) ;
#37396=CARTESIAN_POINT ( 'NONE',  ( 795.1360043628808398, -404.0891481129646650, -360.2193346964456282 ) ) ;
#37399=CARTESIAN_POINT ( 'NONE',  ( 802.1676090361156639, -110.6346026584201638, -327.8955696845344505 ) ) ;
#37407=CARTESIAN_POINT ( 'NONE',  ( 745.5313806188320314, -447.2817908451521021, -333.7943932421247268 ) ) ;
#37408=CARTESIAN_POINT ( 'NONE',  ( 767.7687537140311633, -47.90732993114767169, -372.7932403749916830 ) ) ;
#37411=CARTESIAN_POINT ( 'NONE',  ( 805.1927285166397041, -424.8164208402372992, -341.8018195045277707 ) ) ;
#37412=CARTESIAN_POINT ( 'NONE',  ( 768.0187753319979720, -8.634602658420517329, -318.0580252608186242 ) ) ;
#37416=CARTESIAN_POINT ( 'NONE',  ( 796.9571628226829034, -287.4636090269708575, -321.2382568024804641 ) ) ;
#37417=CARTESIAN_POINT ( 'NONE',  ( 749.2812353651451076, -174.4527844766018063, -323.2262854647983090 ) ) ;
#37421=CARTESIAN_POINT ( 'NONE',  ( 791.3765159950071393, 16.45630643248849623, -314.4691821868552211 ) ) ;
#37423=CARTESIAN_POINT ( 'NONE',  ( 803.8556311672234642, -225.6237781080506011, -365.6418435158340117 ) ) ;
#37428=CARTESIAN_POINT ( 'NONE',  ( 774.6312213355099630, -359.3618753856920875, -364.6798772138717482 ) ) ;
#37431=CARTESIAN_POINT ( 'NONE',  ( 749.5768839229115201, -108.5545181178803915, -358.0661480581553064 ) ) ;
#37432=CARTESIAN_POINT ( 'NONE',  ( 756.1348686366196716, -161.2601417444143976, -347.5531968255698416 ) ) ;
#37435=CARTESIAN_POINT ( 'NONE',  ( 762.3223304703356007, -79.54369356751119824, -322.3223304703362828 ) ) ;
#37436=CARTESIAN_POINT ( 'NONE',  ( 803.8651313633788504, -149.2601417444144261, -332.4468031744301015 ) ) ;
#37438=CARTESIAN_POINT ( 'NONE',  ( 795.6651683502461765, -10.71468719896033761, -371.3240766477733814 ) ) ;
#37444=CARTESIAN_POINT ( 'NONE',  ( 812.3518521366052028, -265.0999726633344267, -326.5853460496235243 ) ) ;
#37452=CARTESIAN_POINT ( 'NONE',  ( 793.9708237608222134, -118.9181544815167229, -319.2295555964448681 ) ) ;
#37453=CARTESIAN_POINT ( 'NONE',  ( 795.1360043628807261, -116.0891481129656029, -360.2193346964456282 ) ) ;
#37454=CARTESIAN_POINT ( 'NONE',  ( 795.1360043628808398, -308.0891481129650629, -360.2193346964456282 ) ) ;
#37456=CARTESIAN_POINT ( 'NONE',  ( 755.0636971347428243, -436.2709662947827951, -341.7834795799807353 ) ) ;
#37461=ORIENTED_EDGE ( 'NONE', *, *, #40197, .T. ) ;
#37462=CARTESIAN_POINT ( 'NONE',  ( 810.4231160770870019, -360.5545181178796383, -321.9338519418446936 ) ) ;
#37464=CARTESIAN_POINT ( 'NONE',  ( 800.2193346964447755, -306.9982390220558273, -355.1360043628815788 ) ) ;
#37467=CARTESIAN_POINT ( 'NONE',  ( 805.2837595273609850, -194.7363362996982517, -340.5290396650784714 ) ) ;
#37469=DIRECTION ( 'NONE',  ( 0.000000000000000000, 0.000000000000000000, -1.000000000000000000 ) ) ;
#37470=CARTESIAN_POINT ( 'NONE',  ( 812.7932403749906598, -399.1800572038738437, -327.7687537140311633 ) ) ;
#37477=CARTESIAN_POINT ( 'NONE',  ( 782.4968714119720516, -34.81642084023861372, -305.0891759886411023 ) ) ;
#37478=CARTESIAN_POINT ( 'NONE',  ( 778.2165204200184689, -262.8164208402379245, -364.9363028652563230 ) ) ;
#37482=CARTESIAN_POINT ( 'NONE',  ( 796.7845633553578182, -57.62377810805111267, -358.5707757039688204 ) ) ;
#37489=CARTESIAN_POINT ( 'NONE',  ( 759.2295555964440155, -376.1692326535046504, -353.9708237608231229 ) ) ;
#37492=CARTESIAN_POINT ( 'NONE',  ( 771.2368401574024119, -373.4419599262319593, -374.2805881961240857 ) ) ;
#37496=ORIENTED_EDGE ( 'NONE', *, *, #25320, .F. ) ;
#37498=CARTESIAN_POINT ( 'NONE',  ( 763.2262854647970016, -200.6346026584199365, -309.2812353651462445 ) ) ;
#37501=CARTESIAN_POINT ( 'NONE',  ( 757.8323909638828582, -194.6346026584199080, -352.1044303154654358 ) ) ;
#37504=CARTESIAN_POINT ( 'NONE',  ( 800.0135310231082713, -326.0891481129649492, -325.0180583372163028 ) ) ;
#37505=CARTESIAN_POINT ( 'NONE',  ( 794.9819416627830151, 11.00176097794305541, -319.9864689768909898 ) ) ;
#37512=CARTESIAN_POINT ( 'NONE',  ( 780.5236548040995785, -452.7363362996975411, -314.9735926884559944 ) ) ;
#37513=CARTESIAN_POINT ( 'NONE',  ( 779.9999999999990905, 18.49609980828599376, -309.9999999999999432 ) ) ;
#37514=CARTESIAN_POINT ( 'NONE',  ( 767.9999999999992042, 205.0000000000000568, -319.9999999999999432 ) ) ;
#37516=CARTESIAN_POINT ( 'NONE',  ( 815.3608509340175488, -242.7363362996980811, -341.2497674668889545 ) ) ;
#37519=CARTESIAN_POINT ( 'NONE',  ( 767.8955696845333705, -192.4527844766016926, -362.1676090361162323 ) ) ;
#37520=CARTESIAN_POINT ( 'NONE',  ( 761.2382568024794409, -375.6237781080501463, -356.9571628226838129 ) ) ;
#37521=CARTESIAN_POINT ( 'NONE',  ( 755.8990559732751535, -227.4636090269709143, -365.9055244015606831 ) ) ;
#37524=CARTESIAN_POINT ( 'NONE',  ( 779.4763451958990572, -80.73633629969864955, -365.0264073115438919 ) ) ;
#37527=CARTESIAN_POINT ( 'NONE',  ( 790.8726784830453198, -418.7146871989590409, -362.5472867521010585 ) ) ;
#37528=CARTESIAN_POINT ( 'NONE',  ( 749.2812353651451076, -270.4527844766014937, -323.2262854647983090 ) ) ;
#37531=CARTESIAN_POINT ( 'NONE',  ( 765.0180583372156207, -48.99823902205675807, -360.0135310231089534 ) ) ;
#37533=CARTESIAN_POINT ( 'NONE',  ( 758.0141637701419768, -159.0783235625962391, -367.2620300519063790 ) ) ;
#37535=CARTESIAN_POINT ( 'NONE',  ( 751.9810565676468741, -410.0891481129647218, -360.9747183278973921 ) ) ;
#37539=CARTESIAN_POINT ( 'NONE',  ( 801.9419747391806368, -426.4527844766010389, -351.9812246680014027 ) ) ;
#37545=CARTESIAN_POINT ( 'NONE',  ( 756.1348686366196716, -233.2601417444141987, -347.5531968255698416 ) ) ;
#37547=CARTESIAN_POINT ( 'NONE',  ( 746.0683387631852383, -259.4419599262322436, -331.3260364891676204 ) ) ;
#37548=DIRECTION ( 'NONE',  ( 0.000000000000000000, 1.000000000000000000, -1.110223024625155554E-15 ) ) ;
#37551=CARTESIAN_POINT ( 'NONE',  ( 797.8594530101008786, -181.5436935675108145, -322.1405469898980982 ) ) ;
#37553=CARTESIAN_POINT ( 'NONE',  ( 754.9967657858570647, -121.5436935675110419, -365.0032342141425374 ) ) ;
#37554=CARTESIAN_POINT ( 'NONE',  ( 803.6646147819162707, -65.90732993114760063, -348.8264449731211130 ) ) ;
#37556=CARTESIAN_POINT ( 'NONE',  ( 755.1538015810308480, -62.19088175424416676, -343.0433043558613804 ) ) ;
#37557=VERTEX_POINT ( 'NONE', #7910 ) ;
#37558=CARTESIAN_POINT ( 'NONE',  ( 790.9844846989617508, -358.3726999360613945, -317.2208543904092721 ) ) ;
#37565=CARTESIAN_POINT ( 'NONE',  ( 804.8461984189677878, -314.1908817542433781, -336.9566956441385628 ) ) ;
#37566=CARTESIAN_POINT ( 'NONE',  ( 805.1927285166397041, -328.8164208402375834, -341.8018195045277707 ) ) ;
#37567=CARTESIAN_POINT ( 'NONE',  ( 788.6739635108323228, -127.6454272087894140, -373.9316612368139090 ) ) ;
#37572=CARTESIAN_POINT ( 'NONE',  ( 805.0264073115434940, -270.3510508353231216, -339.4763451958999099 ) ) ;
#37573=CARTESIAN_POINT ( 'NONE',  ( 797.8822607201568644, -126.5545181178803205, -370.1134526219340160 ) ) ;
#37581=CARTESIAN_POINT ( 'NONE',  ( 805.0032342141413437, -157.5436935675109282, -314.9967657858572352 ) ) ;
#37584=CARTESIAN_POINT ( 'NONE',  ( 745.4481719005789273, -315.7255117493286320, -347.5162901302853129 ) ) ;
#37589=CARTESIAN_POINT ( 'NONE',  ( 746.7653713866222915, -353.2601417444137724, -351.0478386215610271 ) ) ;
#37590=CARTESIAN_POINT ( 'NONE',  ( 755.2512626584698410, -127.5436935675110561, -315.2512626584710915 ) ) ;
#37592=CARTESIAN_POINT ( 'NONE',  ( 796.9462024416508257, -372.4527844766010958, -308.9653473494370246 ) ) ;
#37598=CARTESIAN_POINT ( 'NONE',  ( 801.9858362298568863, -171.0783235625962106, -312.7379699480935642 ) ) ;
#37603=CARTESIAN_POINT ( 'NONE',  ( 756.7813123517142913, 4.012585528312341054, -329.9779781133712504 ) ) ;
#37605=CARTESIAN_POINT ( 'NONE',  ( 807.5423716828161105, -441.0783235625953580, -362.2119215644372048 ) ) ;
#37609=CARTESIAN_POINT ( 'NONE',  ( 813.5763878283155464, -387.8272453906067767, -351.1614460488615350 ) ) ;
#37613=CARTESIAN_POINT ( 'NONE',  ( 790.0220218866281812, -223.0999726633346256, -363.2186876482849129 ) ) ;
#37614=CARTESIAN_POINT ( 'NONE',  ( 804.4286716492782716, -209.3618753856926276, -345.3141322388244703 ) ) ;
#37615=CARTESIAN_POINT ( 'NONE',  ( 778.2165204200184689, -430.8164208402374129, -364.9363028652563230 ) ) ;
#37617=CARTESIAN_POINT ( 'NONE',  ( 762.1405469898971887, -97.54369356751112718, -357.8594530101015607 ) ) ;
#37618=VERTEX_POINT ( 'NONE', #32383 ) ;
#37621=CARTESIAN_POINT ( 'NONE',  ( 776.2046728542105711, -20.19088175424429110, -304.8212110874238761 ) ) ;
#37628=CARTESIAN_POINT ( 'NONE',  ( 807.2620300519052989, -432.0090635724247932, -318.0141637701419768 ) ) ;
#37629=CARTESIAN_POINT ( 'NONE',  ( 744.7301800767020268, -76.81642084023847872, -337.4774526936615189 ) ) ;
#37631=CARTESIAN_POINT ( 'NONE',  ( 774.6312213355099630, -431.3618753856918033, -364.6798772138717482 ) ) ;
#37632=CARTESIAN_POINT ( 'NONE',  ( 768.0187753319979720, -32.63460265842044095, -318.0580252608186242 ) ) ;
#37635=CARTESIAN_POINT ( 'NONE',  ( 804.1105419155481968, -291.8272453906071746, -347.6308680596136469 ) ) ;
#37636=CARTESIAN_POINT ( 'NONE',  ( 782.4968714119720516, -202.8164208402380950, -305.0891759886411023 ) ) ;
#37642=CARTESIAN_POINT ( 'NONE',  ( 801.9858362298568863, -243.0783235625959833, -312.7379699480935642 ) ) ;
#37645=CARTESIAN_POINT ( 'NONE',  ( 782.4968714119720516, -298.8164208402377540, -305.0891759886411023 ) ) ;
#37649=CARTESIAN_POINT ( 'NONE',  ( 778.1981804954714335, -346.2709662947830793, -314.8072714833589885 ) ) ;
#37652=CARTESIAN_POINT ( 'NONE',  ( 758.0141637701419768, -39.07832356259662276, -367.2620300519063790 ) ) ;
#37653=CARTESIAN_POINT ( 'NONE',  ( 798.7617431975189675, -171.6237781080507432, -323.0428371773161871 ) ) ;
#37657=CARTESIAN_POINT ( 'NONE',  ( 802.1676090361156639, -62.63460265842031305, -327.8955696845344505 ) ) ;
#37658=CARTESIAN_POINT ( 'NONE',  ( 754.8983024940795303, -162.8965053807780521, -336.9254006560228163 ) ) ;
#37661=CARTESIAN_POINT ( 'NONE',  ( 810.1134526219336749, -8.532869017142163059, -357.8822607201570349 ) ) ;
#37667=CARTESIAN_POINT ( 'NONE',  ( 771.3260364891663130, -283.6454272087889308, -306.0683387631859773 ) ) ;
#37676=CARTESIAN_POINT ( 'NONE',  ( 755.1538015810308480, -110.1908817542440033, -343.0433043558613804 ) ) ;
#37677=CARTESIAN_POINT ( 'NONE',  ( 755.0636971347428243, -124.2709662947837899, -341.7834795799807353 ) ) ;
#37678=CARTESIAN_POINT ( 'NONE',  ( 771.2633955100217236, -311.9073299311468759, -363.4237431249939618 ) ) ;
#37680=CARTESIAN_POINT ( 'NONE',  ( 768.0187753319979720, -416.6346026584192259, -318.0580252608186242 ) ) ;
#37683=DIRECTION ( 'NONE',  ( 0.000000000000000000, -0.000000000000000000, -1.000000000000000000 ) ) ;
#37689=CARTESIAN_POINT ( 'NONE',  ( 814.8207195650702488, -338.1908817542433212, -336.2433038121456548 ) ) ;
#37691=CARTESIAN_POINT ( 'NONE',  ( 755.0636971347428243, -340.2709662947831362, -341.7834795799807353 ) ) ;
#37693=CARTESIAN_POINT ( 'NONE',  ( 804.6971507214547046, -171.2817908451529263, -344.0799538623459739 ) ) ;
#37696=CARTESIAN_POINT ( 'NONE',  ( 755.2512626584698410, -391.5436935675101608, -315.2512626584710915 ) ) ;
#37702=CARTESIAN_POINT ( 'NONE',  ( 815.2698199232961542, -16.81642084023866701, -342.5225473063383106 ) ) ;
#37703=CARTESIAN_POINT ( 'NONE',  ( 771.2633955100217236, -263.9073299311469327, -363.4237431249939618 ) ) ;
#37707=CARTESIAN_POINT ( 'NONE',  ( 757.2208543904082489, -64.71468719896019195, -350.9844846989624330 ) ) ;
#37715=CARTESIAN_POINT ( 'NONE',  ( 756.5762568750052424, -75.18005720387485269, -348.7366044899774238 ) ) ;
#37716=CARTESIAN_POINT ( 'NONE',  ( 805.0264073115434940, -366.3510508353228374, -339.4763451958999099 ) ) ;
#37719=CARTESIAN_POINT ( 'NONE',  ( 793.4146539503750546, -361.9874144716864635, -307.6481478633938877 ) ) ;
#37721=ORIENTED_EDGE ( 'NONE', *, *, #16294, .T. ) ;
#37725=CARTESIAN_POINT ( 'NONE',  ( 782.4968714119720516, -202.8164208402380950, -305.0891759886411023 ) ) ;
#37727=EDGE_CURVE ( 'NONE', #38644, #35738, #23543, .T. ) ;
#37729=CARTESIAN_POINT ( 'NONE',  ( 768.0187753319979720, -224.6346026584198228, -318.0580252608186242 ) ) ;
#37731=CARTESIAN_POINT ( 'NONE',  ( 756.5762568750052424, -315.1800572038740711, -348.7366044899774238 ) ) ;
#37732=CARTESIAN_POINT ( 'NONE',  ( 778.1981804954714335, 13.72903370521577138, -314.8072714833589885 ) ) ;
#37739=CARTESIAN_POINT ( 'NONE',  ( 791.9460785601769430, -462.7578698805381237, -362.0383033825738721 ) ) ;
#37743=CARTESIAN_POINT ( 'NONE',  ( 797.8822607201568644, -246.5545181178799510, -370.1134526219340160 ) ) ;
#37747=CARTESIAN_POINT ( 'NONE',  ( 758.0580252608178853, -222.4527844766016642, -328.0187753319985404 ) ) ;
#37748=CARTESIAN_POINT ( 'NONE',  ( 784.0799538623451781, -371.8055962898682765, -364.6971507214555572 ) ) ;
#37750=CARTESIAN_POINT ( 'NONE',  ( 760.0363995740630116, -250.9181544815163534, -368.7758568127991907 ) ) ;
#37752=LINE ( 'NONE', #12581, #6105 ) ;
#37753=CARTESIAN_POINT ( 'NONE',  ( 790.0220218866281812, -79.09997266333503774, -363.2186876482849129 ) ) ;
#37757=CARTESIAN_POINT ( 'NONE',  ( 801.3366627262608972, -440.5328690171407970, -353.0897708529566899 ) ) ;
#37758=CARTESIAN_POINT ( 'NONE',  ( 810.7187646348534145, -282.4527844766014937, -356.7737145352016341 ) ) ;
#37761=CARTESIAN_POINT ( 'NONE',  ( 768.0187753319979720, -56.63460265842036279, -318.0580252608186242 ) ) ;
#37763=CARTESIAN_POINT ( 'NONE',  ( 776.2433038121456548, -156.8965053807780805, -374.8207195650711014 ) ) ;
#37765=CARTESIAN_POINT ( 'NONE',  ( 792.2312462859673587, -395.9073299311465348, -307.2067596250082602 ) ) ;
#37769=CARTESIAN_POINT ( 'NONE',  ( 778.2165204200184689, -430.8164208402374129, -364.9363028652563230 ) ) ;
#37775=ORIENTED_EDGE ( 'NONE', *, *, #13697, .T. ) ;
#37776=CARTESIAN_POINT ( 'NONE',  ( 793.2243759319678702, -266.5328690171413655, -318.4439275373583200 ) ) ;
#37779=CARTESIAN_POINT ( 'NONE',  ( 803.8556311672234642, -249.6237781080505158, -365.6418435158340117 ) ) ;
#37785=CARTESIAN_POINT ( 'NONE',  ( 804.4286716492782716, -161.3618753856927697, -345.3141322388244703 ) ) ;
#37787=CARTESIAN_POINT ( 'NONE',  ( 745.7998596910086917, -125.3618753856928834, -332.5602148656461168 ) ) ;
#37788=CARTESIAN_POINT ( 'NONE',  ( 800.2193346964446619, -90.99823902205662307, -355.1360043628816925 ) ) ;
#37790=CARTESIAN_POINT ( 'NONE',  ( 773.4516893846965786, -43.64542720878966975, -315.8398074228977066 ) ) ;
#37791=CARTESIAN_POINT ( 'NONE',  ( 763.0428371773158460, -347.4636090269705733, -358.7617431975195359 ) ) ;
#37799=CARTESIAN_POINT ( 'NONE',  ( 802.5472867521000353, -364.3726999360614514, -350.8726784830461156 ) ) ;
#37800=CARTESIAN_POINT ( 'NONE',  ( 788.7366044899766848, -323.9073299311468190, -316.5762568750059813 ) ) ;
#37802=CARTESIAN_POINT ( 'NONE',  ( 749.5768839229115201, -132.5545181178802920, -358.0661480581553064 ) ) ;
#37804=DIRECTION ( 'NONE',  ( -1.000000000000000000, 0.000000000000000000, 0.000000000000000000 ) ) ;
#37806=CARTESIAN_POINT ( 'NONE',  ( 796.7845633553578182, -273.6237781080504305, -358.5707757039688204 ) ) ;
#37807=CARTESIAN_POINT ( 'NONE',  ( 797.8822607201568644, -150.5545181178802352, -370.1134526219340160 ) ) ;
#37813=CARTESIAN_POINT ( 'NONE',  ( 808.0189434323515343, -182.0891481129654323, -319.0252816721025511 ) ) ;
#37816=CARTESIAN_POINT ( 'NONE',  ( 748.9653473494363425, -290.6346026584195101, -356.9462024416521331 ) ) ;
#37822=CARTESIAN_POINT ( 'NONE',  ( 788.7631598425961101, -361.4419599262319593, -305.7194118038759143 ) ) ;
#37823=CARTESIAN_POINT ( 'NONE',  ( 787.5162901302840055, -131.3618753856928834, -305.4481719005792684 ) ) ;
#37825=CARTESIAN_POINT ( 'NONE',  ( 748.9653473494363425, -386.6346026584191691, -356.9462024416521331 ) ) ;
#37830=CARTESIAN_POINT ( 'NONE',  ( 773.7943932421234194, -143.8055962898690154, -305.5313806188329409 ) ) ;
#37835=ORIENTED_EDGE ( 'NONE', *, *, #4424, .T. ) ;
#37836=CARTESIAN_POINT ( 'NONE',  ( 795.9930595647434757, -3.078323562596726681, -320.7433823573372820 ) ) ;
#37838=CARTESIAN_POINT ( 'NONE',  ( 747.2067596250078623, -3.180057203875080063, -352.2312462859687230 ) ) ;
#37842=CARTESIAN_POINT ( 'NONE',  ( 803.6646147819161570, -185.9073299311472454, -348.8264449731210561 ) ) ;
#37843=CARTESIAN_POINT ( 'NONE',  ( 746.4236121716829757, -399.8272453906067767, -328.8385539511384650 ) ) ;
#37846=CARTESIAN_POINT ( 'NONE',  ( 763.8424801807145741, -258.0090635724253616, -320.5453621957614700 ) ) ;
#37847=CARTESIAN_POINT ( 'NONE',  ( 762.1405469898971887, -217.5436935675107293, -357.8594530101015607 ) ) ;
#37848=CARTESIAN_POINT ( 'NONE',  ( 771.2633955100217236, -407.9073299311465348, -363.4237431249939618 ) ) ;
#37853=CARTESIAN_POINT ( 'NONE',  ( 797.8822607201568644, -6.554518117880697048, -370.1134526219340160 ) ) ;
#37860=CARTESIAN_POINT ( 'NONE',  ( 745.1792804349281596, -446.1908817542429802, -343.7566961878542884 ) ) ;
#37862=CARTESIAN_POINT ( 'NONE',  ( 763.2262854647970016, -80.63460265842029173, -309.2812353651462445 ) ) ;
#37865=CARTESIAN_POINT ( 'NONE',  ( 759.9864689768902508, -434.0891481129646081, -354.9819416627836404 ) ) ;
#37866=CARTESIAN_POINT ( 'NONE',  ( 755.5713283507202505, -29.36187538569318178, -334.6858677611754729 ) ) ;
#37868=CARTESIAN_POINT ( 'NONE',  ( 805.1927285166397041, 7.183579159761247723, -341.8018195045277707 ) ) ;
#37869=CARTESIAN_POINT ( 'NONE',  ( 814.2001403089898304, -185.3618753856926844, -347.4397851343538264 ) ) ;
#37874=CARTESIAN_POINT ( 'NONE',  ( 783.7566961878529810, -288.8965053807775121, -305.1792804349288417 ) ) ;
#37876=CARTESIAN_POINT ( 'NONE',  ( 763.0537975583475827, -288.4527844766014937, -371.0346526505627480 ) ) ;
#37880=CARTESIAN_POINT ( 'NONE',  ( 757.8323909638827445, -338.6346026584195101, -352.1044303154654358 ) ) ;
#37882=CARTESIAN_POINT ( 'NONE',  ( 771.2368401574024119, -37.44195992623299674, -374.2805881961240857 ) ) ;
#37883=CARTESIAN_POINT ( 'NONE',  ( 766.7756240680305382, -158.5328690171417065, -361.5560724626415663 ) ) ;
#37887=ORIENTED_EDGE ( 'NONE', *, *, #32039, .T. ) ;
#37888=CARTESIAN_POINT ( 'NONE',  ( 757.8323909638827445, -74.63460265842032015, -352.1044303154654358 ) ) ;
#37889=CARTESIAN_POINT ( 'NONE',  ( 759.2295555964440155, -160.1692326535053326, -353.9708237608231229 ) ) ;
#37892=CARTESIAN_POINT ( 'NONE',  ( 813.2346286133761168, 18.73985825558501972, -328.9521613784389160 ) ) ;
#37899=CARTESIAN_POINT ( 'NONE',  ( 760.0363995740630116, -322.9181544815161260, -368.7758568127991907 ) ) ;
#37903=CARTESIAN_POINT ( 'NONE',  ( 798.5707757039680246, -125.4636090269712412, -356.7845633553585003 ) ) ;
#37904=CARTESIAN_POINT ( 'NONE',  ( 792.1044303154645831, -108.4527844766019911, -317.8323909638837677 ) ) ;
#37905=CARTESIAN_POINT ( 'NONE',  ( 774.6312213355098493, -311.3618753856923149, -364.6798772138717482 ) ) ;
#37907=CARTESIAN_POINT ( 'NONE',  ( 768.0187753319979720, -440.6346026584191122, -318.0580252608186242 ) ) ;
#37915=CARTESIAN_POINT ( 'NONE',  ( 812.3518521366052028, -337.0999726633342561, -326.5853460496235243 ) ) ;
#37917=CARTESIAN_POINT ( 'NONE',  ( 801.9419747391806368, -330.4527844766013231, -351.9812246680014027 ) ) ;
#37918=DIRECTION ( 'NONE',  ( -1.000000000000000000, -0.000000000000000000, -0.000000000000000000 ) ) ;
#37919=CARTESIAN_POINT ( 'NONE',  ( 800.9840315886518738, -196.9181544815164386, -354.1144889064786412 ) ) ;
#37922=CARTESIAN_POINT ( 'NONE',  ( 763.0537975583476964, -384.4527844766011526, -371.0346526505628617 ) ) ;
#37928=CARTESIAN_POINT ( 'NONE',  ( 767.6429770376289525, -9.180057203875058747, -306.8695393053162093 ) ) ;
#37929=CARTESIAN_POINT ( 'NONE',  ( 792.1044303154645831, -252.4527844766015789, -317.8323909638837677 ) ) ;
#37931=FACE_OUTER_BOUND ( 'NONE', #33088, .T. ) ;
#37934=CARTESIAN_POINT ( 'NONE',  ( 761.2382568024794409, -39.62377810805116951, -356.9571628226838129 ) ) ;
#37943=CARTESIAN_POINT ( 'NONE',  ( 804.4286716492782716, -65.36187538569306810, -345.3141322388244703 ) ) ;
#37947=CARTESIAN_POINT ( 'NONE',  ( 761.2382568024794409, -351.6237781080502032, -356.9571628226838129 ) ) ;
#37950=CARTESIAN_POINT ( 'NONE',  ( 815.0009284576459549, -366.3510508353228374, -338.7629533639073429 ) ) ;
#37955=CARTESIAN_POINT ( 'NONE',  ( 800.9747183278959710, -228.9982390220561683, -311.9810565676471583 ) ) ;
#37958=CARTESIAN_POINT ( 'NONE',  ( 781.7834795799800531, -226.8164208402380098, -315.0636971347436202 ) ) ;
#37962=CARTESIAN_POINT ( 'NONE',  ( 757.8323909638827445, -338.6346026584195101, -352.1044303154654358 ) ) ;
#37963=CARTESIAN_POINT ( 'NONE',  ( 805.1927285166397041, 7.183579159761247723, -341.8018195045277707 ) ) ;
#37968=CARTESIAN_POINT ( 'NONE',  ( 772.4999999999993179, -462.9681489794448339, -369.0473750965555837 ) ) ;
#37971=CARTESIAN_POINT ( 'NONE',  ( 764.8639956371174549, 15.91085188703394238, -319.7806653035542013 ) ) ;
#37976=CARTESIAN_POINT ( 'NONE',  ( 768.9521613784389729, -225.8272453906072599, -373.2346286133773106 ) ) ;
#37980=CARTESIAN_POINT ( 'NONE',  ( 804.9363028652555840, -232.2709662947834488, -338.2165204200192079 ) ) ;
#37981=CARTESIAN_POINT ( 'NONE',  ( 803.2186876482843445, -391.9874144716864066, -350.0220218866286928 ) ) ;
#37982=CARTESIAN_POINT ( 'NONE',  ( 744.6391490659812007, -254.7363362996981095, -338.7502325331110455 ) ) ;
#37983=PLANE ( 'NONE',  #26744 ) ;
#37985=CARTESIAN_POINT ( 'NONE',  ( 755.8894580844503253, -87.82724539060770041, -332.3691319403863531 ) ) ;
#37987=CIRCLE ( 'NONE', #7027, 10.00000000000000888 ) ;
#37991=CARTESIAN_POINT ( 'NONE',  ( 759.2295555964440155, -424.1692326535044799, -353.9708237608231229 ) ) ;
#37992=CARTESIAN_POINT ( 'NONE',  ( 759.0252816721024374, -288.9982390220559978, -368.0189434323527280 ) ) ;
#37995=CARTESIAN_POINT ( 'NONE',  ( 754.8072714833581358, -76.81642084023845030, -338.1981804954720587 ) ) ;
#37998=CARTESIAN_POINT ( 'NONE',  ( 811.6461892240364477, -172.7146871989598083, -324.1737431748509835 ) ) ;
#38000=CARTESIAN_POINT ( 'NONE',  ( 805.0032342141412300, -421.5436935675101040, -314.9967657858571783 ) ) ;
#38006=CARTESIAN_POINT ( 'NONE',  ( 755.3201227861273992, -411.7255117493282910, -345.3687786644892981 ) ) ;
#38014=CARTESIAN_POINT ( 'NONE',  ( 754.8983024940795303, -258.8965053807777963, -336.9254006560228163 ) ) ;
#38016=CARTESIAN_POINT ( 'NONE',  ( 751.2241431872005251, -256.1692326535049915, -359.9636004259367610 ) ) ;
#38022=CARTESIAN_POINT ( 'NONE',  ( 770.0799878456142551, -61.98741447168745822, -362.9823548866085616 ) ) ;
#38023=CARTESIAN_POINT ( 'NONE',  ( 801.9419747391806368, -162.4527844766018632, -351.9812246680014027 ) ) ;
#38026=CARTESIAN_POINT ( 'NONE',  ( 787.5162901302840055, -107.3618753856928976, -305.4481719005792684 ) ) ;
#38027=CARTESIAN_POINT ( 'NONE',  ( 804.6798772138710092, -111.7255117493292857, -334.6312213355106451 ) ) ;
#38029=CARTESIAN_POINT ( 'NONE',  ( 796.1575198192839480, -54.00906357242601530, -359.4546378042384163 ) ) ;
#38030=CARTESIAN_POINT ( 'NONE',  ( 804.1105419155481968, -339.8272453906069472, -347.6308680596136469 ) ) ;
#38037=CARTESIAN_POINT ( 'NONE',  ( 755.3028492785439312, -375.2817908451523294, -335.9200461376539693 ) ) ;
#38038=CARTESIAN_POINT ( 'NONE',  ( 755.3201227861273992, -363.7255117493284047, -345.3687786644892981 ) ) ;
#38039=CARTESIAN_POINT ( 'NONE',  ( 802.2119215644370342, -126.0090635724257737, -367.5423716828165084 ) ) ;
#38044=CARTESIAN_POINT ( 'NONE',  ( 754.3581564841646241, -161.4636090269711133, -316.1443688327762516 ) ) ;
#38050=CARTESIAN_POINT ( 'NONE',  ( 772.5602148656447525, -177.7255117493290868, -305.7998596910095443 ) ) ;
#38053=CARTESIAN_POINT ( 'NONE',  ( 777.5031285880264704, -310.8164208402377540, -374.9108240113588408 ) ) ;
#38061=CARTESIAN_POINT ( 'NONE',  ( 811.6461892240364477, -388.7146871989592114, -324.1737431748509835 ) ) ;
#38062=CARTESIAN_POINT ( 'NONE',  ( 804.7487373415286811, -115.5436935675110988, -364.7487373415288516 ) ) ;
#38064=CARTESIAN_POINT ( 'NONE',  ( 772.4837098697144029, -383.3618753856921444, -374.5518280994205611 ) ) ;
#38067=ORIENTED_EDGE ( 'NONE', *, *, #40134, .T. ) ;
#38069=CARTESIAN_POINT ( 'NONE',  ( 814.8230680027162407, -149.8055962898689870, -333.7305795820267917 ) ) ;
#38074=CARTESIAN_POINT ( 'NONE',  ( 803.2186876482843445, -7.987414471687621642, -350.0220218866286928 ) ) ;
#38076=CARTESIAN_POINT ( 'NONE',  ( 796.7737145352015204, 3.365397341579444479, -370.7187646348536987 ) ) ;
#38079=CARTESIAN_POINT ( 'NONE',  ( 775.9200461376533440, -95.80559628986917176, -315.3028492785443291 ) ) ;
#38081=CARTESIAN_POINT ( 'NONE',  ( 781.7834795799800531, -178.8164208402381519, -315.0636971347436202 ) ) ;
#38082=CARTESIAN_POINT ( 'NONE',  ( 757.7880784355613741, -402.0090635724250205, -312.4576283171834916 ) ) ;
#38084=CARTESIAN_POINT ( 'NONE',  ( 778.1981804954714335, -250.2709662947832783, -314.8072714833589885 ) ) ;
#38088=CARTESIAN_POINT ( 'NONE',  ( 758.4439275373578084, -252.5545181178799226, -353.2243759319684386 ) ) ;
#38089=CARTESIAN_POINT ( 'NONE',  ( 800.2193346964447755, -258.9982390220561115, -355.1360043628815788 ) ) ;
#38090=CARTESIAN_POINT ( 'NONE',  ( 804.9363028652555840, -424.2709662947829088, -338.2165204200192079 ) ) ;
#38091=CARTESIAN_POINT ( 'NONE',  ( 785.3141322388236176, -69.72551174932942786, -364.4286716492789537 ) ) ;
#38096=CARTESIAN_POINT ( 'NONE',  ( 814.8207195650702488, -50.19088175424420939, -336.2433038121456548 ) ) ;
#38101=CARTESIAN_POINT ( 'NONE',  ( 769.9779781133707957, -19.09997266333520116, -316.7813123517150871 ) ) ;
#38102=CARTESIAN_POINT ( 'NONE',  ( 814.5518280994195948, -63.72551174932941365, -332.4837098697145166 ) ) ;
#38105=CARTESIAN_POINT ( 'NONE',  ( 788.7366044899766848, -443.9073299311464780, -316.5762568750059813 ) ) ;
#38106=CARTESIAN_POINT ( 'NONE',  ( 762.1405469898973024, -49.54369356751129772, -357.8594530101016176 ) ) ;
#38108=CARTESIAN_POINT ( 'NONE',  ( 814.5518280994195948, -183.7255117493290015, -332.4837098697145734 ) ) ;
#38115=PLANE ( 'NONE',  #32088 ) ;
#38116=CARTESIAN_POINT ( 'NONE',  ( 810.1134526219336749, -272.5328690171413086, -357.8822607201570349 ) ) ;
#38118=CARTESIAN_POINT ( 'NONE',  ( 748.9653473494363425, -290.6346026584195101, -356.9462024416521331 ) ) ;
#38122=CARTESIAN_POINT ( 'NONE',  ( 795.1360043628807261, -356.0891481129647218, -360.2193346964456282 ) ) ;
#38125=CARTESIAN_POINT ( 'NONE',  ( 778.2165204200184689, -190.8164208402381234, -364.9363028652563230 ) ) ;
#38126=CARTESIAN_POINT ( 'NONE',  ( 776.2433038121456548, -36.89650538077844288, -374.8207195650711014 ) ) ;
#38127=CARTESIAN_POINT ( 'NONE',  ( 789.9200121543843807, -145.9874144716871740, -317.0176451133914384 ) ) ;
#38131=CARTESIAN_POINT ( 'NONE',  ( 762.1405469898971887, -49.54369356751129061, -357.8594530101015607 ) ) ;
#38132=CARTESIAN_POINT ( 'NONE',  ( 789.9200121543843807, -169.9874144716871172, -317.0176451133914384 ) ) ;
#38134=CARTESIAN_POINT ( 'NONE',  ( 815.1787889125755555, -6.896505380778533478, -343.7953271457877804 ) ) ;
#38139=CARTESIAN_POINT ( 'NONE',  ( 752.7379699480933368, -324.0090635724251911, -361.9858362298580232 ) ) ;
#38144=CARTESIAN_POINT ( 'NONE',  ( 763.8424801807145741, -138.0090635724257311, -320.5453621957614700 ) ) ;
#38145=CARTESIAN_POINT ( 'NONE',  ( 757.8323909638827445, -122.6346026584201354, -352.1044303154654358 ) ) ;
#38146=CARTESIAN_POINT ( 'NONE',  ( 794.9819416627830151, -300.9982390220559409, -319.9864689768909898 ) ) ;
#38155=CARTESIAN_POINT ( 'NONE',  ( 814.8207195650702488, -386.1908817542432075, -336.2433038121456548 ) ) ;
#38160=CARTESIAN_POINT ( 'NONE',  ( 755.3201227861273992, -339.7255117493285184, -345.3687786644892981 ) ) ;
#38162=CARTESIAN_POINT ( 'NONE',  ( 786.5483106153019435, -175.6454272087892718, -364.1601925771022366 ) ) ;
#38165=CARTESIAN_POINT ( 'NONE',  ( 751.9810565676468741, -434.0891481129646081, -360.9747183278973921 ) ) ;
#38170=CARTESIAN_POINT ( 'NONE',  ( 772.4837098697144029, -47.36187538569312494, -374.5518280994205611 ) ) ;
#38171=CARTESIAN_POINT ( 'NONE',  ( 805.1927285166397041, -232.8164208402379245, -341.8018195045277707 ) ) ;
#38175=CARTESIAN_POINT ( 'NONE',  ( 786.2694204179717872, -21.28179084515337749, -305.1769319972829067 ) ) ;
#38176=CARTESIAN_POINT ( 'NONE',  ( 794.1144889064781864, -58.16923265350564520, -360.9840315886528401 ) ) ;
#38184=CARTESIAN_POINT ( 'NONE',  ( 771.2633955100217236, -47.90732993114767169, -363.4237431249939618 ) ) ;
#38185=CARTESIAN_POINT ( 'NONE',  ( 787.6308680596127942, -347.2601417444138860, -364.1105419155492768 ) ) ;
#38189=CARTESIAN_POINT ( 'NONE',  ( 747.3154664389472828, -355.9874144716865203, -326.4474001241230781 ) ) ;
#38194=CARTESIAN_POINT ( 'NONE',  ( 763.0537975583475827, -216.4527844766016926, -371.0346526505627480 ) ) ;
#38196=VERTEX_POINT ( 'NONE', #10562 ) ;
#38197=CARTESIAN_POINT ( 'NONE',  ( 797.6776695296629214, -211.5436935675107861, -357.6776695296636603 ) ) ;
#38199=CARTESIAN_POINT ( 'NONE',  ( 757.8323909638827445, -362.6346026584194533, -352.1044303154654358 ) ) ;
#38200=CARTESIAN_POINT ( 'NONE',  ( 755.3201227861273992, -27.72551174932954510, -345.3687786644892981 ) ) ;
#38206=CARTESIAN_POINT ( 'NONE',  ( 800.2193346964447755, 5.001760977943074948, -355.1360043628815788 ) ) ;
#38209=CARTESIAN_POINT ( 'NONE',  ( 757.7880784355613741, -234.0090635724255037, -312.4576283171834916 ) ) ;
#38213=CARTESIAN_POINT ( 'NONE',  ( 804.6798772138708955, -231.7255117493288310, -334.6312213355107019 ) ) ;
#38214=CARTESIAN_POINT ( 'NONE',  ( 759.2295555964440155, -400.1692326535045936, -353.9708237608231229 ) ) ;
#38217=CARTESIAN_POINT ( 'NONE',  ( 802.9823548866075953, -73.09997266333502353, -330.0799878456151077 ) ) ;
#38221=CARTESIAN_POINT ( 'NONE',  ( 752.4576283171824116, 2.921676437403253779, -317.7880784355627952 ) ) ;
#38222=CARTESIAN_POINT ( 'NONE',  ( 792.3570229623691148, -285.1800572038741279, -373.1304606946836770 ) ) ;
#38223=FACE_BOUND ( 'NONE', #35906, .T. ) ;
#38225=CARTESIAN_POINT ( 'NONE',  ( 797.8594530101008786, -85.54369356751118403, -322.1405469898980982 ) ) ;
#38227=CARTESIAN_POINT ( 'NONE',  ( 786.2056067578752163, -179.8055962898688733, -374.4686193811670023 ) ) ;
#38229=CARTESIAN_POINT ( 'NONE',  ( 804.7487373415286811, -403.5436935675101608, -364.7487373415288516 ) ) ;
#38233=ADVANCED_FACE ( 'NONE', ( #3464 ), #16871, .F. ) ;
#38234=CARTESIAN_POINT ( 'NONE',  ( 764.8639956371174549, -416.0891481129645513, -319.7806653035542013 ) ) ;
#38241=CARTESIAN_POINT ( 'NONE',  ( 795.9930595647434757, -243.0783235625959833, -320.7433823573372820 ) ) ;
#38242=EDGE_CURVE ( 'NONE', #26190, #15909, #219, .T. ) ;
#38244=CARTESIAN_POINT ( 'NONE',  ( 814.8230680027162407, -269.8055962898686175, -333.7305795820267917 ) ) ;
#38250=CARTESIAN_POINT ( 'NONE',  ( 805.1016975059191054, -30.89650538077846065, -343.0745993439771837 ) ) ;
#38251=CARTESIAN_POINT ( 'NONE',  ( 778.2165204200184689, -190.8164208402381234, -364.9363028652563230 ) ) ;
#38253=CARTESIAN_POINT ( 'NONE',  ( 745.4481719005789273, -123.7255117493292147, -347.5162901302853129 ) ) ;
#38254=CARTESIAN_POINT ( 'NONE',  ( 792.1044303154646968, -108.4527844766020053, -317.8323909638837677 ) ) ;
#38256=CARTESIAN_POINT ( 'NONE',  ( 804.8461984189677878, -50.19088175424420939, -336.9566956441385628 ) ) ;
#38257=CARTESIAN_POINT ( 'NONE',  ( 779.4763451958990572, -392.7363362996977116, -365.0264073115438919 ) ) ;
#38258=EDGE_CURVE ( 'NONE', #16020, #15909, #3222, .T. ) ;
#38267=CARTESIAN_POINT ( 'NONE',  ( 775.8780910478218402, -345.2817908451523863, -364.9511171171680530 ) ) ;
#38268=CARTESIAN_POINT ( 'NONE',  ( 754.8072714833581358, -364.8164208402374697, -338.1981804954720587 ) ) ;
#38269=CARTESIAN_POINT ( 'NONE',  ( 755.8990559732751535, -131.4636090269711985, -365.9055244015606831 ) ) ;
#38273=CARTESIAN_POINT ( 'NONE',  ( 760.5453621957607311, -309.0783235625957559, -323.8424801807151425 ) ) ;
#38274=CARTESIAN_POINT ( 'NONE',  ( 814.8207195650702488, -146.1908817542438896, -336.2433038121456548 ) ) ;
#38281=CARTESIAN_POINT ( 'NONE',  ( 777.5031285880264704, -166.8164208402382087, -374.9108240113588408 ) ) ;
#38284=CARTESIAN_POINT ( 'NONE',  ( 772.5602148656447525, -321.7255117493286320, -305.7998596910095443 ) ) ;
#38290=CARTESIAN_POINT ( 'NONE',  ( 764.3348316497523456, -382.7146871989591546, -308.6759233522265617 ) ) ;
#38291=CARTESIAN_POINT ( 'NONE',  ( 758.8095938919642549, -128.0891481129655176, -311.6929314249763365 ) ) ;
#38293=CARTESIAN_POINT ( 'NONE',  ( 801.1904061080336987, -404.0891481129646081, -368.3070685750235498 ) ) ;
#38297=ORIENTED_EDGE ( 'NONE', *, *, #37393, .F. ) ;
#38298=CARTESIAN_POINT ( 'NONE',  ( 745.1769319972822814, -161.8055962898689870, -346.2694204179732083 ) ) ;
#38304=CARTESIAN_POINT ( 'NONE',  ( 815.2698199232961542, -16.81642084023866701, -342.5225473063383106 ) ) ;
#38307=CARTESIAN_POINT ( 'NONE',  ( 745.7194118038753459, -421.6454272087885329, -348.7631598425976449 ) ) ;
#38311=CARTESIAN_POINT ( 'NONE',  ( 756.3353852180819104, -269.9073299311468190, -331.1735550268788302 ) ) ;
#38314=EDGE_CURVE ( 'NONE', #43845, #43683, #692, .T. ) ;
#38315=CARTESIAN_POINT ( 'NONE',  ( 804.4086373105744769, -265.6454272087889876, -333.3843516231986541 ) ) ;
#38316=CARTESIAN_POINT ( 'NONE',  ( 785.3141322388236176, -237.7255117493289163, -364.4286716492789537 ) ) ;
#38317=CARTESIAN_POINT ( 'NONE',  ( 768.0187753319979720, -440.6346026584191122, -318.0580252608186242 ) ) ;
#38318=CARTESIAN_POINT ( 'NONE',  ( 795.1360043628807261, -92.08914811296568814, -360.2193346964456282 ) ) ;
#38322=LINE ( 'NONE', #31827, #32988 ) ;
#38323=CARTESIAN_POINT ( 'NONE',  ( 776.2046728542105711, -44.19088175424421649, -304.8212110874238761 ) ) ;
#38329=CARTESIAN_POINT ( 'NONE',  ( 776.9254006560222479, -20.19088175424429110, -314.8983024940802125 ) ) ;
#38330=CARTESIAN_POINT ( 'NONE',  ( 767.6429770376291799, -57.18005720387490243, -306.8695393053162093 ) ) ;
#38332=CARTESIAN_POINT ( 'NONE',  ( 756.3353852180819104, -437.9073299311463074, -331.1735550268788302 ) ) ;
#38333=CARTESIAN_POINT ( 'NONE',  ( 755.0636971347428243, -52.27096629478401724, -341.7834795799807353 ) ) ;
#38335=CARTESIAN_POINT ( 'NONE',  ( 805.0032342141412300, -205.5436935675108430, -314.9967657858571783 ) ) ;
#38340=CARTESIAN_POINT ( 'NONE',  ( 744.8212110874229666, -282.8965053807776258, -336.2046728542121627 ) ) ;
#38343=CARTESIAN_POINT ( 'NONE',  ( 744.7301800767019131, -268.8164208402378108, -337.4774526936615757 ) ) ;
#38344=DIRECTION ( 'NONE',  ( -1.000000000000000000, -0.000000000000000000, -0.000000000000000000 ) ) ;
#38347=CARTESIAN_POINT ( 'NONE',  ( 804.9363028652555840, -400.2709662947828519, -338.2165204200192079 ) ) ;
#38349=CARTESIAN_POINT ( 'NONE',  ( 758.0141637701419768, -63.07832356259653750, -367.2620300519063790 ) ) ;
#38350=CARTESIAN_POINT ( 'NONE',  ( 780.5290396650775619, -180.3510508353234343, -365.2837595273619513 ) ) ;
#38355=CARTESIAN_POINT ( 'NONE',  ( 804.6798772138708955, -63.72551174932939233, -334.6312213355107019 ) ) ;
#38356=CARTESIAN_POINT ( 'NONE',  ( 761.2382568024794409, -207.6237781080506295, -356.9571628226838129 ) ) ;
#38358=CARTESIAN_POINT ( 'NONE',  ( 793.4146539503750546, -1.987414471687640294, -307.6481478633938877 ) ) ;
#38361=ORIENTED_EDGE ( 'NONE', *, *, #4352, .T. ) ;
#38363=CARTESIAN_POINT ( 'NONE',  ( 762.1177392798416577, -306.5545181178797520, -309.8865473780659272 ) ) ;
#38367=CARTESIAN_POINT ( 'NONE',  ( 802.5472867521000353, -148.3726999360620198, -350.8726784830461156 ) ) ;
#38368=CARTESIAN_POINT ( 'NONE',  ( 788.7366044899766848, -131.9073299311473875, -316.5762568750059813 ) ) ;
#38369=CARTESIAN_POINT ( 'NONE',  ( 797.6776695296629214, -307.5436935675104451, -357.6776695296636603 ) ) ;
#38376=CARTESIAN_POINT ( 'NONE',  ( 783.7953271457878373, -392.1908817542432075, -375.1787889125761239 ) ) ;
#38381=CARTESIAN_POINT ( 'NONE',  ( 785.3687786644884454, -323.3618753856923149, -315.3201227861279676 ) ) ;
#38383=CARTESIAN_POINT ( 'NONE',  ( 757.0176451133909268, -205.0999726633346256, -349.9200121543848354 ) ) ;
#38386=CARTESIAN_POINT ( 'NONE',  ( 815.2698199232962679, -424.8164208402373561, -342.5225473063383674 ) ) ;
#38389=CARTESIAN_POINT ( 'NONE',  ( 808.6142084849417415, -454.8672832770561740, -349.9915990122670451 ) ) ;
#38391=CARTESIAN_POINT ( 'NONE',  ( 813.1304606946830518, -65.90732993114758642, -352.3570229623690580 ) ) ;
#38392=CARTESIAN_POINT ( 'NONE',  ( 800.0135310231082713, -278.0891481129651197, -325.0180583372163028 ) ) ;
#38396=CARTESIAN_POINT ( 'NONE',  ( 804.1009440267234822, -23.46360902697155026, -314.0944755984392600 ) ) ;
#38397=CARTESIAN_POINT ( 'NONE',  ( 794.1144889064781864, -34.16923265350572336, -360.9840315886528401 ) ) ;
#38405=CARTESIAN_POINT ( 'NONE',  ( 755.5713283507202505, -53.36187538569310362, -334.6858677611754729 ) ) ;
#38406=CARTESIAN_POINT ( 'NONE',  ( 769.1273215169530886, -358.7146871989592114, -317.4527132478988847 ) ) ;
#38410=CARTESIAN_POINT ( 'NONE',  ( 808.7758568127978833, -412.1692326535045936, -320.0363995740631822 ) ) ;
#38415=CARTESIAN_POINT ( 'NONE',  ( 758.8095938919642549, -224.0891481129653187, -311.6929314249763365 ) ) ;
#38418=CARTESIAN_POINT ( 'NONE',  ( 771.1735550268780344, -225.1800572038743553, -316.3353852180828198 ) ) ;
#38420=CARTESIAN_POINT ( 'NONE',  ( 781.8018195045266339, -358.2709662947829088, -365.1927285166406705 ) ) ;
#38421=CARTESIAN_POINT ( 'NONE',  ( 762.1405469898971887, -1.543693567511449150, -357.8594530101015607 ) ) ;
#38426=VERTEX_POINT ( 'NONE', #20767 ) ;
#38427=CARTESIAN_POINT ( 'NONE',  ( 784.1219089521767955, -453.2817908451519315, -315.0488828828318333 ) ) ;
#38430=CARTESIAN_POINT ( 'NONE',  ( 805.6418435158337843, -269.4636090269708006, -363.8556311672236916 ) ) ;
#38433=CARTESIAN_POINT ( 'NONE',  ( 759.9864689768902508, -218.0891481129653187, -354.9819416627836404 ) ) ;
#38434=CARTESIAN_POINT ( 'NONE',  ( 761.2382568024794409, -399.6237781080500326, -356.9571628226838129 ) ) ;
#38437=CARTESIAN_POINT ( 'NONE',  ( 758.4439275373578084, -108.5545181178803915, -353.2243759319684386 ) ) ;
#38440=CARTESIAN_POINT ( 'NONE',  ( 805.9055244015594326, 20.37622189194865285, -315.8990559732753240 ) ) ;
#38441=CARTESIAN_POINT ( 'NONE',  ( 755.2512626584698410, -319.5436935675104451, -315.2512626584710915 ) ) ;
#38444=CARTESIAN_POINT ( 'NONE',  ( 759.7806653035534055, -78.99823902205662307, -324.8639956371180801 ) ) ;
#38446=CARTESIAN_POINT ( 'NONE',  ( 752.4576283171824116, -165.0783235625962391, -317.7880784355627952 ) ) ;
#38448=CARTESIAN_POINT ( 'NONE',  ( 815.2698199232961542, -448.8164208402371855, -342.5225473063383106 ) ) ;
#38452=CARTESIAN_POINT ( 'NONE',  ( 755.0636971347428243, -412.2709662947829088, -341.7834795799807353 ) ) ;
#38458=CARTESIAN_POINT ( 'NONE',  ( 783.0433043558608688, -264.8965053807776826, -315.1538015810313027 ) ) ;
#38460=CARTESIAN_POINT ( 'NONE',  ( 747.3154664389472828, -283.9874144716867477, -326.4474001241230781 ) ) ;
#38465=CARTESIAN_POINT ( 'NONE',  ( 756.3353852180819104, -149.9073299311473875, -331.1735550268788302 ) ) ;
#38466=CARTESIAN_POINT ( 'NONE',  ( 767.8955696845333705, -216.4527844766016926, -362.1676090361162323 ) ) ;
#38469=CARTESIAN_POINT ( 'NONE',  ( 744.7301800767019131, -100.8164208402383792, -337.4774526936615757 ) ) ;
#38471=CARTESIAN_POINT ( 'NONE',  ( 764.8639956371174549, -104.0891481129656739, -319.7806653035542581 ) ) ;
#38473=CARTESIAN_POINT ( 'NONE',  ( 793.0897708529556667, -390.5545181178794678, -361.3366627262616362 ) ) ;
#38481=CARTESIAN_POINT ( 'NONE',  ( 769.9779781133707957, -355.0999726633341993, -316.7813123517150871 ) ) ;
#38482=CARTESIAN_POINT ( 'NONE',  ( 755.0636971347428243, -340.2709662947831362, -341.7834795799807353 ) ) ;
#38483=CARTESIAN_POINT ( 'NONE',  ( 814.8207195650702488, -170.1908817542438328, -336.2433038121456548 ) ) ;
#38487=CARTESIAN_POINT ( 'NONE',  ( 794.1144889064781864, -298.1692326535049347, -360.9840315886528401 ) ) ;
#38488=CARTESIAN_POINT ( 'NONE',  ( 788.7366044899766848, -443.9073299311464780, -316.5762568750059813 ) ) ;
#38489=CARTESIAN_POINT ( 'NONE',  ( 764.1737431748507561, -154.3726999360620198, -371.6461892240376415 ) ) ;
#38494=CARTESIAN_POINT ( 'NONE',  ( 796.9462024416508257, -204.4527844766016926, -308.9653473494370246 ) ) ;
#38497=CARTESIAN_POINT ( 'NONE',  ( 800.9747183278959710, -348.9982390220558273, -311.9810565676471583 ) ) ;
#38504=CARTESIAN_POINT ( 'NONE',  ( 810.1134526219336749, -368.5328690171409676, -357.8822607201570349 ) ) ;
#38505=CARTESIAN_POINT ( 'NONE',  ( 763.0537975583475827, -120.4527844766019484, -371.0346526505627480 ) ) ;
#38507=CARTESIAN_POINT ( 'NONE',  ( 754.9967657858570647, -433.5436935675099903, -365.0032342141425374 ) ) ;
#38510=EDGE_LOOP ( 'NONE', ( #19428, #35272 ) ) ;
#38512=CARTESIAN_POINT ( 'NONE',  ( 744.8212110874229666, -162.8965053807780521, -336.2046728542121627 ) ) ;
#38516=ORIENTED_EDGE ( 'NONE', *, *, #30652, .F. ) ;
#38517=CARTESIAN_POINT ( 'NONE',  ( 756.7813123517142913, -19.98741447168758256, -329.9779781133712504 ) ) ;
#38520=CARTESIAN_POINT ( 'NONE',  ( 767.6429770376289525, -9.180057203875058747, -306.8695393053162093 ) ) ;
#38521=AXIS2_PLACEMENT_3D ( 'NONE', #15701, #5082, #30235 ) ;
#38524=CARTESIAN_POINT ( 'NONE',  ( 776.2046728542105711, -404.1908817542431507, -304.8212110874238761 ) ) ;
#38527=CARTESIAN_POINT ( 'NONE',  ( 755.5713283507202505, -269.3618753856924286, -334.6858677611754729 ) ) ;
#38531=CARTESIAN_POINT ( 'NONE',  ( 800.9840315886518738, -244.9181544815162681, -354.1144889064786412 ) ) ;
#38532=CARTESIAN_POINT ( 'NONE',  ( 795.1360043628807261, -236.0891481129651766, -360.2193346964456282 ) ) ;
#38535=CARTESIAN_POINT ( 'NONE',  ( 759.9864689768902508, -98.08914811296568814, -354.9819416627836404 ) ) ;
#38541=CARTESIAN_POINT ( 'NONE',  ( 778.7629533639073998, -56.73633629969872771, -375.0009284576466371 ) ) ;
#38547=CARTESIAN_POINT ( 'NONE',  ( 754.7162404726377645, -14.73633629969885384, -339.4709603349214717 ) ) ;
#38548=CARTESIAN_POINT ( 'NONE',  ( 801.1904061080338124, -68.08914811296577341, -368.3070685750236066 ) ) ;
#38552=CARTESIAN_POINT ( 'NONE',  ( 767.7687537140311633, -215.9073299311471317, -372.7932403749916830 ) ) ;
#38558=CARTESIAN_POINT ( 'NONE',  ( 758.0141637701419768, -279.0783235625958127, -367.2620300519063790 ) ) ;
#38561=CARTESIAN_POINT ( 'NONE',  ( 751.6929314249748586, -294.9982390220560546, -318.8095938919659034 ) ) ;
#38565=CARTESIAN_POINT ( 'NONE',  ( 810.1134526219336749, -32.53286901714208312, -357.8822607201570349 ) ) ;
#38566=CARTESIAN_POINT ( 'NONE',  ( 802.1676090361156639, -374.6346026584192828, -327.8955696845344505 ) ) ;
#38569=CARTESIAN_POINT ( 'NONE',  ( 761.9338519418445230, -62.53286901714199786, -370.4231160770881957 ) ) ;
#38570=CARTESIAN_POINT ( 'NONE',  ( 773.3843516231979720, -205.4419599262324425, -364.4086373105754433 ) ) ;
#38574=CARTESIAN_POINT ( 'NONE',  ( 755.0488828828309806, -209.8055962898687881, -344.1219089521771934 ) ) ;
#38577=CARTESIAN_POINT ( 'NONE',  ( 793.4146539503750546, -25.98741447168755769, -307.6481478633938877 ) ) ;
#38583=CARTESIAN_POINT ( 'NONE',  ( 809.0717654672305343, -316.9181544815160692, -360.1688906516309885 ) ) ;
#38587=CARTESIAN_POINT ( 'NONE',  ( 787.5531968255692163, -141.8272453906075157, -316.1348686366205811 ) ) ;
#38588=CARTESIAN_POINT ( 'NONE',  ( 791.9812246680005501, -140.6346026584201070, -361.9419747391813189 ) ) ;
#38590=CARTESIAN_POINT ( 'NONE',  ( 764.8639956371174549, -344.0891481129648355, -319.7806653035542581 ) ) ;
#38597=VERTEX_POINT ( 'NONE', #2170 ) ;
#38598=CARTESIAN_POINT ( 'NONE',  ( 781.2370466360911223, -380.7363362996977116, -304.9990715423533629 ) ) ;
#38603=CARTESIAN_POINT ( 'NONE',  ( 765.0180583372156207, -336.9982390220558273, -360.0135310231089534 ) ) ;
#38606=CARTESIAN_POINT ( 'NONE',  ( 760.7433823573367135, -228.0090635724254753, -355.9930595647440441 ) ) ;
#38610=CARTESIAN_POINT ( 'NONE',  ( 782.5225473063383106, -406.2709662947828519, -375.2698199232970637 ) ) ;
#38615=CARTESIAN_POINT ( 'NONE',  ( 746.8695393053150156, -53.90732993114765037, -327.6429770376306010 ) ) ;
#38616=CARTESIAN_POINT ( 'NONE',  ( 774.6312213355099630, -287.3618753856923718, -364.6798772138717482 ) ) ;
#38621=CARTESIAN_POINT ( 'NONE',  ( 754.3581564841646241, -41.46360902697149697, -316.1443688327762516 ) ) ;
#38622=CARTESIAN_POINT ( 'NONE',  ( 802.7791456095903868, -100.7146871989600356, -329.0155153010375102 ) ) ;
#38629=FACE_OUTER_BOUND ( 'NONE', #19532, .T. ) ;
#38630=CARTESIAN_POINT ( 'NONE',  ( 789.9200121543843807, -97.98741447168734453, -317.0176451133914384 ) ) ;
#38632=CARTESIAN_POINT ( 'NONE',  ( 803.4237431249931660, -63.18005720387488822, -331.2633955100225194 ) ) ;
#38633=CARTESIAN_POINT ( 'NONE',  ( 803.2186876482843445, -391.9874144716864066, -350.0220218866286928 ) ) ;
#38637=CARTESIAN_POINT ( 'NONE',  ( 778.7502325331095108, -384.3510508353227806, -304.6391490659818828 ) ) ;
#38644=VERTEX_POINT ( 'NONE', #40132 ) ;
#38645=CARTESIAN_POINT ( 'NONE',  ( 755.2512626584698410, -247.5436935675106724, -315.2512626584710915 ) ) ;
#38648=CARTESIAN_POINT ( 'NONE',  ( 802.1676090361155502, -230.6346026584197944, -327.8955696845344505 ) ) ;
#38650=CARTESIAN_POINT ( 'NONE',  ( 795.1360043628807261, -356.0891481129647218, -360.2193346964456282 ) ) ;
#38651=CARTESIAN_POINT ( 'NONE',  ( 785.3141322388236176, 2.274488250670355871, -364.4286716492789537 ) ) ;
#38656=CARTESIAN_POINT ( 'NONE',  ( 804.6798772138708955, -15.72551174932958951, -334.6312213355107019 ) ) ;
#38660=ORIENTED_EDGE ( 'NONE', *, *, #12031, .F. ) ;
#38661=CARTESIAN_POINT ( 'NONE',  ( 814.2805881961230625, -265.6454272087889876, -331.2368401574024119 ) ) ;
#38665=CARTESIAN_POINT ( 'NONE',  ( 781.8018195045266339, -238.2709662947833920, -365.1927285166406705 ) ) ;
#38666=CARTESIAN_POINT ( 'NONE',  ( 780.5290396650775619, -396.3510508353228374, -365.2837595273619513 ) ) ;
#38667=FACE_BOUND ( 'NONE', #10596, .T. ) ;
#38669=CARTESIAN_POINT ( 'NONE',  ( 766.0291762391763086, -130.9181544815166660, -360.7704444035551319 ) ) ;
#38672=CARTESIAN_POINT ( 'NONE',  ( 773.7943932421234194, 24.19440371013046231, -305.5313806188329409 ) ) ;
#38673=CARTESIAN_POINT ( 'NONE',  ( 772.5602148656447525, -321.7255117493286320, -305.7998596910095443 ) ) ;
#38676=CARTESIAN_POINT ( 'NONE',  ( 778.2165204200184689, -94.81642084023843609, -364.9363028652563230 ) ) ;
#38679=CARTESIAN_POINT ( 'NONE',  ( 801.9858362298568863, -219.0783235625960401, -312.7379699480935642 ) ) ;
#38681=CARTESIAN_POINT ( 'NONE',  ( 749.2812353651451076, -438.4527844766009821, -323.2262854647983090 ) ) ;
#38687=CARTESIAN_POINT ( 'NONE',  ( 783.0433043558608688, 23.10349461922137237, -315.1538015810313027 ) ) ;
#38694=CARTESIAN_POINT ( 'NONE',  ( 756.7813123517142913, -259.9874144716869182, -329.9779781133712504 ) ) ;
#38696=CARTESIAN_POINT ( 'NONE',  ( 776.2433038121456548, -300.8965053807775689, -374.8207195650711014 ) ) ;
#38701=CARTESIAN_POINT ( 'NONE',  ( 755.0488828828309806, -41.80559628986934229, -344.1219089521771934 ) ) ;
#38702=CARTESIAN_POINT ( 'NONE',  ( 764.8639956371174549, -176.0891481129653755, -319.7806653035542013 ) ) ;
#38703=CARTESIAN_POINT ( 'NONE',  ( 794.9819416627830151, -204.9982390220562820, -319.9864689768909898 ) ) ;
#38705=CARTESIAN_POINT ( 'NONE',  ( 808.0189434323515343, -158.0891481129655176, -319.0252816721025511 ) ) ;
#38706=CARTESIAN_POINT ( 'NONE',  ( 768.0187753319979720, -104.6346026584202207, -318.0580252608186242 ) ) ;
#38708=CARTESIAN_POINT ( 'NONE',  ( 755.1538015810308480, -374.1908817542432075, -343.0433043558613804 ) ) ;
#38718=CARTESIAN_POINT ( 'NONE',  ( 796.1575198192839480, -366.0090635724250774, -359.4546378042384163 ) ) ;
#38719=CARTESIAN_POINT ( 'NONE',  ( 764.8639956371174549, -368.0891481129647786, -319.7806653035542013 ) ) ;
#38720=CARTESIAN_POINT ( 'NONE',  ( 786.2694204179717872, -165.2817908451529547, -305.1769319972829067 ) ) ;
#38724=CARTESIAN_POINT ( 'NONE',  ( 780.5290396650775619, -300.3510508353230080, -365.2837595273619513 ) ) ;
#38725=DIRECTION ( 'NONE',  ( -1.000000000000000000, -0.000000000000000000, -0.000000000000000000 ) ) ;
#38726=CARTESIAN_POINT ( 'NONE',  ( 807.2620300519052989, -168.0090635724256458, -318.0141637701419768 ) ) ;
#38733=CARTESIAN_POINT ( 'NONE',  ( 772.5602148656447525, -201.7255117493290015, -305.7998596910095443 ) ) ;
#38739=CARTESIAN_POINT ( 'NONE',  ( 815.0009284576459549, -102.3510508353236901, -338.7629533639073429 ) ) ;
#38740=CARTESIAN_POINT ( 'NONE',  ( 815.2698199232961542, -328.8164208402375834, -342.5225473063383106 ) ) ;
#38748=CARTESIAN_POINT ( 'NONE',  ( 786.2056067578752163, -371.8055962898682765, -374.4686193811670023 ) ) ;
#38749=CARTESIAN_POINT ( 'NONE',  ( 772.4837098697144029, -143.3618753856927697, -374.5518280994205611 ) ) ;
#38751=CARTESIAN_POINT ( 'NONE',  ( 748.9653473494363425, -410.6346026584191122, -356.9462024416521331 ) ) ;
#38756=CARTESIAN_POINT ( 'NONE',  ( 761.9338519418445230, -182.5328690171416497, -370.4231160770881957 ) ) ;
#38762=CARTESIAN_POINT ( 'NONE',  ( 808.3070685750230950, 5.001760977943074948, -361.1904061080339261 ) ) ;
#38765=CARTESIAN_POINT ( 'NONE',  ( 776.2046728542105711, -428.1908817542430938, -304.8212110874238761 ) ) ;
#38770=CARTESIAN_POINT ( 'NONE',  ( 756.3353852180819104, -245.9073299311469896, -331.1735550268788302 ) ) ;
#38774=CARTESIAN_POINT ( 'NONE',  ( 802.5472867521000353, -244.3726999360617924, -350.8726784830461156 ) ) ;
#38775=CARTESIAN_POINT ( 'NONE',  ( 801.9419747391806368, -258.4527844766016074, -351.9812246680014027 ) ) ;
#38777=CARTESIAN_POINT ( 'NONE',  ( 800.2193346964447755, -114.9982390220565236, -355.1360043628815788 ) ) ;
#38782=PLANE ( 'NONE',  #13778 ) ;
#38783=CARTESIAN_POINT ( 'NONE',  ( 783.7953271457878373, -56.19088175424417386, -375.1787889125761239 ) ) ;
#38792=CARTESIAN_POINT ( 'NONE',  ( 793.9708237608222134, 1.081845518482914104, -319.2295555964448681 ) ) ;
#38793=CARTESIAN_POINT ( 'NONE',  ( 808.3070685750232087, -90.99823902205662307, -361.1904061080339829 ) ) ;
#38795=PLANE ( 'NONE',  #1982 ) ;
#38797=CARTESIAN_POINT ( 'NONE',  ( 759.0252816721024374, -240.9982390220561683, -368.0189434323527280 ) ) ;
#38801=AXIS2_PLACEMENT_3D ( 'NONE', #17869, #24324, #18104 ) ;
#38803=CARTESIAN_POINT ( 'NONE',  ( 746.7653713866222915, -281.2601417444139997, -351.0478386215610271 ) ) ;
#38806=CARTESIAN_POINT ( 'NONE',  ( 814.5518280994195948, -303.7255117493287457, -332.4837098697145734 ) ) ;
#38810=CARTESIAN_POINT ( 'NONE',  ( 756.3353852180819104, -389.9073299311465348, -331.1735550268788302 ) ) ;
#38813=CARTESIAN_POINT ( 'NONE',  ( 744.8212110874229666, -90.89650538077827946, -336.2046728542121627 ) ) ;
#38820=CARTESIAN_POINT ( 'NONE',  ( 800.0135310231082713, -86.08914811296573077, -325.0180583372163028 ) ) ;
#38821=CARTESIAN_POINT ( 'NONE',  ( 759.2295555964440155, -208.1692326535051905, -353.9708237608231229 ) ) ;
#38825=CARTESIAN_POINT ( 'NONE',  ( 778.7502325331095108, -48.35105083532386061, -304.6391490659818828 ) ) ;
#38831=CARTESIAN_POINT ( 'NONE',  ( 797.8822607201568644, -294.5545181178797520, -370.1134526219340160 ) ) ;
#38834=CARTESIAN_POINT ( 'NONE',  ( 755.1538015810308480, -134.1908817542439181, -343.0433043558613804 ) ) ;
#38835=CARTESIAN_POINT ( 'NONE',  ( 804.4286716492782716, -161.3618753856927697, -345.3141322388244703 ) ) ;
#38836=CARTESIAN_POINT ( 'NONE',  ( 774.6312213355098493, -335.3618753856921444, -364.6798772138717482 ) ) ;
#38838=CARTESIAN_POINT ( 'NONE',  ( 803.6646147819161570, -449.9073299311463643, -348.8264449731210561 ) ) ;
#38848=CARTESIAN_POINT ( 'NONE',  ( 788.6739635108323228, -391.6454272087885897, -373.9316612368139090 ) ) ;
#38849=CARTESIAN_POINT ( 'NONE',  ( 800.9747183278959710, 11.00176097794305541, -311.9810565676471583 ) ) ;
#38853=CARTESIAN_POINT ( 'NONE',  ( 802.1676090361156639, -350.6346026584192828, -327.8955696845344505 ) ) ;
#38856=CARTESIAN_POINT ( 'NONE',  ( 761.4292242960306112, -233.4636090269708575, -323.2154366446414429 ) ) ;
#38861=CARTESIAN_POINT ( 'NONE',  ( 745.0891759886404770, -412.2709662947829088, -342.4968714119734159 ) ) ;
#38865=CARTESIAN_POINT ( 'NONE',  ( 810.7187646348534145, -42.45278447660223264, -356.7737145352016341 ) ) ;
#38866=CARTESIAN_POINT ( 'NONE',  ( 771.2633955100217236, -287.9073299311468759, -363.4237431249939618 ) ) ;
#38870=CARTESIAN_POINT ( 'NONE',  ( 781.2370466360911223, -20.73633629969883430, -304.9990715423533629 ) ) ;
#38871=CARTESIAN_POINT ( 'NONE',  ( 802.7791456095903868, -76.71468719896012090, -329.0155153010375102 ) ) ;
#38878=CARTESIAN_POINT ( 'NONE',  ( 800.0135310231082713, -86.08914811296573077, -325.0180583372163028 ) ) ;
#38880=CARTESIAN_POINT ( 'NONE',  ( 754.9735926884551418, -402.3510508353228374, -340.5236548041000333 ) ) ;
#38883=CARTESIAN_POINT ( 'NONE',  ( 807.5423716828161105, -393.0783235625954717, -362.2119215644372048 ) ) ;
#38888=CIRCLE ( 'NONE', #18962, 10.00000000000000888 ) ;
#38891=CARTESIAN_POINT ( 'NONE',  ( 800.9747183278959710, -252.9982390220560831, -311.9810565676471583 ) ) ;
#38894=ORIENTED_EDGE ( 'NONE', *, *, #3815, .T. ) ;
#38896=CARTESIAN_POINT ( 'NONE',  ( 788.7366044899766848, -251.9073299311470748, -316.5762568750059813 ) ) ;
#38898=CARTESIAN_POINT ( 'NONE',  ( 768.0187753319979720, -368.6346026584193964, -318.0580252608186242 ) ) ;
#38899=CARTESIAN_POINT ( 'NONE',  ( 755.0636971347428243, -28.27096629478409540, -341.7834795799807353 ) ) ;
#38900=ADVANCED_FACE ( 'NONE', ( #9787 ), #21101, .T. ) ;
#38905=CARTESIAN_POINT ( 'NONE',  ( 768.0187753319979720, -8.634602658420517329, -318.0580252608186242 ) ) ;
#38909=CARTESIAN_POINT ( 'NONE',  ( 757.7880784355613741, -258.0090635724253616, -312.4576283171834916 ) ) ;
#38913=CARTESIAN_POINT ( 'NONE',  ( 771.2633955100217236, -263.9073299311469327, -363.4237431249939618 ) ) ;
#38914=CARTESIAN_POINT ( 'NONE',  ( 769.1273215169530886, -382.7146871989591546, -317.4527132478988847 ) ) ;
#38916=CARTESIAN_POINT ( 'NONE',  ( 775.8780910478218402, -129.2817908451530400, -364.9511171171680530 ) ) ;
#38920=CARTESIAN_POINT ( 'NONE',  ( 783.7566961878529810, -0.8965053807785533513, -305.1792804349288417 ) ) ;
#38921=CARTESIAN_POINT ( 'NONE',  ( 772.5602148656447525, -297.7255117493286889, -305.7998596910095443 ) ) ;
#38924=CARTESIAN_POINT ( 'NONE',  ( 756.5762568750052424, -75.18005720387485269, -348.7366044899774238 ) ) ;
#38927=CARTESIAN_POINT ( 'NONE',  ( 778.7502325331095108, -192.3510508353233774, -304.6391490659818828 ) ) ;
#38929=CARTESIAN_POINT ( 'NONE',  ( 796.7737145352015204, -428.6346026584192259, -370.7187646348536987 ) ) ;
#38933=CARTESIAN_POINT ( 'NONE',  ( 757.2208543904082489, 7.285312801039605546, -350.9844846989624330 ) ) ;
#38939=CARTESIAN_POINT ( 'NONE',  ( 780.5290396650775619, -300.3510508353230080, -365.2837595273619513 ) ) ;
#38942=CARTESIAN_POINT ( 'NONE',  ( 759.8311093483677041, -286.1692326535048778, -310.9282345327691814 ) ) ;
#38947=CARTESIAN_POINT ( 'NONE',  ( 798.7617431975189675, -51.62377810805111267, -323.0428371773161871 ) ) ;
#38948=CARTESIAN_POINT ( 'NONE',  ( 755.3201227861273992, -171.7255117493291152, -345.3687786644892981 ) ) ;
#38949=CARTESIAN_POINT ( 'NONE',  ( 756.3353852180819104, -221.9073299311470464, -331.1735550268788302 ) ) ;
#38951=CARTESIAN_POINT ( 'NONE',  ( 787.4397851343537695, -141.7255117493291721, -374.2001403089903988 ) ) ;
#38952=ORIENTED_EDGE ( 'NONE', *, *, #34008, .T. ) ;
#38953=CARTESIAN_POINT ( 'NONE',  ( 797.6776695296629214, -139.5436935675110135, -357.6776695296636603 ) ) ;
#38955=CARTESIAN_POINT ( 'NONE',  ( 763.8424801807145741, -402.0090635724250205, -320.5453621957614700 ) ) ;
#38963=CARTESIAN_POINT ( 'NONE',  ( 759.0159684113467620, -400.9181544815159555, -325.8855110935213020 ) ) ;
#38964=CARTESIAN_POINT ( 'NONE',  ( 771.1735550268778070, -369.1800572038739574, -316.3353852180827630 ) ) ;
#38965=CARTESIAN_POINT ( 'NONE',  ( 755.8990559732751535, -155.4636090269711417, -365.9055244015606831 ) ) ;
#38968=LINE ( 'NONE', #24164, #28438 ) ;
#38969=CARTESIAN_POINT ( 'NONE',  ( 775.9200461376533440, -287.8055962898685038, -315.3028492785443291 ) ) ;
#38970=CARTESIAN_POINT ( 'NONE',  ( 799.9999999999993179, 205.0000000000000568, -329.9999999999999432 ) ) ;
#38971=CARTESIAN_POINT ( 'NONE',  ( 752.7379699480933368, -204.0090635724255606, -361.9858362298580232 ) ) ;
#38976=CARTESIAN_POINT ( 'NONE',  ( 763.2262854647970016, -200.6346026584199365, -309.2812353651462445 ) ) ;
#38978=CARTESIAN_POINT ( 'NONE',  ( 804.4286716492782716, 6.638124614306706306, -345.3141322388244703 ) ) ;
#38980=CARTESIAN_POINT ( 'NONE',  ( 766.5853460496234675, -85.98741447168738716, -372.3518521366060554 ) ) ;
#38982=CARTESIAN_POINT ( 'NONE',  ( 810.7187646348534145, -354.4527844766012095, -356.7737145352016341 ) ) ;
#38983=DIRECTION ( 'NONE',  ( 0.000000000000000000, 0.000000000000000000, 1.000000000000000000 ) ) ;
#38987=CARTESIAN_POINT ( 'NONE',  ( 813.2346286133761168, -413.2601417444136018, -328.9521613784389160 ) ) ;
#38988=CARTESIAN_POINT ( 'NONE',  ( 754.9967657858570647, -409.5436935675101040, -365.0032342141425374 ) ) ;
#38992=CARTESIAN_POINT ( 'NONE',  ( 778.7502325331095108, -192.3510508353233774, -304.6391490659818828 ) ) ;
#38998=CARTESIAN_POINT ( 'NONE',  ( 805.0032342141412300, -37.54369356751132614, -314.9967657858571783 ) ) ;
#39001=CARTESIAN_POINT ( 'NONE',  ( 749.5768839229115201, -444.5545181178792973, -358.0661480581553064 ) ) ;
#39005=CARTESIAN_POINT ( 'NONE',  ( 795.1360043628807261, -308.0891481129650629, -360.2193346964456282 ) ) ;
#39009=CARTESIAN_POINT ( 'NONE',  ( 763.8424801807145741, -282.0090635724253048, -320.5453621957614700 ) ) ;
#39010=CARTESIAN_POINT ( 'NONE',  ( 788.8264449731200330, -261.1800572038741848, -363.6646147819171233 ) ) ;
#39012=CARTESIAN_POINT ( 'NONE',  ( 758.0580252608178853, -126.4527844766019626, -328.0187753319985404 ) ) ;
#39016=DIRECTION ( 'NONE',  ( 0.000000000000000000, 0.000000000000000000, 1.000000000000000000 ) ) ;
#39018=CARTESIAN_POINT ( 'NONE',  ( 748.6759233522253680, -64.37269993606231822, -324.3348316497537098 ) ) ;
#39024=CARTESIAN_POINT ( 'NONE',  ( 766.9102291470427417, -18.55451811788065797, -318.6633372737382501 ) ) ;
#39025=CARTESIAN_POINT ( 'NONE',  ( 814.2001403089898304, -113.3618753856929260, -347.4397851343538264 ) ) ;
#39029=CARTESIAN_POINT ( 'NONE',  ( 746.8695393053150156, -221.9073299311470464, -327.6429770376306010 ) ) ;
#39034=CARTESIAN_POINT ( 'NONE',  ( 781.2497674668890113, -300.3510508353230080, -375.3608509340180603 ) ) ;
#39036=CARTESIAN_POINT ( 'NONE',  ( 747.2067596250078623, -315.1800572038740711, -352.2312462859687230 ) ) ;
#39040=CARTESIAN_POINT ( 'NONE',  ( 797.6776695296629214, -403.5436935675101608, -357.6776695296636603 ) ) ;
#39042=CARTESIAN_POINT ( 'NONE',  ( 768.0187753319979720, -200.6346026584199365, -318.0580252608186242 ) ) ;
#39043=CARTESIAN_POINT ( 'NONE',  ( 768.8385539511368734, -71.26014174441469606, -306.4236121716840557 ) ) ;
#39048=CARTESIAN_POINT ( 'NONE',  ( 756.7813123517142913, -187.9874144716870603, -329.9779781133712504 ) ) ;
#39051=CARTESIAN_POINT ( 'NONE',  ( 758.0141637701419768, -39.07832356259662276, -367.2620300519063790 ) ) ;
#39053=CARTESIAN_POINT ( 'NONE',  ( 790.0183182880230106, -452.9681489794449476, -362.9048749981275250 ) ) ;
#39057=CARTESIAN_POINT ( 'NONE',  ( 778.7629533639073998, -344.7363362996978253, -375.0009284576466371 ) ) ;
#39061=CARTESIAN_POINT ( 'NONE',  ( 757.0176451133909268, -157.0999726633347962, -349.9200121543848354 ) ) ;
#39062=CARTESIAN_POINT ( 'NONE',  ( 756.5762568750052424, -147.1800572038746395, -348.7366044899774238 ) ) ;
#39063=CARTESIAN_POINT ( 'NONE',  ( 804.4286716492782716, -353.3618753856922012, -345.3141322388244703 ) ) ;
#39065=CARTESIAN_POINT ( 'NONE',  ( 801.9419747391806368, -450.4527844766009821, -351.9812246680014027 ) ) ;
#39072=EDGE_LOOP ( 'NONE', ( #31251, #3425, #8108, #35343 ) ) ;
#39073=CARTESIAN_POINT ( 'NONE',  ( 745.1792804349281596, -374.1908817542432075, -343.7566961878542884 ) ) ;
#39074=CARTESIAN_POINT ( 'NONE',  ( 814.2001403089898304, 6.638124614306706306, -347.4397851343538264 ) ) ;
#39077=CARTESIAN_POINT ( 'NONE',  ( 778.1981804954714335, -346.2709662947830793, -314.8072714833589885 ) ) ;
#39078=EDGE_CURVE ( 'NONE', #18205, #911, #2925, .T. ) ;
#39081=CARTESIAN_POINT ( 'NONE',  ( 793.9708237608222134, -214.9181544815164386, -319.2295555964448681 ) ) ;
#39084=CARTESIAN_POINT ( 'NONE',  ( 782.5225473063383106, -430.2709662947827383, -375.2698199232970637 ) ) ;
#39087=CARTESIAN_POINT ( 'NONE',  ( 809.7763221938408833, -453.1000272243879863, -336.1997354883953903 ) ) ;
#39089=CARTESIAN_POINT ( 'NONE',  ( 814.2001403089898304, -65.36187538569306810, -347.4397851343538264 ) ) ;
#39090=CARTESIAN_POINT ( 'NONE',  ( 767.8955696845333705, -288.4527844766014937, -362.1676090361162323 ) ) ;
#39094=CARTESIAN_POINT ( 'NONE',  ( 812.3518521366052028, -73.09997266333502353, -326.5853460496235243 ) ) ;
#39095=CARTESIAN_POINT ( 'NONE',  ( 763.2154366446407039, -69.62377810805107003, -321.4292242960311228 ) ) ;
#39098=EDGE_CURVE ( 'NONE', #35055, #29607, #30811, .T. ) ;
#39099=CARTESIAN_POINT ( 'NONE',  ( 785.3687786644884454, 12.63812461430668321, -315.3201227861279676 ) ) ;
#39101=CARTESIAN_POINT ( 'NONE',  ( 762.1405469898971887, -97.54369356751112718, -357.8594530101015607 ) ) ;
#39103=CARTESIAN_POINT ( 'NONE',  ( 783.0433043558608688, -384.8965053807772847, -315.1538015810313027 ) ) ;
#39106=EDGE_LOOP ( 'NONE', ( #35571, #24726, #30614, #32346 ) ) ;
#39107=CARTESIAN_POINT ( 'NONE',  ( 815.0009284576459549, -414.3510508353227237, -338.7629533639073429 ) ) ;
#39113=CARTESIAN_POINT ( 'NONE',  ( 746.8695393053150156, -245.9073299311469896, -327.6429770376306010 ) ) ;
#39118=CARTESIAN_POINT ( 'NONE',  ( 802.5472867521000353, -52.37269993606237506, -350.8726784830461156 ) ) ;
#39119=CARTESIAN_POINT ( 'NONE',  ( 759.7806653035535192, -246.9982390220560831, -324.8639956371181370 ) ) ;
#39120=ORIENTED_EDGE ( 'NONE', *, *, #9907, .F. ) ;
#39121=CARTESIAN_POINT ( 'NONE',  ( 797.8594530101008786, -373.5436935675101040, -322.1405469898980982 ) ) ;
#39122=CARTESIAN_POINT ( 'NONE',  ( 781.7834795799800531, -10.81642084023869543, -315.0636971347436202 ) ) ;
#39127=CARTESIAN_POINT ( 'NONE',  ( 795.1360043628807261, -20.08914811296592973, -360.2193346964456282 ) ) ;
#39130=EDGE_LOOP ( 'NONE', ( #28529, #9041 ) ) ;
#39131=CARTESIAN_POINT ( 'NONE',  ( 757.7880784355613741, -282.0090635724253048, -312.4576283171834916 ) ) ;
#39135=CARTESIAN_POINT ( 'NONE',  ( 758.0580252608178853, -270.4527844766014937, -328.0187753319985404 ) ) ;
#39138=CARTESIAN_POINT ( 'NONE',  ( 793.9708237608222134, -118.9181544815167229, -319.2295555964448681 ) ) ;
#39140=CARTESIAN_POINT ( 'NONE',  ( 788.4001350590139054, -443.1233509495419298, -363.5803521658918385 ) ) ;
#39141=CARTESIAN_POINT ( 'NONE',  ( 810.7187646348534145, -306.4527844766013800, -356.7737145352016341 ) ) ;
#39145=CARTESIAN_POINT ( 'NONE',  ( 815.1787889125755555, -198.8965053807779384, -343.7953271457877804 ) ) ;
#39147=CARTESIAN_POINT ( 'NONE',  ( 814.2001403089898304, -449.3618753856918602, -347.4397851343538264 ) ) ;
#39152=CARTESIAN_POINT ( 'NONE',  ( 801.9419747391806368, -450.4527844766009821, -351.9812246680014027 ) ) ;
#39154=EDGE_CURVE ( 'NONE', #31261, #29612, #43256, .T. ) ;
#39159=CARTESIAN_POINT ( 'NONE',  ( 802.1676090361156639, -38.63460265842041252, -327.8955696845344505 ) ) ;
#39160=ADVANCED_FACE ( 'NONE', ( #304 ), #43026, .F. ) ;
#39161=CARTESIAN_POINT ( 'NONE',  ( 756.7813123517142913, -283.9874144716867477, -329.9779781133712504 ) ) ;
#39163=CARTESIAN_POINT ( 'NONE',  ( 808.7758568127978833, -292.1692326535048210, -320.0363995740631822 ) ) ;
#39168=CARTESIAN_POINT ( 'NONE',  ( 755.8398074228967971, -91.44195992623282621, -333.4516893846970333 ) ) ;
#39169=CARTESIAN_POINT ( 'NONE',  ( 759.7806653035534055, -150.9982390220563957, -324.8639956371180801 ) ) ;
#39170=CARTESIAN_POINT ( 'NONE',  ( 788.7366044899766848, -203.9073299311471885, -316.5762568750059813 ) ) ;
#39173=CARTESIAN_POINT ( 'NONE',  ( 767.6429770376289525, -153.1800572038746395, -306.8695393053162093 ) ) ;
#39175=CARTESIAN_POINT ( 'NONE',  ( 755.0636971347428243, -148.2709662947837330, -341.7834795799807353 ) ) ;
#39176=ORIENTED_EDGE ( 'NONE', *, *, #29090, .T. ) ;
#39177=CARTESIAN_POINT ( 'NONE',  ( 787.5531968255692163, -405.8272453906067199, -316.1348686366205811 ) ) ;
#39184=CARTESIAN_POINT ( 'NONE',  ( 773.4516893846965786, -403.6454272087884760, -315.8398074228977066 ) ) ;
#39186=CARTESIAN_POINT ( 'NONE',  ( 745.5313806188320314, -183.2817908451528695, -333.7943932421247268 ) ) ;
#39189=DIRECTION ( 'NONE',  ( 1.000000000000000000, 0.000000000000000000, 0.000000000000000000 ) ) ;
#39190=CARTESIAN_POINT ( 'NONE',  ( 755.0488828828309806, -305.8055962898684470, -344.1219089521771934 ) ) ;
#39191=CARTESIAN_POINT ( 'NONE',  ( 757.8323909638827445, -434.6346026584190554, -352.1044303154654358 ) ) ;
#39192=CARTESIAN_POINT ( 'NONE',  ( 773.7305795820266212, -177.2817908451528695, -374.8230680027170365 ) ) ;
#39193=CARTESIAN_POINT ( 'NONE',  ( 759.9999999999992042, -512.9681489794448908, -309.9999999999998863 ) ) ;
#39197=CARTESIAN_POINT ( 'NONE',  ( 745.0891759886404770, -220.2709662947834772, -342.4968714119734159 ) ) ;
#39198=FACE_OUTER_BOUND ( 'NONE', #39072, .T. ) ;
#39199=DIRECTION ( 'NONE',  ( 0.000000000000000000, 0.000000000000000000, -1.000000000000000000 ) ) ;
#39201=CARTESIAN_POINT ( 'NONE',  ( 793.4146539503750546, -97.98741447168734453, -307.6481478633938877 ) ) ;
#39203=CARTESIAN_POINT ( 'NONE',  ( 744.7301800767019131, -340.8164208402376971, -337.4774526936615757 ) ) ;
#39208=CARTESIAN_POINT ( 'NONE',  ( 778.7502325331095108, -408.3510508353227806, -304.6391490659818828 ) ) ;
#39209=CARTESIAN_POINT ( 'NONE',  ( 787.4397851343537695, -429.7255117493282910, -374.2001403089903988 ) ) ;
#39214=CARTESIAN_POINT ( 'NONE',  ( 815.0009284576459549, -198.3510508353234059, -338.7629533639073429 ) ) ;
#39220=CARTESIAN_POINT ( 'NONE',  ( 814.9108240113580450, -40.27096629478405987, -337.5031285880265273 ) ) ;
#39223=CARTESIAN_POINT ( 'NONE',  ( 786.2694204179717872, -453.2817908451519315, -305.1769319972829067 ) ) ;
#39227=CARTESIAN_POINT ( 'NONE',  ( 767.8955696845333705, -288.4527844766014937, -362.1676090361162323 ) ) ;
#39231=CARTESIAN_POINT ( 'NONE',  ( 766.0291762391763086, -274.9181544815161828, -360.7704444035551319 ) ) ;
#39232=CARTESIAN_POINT ( 'NONE',  ( 800.0135310231082713, -278.0891481129651197, -325.0180583372163028 ) ) ;
#39233=CARTESIAN_POINT ( 'NONE',  ( 759.7806653035535192, -438.9982390220554294, -324.8639956371181370 ) ) ;
#39234=CARTESIAN_POINT ( 'NONE',  ( 794.9819416627830151, -132.9982390220564810, -319.9864689768909898 ) ) ;
#39239=CARTESIAN_POINT ( 'NONE',  ( 811.3240766477731540, -76.37269993606228979, -355.6651683502462902 ) ) ;
#39245=CARTESIAN_POINT ( 'NONE',  ( 796.9571628226829034, -47.46360902697148987, -321.2382568024804641 ) ) ;
#39247=CARTESIAN_POINT ( 'NONE',  ( 759.0252816721024374, -96.99823902205660886, -368.0189434323527280 ) ) ;
#39251=CARTESIAN_POINT ( 'NONE',  ( 792.2312462859673587, -227.9073299311471033, -307.2067596250082602 ) ) ;
#39254=CARTESIAN_POINT ( 'NONE',  ( 744.9990715423526808, -306.3510508353230648, -341.2370466360926002 ) ) ;
#39256=CARTESIAN_POINT ( 'NONE',  ( 751.6929314249748586, -318.9982390220557704, -318.8095938919659034 ) ) ;
#39259=CARTESIAN_POINT ( 'NONE',  ( 791.9812246680005501, -428.6346026584192259, -361.9419747391813189 ) ) ;
#39261=CARTESIAN_POINT ( 'NONE',  ( 751.2241431872005251, -88.16923265350555994, -359.9636004259367610 ) ) ;
#39264=VERTEX_POINT ( 'NONE', #28240 ) ;
#39265=CARTESIAN_POINT ( 'NONE',  ( 757.2208543904082489, -184.7146871989598083, -350.9844846989624330 ) ) ;
#39267=CARTESIAN_POINT ( 'NONE',  ( 815.1787889125755555, -30.89650538077846065, -343.7953271457877804 ) ) ;
#39269=AXIS2_PLACEMENT_3D ( 'NONE', #8221, #22290, #36386 ) ;
#39270=CARTESIAN_POINT ( 'NONE',  ( 808.5285127195401174, -452.9681489794448339, -336.5948204574517035 ) ) ;
#39274=CARTESIAN_POINT ( 'NONE',  ( 804.1009440267234822, -335.4636090269705733, -314.0944755984392600 ) ) ;
#39278=CARTESIAN_POINT ( 'NONE',  ( 800.9840315886518738, -196.9181544815164386, -354.1144889064786412 ) ) ;
#39279=CARTESIAN_POINT ( 'NONE',  ( 795.1360043628807261, -164.0891481129655176, -360.2193346964456282 ) ) ;
#39280=CARTESIAN_POINT ( 'NONE',  ( 801.9419747391806368, -354.4527844766012095, -351.9812246680014027 ) ) ;
#39282=CARTESIAN_POINT ( 'NONE',  ( 761.2382568024794409, 8.376221891948691933, -356.9571628226838129 ) ) ;
#39290=CARTESIAN_POINT ( 'NONE',  ( 757.7880784355613741, -402.0090635724250205, -312.4576283171834916 ) ) ;
#39292=CARTESIAN_POINT ( 'NONE',  ( 745.4481719005789273, -3.725511749329622813, -347.5162901302853697 ) ) ;
#39295=CARTESIAN_POINT ( 'NONE',  ( 774.6312213355099630, -359.3618753856920875, -364.6798772138717482 ) ) ;
#39298=CARTESIAN_POINT ( 'NONE',  ( 783.0745993439762742, -224.1908817542436623, -365.1016975059196739 ) ) ;
#39303=CARTESIAN_POINT ( 'NONE',  ( 810.7187646348534145, -450.4527844766009821, -356.7737145352016341 ) ) ;
#39308=CARTESIAN_POINT ( 'NONE',  ( 754.9967657858570647, -73.54369356751118403, -365.0032342141425374 ) ) ;
#39310=CARTESIAN_POINT ( 'NONE',  ( 756.3353852180819104, -269.9073299311468190, -331.1735550268788302 ) ) ;
#39313=CARTESIAN_POINT ( 'NONE',  ( 809.0717654672305343, -76.91815448151683654, -360.1688906516309885 ) ) ;
#39314=CARTESIAN_POINT ( 'NONE',  ( 755.8398074228967971, -91.44195992623282621, -333.4516893846970333 ) ) ;
#39318=CARTESIAN_POINT ( 'NONE',  ( 768.0187753319979720, 15.36539734157940629, -318.0580252608186242 ) ) ;
#39319=CARTESIAN_POINT ( 'NONE',  ( 787.6308680596127942, -107.2601417444145824, -364.1105419155492768 ) ) ;
#39321=CARTESIAN_POINT ( 'NONE',  ( 758.0580252608178853, -102.4527844766020337, -328.0187753319985404 ) ) ;
#39322=CARTESIAN_POINT ( 'NONE',  ( 805.0264073115434940, -414.3510508353227237, -339.4763451958999099 ) ) ;
#39326=CARTESIAN_POINT ( 'NONE',  ( 759.8311093483677041, -406.1692326535045368, -310.9282345327691814 ) ) ;
#39330=CARTESIAN_POINT ( 'NONE',  ( 755.2512626584698410, -247.5436935675106724, -315.2512626584710915 ) ) ;
#39332=CARTESIAN_POINT ( 'NONE',  ( 763.0537975583475827, -264.4527844766016074, -371.0346526505627480 ) ) ;
#39337=CARTESIAN_POINT ( 'NONE',  ( 755.3028492785439312, -87.28179084515316788, -335.9200461376539693 ) ) ;
#39339=CARTESIAN_POINT ( 'NONE',  ( 792.1044303154646968, -252.4527844766015789, -317.8323909638837677 ) ) ;
#39341=CARTESIAN_POINT ( 'NONE',  ( 755.5713283507202505, -389.3618753856919739, -334.6858677611754729 ) ) ;
#39342=CARTESIAN_POINT ( 'NONE',  ( 785.3687786644884454, -59.36187538569306810, -315.3201227861279676 ) ) ;
#39347=CARTESIAN_POINT ( 'NONE',  ( 792.1044303154645831, -12.45278447660232146, -317.8323909638837677 ) ) ;
#39351=CARTESIAN_POINT ( 'NONE',  ( 804.1009440267234822, -287.4636090269708575, -314.0944755984392600 ) ) ;
#39354=CARTESIAN_POINT ( 'NONE',  ( 785.3687786644884454, -251.3618753856923149, -315.3201227861279676 ) ) ;
#39355=CARTESIAN_POINT ( 'NONE',  ( 787.5531968255692163, -117.8272453906076151, -316.1348686366205811 ) ) ;
#39360=CARTESIAN_POINT ( 'NONE',  ( 787.5162901302840055, -323.3618753856922581, -305.4481719005793252 ) ) ;
#39365=CARTESIAN_POINT ( 'NONE',  ( 756.1443688327750579, -213.6237781080506011, -314.3581564841659315 ) ) ;
#39367=CARTESIAN_POINT ( 'NONE',  ( 771.3260364891663130, 4.354572791210176597, -306.0683387631859773 ) ) ;
#39373=CARTESIAN_POINT ( 'NONE',  ( 797.6776695296629214, -451.5436935675099903, -357.6776695296636603 ) ) ;
#39380=CARTESIAN_POINT ( 'NONE',  ( 788.7366044899766848, -35.90732993114770011, -316.5762568750059813 ) ) ;
#39381=CARTESIAN_POINT ( 'NONE',  ( 775.9200461376533440, -287.8055962898685038, -315.3028492785443291 ) ) ;
#39382=UNCERTAINTY_MEASURE_WITH_UNIT (LENGTH_MEASURE( 1.000000000000000082E-05 ), #6539, 'distance_accuracy_value', 'NONE');
#39384=CARTESIAN_POINT ( 'NONE',  ( 764.3348316497523456, -310.7146871989593251, -308.6759233522265617 ) ) ;
#39388=ORIENTED_EDGE ( 'NONE', *, *, #13125, .F. ) ;
#39391=CARTESIAN_POINT ( 'NONE',  ( 803.8651313633788504, -77.26014174441466764, -332.4468031744301015 ) ) ;
#39393=CARTESIAN_POINT ( 'NONE',  ( 811.0346526505616112, -158.6346026584199933, -323.0537975583477532 ) ) ;
#39397=CARTESIAN_POINT ( 'NONE',  ( 792.1044303154646968, -156.4527844766018916, -317.8323909638837677 ) ) ;
#39399=CARTESIAN_POINT ( 'NONE',  ( 802.5472867521000353, -412.3726999360612808, -350.8726784830461156 ) ) ;
#39403=FACE_OUTER_BOUND ( 'NONE', #12777, .T. ) ;
#39407=CARTESIAN_POINT ( 'NONE',  ( 786.5483106153019435, -391.6454272087885897, -364.1601925771022366 ) ) ;
#39409=CARTESIAN_POINT ( 'NONE',  ( 807.2620300519052989, -168.0090635724256458, -318.0141637701419768 ) ) ;
#39415=CARTESIAN_POINT ( 'NONE',  ( 790.8726784830453198, -322.7146871989593819, -362.5472867521010585 ) ) ;
#39416=CARTESIAN_POINT ( 'NONE',  ( 759.7806653035534055, -438.9982390220553157, -324.8639956371180801 ) ) ;
#39417=CARTESIAN_POINT ( 'NONE',  ( 783.7953271457878373, -176.1908817542438328, -375.1787889125761239 ) ) ;
#39423=CARTESIAN_POINT ( 'NONE',  ( 800.9747183278959710, -204.9982390220562820, -311.9810565676471583 ) ) ;
#39425=CARTESIAN_POINT ( 'NONE',  ( 759.7806653035534055, -30.99823902205680071, -324.8639956371180801 ) ) ;
#39427=CARTESIAN_POINT ( 'NONE',  ( 803.8556311672234642, -105.6237781080509421, -365.6418435158340117 ) ) ;
#39429=CARTESIAN_POINT ( 'NONE',  ( 755.2512626584698410, -343.5436935675103314, -315.2512626584710915 ) ) ;
#39438=CARTESIAN_POINT ( 'NONE',  ( 795.6651683502461765, -394.7146871989591546, -371.3240766477733814 ) ) ;
#39439=CARTESIAN_POINT ( 'NONE',  ( 792.3570229623688874, -405.1800572038737300, -373.1304606946836202 ) ) ;
#39443=CARTESIAN_POINT ( 'NONE',  ( 756.7813123517142913, -187.9874144716870603, -329.9779781133712504 ) ) ;
#39444=CARTESIAN_POINT ( 'NONE',  ( 771.2633955100217236, -119.9073299311474443, -363.4237431249939618 ) ) ;
#39446=CARTESIAN_POINT ( 'NONE',  ( 766.5853460496234675, -205.9874144716870035, -372.3518521366060554 ) ) ;
#39453=CARTESIAN_POINT ( 'NONE',  ( 747.2067596250078623, -51.18005720387493085, -352.2312462859687230 ) ) ;
#39456=CARTESIAN_POINT ( 'NONE',  ( 811.3240766477731540, -460.3726999360611103, -355.6651683502462902 ) ) ;
#39461=CARTESIAN_POINT ( 'NONE',  ( 797.6776695296629214, -283.5436935675105019, -357.6776695296636603 ) ) ;
#39464=CARTESIAN_POINT ( 'NONE',  ( 793.9708237608222134, -286.9181544815161828, -319.2295555964448681 ) ) ;
#39465=CARTESIAN_POINT ( 'NONE',  ( 785.3687786644884454, -275.3618753856923149, -315.3201227861279676 ) ) ;
#39467=CARTESIAN_POINT ( 'NONE',  ( 803.4237431249931660, -111.1800572038747532, -331.2633955100225194 ) ) ;
#39476=CARTESIAN_POINT ( 'NONE',  ( 815.3608509340175488, -74.73633629969866377, -341.2497674668889545 ) ) ;
#39482=CARTESIAN_POINT ( 'NONE',  ( 763.0428371773158460, -35.46360902697151829, -358.7617431975195359 ) ) ;
#39487=CARTESIAN_POINT ( 'NONE',  ( 758.8095938919642549, -248.0891481129651481, -311.6929314249763365 ) ) ;
#39490=AXIS2_PLACEMENT_3D ( 'NONE', #37052, #41609, #5404 ) ;
#39494=CARTESIAN_POINT ( 'NONE',  ( 811.6461892240364477, -292.7146871989594956, -324.1737431748509835 ) ) ;
#39496=CARTESIAN_POINT ( 'NONE',  ( 800.9747183278959710, -300.9982390220559409, -311.9810565676471583 ) ) ;
#39500=CARTESIAN_POINT ( 'NONE',  ( 800.0135310231082713, -422.0891481129647218, -325.0180583372163028 ) ) ;
#39503=CARTESIAN_POINT ( 'NONE',  ( 757.8323909638827445, -194.6346026584198796, -352.1044303154654358 ) ) ;
#39505=CARTESIAN_POINT ( 'NONE',  ( 788.7631598425961101, -73.44195992623286884, -305.7194118038759143 ) ) ;
#39510=CARTESIAN_POINT ( 'NONE',  ( 805.1016975059191054, -246.8965053807777679, -343.0745993439771837 ) ) ;
#39512=CARTESIAN_POINT ( 'NONE',  ( 746.0683387631852383, -43.44195992623296831, -331.3260364891676204 ) ) ;
#39515=CARTESIAN_POINT ( 'NONE',  ( 795.1526350630804245, -452.9681489794450044, -359.9976132353968410 ) ) ;
#39519=CARTESIAN_POINT ( 'NONE',  ( 809.0717654672305343, -340.9181544815160123, -360.1688906516309885 ) ) ;
#39524=CARTESIAN_POINT ( 'NONE',  ( 757.0176451133909268, -181.0999726633347109, -349.9200121543848354 ) ) ;
#39525=CARTESIAN_POINT ( 'NONE',  ( 797.6776695296629214, -187.5436935675108430, -357.6776695296636603 ) ) ;
#39526=CARTESIAN_POINT ( 'NONE',  ( 791.9812246680005501, -332.6346026584195101, -361.9419747391813189 ) ) ;
#39528=CARTESIAN_POINT ( 'NONE',  ( 786.6156483768007774, 22.55804007376682918, -315.5913626894246136 ) ) ;
#39536=CARTESIAN_POINT ( 'NONE',  ( 747.6481478633932056, -397.0999726633340288, -353.4146539503763620 ) ) ;
#39538=CARTESIAN_POINT ( 'NONE',  ( 814.9108240113580450, 7.729033705215793582, -337.5031285880265273 ) ) ;
#39542=CARTESIAN_POINT ( 'NONE',  ( 788.7366044899766848, -347.9073299311467053, -316.5762568750059813 ) ) ;
#39546=CARTESIAN_POINT ( 'NONE',  ( 775.8780910478218402, -249.2817908451526421, -364.9511171171680530 ) ) ;
#39557=CARTESIAN_POINT ( 'NONE',  ( 801.9419747391806368, -306.4527844766013800, -351.9812246680014027 ) ) ;
#39561=CARTESIAN_POINT ( 'NONE',  ( 760.0363995740630116, -58.91815448151690759, -368.7758568127991907 ) ) ;
#39562=CARTESIAN_POINT ( 'NONE',  ( 766.7756240680305382, -86.53286901714194812, -361.5560724626415663 ) ) ;
#39566=CARTESIAN_POINT ( 'NONE',  ( 788.7366044899766848, 12.09267006885214180, -316.5762568750059813 ) ) ;
#39567=CARTESIAN_POINT ( 'NONE',  ( 756.1348686366196716, -137.2601417444144829, -347.5531968255698416 ) ) ;
#39569=CARTESIAN_POINT ( 'NONE',  ( 792.1044303154645831, -108.4527844766019911, -317.8323909638837677 ) ) ;
#39570=CARTESIAN_POINT ( 'NONE',  ( 801.3366627262608972, -392.5328690171409107, -353.0897708529566899 ) ) ;
#39580=ORIENTED_EDGE ( 'NONE', *, *, #8079, .T. ) ;
#39581=CARTESIAN_POINT ( 'NONE',  ( 769.9779781133707957, -91.09997266333496668, -316.7813123517150871 ) ) ;
#39583=CARTESIAN_POINT ( 'NONE',  ( 785.3687786644885591, -251.3618753856923718, -315.3201227861280813 ) ) ;
#39586=CARTESIAN_POINT ( 'NONE',  ( 788.7366044899766848, -395.9073299311465348, -316.5762568750059813 ) ) ;
#39587=CARTESIAN_POINT ( 'NONE',  ( 762.3223304703356007, -55.54369356751127640, -322.3223304703362828 ) ) ;
#39592=CARTESIAN_POINT ( 'NONE',  ( 791.9812246680005501, -20.63460265842048003, -361.9419747391813189 ) ) ;
#39595=CARTESIAN_POINT ( 'NONE',  ( 744.6391490659812007, -302.7363362996979959, -338.7502325331110455 ) ) ;
#39598=CARTESIAN_POINT ( 'NONE',  ( 757.8323909638827445, -266.6346026584197375, -352.1044303154654358 ) ) ;
#39600=CARTESIAN_POINT ( 'NONE',  ( 799.2566176426618085, -144.0090635724257027, -324.0069404352559559 ) ) ;
#39602=CARTESIAN_POINT ( 'NONE',  ( 761.9338519418445230, -14.53286901714214707, -370.4231160770881957 ) ) ;
#39603=CARTESIAN_POINT ( 'NONE',  ( 805.0032342141413437, -349.5436935675103314, -314.9967657858572352 ) ) ;
#39607=CARTESIAN_POINT ( 'NONE',  ( 803.8556311672234642, -249.6237781080505158, -365.6418435158340117 ) ) ;
#39609=CARTESIAN_POINT ( 'NONE',  ( 756.1443688327750579, -429.6237781080499190, -314.3581564841659315 ) ) ;
#39616=CARTESIAN_POINT ( 'NONE',  ( 802.7791456095903868, 19.28531280103956647, -329.0155153010375102 ) ) ;
#39623=CIRCLE ( 'NONE', #30762, 20.00000000000001776 ) ;
#39624=CARTESIAN_POINT ( 'NONE',  ( 759.2295555964440155, -304.1692326535048210, -353.9708237608231229 ) ) ;
#39626=CARTESIAN_POINT ( 'NONE',  ( 783.7566961878529810, -312.8965053807775689, -305.1792804349288417 ) ) ;
#39627=DIRECTION ( 'NONE',  ( 0.000000000000000000, 0.000000000000000000, -1.000000000000000000 ) ) ;
#39631=CARTESIAN_POINT ( 'NONE',  ( 763.2154366446407039, -93.62377810805098477, -321.4292242960311228 ) ) ;
#39634=CARTESIAN_POINT ( 'NONE',  ( 792.2312462859673587, -131.9073299311473875, -307.2067596250082602 ) ) ;
#39636=CARTESIAN_POINT ( 'NONE',  ( 768.0187753319979720, -128.6346026584201354, -318.0580252608186242 ) ) ;
#39637=ORIENTED_EDGE ( 'NONE', *, *, #38258, .F. ) ;
#39639=CARTESIAN_POINT ( 'NONE',  ( 755.5913626894240451, -421.6454272087885329, -346.6156483768012890 ) ) ;
#39648=CARTESIAN_POINT ( 'NONE',  ( 757.0176451133909268, -397.0999726633340288, -349.9200121543848354 ) ) ;
#39650=CARTESIAN_POINT ( 'NONE',  ( 807.2620300519052989, -216.0090635724255037, -318.0141637701419768 ) ) ;
#39655=CARTESIAN_POINT ( 'NONE',  ( 756.7813123517142913, -331.9874144716865203, -329.9779781133712504 ) ) ;
#39657=CARTESIAN_POINT ( 'NONE',  ( 814.2805881961230625, -193.6454272087891582, -331.2368401574024119 ) ) ;
#39659=DIRECTION ( 'NONE',  ( 0.7071067811865753283, 0.000000000000000000, -0.7071067811865198172 ) ) ;
#39662=CARTESIAN_POINT ( 'NONE',  ( 796.9462024416508257, -228.4527844766016074, -308.9653473494370246 ) ) ;
#39665=CARTESIAN_POINT ( 'NONE',  ( 804.6798772138708955, -15.72551174932958951, -334.6312213355107019 ) ) ;
#39668=CARTESIAN_POINT ( 'NONE',  ( 748.3538107759620743, -88.71468719896009247, -355.8262568251490165 ) ) ;
#39670=CARTESIAN_POINT ( 'NONE',  ( 745.0891759886404770, -388.2709662947829656, -342.4968714119734159 ) ) ;
#39676=CARTESIAN_POINT ( 'NONE',  ( 781.2497674668890113, -420.3510508353225532, -375.3608509340180603 ) ) ;
#39677=CARTESIAN_POINT ( 'NONE',  ( 771.3260364891663130, 4.354572791210176597, -306.0683387631859773 ) ) ;
#39682=CARTESIAN_POINT ( 'NONE',  ( 761.2382568024794409, -183.6237781080507148, -356.9571628226838129 ) ) ;
#39684=CARTESIAN_POINT ( 'NONE',  ( 803.8556311672234642, -201.6237781080506863, -365.6418435158340117 ) ) ;
#39691=CARTESIAN_POINT ( 'NONE',  ( 756.3353852180819104, -149.9073299311473875, -331.1735550268788302 ) ) ;
#39694=CARTESIAN_POINT ( 'NONE',  ( 749.2812353651451076, -54.45278447660219001, -323.2262854647983090 ) ) ;
#39696=CARTESIAN_POINT ( 'NONE',  ( 783.7953271457878373, -440.1908817542430370, -375.1787889125761239 ) ) ;
#39698=CARTESIAN_POINT ( 'NONE',  ( 758.4439275373578084, -324.5545181178796952, -353.2243759319684386 ) ) ;
#39701=CARTESIAN_POINT ( 'NONE',  ( 765.0180583372156207, -288.9982390220559978, -360.0135310231089534 ) ) ;
#39705=CARTESIAN_POINT ( 'NONE',  ( 802.9823548866075953, -289.0999726633343698, -330.0799878456151077 ) ) ;
#39706=CARTESIAN_POINT ( 'NONE',  ( 757.8323909638827445, -290.6346026584195101, -352.1044303154654358 ) ) ;
#39708=CARTESIAN_POINT ( 'NONE',  ( 774.6312213355099630, -167.3618753856927412, -364.6798772138717482 ) ) ;
#39714=CARTESIAN_POINT ( 'NONE',  ( 744.6391490659812007, -86.73633629969862113, -338.7502325331110455 ) ) ;
#39719=ORIENTED_EDGE ( 'NONE', *, *, #20624, .T. ) ;
#39720=CARTESIAN_POINT ( 'NONE',  ( 754.9967657858570647, -97.54369356751114140, -365.0032342141425943 ) ) ;
#39726=CARTESIAN_POINT ( 'NONE',  ( 814.9108240113580450, -232.2709662947834488, -337.5031285880265273 ) ) ;
#39730=CARTESIAN_POINT ( 'NONE',  ( 776.2433038121456548, -300.8965053807775689, -374.8207195650711014 ) ) ;
#39732=CARTESIAN_POINT ( 'NONE',  ( 777.4774526936600978, -322.2709662947830225, -304.7301800767027657 ) ) ;
#39736=CARTESIAN_POINT ( 'NONE',  ( 797.6776695296629214, -427.5436935675101040, -357.6776695296636603 ) ) ;
#39737=CARTESIAN_POINT ( 'NONE',  ( 788.7366044899766848, -227.9073299311471033, -316.5762568750059813 ) ) ;
#39738=CARTESIAN_POINT ( 'NONE',  ( 801.9858362298568863, -99.07832356259642381, -312.7379699480935642 ) ) ;
#39743=VERTEX_POINT ( 'NONE', #12071 ) ;
#39744=CARTESIAN_POINT ( 'NONE',  ( 805.1016975059191054, -222.8965053807778531, -343.0745993439771837 ) ) ;
#39747=CARTESIAN_POINT ( 'NONE',  ( 783.7566961878529810, -72.89650538077830788, -305.1792804349288417 ) ) ;
#39750=CARTESIAN_POINT ( 'NONE',  ( 795.8262568251477660, -358.3726999360613945, -308.3538107759623585 ) ) ;
#39756=CARTESIAN_POINT ( 'NONE',  ( 799.2566176426618085, -168.0090635724256458, -324.0069404352559559 ) ) ;
#39757=CARTESIAN_POINT ( 'NONE',  ( 758.0580252608178853, -198.4527844766017495, -328.0187753319985404 ) ) ;
#39758=CARTESIAN_POINT ( 'NONE',  ( 767.8955696845334842, -384.4527844766011526, -362.1676090361161755 ) ) ;
#39760=CARTESIAN_POINT ( 'NONE',  ( 799.4546378042377910, 14.92167643740321381, -356.1575198192848006 ) ) ;
#39769=CARTESIAN_POINT ( 'NONE',  ( 813.5763878283155464, -411.8272453906067199, -351.1614460488615350 ) ) ;
#39770=CARTESIAN_POINT ( 'NONE',  ( 772.5602148656447525, 14.27448825067031812, -305.7998596910095443 ) ) ;
#39773=CARTESIAN_POINT ( 'NONE',  ( 803.4237431249931660, -375.1800572038739574, -331.2633955100225194 ) ) ;
#39777=CARTESIAN_POINT ( 'NONE',  ( 776.9254006560222479, -260.1908817542435486, -314.8983024940802125 ) ) ;
#39781=CIRCLE ( 'NONE', #5068, 4.999999999999984901 ) ;
#39785=CARTESIAN_POINT ( 'NONE',  ( 794.9819416627830151, -300.9982390220559409, -319.9864689768909898 ) ) ;
#39789=CARTESIAN_POINT ( 'NONE',  ( 809.0717654672305343, -52.91815448151692891, -360.1688906516309885 ) ) ;
#39790=CARTESIAN_POINT ( 'NONE',  ( 805.0264073115434940, -126.3510508353236048, -339.4763451958999099 ) ) ;
#39794=CARTESIAN_POINT ( 'NONE',  ( 788.8264449731200330, -45.18005720387493085, -363.6646147819171233 ) ) ;
#39795=CARTESIAN_POINT ( 'NONE',  ( 804.9511171171677688, -125.8055962898690581, -335.8780910478229202 ) ) ;
#39796=CARTESIAN_POINT ( 'NONE',  ( 805.1927285166397041, -112.8164208402383508, -341.8018195045277707 ) ) ;
#39797=CARTESIAN_POINT ( 'NONE',  ( 796.7845633553578182, -417.6237781080499190, -358.5707757039688204 ) ) ;
#39808=CARTESIAN_POINT ( 'NONE',  ( 804.6971507214547046, -75.28179084515321051, -344.0799538623459739 ) ) ;
#39810=CARTESIAN_POINT ( 'NONE',  ( 803.4237431249931660, -279.1800572038741848, -331.2633955100225194 ) ) ;
#39813=CARTESIAN_POINT ( 'NONE',  ( 791.9812246680005501, -404.6346026584193396, -361.9419747391813189 ) ) ;
#39814=CARTESIAN_POINT ( 'NONE',  ( 800.0135310231082713, -62.08914811296580183, -325.0180583372163028 ) ) ;
#39816=CARTESIAN_POINT ( 'NONE',  ( 779.9999999999992042, -452.9681489794448339, -339.9999999999999432 ) ) ;
#39818=CARTESIAN_POINT ( 'NONE',  ( 799.9636004259356241, -22.91815448151701062, -311.2241431872006956 ) ) ;
#39821=CARTESIAN_POINT ( 'NONE',  ( 811.3240766477731540, -316.3726999360615082, -355.6651683502462902 ) ) ;
#39824=CARTESIAN_POINT ( 'NONE',  ( 757.8323909638827445, -242.6346026584197659, -352.1044303154654358 ) ) ;
#39827=CARTESIAN_POINT ( 'NONE',  ( 754.7162404726377645, -134.7363362996984790, -339.4709603349214717 ) ) ;
#39830=CARTESIAN_POINT ( 'NONE',  ( 778.7502325331095108, -24.35105083532392811, -304.6391490659818828 ) ) ;
#39831=CARTESIAN_POINT ( 'NONE',  ( 812.7932403749906598, -351.1800572038740142, -327.7687537140311633 ) ) ;
#39836=CARTESIAN_POINT ( 'NONE',  ( 798.0661480581538854, -242.5328690171414507, -309.5768839229118043 ) ) ;
#39838=CARTESIAN_POINT ( 'NONE',  ( 805.0032342141412300, 10.45630643248850866, -314.9967657858571783 ) ) ;
#39843=CARTESIAN_POINT ( 'NONE',  ( 805.0264073115434940, -30.35105083532391390, -339.4763451958999099 ) ) ;
#39849=CARTESIAN_POINT ( 'NONE',  ( 787.6308680596127942, -299.2601417444139997, -364.1105419155492768 ) ) ;
#39852=CARTESIAN_POINT ( 'NONE',  ( 813.9316612368132837, -319.4419599262320730, -348.6739635108323228 ) ) ;
#39853=CARTESIAN_POINT ( 'NONE',  ( 791.7608162188021197, 205.0000000000000568, -339.9999999999999432 ) ) ;
#39857=CARTESIAN_POINT ( 'NONE',  ( 763.2154366446407039, -69.62377810805107003, -321.4292242960311228 ) ) ;
#39860=CARTESIAN_POINT ( 'NONE',  ( 751.6929314249748586, -198.9982390220562252, -318.8095938919659034 ) ) ;
#39862=CARTESIAN_POINT ( 'NONE',  ( 778.1981804954715471, -130.2709662947837614, -314.8072714833591021 ) ) ;
#39864=CARTESIAN_POINT ( 'NONE',  ( 798.5707757039680246, -413.4636090269704027, -356.7845633553585003 ) ) ;
#39871=CARTESIAN_POINT ( 'NONE',  ( 758.4439275373578084, -396.5545181178794678, -353.2243759319684386 ) ) ;
#39873=CARTESIAN_POINT ( 'NONE',  ( 791.0478386215596629, -189.8272453906073736, -306.7653713866226326 ) ) ;
#39876=DIRECTION ( 'NONE',  ( 0.000000000000000000, 0.000000000000000000, -1.000000000000000000 ) ) ;
#39877=CARTESIAN_POINT ( 'NONE',  ( 755.0488828828309806, -329.8055962898683902, -344.1219089521771934 ) ) ;
#39879=CARTESIAN_POINT ( 'NONE',  ( 788.6739635108323228, -199.6454272087891582, -373.9316612368139090 ) ) ;
#39880=FACE_OUTER_BOUND ( 'NONE', #44620, .T. ) ;
#39883=CARTESIAN_POINT ( 'NONE',  ( 808.0189434323515343, -254.0891481129652334, -319.0252816721025511 ) ) ;
#39885=CARTESIAN_POINT ( 'NONE',  ( 797.6776695296629214, -19.54369356751139364, -357.6776695296636603 ) ) ;
#39887=CARTESIAN_POINT ( 'NONE',  ( 747.3154664389472828, -139.9874144716872024, -326.4474001241230781 ) ) ;
#39889=CARTESIAN_POINT ( 'NONE',  ( 812.7932403749906598, -375.1800572038739574, -327.7687537140311633 ) ) ;
#39894=CARTESIAN_POINT ( 'NONE',  ( 761.9338519418445230, -422.5328690171408539, -370.4231160770881957 ) ) ;
#39895=CARTESIAN_POINT ( 'NONE',  ( 755.8990559732751535, -11.46360902697159290, -365.9055244015606831 ) ) ;
#39898=ORIENTED_EDGE ( 'NONE', *, *, #17738, .T. ) ;
#39902=CARTESIAN_POINT ( 'NONE',  ( 776.9566956441375396, -204.8965053807779100, -364.8461984189686405 ) ) ;
#39904=CARTESIAN_POINT ( 'NONE',  ( 788.7631598425961101, -241.4419599262322720, -305.7194118038759143 ) ) ;
#39906=CARTESIAN_POINT ( 'NONE',  ( 774.6858677611749044, -81.72551174932937101, -315.5713283507209894 ) ) ;
#39908=CARTESIAN_POINT ( 'NONE',  ( 803.4237431249931660, -135.1800572038746679, -331.2633955100225194 ) ) ;
#39910=CARTESIAN_POINT ( 'NONE',  ( 808.3070685750230950, -90.99823902205663728, -361.1904061080339261 ) ) ;
#39911=ORIENTED_EDGE ( 'NONE', *, *, #13176, .T. ) ;
#39912=CARTESIAN_POINT ( 'NONE',  ( 769.9779781133707957, 4.900027336664720679, -316.7813123517150871 ) ) ;
#39914=CARTESIAN_POINT ( 'NONE',  ( 800.9840315886518738, -316.9181544815160692, -354.1144889064786412 ) ) ;
#39917=CARTESIAN_POINT ( 'NONE',  ( 756.5762568750052424, -291.1800572038741848, -348.7366044899774238 ) ) ;
#39920=CARTESIAN_POINT ( 'NONE',  ( 779.4763451958990572, -296.7363362996979390, -365.0264073115438919 ) ) ;
#39921=CARTESIAN_POINT ( 'NONE',  ( 771.1735550268778070, -297.1800572038740711, -316.3353852180827630 ) ) ;
#39923=CARTESIAN_POINT ( 'NONE',  ( 785.3141322388236176, -165.7255117493291152, -364.4286716492789537 ) ) ;
#39928=CARTESIAN_POINT ( 'NONE',  ( 811.3240766477731540, -100.3726999360622187, -355.6651683502462902 ) ) ;
#39934=CARTESIAN_POINT ( 'NONE',  ( 749.2812353651451076, -126.4527844766019626, -323.2262854647983090 ) ) ;
#39937=CARTESIAN_POINT ( 'NONE',  ( 780.5290396650775619, -420.3510508353225532, -365.2837595273619513 ) ) ;
#39940=CARTESIAN_POINT ( 'NONE',  ( 745.7998596910086917, -269.3618753856924286, -332.5602148656461168 ) ) ;
#39944=CARTESIAN_POINT ( 'NONE',  ( 803.8556311672234642, -297.6237781080502600, -365.6418435158340117 ) ) ;
#39946=CARTESIAN_POINT ( 'NONE',  ( 814.5518280994195948, -351.7255117493284047, -332.4837098697145734 ) ) ;
#39950=CARTESIAN_POINT ( 'NONE',  ( 759.9864689768902508, -410.0891481129647218, -354.9819416627836404 ) ) ;
#39952=CARTESIAN_POINT ( 'NONE',  ( 756.5762568750052424, -219.1800572038744122, -348.7366044899774238 ) ) ;
#39953=CARTESIAN_POINT ( 'NONE',  ( 798.0661480581538854, -122.5328690171417918, -309.5768839229118043 ) ) ;
#39958=CARTESIAN_POINT ( 'NONE',  ( 808.7758568127978833, -52.16923265350567362, -320.0363995740631822 ) ) ;
#39963=CARTESIAN_POINT ( 'NONE',  ( 748.6759233522253680, -328.3726999360615650, -324.3348316497537098 ) ) ;
#39967=CARTESIAN_POINT ( 'NONE',  ( 780.5236548040995785, -188.7363362996983085, -314.9735926884559944 ) ) ;
#39968=CARTESIAN_POINT ( 'NONE',  ( 762.1405469898971887, -193.5436935675108714, -357.8594530101015607 ) ) ;
#39969=CARTESIAN_POINT ( 'NONE',  ( 774.6858677611749044, -369.7255117493284615, -315.5713283507209894 ) ) ;
#39973=DIRECTION ( 'NONE',  ( 0.000000000000000000, -0.000000000000000000, -1.000000000000000000 ) ) ;
#39978=CARTESIAN_POINT ( 'NONE',  ( 757.7880784355613741, -426.0090635724247932, -312.4576283171834916 ) ) ;
#39980=CARTESIAN_POINT ( 'NONE',  ( 814.5518280994195948, -39.72551174932951312, -332.4837098697145166 ) ) ;
#39982=CARTESIAN_POINT ( 'NONE',  ( 788.8264449731200330, -381.1800572038737869, -363.6646147819171233 ) ) ;
#39983=CARTESIAN_POINT ( 'NONE',  ( 785.3141322388236176, 2.274488250670355871, -364.4286716492789537 ) ) ;
#39987=CARTESIAN_POINT ( 'NONE',  ( 796.1575198192839480, -246.0090635724253900, -359.4546378042384163 ) ) ;
#39988=CARTESIAN_POINT ( 'NONE',  ( 796.9462024416508257, -156.4527844766018916, -308.9653473494370246 ) ) ;
#39992=CARTESIAN_POINT ( 'NONE',  ( 763.3756531158825283, 16.45630643248848912, -321.2690078247891847 ) ) ;
#39996=CARTESIAN_POINT ( 'NONE',  ( 781.8018195045266339, -310.2709662947832499, -365.1927285166406705 ) ) ;
#39999=CARTESIAN_POINT ( 'NONE',  ( 810.4231160770870019, -48.55451811788057626, -321.9338519418446936 ) ) ;
#40000=CARTESIAN_POINT ( 'NONE',  ( 786.6156483768007774, -121.4419599262327267, -315.5913626894246136 ) ) ;
#40003=CARTESIAN_POINT ( 'NONE',  ( 785.3687786644884454, -11.36187538569323863, -315.3201227861279676 ) ) ;
#40004=CARTESIAN_POINT ( 'NONE',  ( 798.7617431975189675, -123.6237781080508569, -323.0428371773161871 ) ) ;
#40005=CARTESIAN_POINT ( 'NONE',  ( 781.8018195045266339, -142.2709662947837330, -365.1927285166406705 ) ) ;
#40006=CARTESIAN_POINT ( 'NONE',  ( 793.4146539503750546, 22.01258552831228599, -307.6481478633938877 ) ) ;
#40017=CARTESIAN_POINT ( 'NONE',  ( 755.8894580844503253, -87.82724539060770041, -332.3691319403863531 ) ) ;
#40020=CARTESIAN_POINT ( 'NONE',  ( 804.6798772138710092, -279.7255117493288026, -334.6312213355106451 ) ) ;
#40022=CARTESIAN_POINT ( 'NONE',  ( 800.2193346964447755, -378.9982390220555999, -355.1360043628815788 ) ) ;
#40023=CARTESIAN_POINT ( 'NONE',  ( 757.8323909638827445, -50.63460265842036989, -352.1044303154654358 ) ) ;
#40027=CARTESIAN_POINT ( 'NONE',  ( 757.7880784355613741, -18.00906357242611477, -312.4576283171834916 ) ) ;
#40030=CARTESIAN_POINT ( 'NONE',  ( 768.9521613784389729, -321.8272453906070609, -373.2346286133773106 ) ) ;
#40033=CARTESIAN_POINT ( 'NONE',  ( 785.3141322388236176, -309.7255117493287457, -364.4286716492789537 ) ) ;
#40034=CARTESIAN_POINT ( 'NONE',  ( 769.9779781133707957, -139.0999726633348530, -316.7813123517150871 ) ) ;
#40036=PLANE ( 'NONE',  #6236 ) ;
#40037=CARTESIAN_POINT ( 'NONE',  ( 808.3070685750232087, -330.9982390220558273, -361.1904061080339829 ) ) ;
#40041=CARTESIAN_POINT ( 'NONE',  ( 786.2056067578752163, -251.8055962898686744, -374.4686193811670023 ) ) ;
#40043=CARTESIAN_POINT ( 'NONE',  ( 787.4397851343537695, 2.274488250670355871, -374.2001403089903988 ) ) ;
#40045=ORIENTED_EDGE ( 'NONE', *, *, #7796, .F. ) ;
#40048=CARTESIAN_POINT ( 'NONE',  ( 756.1348686366196716, -17.26014174441486659, -347.5531968255698416 ) ) ;
#40052=VERTEX_POINT ( 'NONE', #41604 ) ;
#40053=CARTESIAN_POINT ( 'NONE',  ( 805.1016975059191054, -342.8965053807773984, -343.0745993439771837 ) ) ;
#40055=CARTESIAN_POINT ( 'NONE',  ( 748.3538107759620743, -328.7146871989592682, -355.8262568251490165 ) ) ;
#40058=ORIENTED_EDGE ( 'NONE', *, *, #37012, .F. ) ;
#40060=CARTESIAN_POINT ( 'NONE',  ( 754.9735926884551418, -66.35105083532378956, -340.5236548041000333 ) ) ;
#40063=CARTESIAN_POINT ( 'NONE',  ( 748.9653473494363425, -170.6346026584199649, -356.9462024416521331 ) ) ;
#40065=CARTESIAN_POINT ( 'NONE',  ( 781.8018195045267476, -166.2709662947836478, -365.1927285166407273 ) ) ;
#40067=CARTESIAN_POINT ( 'NONE',  ( 790.9844846989617508, -430.3726999360611671, -317.2208543904092721 ) ) ;
#40074=CARTESIAN_POINT ( 'NONE',  ( 763.0428371773158460, -419.4636090269702891, -358.7617431975195359 ) ) ;
#40077=CARTESIAN_POINT ( 'NONE',  ( 811.3240766477731540, -196.3726999360619061, -355.6651683502462902 ) ) ;
#40082=CARTESIAN_POINT ( 'NONE',  ( 803.2186876482843445, -319.9874144716866340, -350.0220218866286928 ) ) ;
#40084=CARTESIAN_POINT ( 'NONE',  ( 764.1737431748507561, -226.3726999360617924, -371.6461892240376415 ) ) ;
#40088=CARTESIAN_POINT ( 'NONE',  ( 815.2698199232962679, -232.8164208402379529, -342.5225473063383674 ) ) ;
#40090=CARTESIAN_POINT ( 'NONE',  ( 756.5762568750052424, -3.180057203875080063, -348.7366044899774238 ) ) ;
#40093=CARTESIAN_POINT ( 'NONE',  ( 801.9858362298568863, -123.0783235625963385, -312.7379699480935642 ) ) ;
#40095=CARTESIAN_POINT ( 'NONE',  ( 814.9108240113580450, -376.2709662947829656, -337.5031285880265273 ) ) ;
#40097=DIRECTION ( 'NONE',  ( 0.000000000000000000, 0.000000000000000000, -1.000000000000000000 ) ) ;
#40100=CARTESIAN_POINT ( 'NONE',  ( 754.8072714833581358, -388.8164208402374129, -338.1981804954720587 ) ) ;
#40101=CARTESIAN_POINT ( 'NONE',  ( 811.3240766477731540, -4.372699936062523385, -355.6651683502462902 ) ) ;
#40106=CARTESIAN_POINT ( 'NONE',  ( 783.0433043558608688, -240.8965053807777963, -315.1538015810313027 ) ) ;
#40109=CARTESIAN_POINT ( 'NONE',  ( 746.0683387631852383, -211.4419599262324709, -331.3260364891676204 ) ) ;
#40116=CARTESIAN_POINT ( 'NONE',  ( 767.7687537140311633, -71.90732993114760063, -372.7932403749916830 ) ) ;
#40117=CARTESIAN_POINT ( 'NONE',  ( 759.7806653035535192, -78.99823902205665149, -324.8639956371181370 ) ) ;
#40119=CARTESIAN_POINT ( 'NONE',  ( 755.5913626894240451, -13.64542720878976390, -346.6156483768012890 ) ) ;
#40121=CARTESIAN_POINT ( 'NONE',  ( 799.2566176426618085, -312.0090635724251911, -324.0069404352559559 ) ) ;
#40123=VECTOR ( 'NONE', #43751, 1000.000000000000000 ) ;
#40126=CARTESIAN_POINT ( 'NONE',  ( 755.5713283507202505, -317.3618753856922581, -334.6858677611754729 ) ) ;
#40130=CARTESIAN_POINT ( 'NONE',  ( 805.2837595273609850, -338.7363362996978822, -340.5290396650784714 ) ) ;
#40131=CARTESIAN_POINT ( 'NONE',  ( 778.2165204200184689, -286.8164208402378677, -364.9363028652563230 ) ) ;
#40132=CARTESIAN_POINT ( 'NONE',  ( 791.7608162188021197, 178.9475563372491251, -320.0000000000000000 ) ) ;
#40133=CARTESIAN_POINT ( 'NONE',  ( 762.1405469898971887, -145.5436935675109851, -357.8594530101015607 ) ) ;
#40134=EDGE_CURVE ( 'NONE', #35503, #9202, #13215, .T. ) ;
#40139=CARTESIAN_POINT ( 'NONE',  ( 771.3260364891663130, -91.64542720878951343, -306.0683387631859773 ) ) ;
#40142=EDGE_CURVE ( 'NONE', #38597, #24791, #34200, .T. ) ;
#40148=CARTESIAN_POINT ( 'NONE',  ( 758.8095938919644823, -128.0891481129655745, -311.6929314249762797 ) ) ;
#40151=CARTESIAN_POINT ( 'NONE',  ( 772.4837098697144029, -263.3618753856924855, -374.5518280994205611 ) ) ;
#40154=CARTESIAN_POINT ( 'NONE',  ( 800.1688906516307043, -346.1692326535047641, -369.0717654672308186 ) ) ;
#40155=CARTESIAN_POINT ( 'NONE',  ( 751.6929314249748586, -78.99823902205662307, -318.8095938919659034 ) ) ;
#40156=CIRCLE ( 'NONE', #6948, 30.00000000000008171 ) ;
#40158=CARTESIAN_POINT ( 'NONE',  ( 745.4481719005789273, -363.7255117493284047, -347.5162901302853129 ) ) ;
#40159=DIRECTION ( 'NONE',  ( 0.000000000000000000, 0.000000000000000000, 1.000000000000000000 ) ) ;
#40163=CARTESIAN_POINT ( 'NONE',  ( 771.2633955100217236, -431.9073299311464211, -363.4237431249939618 ) ) ;
#40165=CARTESIAN_POINT ( 'NONE',  ( 778.7502325331095108, -120.3510508353236048, -304.6391490659818828 ) ) ;
#40170=CARTESIAN_POINT ( 'NONE',  ( 804.1601925771018387, -247.4419599262323004, -346.5483106153029098 ) ) ;
#40172=CARTESIAN_POINT ( 'NONE',  ( 777.4774526936600978, 13.72903370521577138, -304.7301800767027657 ) ) ;
#40173=CARTESIAN_POINT ( 'NONE',  ( 766.5853460496234675, -61.98741447168745822, -372.3518521366060554 ) ) ;
#40178=CARTESIAN_POINT ( 'NONE',  ( 795.8262568251477660, -382.3726999360613945, -308.3538107759623585 ) ) ;
#40183=CARTESIAN_POINT ( 'NONE',  ( 772.4468031744293057, -177.8272453906074304, -363.8651313633793620 ) ) ;
#40184=CARTESIAN_POINT ( 'NONE',  ( 754.8072714833581358, -172.8164208402381234, -338.1981804954720587 ) ) ;
#40185=CARTESIAN_POINT ( 'NONE',  ( 804.9363028652555840, -400.2709662947828519, -338.2165204200192079 ) ) ;
#40189=CARTESIAN_POINT ( 'NONE',  ( 795.1360043628807261, -452.0891481129646650, -360.2193346964456282 ) ) ;
#40197=EDGE_CURVE ( 'NONE', #14073, #811, #34794, .T. ) ;
#40202=CARTESIAN_POINT ( 'NONE',  ( 746.4236121716829757, -399.8272453906067767, -328.8385539511384650 ) ) ;
#40203=CARTESIAN_POINT ( 'NONE',  ( 763.2262854647970016, -32.63460265842044095, -309.2812353651462445 ) ) ;
#40205=CARTESIAN_POINT ( 'NONE',  ( 759.9864689768902508, -410.0891481129647218, -354.9819416627836404 ) ) ;
#40206=CARTESIAN_POINT ( 'NONE',  ( 805.1927285166399315, -16.81642084023867412, -341.8018195045277707 ) ) ;
#40208=CARTESIAN_POINT ( 'NONE',  ( 799.9999999999993179, -512.9681489794448908, -329.9999999999999432 ) ) ;
#40209=CARTESIAN_POINT ( 'NONE',  ( 802.5472867521000353, -244.3726999360617924, -350.8726784830461156 ) ) ;
#40210=CARTESIAN_POINT ( 'NONE',  ( 815.2698199232961542, -160.8164208402382371, -342.5225473063383106 ) ) ;
#40223=CARTESIAN_POINT ( 'NONE',  ( 804.9363028652555840, -328.2709662947831362, -338.2165204200192079 ) ) ;
#40226=CARTESIAN_POINT ( 'NONE',  ( 750.9282345327678740, -112.9181544815167229, -319.8311093483690115 ) ) ;
#40227=CARTESIAN_POINT ( 'NONE',  ( 784.0799538623451781, -107.8055962898691433, -364.6971507214555572 ) ) ;
#40232=CARTESIAN_POINT ( 'NONE',  ( 765.0180583372156207, -24.99823902205683268, -360.0135310231089534 ) ) ;
#40233=CARTESIAN_POINT ( 'NONE',  ( 755.0488828828309806, -137.8055962898690154, -344.1219089521771934 ) ) ;
#40234=CARTESIAN_POINT ( 'NONE',  ( 759.7806653035534055, -126.9982390220565094, -324.8639956371180801 ) ) ;
#40237=CARTESIAN_POINT ( 'NONE',  ( 776.9566956441375396, -420.8965053807772279, -364.8461984189686405 ) ) ;
#40243=CARTESIAN_POINT ( 'NONE',  ( 768.9521613784389729, -273.8272453906071746, -373.2346286133773106 ) ) ;
#40252=CARTESIAN_POINT ( 'NONE',  ( 783.0745993439762742, -80.19088175424411702, -365.1016975059196739 ) ) ;
#40253=CARTESIAN_POINT ( 'NONE',  ( 762.3223304703356007, -271.5436935675106156, -322.3223304703362828 ) ) ;
#40256=CARTESIAN_POINT ( 'NONE',  ( 771.2633955100217236, -407.9073299311465348, -363.4237431249939618 ) ) ;
#40257=CARTESIAN_POINT ( 'NONE',  ( 756.5762568750052424, -51.18005720387493085, -348.7366044899774238 ) ) ;
#40263=EDGE_CURVE ( 'NONE', #36235, #3824, #31877, .T. ) ;
#40264=CARTESIAN_POINT ( 'NONE',  ( 783.7953271457878373, -8.190881754244330182, -375.1787889125761239 ) ) ;
#40267=CARTESIAN_POINT ( 'NONE',  ( 754.3581564841646241, -305.4636090269706870, -316.1443688327762516 ) ) ;
#40271=CARTESIAN_POINT ( 'NONE',  ( 755.5713283507202505, -293.3618753856923718, -334.6858677611754729 ) ) ;
#40272=CARTESIAN_POINT ( 'NONE',  ( 787.5531968255692163, -165.8272453906074873, -316.1348686366205811 ) ) ;
#40276=CARTESIAN_POINT ( 'NONE',  ( 746.7653713866222915, -17.26014174441486659, -351.0478386215610271 ) ) ;
#40277=CARTESIAN_POINT ( 'NONE',  ( 792.3570229623691148, -333.1800572038740142, -373.1304606946836770 ) ) ;
#40282=CARTESIAN_POINT ( 'NONE',  ( 798.0661480581538854, -434.5328690171407970, -309.5768839229118043 ) ) ;
#40287=CARTESIAN_POINT ( 'NONE',  ( 761.2382568024794409, -15.62377810805123524, -356.9571628226838129 ) ) ;
#40294=CARTESIAN_POINT ( 'NONE',  ( 791.9812246680005501, -44.63460265842040542, -361.9419747391813189 ) ) ;
#40296=CARTESIAN_POINT ( 'NONE',  ( 786.6156483768007774, -337.4419599262319593, -315.5913626894246136 ) ) ;
#40299=CARTESIAN_POINT ( 'NONE',  ( 815.0009284576459549, -318.3510508353230080, -338.7629533639073429 ) ) ;
#40308=CARTESIAN_POINT ( 'NONE',  ( 763.2262854647970016, -176.6346026584199933, -309.2812353651462445 ) ) ;
#40311=CARTESIAN_POINT ( 'NONE',  ( 755.0636971347428243, -172.2709662947836478, -341.7834795799807353 ) ) ;
#40313=CARTESIAN_POINT ( 'NONE',  ( 801.5560724626406000, -408.5545181178794110, -326.7756240680316182 ) ) ;
#40321=CARTESIAN_POINT ( 'NONE',  ( 796.1575198192839480, -414.0090635724249637, -359.4546378042384163 ) ) ;
#40323=CARTESIAN_POINT ( 'NONE',  ( 745.5313806188320314, -207.2817908451527842, -333.7943932421247268 ) ) ;
#40325=AXIS2_PLACEMENT_3D ( 'NONE', #33767, #1880, #44379 ) ;
#40327=CARTESIAN_POINT ( 'NONE',  ( 768.0187753319979720, -176.6346026584199933, -318.0580252608186242 ) ) ;
#40328=CARTESIAN_POINT ( 'NONE',  ( 805.1016975059191054, -342.8965053807773984, -343.0745993439771837 ) ) ;
#40330=CARTESIAN_POINT ( 'NONE',  ( 745.7194118038753459, -229.6454272087890729, -348.7631598425976449 ) ) ;
#40333=CARTESIAN_POINT ( 'NONE',  ( 755.3028492785439312, -39.28179084515331709, -335.9200461376539693 ) ) ;
#40336=CARTESIAN_POINT ( 'NONE',  ( 767.6429770376291799, -225.1800572038743553, -306.8695393053162093 ) ) ;
#40339=CARTESIAN_POINT ( 'NONE',  ( 778.1981804954714335, -10.27096629478414691, -314.8072714833589885 ) ) ;
#40341=CARTESIAN_POINT ( 'NONE',  ( 749.8865473780648472, -140.5328690171417634, -322.1177392798429082 ) ) ;
#40343=CARTESIAN_POINT ( 'NONE',  ( 745.4481719005789273, -387.7255117493283478, -347.5162901302853129 ) ) ;
#40348=CARTESIAN_POINT ( 'NONE',  ( 803.4237431249931660, -399.1800572038738437, -331.2633955100225194 ) ) ;
#40350=CARTESIAN_POINT ( 'NONE',  ( 782.4968714119720516, -442.8164208402372992, -305.0891759886411023 ) ) ;
#40354=CARTESIAN_POINT ( 'NONE',  ( 799.4546378042377910, -225.0783235625959833, -356.1575198192848006 ) ) ;
#40356=CARTESIAN_POINT ( 'NONE',  ( 759.8311093483677041, -214.1692326535052189, -310.9282345327691814 ) ) ;
#40359=ORIENTED_EDGE ( 'NONE', *, *, #40263, .T. ) ;
#40361=CARTESIAN_POINT ( 'NONE',  ( 802.7791456095903868, -28.71468719896028077, -329.0155153010375102 ) ) ;
#40364=CARTESIAN_POINT ( 'NONE',  ( 782.5225473063381969, -70.27096629478397460, -375.2698199232970637 ) ) ;
#40365=CARTESIAN_POINT ( 'NONE',  ( 802.1676090361155502, -86.63460265842024910, -327.8955696845344505 ) ) ;
#40366=ORIENTED_EDGE ( 'NONE', *, *, #14121, .F. ) ;
#40367=CARTESIAN_POINT ( 'NONE',  ( 790.9844846989617508, -22.37269993606246743, -317.2208543904092721 ) ) ;
#40370=CARTESIAN_POINT ( 'NONE',  ( 759.0159684113467620, -304.9181544815161828, -325.8855110935213020 ) ) ;
#40373=VECTOR ( 'NONE', #32476, 1000.000000000000000 ) ;
#40378=CARTESIAN_POINT ( 'NONE',  ( 804.6971507214547046, -339.2817908451524431, -344.0799538623459739 ) ) ;
#40379=CARTESIAN_POINT ( 'NONE',  ( 804.9363028652555840, -328.2709662947831362, -338.2165204200192079 ) ) ;
#40380=CARTESIAN_POINT ( 'NONE',  ( 778.2165204200184689, -142.8164208402382656, -364.9363028652563230 ) ) ;
#40384=CARTESIAN_POINT ( 'NONE',  ( 799.9636004259356241, -118.9181544815167229, -311.2241431872006956 ) ) ;
#40390=CARTESIAN_POINT ( 'NONE',  ( 808.0189434323515343, -134.0891481129655745, -319.0252816721025511 ) ) ;
#40393=CARTESIAN_POINT ( 'NONE',  ( 772.5602148656447525, -273.7255117493288026, -305.7998596910095443 ) ) ;
#40394=CARTESIAN_POINT ( 'NONE',  ( 787.5162901302840055, -443.3618753856917465, -305.4481719005793252 ) ) ;
#40397=CARTESIAN_POINT ( 'NONE',  ( 783.7566961878529810, -336.8965053807774552, -305.1792804349288417 ) ) ;
#40399=CARTESIAN_POINT ( 'NONE',  ( 748.9653473494363425, -74.63460265842032015, -356.9462024416521331 ) ) ;
#40401=CARTESIAN_POINT ( 'NONE',  ( 792.2312462859673587, -347.9073299311467053, -307.2067596250082602 ) ) ;
#40402=CARTESIAN_POINT ( 'NONE',  ( 759.9999999999992042, 205.0000000000000568, -329.9999999999999432 ) ) ;
#40404=EDGE_LOOP ( 'NONE', ( #21449, #37386, #29041, #2265 ) ) ;
#40406=CARTESIAN_POINT ( 'NONE',  ( 756.1443688327750579, -117.6237781080509279, -314.3581564841659315 ) ) ;
#40412=CARTESIAN_POINT ( 'NONE',  ( 788.7631598425961101, -433.4419599262316183, -305.7194118038759143 ) ) ;
#40413=CARTESIAN_POINT ( 'NONE',  ( 747.3154664389472828, -67.98741447168742980, -326.4474001241230781 ) ) ;
#40419=CARTESIAN_POINT ( 'NONE',  ( 758.4439275373578084, -204.5545181178800931, -353.2243759319684386 ) ) ;
#40420=CARTESIAN_POINT ( 'NONE',  ( 792.1044303154645831, -228.4527844766015789, -317.8323909638837677 ) ) ;
#40421=CARTESIAN_POINT ( 'NONE',  ( 794.9819416627830151, -372.9982390220557704, -319.9864689768909898 ) ) ;
#40423=CARTESIAN_POINT ( 'NONE',  ( 785.3687786644884454, -107.3618753856928976, -315.3201227861279676 ) ) ;
#40433=CARTESIAN_POINT ( 'NONE',  ( 766.9102291470427417, 5.445481882119263872, -318.6633372737382501 ) ) ;
#40434=CARTESIAN_POINT ( 'NONE',  ( 751.9810565676468741, -50.08914811296584446, -360.9747183278973921 ) ) ;
#40436=CARTESIAN_POINT ( 'NONE',  ( 768.0187753319979720, -392.6346026584193396, -318.0580252608186242 ) ) ;
#40437=CARTESIAN_POINT ( 'NONE',  ( 771.2633955100217236, 0.09267006885218045942, -363.4237431249939618 ) ) ;
#40440=CARTESIAN_POINT ( 'NONE',  ( 798.5707757039680246, -269.4636090269708006, -356.7845633553585003 ) ) ;
#40441=CARTESIAN_POINT ( 'NONE',  ( 759.0252816721024374, -168.9982390220563673, -368.0189434323527280 ) ) ;
#40444=CARTESIAN_POINT ( 'NONE',  ( 774.9293440288117836, 16.45630643248849623, -314.9535949064562601 ) ) ;
#40447=CARTESIAN_POINT ( 'NONE',  ( 800.0135310231082713, -326.0891481129649492, -325.0180583372163028 ) ) ;
#40450=CARTESIAN_POINT ( 'NONE',  ( 814.4686193811664907, -99.28179084515313946, -346.2056067578752732 ) ) ;
#40451=CARTESIAN_POINT ( 'NONE',  ( 780.5290396650775619, -132.3510508353235764, -365.2837595273619513 ) ) ;
#40455=CARTESIAN_POINT ( 'NONE',  ( 781.8018195045266339, -22.27096629478410250, -365.1927285166406705 ) ) ;
#40456=CARTESIAN_POINT ( 'NONE',  ( 765.8855110935204493, -142.1692326535054178, -319.0159684113471599 ) ) ;
#40457=CARTESIAN_POINT ( 'NONE',  ( 791.9812246680005501, -116.6346026584201780, -361.9419747391813189 ) ) ;
#40459=EDGE_CURVE ( 'NONE', #2036, #22721, #38888, .T. ) ;
#40460=CARTESIAN_POINT ( 'NONE',  ( 756.1348686366196716, -425.2601417444136018, -347.5531968255698416 ) ) ;
#40464=ORIENTED_EDGE ( 'NONE', *, *, #36589, .F. ) ;
#40466=CARTESIAN_POINT ( 'NONE',  ( 781.2370466360911223, -284.7363362996979390, -304.9990715423533629 ) ) ;
#40467=EDGE_LOOP ( 'NONE', ( #44305, #40728, #760, #28241 ) ) ;
#40473=CARTESIAN_POINT ( 'NONE',  ( 766.0291762391763086, -106.9181544815167371, -360.7704444035551319 ) ) ;
#40474=CARTESIAN_POINT ( 'NONE',  ( 758.0580252608178853, -270.4527844766014937, -328.0187753319985404 ) ) ;
#40476=CARTESIAN_POINT ( 'NONE',  ( 805.1927285166397041, -424.8164208402372992, -341.8018195045277707 ) ) ;
#40477=CARTESIAN_POINT ( 'NONE',  ( 755.5713283507202505, -101.3618753856929544, -334.6858677611754729 ) ) ;
#40481=CARTESIAN_POINT ( 'NONE',  ( 754.3581564841646241, -17.46360902697157513, -316.1443688327762516 ) ) ;
#40484=CARTESIAN_POINT ( 'NONE',  ( 748.6759233522253680, -352.3726999360614514, -324.3348316497537098 ) ) ;
#40488=CARTESIAN_POINT ( 'NONE',  ( 757.8323909638827445, -290.6346026584195101, -352.1044303154654358 ) ) ;
#40490=CARTESIAN_POINT ( 'NONE',  ( 766.0291762391763086, -154.9181544815165523, -360.7704444035551319 ) ) ;
#40493=CARTESIAN_POINT ( 'NONE',  ( 777.5031285880264704, -334.8164208402376403, -374.9108240113588408 ) ) ;
#40499=CARTESIAN_POINT ( 'NONE',  ( 810.7187646348534145, 5.547215523397618142, -356.7737145352016341 ) ) ;
#40505=CARTESIAN_POINT ( 'NONE',  ( 802.7791456095903868, -28.71468719896028077, -329.0155153010375102 ) ) ;
#40511=CARTESIAN_POINT ( 'NONE',  ( 790.8726784830453198, -346.7146871989592682, -362.5472867521010585 ) ) ;
#40514=CARTESIAN_POINT ( 'NONE',  ( 764.3348316497523456, -334.7146871989593251, -308.6759233522265617 ) ) ;
#40521=CARTESIAN_POINT ( 'NONE',  ( 800.9747183278959710, -180.9982390220563389, -311.9810565676471583 ) ) ;
#40524=CARTESIAN_POINT ( 'NONE',  ( 804.6798772138710092, -183.7255117493290300, -334.6312213355106451 ) ) ;
#40527=CARTESIAN_POINT ( 'NONE',  ( 790.9844846989617508, -454.3726999360611103, -317.2208543904092721 ) ) ;
#40534=CARTESIAN_POINT ( 'NONE',  ( 755.5913626894240451, -445.6454272087883055, -346.6156483768012890 ) ) ;
#40536=CARTESIAN_POINT ( 'NONE',  ( 760.0363995740630116, -202.9181544815164386, -368.7758568127991907 ) ) ;
#40539=CARTESIAN_POINT ( 'NONE',  ( 756.3353852180819104, -197.9073299311472169, -331.1735550268788302 ) ) ;
#40540=CARTESIAN_POINT ( 'NONE',  ( 770.0799878456142551, -349.9874144716865771, -362.9823548866085616 ) ) ;
#40542=CARTESIAN_POINT ( 'NONE',  ( 762.1177392798416577, -210.5545181178800647, -309.8865473780659272 ) ) ;
#40545=CARTESIAN_POINT ( 'NONE',  ( 776.9254006560222479, -44.19088175424421649, -314.8983024940802125 ) ) ;
#40547=CARTESIAN_POINT ( 'NONE',  ( 814.2001403089898304, -233.3618753856925423, -347.4397851343538264 ) ) ;
#40550=CARTESIAN_POINT ( 'NONE',  ( 754.8072714833581358, -52.81642084023856398, -338.1981804954720587 ) ) ;
#40555=CARTESIAN_POINT ( 'NONE',  ( 768.8385539511368734, -143.2601417444144829, -306.4236121716840557 ) ) ;
#40557=CARTESIAN_POINT ( 'NONE',  ( 810.7187646348534145, -378.4527844766011526, -356.7737145352016341 ) ) ;
#40562=CARTESIAN_POINT ( 'NONE',  ( 797.6776695296629214, -403.5436935675101608, -357.6776695296636603 ) ) ;
#40564=CARTESIAN_POINT ( 'NONE',  ( 814.5518280994195948, -447.7255117493280636, -332.4837098697145734 ) ) ;
#40569=CARTESIAN_POINT ( 'NONE',  ( 795.9930595647434757, -219.0783235625960401, -320.7433823573372820 ) ) ;
#40571=CARTESIAN_POINT ( 'NONE',  ( 807.5423716828161105, -225.0783235625959833, -362.2119215644372048 ) ) ;
#40576=CARTESIAN_POINT ( 'NONE',  ( 791.9812246680005501, -140.6346026584201070, -361.9419747391813189 ) ) ;
#40578=CARTESIAN_POINT ( 'NONE',  ( 814.2001403089898304, -65.36187538569306810, -347.4397851343538264 ) ) ;
#40579=CARTESIAN_POINT ( 'NONE',  ( 762.1405469898973024, -73.54369356751121245, -357.8594530101016176 ) ) ;
#40581=CARTESIAN_POINT ( 'NONE',  ( 800.9840315886518738, -4.918154481517067467, -354.1144889064786412 ) ) ;
#40583=CARTESIAN_POINT ( 'NONE',  ( 776.9254006560222479, -332.1908817542433781, -314.8983024940802125 ) ) ;
#40590=CARTESIAN_POINT ( 'NONE',  ( 759.0159684113467620, -328.9181544815160692, -325.8855110935213020 ) ) ;
#40591=CARTESIAN_POINT ( 'NONE',  ( 774.6312213355099630, -335.3618753856920307, -364.6798772138717482 ) ) ;
#40592=CARTESIAN_POINT ( 'NONE',  ( 801.9419747391806368, -162.4527844766018632, -351.9812246680014027 ) ) ;
#40596=CARTESIAN_POINT ( 'NONE',  ( 814.8207195650702488, -122.1908817542439749, -336.2433038121456548 ) ) ;
#40602=CARTESIAN_POINT ( 'NONE',  ( 751.6929314249750860, -150.9982390220564241, -318.8095938919659034 ) ) ;
#40605=CARTESIAN_POINT ( 'NONE',  ( 759.0252816721024374, -264.9982390220561115, -368.0189434323527280 ) ) ;
#40609=CARTESIAN_POINT ( 'NONE',  ( 815.0009284576459549, -342.3510508353228943, -338.7629533639073429 ) ) ;
#40610=CARTESIAN_POINT ( 'NONE',  ( 815.2698199232961542, -88.81642084023842187, -342.5225473063383106 ) ) ;
#40612=CARTESIAN_POINT ( 'NONE',  ( 805.0032342141412300, -349.5436935675102745, -314.9967657858571783 ) ) ;
#40617=CARTESIAN_POINT ( 'NONE',  ( 748.3538107759620743, -136.7146871989600072, -355.8262568251490165 ) ) ;
#40624=CARTESIAN_POINT ( 'NONE',  ( 803.8556311672234642, -417.6237781080499190, -365.6418435158340117 ) ) ;
#40628=CARTESIAN_POINT ( 'NONE',  ( 809.0717654672305343, -388.9181544815158986, -360.1688906516309885 ) ) ;
#40631=CARTESIAN_POINT ( 'NONE',  ( 780.5236548040995785, -212.7363362996982232, -314.9735926884559944 ) ) ;
#40632=CARTESIAN_POINT ( 'NONE',  ( 768.0187753319979720, -224.6346026584198228, -318.0580252608186242 ) ) ;
#40633=CARTESIAN_POINT ( 'NONE',  ( 797.8594530101009923, -397.5436935675101040, -322.1405469898982119 ) ) ;
#40634=ORIENTED_EDGE ( 'NONE', *, *, #22448, .F. ) ;
#40636=CARTESIAN_POINT ( 'NONE',  ( 800.2193346964447755, -90.99823902205663728, -355.1360043628815788 ) ) ;
#40645=CARTESIAN_POINT ( 'NONE',  ( 810.4231160770870019, -456.5545181178792404, -321.9338519418446936 ) ) ;
#40646=CARTESIAN_POINT ( 'NONE',  ( 810.7187646348534145, -18.45278447660230725, -356.7737145352016341 ) ) ;
#40648=CARTESIAN_POINT ( 'NONE',  ( 762.3223304703356007, -391.5436935675101608, -322.3223304703362828 ) ) ;
#40649=CARTESIAN_POINT ( 'NONE',  ( 804.9363028652555840, -16.27096629478413092, -338.2165204200192079 ) ) ;
#40651=CARTESIAN_POINT ( 'NONE',  ( 799.9999999999993179, -462.9681489794448339, -317.6393202250019954 ) ) ;
#40652=CARTESIAN_POINT ( 'NONE',  ( 793.9708237608222134, -286.9181544815161828, -319.2295555964448681 ) ) ;
#40653=CARTESIAN_POINT ( 'NONE',  ( 814.5518280994195948, -159.7255117493291436, -332.4837098697145734 ) ) ;
#40656=CARTESIAN_POINT ( 'NONE',  ( 789.5497161195852414, 16.45630643248838609, -314.2297168413928148 ) ) ;
#40660=CARTESIAN_POINT ( 'NONE',  ( 758.0580252608178853, -342.4527844766013231, -328.0187753319985404 ) ) ;
#40662=CARTESIAN_POINT ( 'NONE',  ( 744.6391490659812007, -86.73633629969862113, -338.7502325331110455 ) ) ;
#40663=CARTESIAN_POINT ( 'NONE',  ( 770.0799878456142551, -133.9874144716872024, -362.9823548866085616 ) ) ;
#40666=CARTESIAN_POINT ( 'NONE',  ( 764.8639956371174549, -32.08914811296588709, -319.7806653035542013 ) ) ;
#40667=CARTESIAN_POINT ( 'NONE',  ( 779.4709603349208464, -168.3510508353234911, -314.7162404726379918 ) ) ;
#40669=CARTESIAN_POINT ( 'NONE',  ( 773.3843516231979720, -421.4419599262317888, -364.4086373105754433 ) ) ;
#40676=CARTESIAN_POINT ( 'NONE',  ( 805.6418435158337843, -269.4636090269708006, -363.8556311672236916 ) ) ;
#40683=CARTESIAN_POINT ( 'NONE',  ( 755.3028492785439312, -111.2817908451530968, -335.9200461376539693 ) ) ;
#40684=CARTESIAN_POINT ( 'NONE',  ( 755.3201227861273992, -123.7255117493292147, -345.3687786644892981 ) ) ;
#40685=CARTESIAN_POINT ( 'NONE',  ( 778.1981804954715471, -274.2709662947832499, -314.8072714833591021 ) ) ;
#40687=CARTESIAN_POINT ( 'NONE',  ( 781.8018195045266339, -430.2709662947827383, -365.1927285166406705 ) ) ;
#40688=CARTESIAN_POINT ( 'NONE',  ( 797.8594530101008786, -85.54369356751118403, -322.1405469898980982 ) ) ;
#40694=CARTESIAN_POINT ( 'NONE',  ( 771.3260364891663130, -355.6454272087887603, -306.0683387631859773 ) ) ;
#40697=DIRECTION ( 'NONE',  ( 1.000000000000000000, 0.000000000000000000, 0.000000000000000000 ) ) ;
#40698=CARTESIAN_POINT ( 'NONE',  ( 788.7366044899766848, -275.9073299311469896, -316.5762568750059813 ) ) ;
#40700=CARTESIAN_POINT ( 'NONE',  ( 779.4763451958990572, -176.7363362996983369, -365.0264073115438919 ) ) ;
#40701=ADVANCED_FACE ( 'NONE', ( #16153 ), #19616, .F. ) ;
#40705=CARTESIAN_POINT ( 'NONE',  ( 746.8695393053151292, -389.9073299311465917, -327.6429770376306578 ) ) ;
#40710=CARTESIAN_POINT ( 'NONE',  ( 801.1904061080336987, -20.08914811296592973, -368.3070685750235498 ) ) ;
#40711=CARTESIAN_POINT ( 'NONE',  ( 781.8018195045266339, -262.2709662947831930, -365.1927285166406705 ) ) ;
#40715=CARTESIAN_POINT ( 'NONE',  ( 789.9200121543843807, -1.987414471687640294, -317.0176451133914384 ) ) ;
#40719=ORIENTED_EDGE ( 'NONE', *, *, #22865, .T. ) ;
#40720=CARTESIAN_POINT ( 'NONE',  ( 793.2243759319678702, -314.5328690171411949, -318.4439275373583200 ) ) ;
#40724=CARTESIAN_POINT ( 'NONE',  ( 781.2497674668890113, -348.3510508353228943, -375.3608509340180603 ) ) ;
#40728=ORIENTED_EDGE ( 'NONE', *, *, #151, .T. ) ;
#40730=CARTESIAN_POINT ( 'NONE',  ( 745.0891759886404770, -196.2709662947835909, -342.4968714119734159 ) ) ;
#40734=CARTESIAN_POINT ( 'NONE',  ( 794.9819416627830151, -180.9982390220563389, -319.9864689768909898 ) ) ;
#40735=ORIENTED_EDGE ( 'NONE', *, *, #31205, .T. ) ;
#40736=CARTESIAN_POINT ( 'NONE',  ( 793.9708237608222134, -454.9181544815156713, -319.2295555964448681 ) ) ;
#40743=CARTESIAN_POINT ( 'NONE',  ( 805.2837595273609850, -434.7363362996975980, -340.5290396650784714 ) ) ;
#40746=CARTESIAN_POINT ( 'NONE',  ( 778.7629533639073998, -224.7363362996982232, -375.0009284576466371 ) ) ;
#40749=CARTESIAN_POINT ( 'NONE',  ( 781.8018195045266339, -190.2709662947835909, -365.1927285166406705 ) ) ;
#40750=CARTESIAN_POINT ( 'NONE',  ( 759.2295555964440155, -352.1692326535046504, -353.9708237608231229 ) ) ;
#40752=CARTESIAN_POINT ( 'NONE',  ( 799.9636004259356241, -238.9181544815163534, -311.2241431872006956 ) ) ;
#40755=CARTESIAN_POINT ( 'NONE',  ( 769.0155153010367712, -34.37269993606243901, -362.7791456095907279 ) ) ;
#40760=CARTESIAN_POINT ( 'NONE',  ( 776.9566956441375396, -420.8965053807772279, -364.8461984189686405 ) ) ;
#40761=CARTESIAN_POINT ( 'NONE',  ( 754.9967657858570647, -289.5436935675105019, -365.0032342141425943 ) ) ;
#40765=CARTESIAN_POINT ( 'NONE',  ( 778.2165204200184689, -46.81642084023858530, -364.9363028652563230 ) ) ;
#40767=CARTESIAN_POINT ( 'NONE',  ( 814.8230680027162407, -125.8055962898690581, -333.7305795820267917 ) ) ;
#40769=CARTESIAN_POINT ( 'NONE',  ( 746.8695393053150156, -413.9073299311465348, -327.6429770376306010 ) ) ;
#40773=EDGE_CURVE ( 'NONE', #37557, #17589, #1604, .T. ) ;
#40774=CARTESIAN_POINT ( 'NONE',  ( 805.1927285166397041, -400.8164208402373561, -341.8018195045277707 ) ) ;
#40776=CARTESIAN_POINT ( 'NONE',  ( 771.3260364891663130, -43.64542720878966975, -306.0683387631859773 ) ) ;
#40781=CARTESIAN_POINT ( 'NONE',  ( 754.9735926884551418, -234.3510508353232638, -340.5236548041000333 ) ) ;
#40784=CARTESIAN_POINT ( 'NONE',  ( 745.1769319972822814, -209.8055962898687881, -346.2694204179732083 ) ) ;
#40789=CARTESIAN_POINT ( 'NONE',  ( 801.9419747391806368, -186.4527844766017779, -351.9812246680014027 ) ) ;
#40791=CARTESIAN_POINT ( 'NONE',  ( 800.9747183278959710, -84.99823902205663728, -311.9810565676471583 ) ) ;
#40793=CARTESIAN_POINT ( 'NONE',  ( 804.4286716492782716, -89.36187538569299704, -345.3141322388244703 ) ) ;
#40795=CARTESIAN_POINT ( 'NONE',  ( 799.2566176426618085, -24.00906357242609346, -324.0069404352559559 ) ) ;
#40797=CARTESIAN_POINT ( 'NONE',  ( 755.5913626894240451, -349.6454272087887603, -346.6156483768012890 ) ) ;
#40805=CARTESIAN_POINT ( 'NONE',  ( 780.5236548040995785, -332.7363362996979390, -314.9735926884559944 ) ) ;
#40806=CARTESIAN_POINT ( 'NONE',  ( 800.0135310231082713, -326.0891481129649492, -325.0180583372163028 ) ) ;
#40807=CARTESIAN_POINT ( 'NONE',  ( 814.2805881961230625, -145.6454272087893287, -331.2368401574024119 ) ) ;
#40809=STYLED_ITEM('',(#45765),#33039);
#40812=CARTESIAN_POINT ( 'NONE',  ( 776.9566956441375396, -252.8965053807777394, -364.8461984189686405 ) ) ;
#40813=CARTESIAN_POINT ( 'NONE',  ( 802.2119215644370342, -126.0090635724257737, -367.5423716828165084 ) ) ;
#40814=DIRECTION ( 'NONE',  ( 0.000000000000000000, 0.000000000000000000, -1.000000000000000000 ) ) ;
#40822=CARTESIAN_POINT ( 'NONE',  ( 744.7301800767020268, -148.8164208402382656, -337.4774526936615189 ) ) ;
#40825=CARTESIAN_POINT ( 'NONE',  ( 813.1304606946830518, -281.9073299311468759, -352.3570229623690580 ) ) ;
#40826=CARTESIAN_POINT ( 'NONE',  ( 808.3070685750232087, -450.9982390220554294, -361.1904061080339829 ) ) ;
#40830=CARTESIAN_POINT ( 'NONE',  ( 756.1443688327750579, -357.6237781080501463, -314.3581564841659315 ) ) ;
#40832=CARTESIAN_POINT ( 'NONE',  ( 801.1904061080336987, -92.08914811296568814, -368.3070685750235498 ) ) ;
#40834=CARTESIAN_POINT ( 'NONE',  ( 763.2262854647970016, -344.6346026584195101, -309.2812353651462445 ) ) ;
#40835=DIRECTION ( 'NONE',  ( 0.000000000000000000, 0.000000000000000000, -1.000000000000000000 ) ) ;
#40838=CARTESIAN_POINT ( 'NONE',  ( 783.7566961878529810, -120.8965053807781800, -305.1792804349288417 ) ) ;
#40845=CARTESIAN_POINT ( 'NONE',  ( 811.6461892240364477, -436.7146871989589272, -324.1737431748509835 ) ) ;
#40847=EDGE_LOOP ( 'NONE', ( #39120, #10978, #27010, #40366 ) ) ;
#40849=CARTESIAN_POINT ( 'NONE',  ( 814.2805881961230625, -385.6454272087888171, -331.2368401574024119 ) ) ;
#40855=CARTESIAN_POINT ( 'NONE',  ( 766.9102291470427417, -210.5545181178800647, -318.6633372737382501 ) ) ;
#40856=CARTESIAN_POINT ( 'NONE',  ( 804.4286716492782716, -233.3618753856925423, -345.3141322388244703 ) ) ;
#40858=CARTESIAN_POINT ( 'NONE',  ( 800.2193346964446619, -426.9982390220555430, -355.1360043628816925 ) ) ;
#40862=CARTESIAN_POINT ( 'NONE',  ( 805.1927285166397041, -112.8164208402383508, -341.8018195045277707 ) ) ;
#40871=CARTESIAN_POINT ( 'NONE',  ( 799.9636004259356241, -430.9181544815157849, -311.2241431872006956 ) ) ;
#40872=CARTESIAN_POINT ( 'NONE',  ( 796.7737145352015204, -44.63460265842040542, -370.7187646348536987 ) ) ;
#40874=CARTESIAN_POINT ( 'NONE',  ( 788.8264449731200330, -405.1800572038737300, -363.6646147819171233 ) ) ;
#40875=CARTESIAN_POINT ( 'NONE',  ( 759.9864689768902508, -26.08914811296592262, -354.9819416627836404 ) ) ;
#40878=CARTESIAN_POINT ( 'NONE',  ( 791.7608162188021197, 205.0000000000000568, -360.0000000000000000 ) ) ;
#40879=CARTESIAN_POINT ( 'NONE',  ( 805.2837595273609850, -290.7363362996980527, -340.5290396650784714 ) ) ;
#40880=CARTESIAN_POINT ( 'NONE',  ( 767.6429770376289525, -153.1800572038746395, -306.8695393053162093 ) ) ;
#40883=CARTESIAN_POINT ( 'NONE',  ( 792.8389451398237497, 16.45630643248849978, -314.6345231965543121 ) ) ;
#40885=CARTESIAN_POINT ( 'NONE',  ( 786.2056067578752163, -227.8055962898687596, -374.4686193811670023 ) ) ;
#40889=CARTESIAN_POINT ( 'NONE',  ( 762.3223304703356007, -367.5436935675102745, -322.3223304703362828 ) ) ;
#40891=CARTESIAN_POINT ( 'NONE',  ( 776.2046728542105711, -116.1908817542440033, -304.8212110874238761 ) ) ;
#40892=CARTESIAN_POINT ( 'NONE',  ( 765.8855110935204493, -142.1692326535054178, -319.0159684113471599 ) ) ;
#40895=CARTESIAN_POINT ( 'NONE',  ( 785.3141322388236176, -69.72551174932942786, -364.4286716492789537 ) ) ;
#40896=CARTESIAN_POINT ( 'NONE',  ( 784.0799538623451781, -155.8055962898689586, -364.6971507214555572 ) ) ;
#40897=CARTESIAN_POINT ( 'NONE',  ( 797.6776695296629214, -115.5436935675110988, -357.6776695296636603 ) ) ;
#40899=CARTESIAN_POINT ( 'NONE',  ( 803.8556311672234642, -9.623778108051251223, -365.6418435158340117 ) ) ;
#40904=CARTESIAN_POINT ( 'NONE',  ( 814.2805881961230625, -265.6454272087889876, -331.2368401574024119 ) ) ;
#40913=CARTESIAN_POINT ( 'NONE',  ( 783.0745993439762742, -128.1908817542439465, -365.1016975059196739 ) ) ;
#40914=CARTESIAN_POINT ( 'NONE',  ( 781.7834795799800531, -106.8164208402383935, -315.0636971347436202 ) ) ;
#40915=CARTESIAN_POINT ( 'NONE',  ( 778.1981804954715471, -322.2709662947830793, -314.8072714833591021 ) ) ;
#40918=CARTESIAN_POINT ( 'NONE',  ( 803.4237431249931660, -423.1800572038737300, -331.2633955100225194 ) ) ;
#40924=CARTESIAN_POINT ( 'NONE',  ( 804.1009440267234822, -359.4636090269705164, -314.0944755984392600 ) ) ;
#40928=CARTESIAN_POINT ( 'NONE',  ( 805.1927285166397041, -304.8164208402376403, -341.8018195045277707 ) ) ;
#40930=CARTESIAN_POINT ( 'NONE',  ( 804.8461984189677878, -194.1908817542437475, -336.9566956441385628 ) ) ;
#40933=CARTESIAN_POINT ( 'NONE',  ( 772.5602148656447525, -393.7255117493283478, -305.7998596910095443 ) ) ;
#40939=CARTESIAN_POINT ( 'NONE',  ( 777.4774526936600978, -34.27096629478407408, -304.7301800767027657 ) ) ;
#40940=CARTESIAN_POINT ( 'NONE',  ( 785.3141322388236176, -261.7255117493288026, -364.4286716492789537 ) ) ;
#40943=AXIS2_PLACEMENT_3D ( 'NONE', #36623, #11904, #11460 ) ;
#40946=CARTESIAN_POINT ( 'NONE',  ( 763.2154366446407039, -45.62377810805114109, -321.4292242960311228 ) ) ;
#40955=CARTESIAN_POINT ( 'NONE',  ( 803.8651313633788504, -341.2601417444138292, -332.4468031744301015 ) ) ;
#40958=CARTESIAN_POINT ( 'NONE',  ( 764.3348316497523456, -358.7146871989592114, -308.6759233522265617 ) ) ;
#40965=CARTESIAN_POINT ( 'NONE',  ( 810.7187646348534145, -234.4527844766016358, -356.7737145352016341 ) ) ;
#40968=CARTESIAN_POINT ( 'NONE',  ( 803.4237431249931660, -183.1800572038744974, -331.2633955100225194 ) ) ;
#40970=CARTESIAN_POINT ( 'NONE',  ( 754.8072714833581358, -316.8164208402377540, -338.1981804954720587 ) ) ;
#40971=CARTESIAN_POINT ( 'NONE',  ( 784.1219089521767955, -453.2817908451519315, -315.0488828828318333 ) ) ;
#40976=CARTESIAN_POINT ( 'NONE',  ( 759.9999999999992042, 205.0000000000000568, -339.9999999999999432 ) ) ;
#40981=CARTESIAN_POINT ( 'NONE',  ( 800.9840315886518738, -412.9181544815157281, -354.1144889064786412 ) ) ;
#40985=CARTESIAN_POINT ( 'NONE',  ( 762.1177392798416577, -234.5545181178799794, -309.8865473780659272 ) ) ;
#40988=CARTESIAN_POINT ( 'NONE',  ( 757.8323909638827445, -194.6346026584198796, -352.1044303154654358 ) ) ;
#40989=CARTESIAN_POINT ( 'NONE',  ( 770.0799878456142551, -373.9874144716864066, -362.9823548866085616 ) ) ;
#40990=CARTESIAN_POINT ( 'NONE',  ( 750.9282345327678740, -208.9181544815164102, -319.8311093483690115 ) ) ;
#40993=CARTESIAN_POINT ( 'NONE',  ( 804.6971507214547046, -75.28179084515321051, -344.0799538623459739 ) ) ;
#40998=CARTESIAN_POINT ( 'NONE',  ( 747.2067596250078623, -267.1800572038742985, -352.2312462859687230 ) ) ;
#41001=CARTESIAN_POINT ( 'NONE',  ( 771.1735550268778070, -57.18005720387489532, -316.3353852180827630 ) ) ;
#41004=CARTESIAN_POINT ( 'NONE',  ( 800.1688906516307043, -154.1692326535053894, -369.0717654672308186 ) ) ;
#41006=CARTESIAN_POINT ( 'NONE',  ( 787.4397851343537695, -405.7255117493283478, -374.2001403089903988 ) ) ;
#41010=CARTESIAN_POINT ( 'NONE',  ( 754.8072714833581358, -436.8164208402372992, -338.1981804954720587 ) ) ;
#41018=CARTESIAN_POINT ( 'NONE',  ( 759.2295555964440155, -208.1692326535051905, -353.9708237608231229 ) ) ;
#41020=CARTESIAN_POINT ( 'NONE',  ( 747.3154664389472828, -259.9874144716869182, -326.4474001241230781 ) ) ;
#41021=DIRECTION ( 'NONE',  ( 0.000000000000000000, 1.110223024625155554E-15, 1.000000000000000000 ) ) ;
#41024=CARTESIAN_POINT ( 'NONE',  ( 764.8639956371174549, -176.0891481129653755, -319.7806653035542013 ) ) ;
#41027=CARTESIAN_POINT ( 'NONE',  ( 811.0346526505616112, -110.6346026584201638, -323.0537975583477532 ) ) ;
#41028=CARTESIAN_POINT ( 'NONE',  ( 774.6858677611749044, -57.72551174932945628, -315.5713283507209894 ) ) ;
#41030=CARTESIAN_POINT ( 'NONE',  ( 779.4763451958990572, -56.73633629969872771, -365.0264073115438919 ) ) ;
#41031=CARTESIAN_POINT ( 'NONE',  ( 757.0176451133909268, -349.0999726633342561, -349.9200121543848354 ) ) ;
#41038=CARTESIAN_POINT ( 'NONE',  ( 769.9779781133707957, -307.0999726633343130, -316.7813123517150871 ) ) ;
#41039=CARTESIAN_POINT ( 'NONE',  ( 755.5713283507202505, -317.3618753856922581, -334.6858677611754729 ) ) ;
#41040=CARTESIAN_POINT ( 'NONE',  ( 768.9521613784389729, -129.8272453906075725, -373.2346286133773106 ) ) ;
#41045=CARTESIAN_POINT ( 'NONE',  ( 755.0488828828309806, -257.8055962898686744, -344.1219089521771934 ) ) ;
#41047=CARTESIAN_POINT ( 'NONE',  ( 762.1177392798416577, -114.5545181178803631, -309.8865473780659272 ) ) ;
#41049=DIRECTION ( 'NONE',  ( -1.000000000000000000, -0.000000000000000000, -0.000000000000000000 ) ) ;
#41053=EDGE_LOOP ( 'NONE', ( #34662, #38894, #36368, #34237 ) ) ;
#41055=CARTESIAN_POINT ( 'NONE',  ( 744.7301800767020268, -172.8164208402381519, -337.4774526936615189 ) ) ;
#41058=CARTESIAN_POINT ( 'NONE',  ( 763.2262854647970016, -296.6346026584195670, -309.2812353651462445 ) ) ;
#41063=CARTESIAN_POINT ( 'NONE',  ( 786.2056067578752163, -347.8055962898683333, -374.4686193811670023 ) ) ;
#41064=CARTESIAN_POINT ( 'NONE',  ( 815.2698199232961542, -112.8164208402383508, -342.5225473063383106 ) ) ;
#41067=CARTESIAN_POINT ( 'NONE',  ( 747.2067596250078623, -387.1800572038738437, -352.2312462859687230 ) ) ;
#41072=VECTOR ( 'NONE', #13035, 1000.000000000000000 ) ;
#41074=CARTESIAN_POINT ( 'NONE',  ( 800.0135310231082713, -230.0891481129652618, -325.0180583372163028 ) ) ;
#41076=CARTESIAN_POINT ( 'NONE',  ( 751.2241431872005251, -160.1692326535053326, -359.9636004259367610 ) ) ;
#41082=CARTESIAN_POINT ( 'NONE',  ( 805.1016975059191054, -6.896505380778533478, -343.0745993439771837 ) ) ;
#41086=CARTESIAN_POINT ( 'NONE',  ( 813.9316612368132837, -439.4419599262316751, -348.6739635108323228 ) ) ;
#41090=CARTESIAN_POINT ( 'NONE',  ( 783.7953271457878373, -368.1908817542433212, -375.1787889125761239 ) ) ;
#41093=CARTESIAN_POINT ( 'NONE',  ( 759.0159684113467620, -232.9181544815163249, -325.8855110935213020 ) ) ;
#41094=CARTESIAN_POINT ( 'NONE',  ( 774.6858677611749044, -201.7255117493290015, -315.5713283507209894 ) ) ;
#41095=CARTESIAN_POINT ( 'NONE',  ( 797.8594530101009923, -421.5436935675101040, -322.1405469898982119 ) ) ;
#41096=VERTEX_POINT ( 'NONE', #20532 ) ;
#41098=CARTESIAN_POINT ( 'NONE',  ( 771.1735550268778070, -105.1800572038747248, -316.3353852180827630 ) ) ;
#41099=VERTEX_POINT ( 'NONE', #6204 ) ;
#41110=CARTESIAN_POINT ( 'NONE',  ( 768.9521613784389729, -441.8272453906066630, -373.2346286133773106 ) ) ;
#41111=CARTESIAN_POINT ( 'NONE',  ( 777.5031285880264704, -70.81642084023850714, -374.9108240113588408 ) ) ;
#41114=CARTESIAN_POINT ( 'NONE',  ( 788.7366044899766848, -419.9073299311465348, -316.5762568750059813 ) ) ;
#41115=CARTESIAN_POINT ( 'NONE',  ( 804.6798772138710092, -39.72551174932951312, -334.6312213355106451 ) ) ;
#41117=CARTESIAN_POINT ( 'NONE',  ( 795.1360043628807261, 3.910851887033985896, -360.2193346964456282 ) ) ;
#41118=CARTESIAN_POINT ( 'NONE',  ( 763.0428371773158460, -275.4636090269708575, -358.7617431975195359 ) ) ;
#41119=CARTESIAN_POINT ( 'NONE',  ( 751.6929314249748586, -198.9982390220562252, -318.8095938919659034 ) ) ;
#41124=CARTESIAN_POINT ( 'NONE',  ( 776.2433038121456548, -228.8965053807778816, -374.8207195650711014 ) ) ;
#41127=CARTESIAN_POINT ( 'NONE',  ( 772.5602148656447525, -297.7255117493286889, -305.7998596910095443 ) ) ;
#41131=CARTESIAN_POINT ( 'NONE',  ( 800.2193346964447755, -354.9982390220557704, -355.1360043628815788 ) ) ;
#41134=CARTESIAN_POINT ( 'NONE',  ( 752.7379699480933368, -84.00906357242590161, -361.9858362298580232 ) ) ;
#41135=CARTESIAN_POINT ( 'NONE',  ( 789.9200121543843807, -169.9874144716871172, -317.0176451133914384 ) ) ;
#41139=CARTESIAN_POINT ( 'NONE',  ( 778.2165204200184689, -70.81642084023850714, -364.9363028652563230 ) ) ;
#41140=CARTESIAN_POINT ( 'NONE',  ( 794.1144889064781864, -154.1692326535053894, -360.9840315886528401 ) ) ;
#41142=CARTESIAN_POINT ( 'NONE',  ( 771.2368401574024119, 10.55804007376686826, -374.2805881961240857 ) ) ;
#41148=CARTESIAN_POINT ( 'NONE',  ( 807.2620300519052989, -288.0090635724252479, -318.0141637701419768 ) ) ;
#41156=CARTESIAN_POINT ( 'NONE',  ( 802.5472867521000353, -100.3726999360622187, -350.8726784830461156 ) ) ;
#41157=CARTESIAN_POINT ( 'NONE',  ( 768.0187753319979720, -104.6346026584202207, -318.0580252608186242 ) ) ;
#41158=CARTESIAN_POINT ( 'NONE',  ( 755.3201227861273992, -315.7255117493286320, -345.3687786644892981 ) ) ;
#41160=CARTESIAN_POINT ( 'NONE',  ( 756.5762568750052424, -435.1800572038737869, -348.7366044899774238 ) ) ;
#41162=DIRECTION ( 'NONE',  ( 0.000000000000000000, 0.000000000000000000, -1.000000000000000000 ) ) ;
#41167=CARTESIAN_POINT ( 'NONE',  ( 811.3240766477731540, -340.3726999360615082, -355.6651683502462902 ) ) ;
#41169=CARTESIAN_POINT ( 'NONE',  ( 768.0187753319979720, -320.6346026584195670, -318.0580252608186242 ) ) ;
#41170=CARTESIAN_POINT ( 'NONE',  ( 799.2566176426618085, -192.0090635724255606, -324.0069404352559559 ) ) ;
#41173=CARTESIAN_POINT ( 'NONE',  ( 751.9810565676468741, -386.0891481129647786, -360.9747183278973921 ) ) ;
#41178=CARTESIAN_POINT ( 'NONE',  ( 754.9967657858570647, -25.54369356751136877, -365.0032342141425374 ) ) ;
#41179=CARTESIAN_POINT ( 'NONE',  ( 774.6312213355099630, -263.3618753856924855, -364.6798772138717482 ) ) ;
#41183=CARTESIAN_POINT ( 'NONE',  ( 805.1016975059191054, -54.89650538077837183, -343.0745993439771837 ) ) ;
#41191=CARTESIAN_POINT ( 'NONE',  ( 771.1735550268778070, -57.18005720387489532, -316.3353852180827630 ) ) ;
#41192=CARTESIAN_POINT ( 'NONE',  ( 754.9735926884551418, -354.3510508353228943, -340.5236548041000333 ) ) ;
#41195=CARTESIAN_POINT ( 'NONE',  ( 748.3538107759620743, -376.7146871989592682, -355.8262568251490165 ) ) ;
#41200=CARTESIAN_POINT ( 'NONE',  ( 751.9810565676468741, -218.0891481129653187, -360.9747183278973921 ) ) ;
#41203=CARTESIAN_POINT ( 'NONE',  ( 756.3353852180820240, -221.9073299311471033, -331.1735550268787733 ) ) ;
#41206=CARTESIAN_POINT ( 'NONE',  ( 774.6858677611749044, -321.7255117493286320, -315.5713283507209894 ) ) ;
#41207=CARTESIAN_POINT ( 'NONE',  ( 796.1575198192839480, -462.0090635724247932, -359.4546378042384163 ) ) ;
#41214=CARTESIAN_POINT ( 'NONE',  ( 805.2837595273609850, -458.7363362996973706, -340.5290396650784714 ) ) ;
#41217=CARTESIAN_POINT ( 'NONE',  ( 805.6418435158337843, -245.4636090269709143, -363.8556311672236916 ) ) ;
#41220=CARTESIAN_POINT ( 'NONE',  ( 764.8639956371174549, -224.0891481129653187, -319.7806653035542013 ) ) ;
#41221=CARTESIAN_POINT ( 'NONE',  ( 755.0488828828309806, -353.8055962898683333, -344.1219089521771934 ) ) ;
#41222=CARTESIAN_POINT ( 'NONE',  ( 773.7305795820266212, -249.2817908451526421, -374.8230680027170365 ) ) ;
#41225=CARTESIAN_POINT ( 'NONE',  ( 769.9779781133707957, -67.09997266333506616, -316.7813123517150871 ) ) ;
#41228=CARTESIAN_POINT ( 'NONE',  ( 815.2698199232962679, -280.8164208402378108, -342.5225473063383674 ) ) ;
#41231=CARTESIAN_POINT ( 'NONE',  ( 781.8018195045266339, -46.27096629478404566, -365.1927285166406705 ) ) ;
#41233=CARTESIAN_POINT ( 'NONE',  ( 756.1443688327750579, -165.6237781080507716, -314.3581564841659315 ) ) ;
#41235=CARTESIAN_POINT ( 'NONE',  ( 808.0189434323515343, -398.0891481129647218, -319.0252816721025511 ) ) ;
#41240=CARTESIAN_POINT ( 'NONE',  ( 804.6798772138708955, -423.7255117493281205, -334.6312213355107019 ) ) ;
#41242=LINE ( 'NONE', #3112, #10680 ) ;
#41247=CARTESIAN_POINT ( 'NONE',  ( 773.3843516231979720, -253.4419599262323572, -364.4086373105754433 ) ) ;
#41249=CARTESIAN_POINT ( 'NONE',  ( 752.4576283171824116, -261.0783235625959264, -317.7880784355627952 ) ) ;
#41255=CARTESIAN_POINT ( 'NONE',  ( 775.9200461376533440, -23.80559628986938847, -315.3028492785443291 ) ) ;
#41256=CARTESIAN_POINT ( 'NONE',  ( 802.1676090361156639, -158.6346026584199933, -327.8955696845344505 ) ) ;
#41258=CARTESIAN_POINT ( 'NONE',  ( 746.8695393053150156, -101.9073299311474727, -327.6429770376306010 ) ) ;
#41259=CARTESIAN_POINT ( 'NONE',  ( 801.9419747391806368, -90.45278447660209054, -351.9812246680014027 ) ) ;
#41261=CARTESIAN_POINT ( 'NONE',  ( 763.0428371773158460, -35.46360902697151829, -358.7617431975195359 ) ) ;
#41262=CARTESIAN_POINT ( 'NONE',  ( 763.8424801807145741, -354.0090635724250774, -320.5453621957614700 ) ) ;
#41270=CARTESIAN_POINT ( 'NONE',  ( 766.0291762391763086, -370.9181544815159555, -360.7704444035551319 ) ) ;
#41271=CARTESIAN_POINT ( 'NONE',  ( 795.1360043628807261, -308.0891481129650629, -360.2193346964456282 ) ) ;
#41272=CARTESIAN_POINT ( 'NONE',  ( 812.3518521366052028, -121.0999726633348956, -326.5853460496235243 ) ) ;
#41277=CARTESIAN_POINT ( 'NONE',  ( 765.8855110935204493, -262.1692326535049347, -319.0159684113471599 ) ) ;
#41278=CARTESIAN_POINT ( 'NONE',  ( 788.6739635108323228, -127.6454272087894140, -373.9316612368139090 ) ) ;
#41284=CARTESIAN_POINT ( 'NONE',  ( 812.7932403749906598, -159.1800572038746111, -327.7687537140311633 ) ) ;
#41286=( BOUNDED_CURVE ( )  B_SPLINE_CURVE ( 2, ( #31222, #6973, #20813, #21058, #17829, #10206, #31897, #38389, #269, #6517, #13680, #39087, #35142 ),
 .UNSPECIFIED., .F., .T. ) 
 B_SPLINE_CURVE_WITH_KNOTS ( ( 3, 2, 2, 2, 2, 2, 3 ),
 ( 0.000000000000000000, 0.0008527428137030668154, 0.003125470086430381933, 0.005398197359157586028, 0.007670924631884902013, 0.009943651904612216264, 0.01049328897333767253 ),
 .UNSPECIFIED. ) 
 CURVE ( )  GEOMETRIC_REPRESENTATION_ITEM ( )  RATIONAL_B_SPLINE_CURVE ( ( 0.4976140944542620792, 0.4980906878130254567, 0.5000002209606652093, 0.4949109396520706139, 0.5000002209606652093, 0.4949109396520706139, 0.5000002209606652093, 0.4949109396520706139, 0.5000002209606652093, 0.4949109396520706139, 0.5000002209606652093, 0.4987694275901001228, 0.4981339451206906466 ) ) 
 REPRESENTATION_ITEM ( '' )  );
#41288=CARTESIAN_POINT ( 'NONE',  ( 787.4397851343537695, -309.7255117493287457, -374.2001403089903988 ) ) ;
#41296=CARTESIAN_POINT ( 'NONE',  ( 805.9055244015594326, -387.6237781080499758, -315.8990559732753240 ) ) ;
#41297=CARTESIAN_POINT ( 'NONE',  ( 747.2067596250078623, -123.1800572038747106, -352.2312462859687230 ) ) ;
#41299=CARTESIAN_POINT ( 'NONE',  ( 796.7737145352015204, -380.6346026584192828, -370.7187646348536987 ) ) ;
#41304=CARTESIAN_POINT ( 'NONE',  ( 801.9858362298568863, -147.0783235625962959, -312.7379699480935642 ) ) ;
#41309=CARTESIAN_POINT ( 'NONE',  ( 798.7617431975189675, -3.623778108051270319, -323.0428371773161871 ) ) ;
#41311=CARTESIAN_POINT ( 'NONE',  ( 759.0252816721024374, -0.9982390220569063999, -368.0189434323527280 ) ) ;
#41315=CARTESIAN_POINT ( 'NONE',  ( 803.4237431249931660, -183.1800572038744974, -331.2633955100225194 ) ) ;
#41316=CARTESIAN_POINT ( 'NONE',  ( 749.5768839229115201, -396.5545181178794678, -358.0661480581553064 ) ) ;
#41317=CARTESIAN_POINT ( 'NONE',  ( 792.1044303154645831, -276.4527844766013800, -317.8323909638837677 ) ) ;
#41320=CARTESIAN_POINT ( 'NONE',  ( 790.9844846989617508, -238.3726999360617640, -317.2208543904092721 ) ) ;
#41321=CARTESIAN_POINT ( 'NONE',  ( 762.3223304703356007, -223.5436935675107577, -322.3223304703362828 ) ) ;
#41322=CARTESIAN_POINT ( 'NONE',  ( 759.7806653035535192, -414.9982390220555430, -324.8639956371181370 ) ) ;
#41327=CARTESIAN_POINT ( 'NONE',  ( 795.8262568251477660, -22.37269993606246743, -308.3538107759623585 ) ) ;
#41333=CARTESIAN_POINT ( 'NONE',  ( 788.6739635108323228, -439.6454272087884760, -373.9316612368139090 ) ) ;
#41334=CARTESIAN_POINT ( 'NONE',  ( 782.5225473063383106, -70.27096629478397460, -375.2698199232970637 ) ) ;
#41336=CARTESIAN_POINT ( 'NONE',  ( 795.1360043628807261, -428.0891481129644944, -360.2193346964456282 ) ) ;
#41337=CARTESIAN_POINT ( 'NONE',  ( 804.4286716492782716, -41.36187538569314626, -345.3141322388244703 ) ) ;
#41340=CARTESIAN_POINT ( 'NONE',  ( 755.8894580844503253, -279.8272453906071746, -332.3691319403863531 ) ) ;
#41341=CARTESIAN_POINT ( 'NONE',  ( 772.4837098697144029, -191.3618753856925991, -374.5518280994205611 ) ) ;
#41347=CARTESIAN_POINT ( 'NONE',  ( 759.8311093483677041, -286.1692326535048778, -310.9282345327691814 ) ) ;
#41349=CARTESIAN_POINT ( 'NONE',  ( 804.7487373415286811, -283.5436935675105019, -364.7487373415288516 ) ) ;
#41353=CARTESIAN_POINT ( 'NONE',  ( 785.3687786644884454, -347.3618753856922012, -315.3201227861279676 ) ) ;
#41355=CARTESIAN_POINT ( 'NONE',  ( 746.0683387631852383, -43.44195992623296831, -331.3260364891676204 ) ) ;
#41356=CARTESIAN_POINT ( 'NONE',  ( 784.0799538623451781, -155.8055962898689586, -364.6971507214555572 ) ) ;
#41362=ORIENTED_EDGE ( 'NONE', *, *, #13125, .T. ) ;
#41363=CARTESIAN_POINT ( 'NONE',  ( 781.8018195045266339, -70.27096629478397460, -365.1927285166406705 ) ) ;
#41364=CARTESIAN_POINT ( 'NONE',  ( 770.0799878456142551, -157.9874144716871456, -362.9823548866085616 ) ) ;
#41365=PRODUCT_DEFINITION_CONTEXT ( 'detailed design', #11927, 'design' ) ;
#41367=CARTESIAN_POINT ( 'NONE',  ( 786.2056067578752163, 12.19440371013049784, -374.4686193811670023 ) ) ;
#41370=CARTESIAN_POINT ( 'NONE',  ( 779.9999999999990905, 18.49609980828599376, -309.9999999999999432 ) ) ;
#41373=CARTESIAN_POINT ( 'NONE',  ( 768.9521613784389729, -321.8272453906070609, -373.2346286133773106 ) ) ;
#41378=CARTESIAN_POINT ( 'NONE',  ( 804.1105419155481968, -99.82724539060768620, -347.6308680596136469 ) ) ;
#41379=CARTESIAN_POINT ( 'NONE',  ( 759.7806653035534055, -126.9982390220565094, -324.8639956371180801 ) ) ;
#41380=CARTESIAN_POINT ( 'NONE',  ( 804.9363028652555840, -304.2709662947832499, -338.2165204200192079 ) ) ;
#41382=CARTESIAN_POINT ( 'NONE',  ( 804.4286716492782716, -425.3618753856919170, -345.3141322388244703 ) ) ;
#41390=CARTESIAN_POINT ( 'NONE',  ( 776.2046728542105711, -332.1908817542433781, -304.8212110874238761 ) ) ;
#41392=CARTESIAN_POINT ( 'NONE',  ( 774.6312213355099630, -311.3618753856922581, -364.6798772138717482 ) ) ;
#41394=CARTESIAN_POINT ( 'NONE',  ( 773.4516893846965786, -187.6454272087892434, -315.8398074228977066 ) ) ;
#41398=CARTESIAN_POINT ( 'NONE',  ( 811.0346526505617248, -374.6346026584193396, -323.0537975583478101 ) ) ;
#41403=CARTESIAN_POINT ( 'NONE',  ( 782.4968714119720516, -10.81642084023869543, -305.0891759886411023 ) ) ;
#41404=CARTESIAN_POINT ( 'NONE',  ( 756.3353852180819104, -245.9073299311469896, -331.1735550268788302 ) ) ;
#41408=CARTESIAN_POINT ( 'NONE',  ( 804.1601925771018387, -55.44195992623293989, -346.5483106153029098 ) ) ;
#41415=CARTESIAN_POINT ( 'NONE',  ( 754.8072714833581358, -76.81642084023845030, -338.1981804954720587 ) ) ;
#41416=CARTESIAN_POINT ( 'NONE',  ( 803.8651313633788504, -365.2601417444137155, -332.4468031744301015 ) ) ;
#41419=CARTESIAN_POINT ( 'NONE',  ( 786.2056067578752163, -371.8055962898682765, -374.4686193811670023 ) ) ;
#41425=CARTESIAN_POINT ( 'NONE',  ( 792.2312462859673587, -227.9073299311471033, -307.2067596250082602 ) ) ;
#41428=CARTESIAN_POINT ( 'NONE',  ( 764.8639956371174549, -200.0891481129653471, -319.7806653035542581 ) ) ;
#41430=CARTESIAN_POINT ( 'NONE',  ( 802.1676090361156639, -326.6346026584193396, -327.8955696845344505 ) ) ;
#41431=CARTESIAN_POINT ( 'NONE',  ( 755.3028492785439312, -447.2817908451521021, -335.9200461376539693 ) ) ;
#41433=CARTESIAN_POINT ( 'NONE',  ( 779.9999999999992042, -452.9681489794448339, -339.9999999999999432 ) ) ;
#41437=CARTESIAN_POINT ( 'NONE',  ( 792.1044303154645831, 11.54721552339760038, -317.8323909638837677 ) ) ;
#41441=CARTESIAN_POINT ( 'NONE',  ( 744.6391490659812007, -254.7363362996981095, -338.7502325331110455 ) ) ;
#41444=CARTESIAN_POINT ( 'NONE',  ( 755.0636971347428243, -220.2709662947834772, -341.7834795799807353 ) ) ;
#41445=CARTESIAN_POINT ( 'NONE',  ( 755.8398074228967971, -379.4419599262318457, -333.4516893846970333 ) ) ;
#41446=CARTESIAN_POINT ( 'NONE',  ( 783.7953271457878373, -248.1908817542435202, -375.1787889125761239 ) ) ;
#41449=CARTESIAN_POINT ( 'NONE',  ( 755.1538015810308480, -86.19088175424408860, -343.0433043558613804 ) ) ;
#41452=CARTESIAN_POINT ( 'NONE',  ( 755.8398074228967971, -427.4419599262317888, -333.4516893846970333 ) ) ;
#41453=CARTESIAN_POINT ( 'NONE',  ( 767.7687537140311633, -287.9073299311468759, -372.7932403749916830 ) ) ;
#41456=CARTESIAN_POINT ( 'NONE',  ( 797.8594530101008786, -61.54369356751124087, -322.1405469898980982 ) ) ;
#41458=CARTESIAN_POINT ( 'NONE',  ( 749.8865473780648472, -164.5328690171416781, -322.1177392798429082 ) ) ;
#41460=CARTESIAN_POINT ( 'NONE',  ( 751.6929314249748586, -414.9982390220555430, -318.8095938919659034 ) ) ;
#41464=CARTESIAN_POINT ( 'NONE',  ( 767.8955696845333705, -432.4527844766008684, -362.1676090361162323 ) ) ;
#41470=CARTESIAN_POINT ( 'NONE',  ( 769.1273215169530886, -262.7146871989594956, -317.4527132478988847 ) ) ;
#41471=CARTESIAN_POINT ( 'NONE',  ( 762.1405469898971887, -121.5436935675110419, -357.8594530101015607 ) ) ;
#41474=CARTESIAN_POINT ( 'NONE',  ( 801.9858362298568863, -267.0783235625958696, -312.7379699480935642 ) ) ;
#41479=CARTESIAN_POINT ( 'NONE',  ( 789.9200121543843807, -49.98741447168749374, -317.0176451133914384 ) ) ;
#41480=CARTESIAN_POINT ( 'NONE',  ( 797.8594530101008786, -157.5436935675108998, -322.1405469898980982 ) ) ;
#41482=CARTESIAN_POINT ( 'NONE',  ( 805.0032342141412300, -109.5436935675110988, -314.9967657858571783 ) ) ;
#41483=CARTESIAN_POINT ( 'NONE',  ( 800.0135310231082713, -110.0891481129656597, -325.0180583372163028 ) ) ;
#41485=CARTESIAN_POINT ( 'NONE',  ( 761.4292242960306112, -41.46360902697149697, -323.2154366446414429 ) ) ;
#41486=CARTESIAN_POINT ( 'NONE',  ( 805.2837595273609850, -338.7363362996978822, -340.5290396650784714 ) ) ;
#41493=CARTESIAN_POINT ( 'NONE',  ( 763.0428371773158460, -347.4636090269705733, -358.7617431975195359 ) ) ;
#41494=CARTESIAN_POINT ( 'NONE',  ( 768.0187753319979720, -344.6346026584195101, -318.0580252608186242 ) ) ;
#41496=CARTESIAN_POINT ( 'NONE',  ( 793.5525998758768083, -127.0999726633348672, -372.6845335610516941 ) ) ;
#41501=CARTESIAN_POINT ( 'NONE',  ( 760.5453621957607311, -261.0783235625959264, -323.8424801807151425 ) ) ;
#41502=CARTESIAN_POINT ( 'NONE',  ( 799.9636004259356241, -166.9181544815165523, -311.2241431872006956 ) ) ;
#41509=CARTESIAN_POINT ( 'NONE',  ( 815.2698199232962679, -184.8164208402381234, -342.5225473063383674 ) ) ;
#41512=CARTESIAN_POINT ( 'NONE',  ( 747.2067596250078623, -315.1800572038740711, -352.2312462859687230 ) ) ;
#41513=DIRECTION ( 'NONE',  ( 0.000000000000000000, 0.000000000000000000, 1.000000000000000000 ) ) ;
#41518=CARTESIAN_POINT ( 'NONE',  ( 815.1787889125755555, -366.8965053807773984, -343.7953271457877804 ) ) ;
#41519=CARTESIAN_POINT ( 'NONE',  ( 805.0032342141412300, -133.5436935675110135, -314.9967657858571783 ) ) ;
#41521=CARTESIAN_POINT ( 'NONE',  ( 792.2312462859673587, -395.9073299311465348, -307.2067596250082602 ) ) ;
#41525=CARTESIAN_POINT ( 'NONE',  ( 793.4146539503750546, -145.9874144716871740, -307.6481478633938877 ) ) ;
#41532=CARTESIAN_POINT ( 'NONE',  ( 782.5225473063381969, 1.729033705215812011, -375.2698199232970637 ) ) ;
#41537=CARTESIAN_POINT ( 'NONE',  ( 773.7305795820266212, -417.2817908451522158, -374.8230680027170365 ) ) ;
#41541=CARTESIAN_POINT ( 'NONE',  ( 786.5483106153019435, -271.6454272087889876, -364.1601925771022366 ) ) ;
#41542=CARTESIAN_POINT ( 'NONE',  ( 774.6312213355099630, -263.3618753856924855, -364.6798772138717482 ) ) ;
#41543=CARTESIAN_POINT ( 'NONE',  ( 756.3353852180820240, -413.9073299311465348, -331.1735550268787733 ) ) ;
#41544=CARTESIAN_POINT ( 'NONE',  ( 805.1927285166397041, -88.81642084023842187, -341.8018195045277707 ) ) ;
#41546=ORIENTED_EDGE ( 'NONE', *, *, #29496, .F. ) ;
#41549=CARTESIAN_POINT ( 'NONE',  ( 773.7305795820266212, -33.28179084515333130, -374.8230680027170365 ) ) ;
#41555=CARTESIAN_POINT ( 'NONE',  ( 802.9823548866075953, -25.09997266333519050, -330.0799878456151077 ) ) ;
#41556=CARTESIAN_POINT ( 'NONE',  ( 744.7301800767020268, -52.81642084023856398, -337.4774526936615189 ) ) ;
#41559=CARTESIAN_POINT ( 'NONE',  ( 774.6858677611749044, -441.7255117493282910, -315.5713283507209894 ) ) ;
#41560=CARTESIAN_POINT ( 'NONE',  ( 759.9864689768902508, -50.08914811296584446, -354.9819416627836404 ) ) ;
#41562=CARTESIAN_POINT ( 'NONE',  ( 763.2262854647970016, -200.6346026584199365, -309.2812353651462445 ) ) ;
#41568=CARTESIAN_POINT ( 'NONE',  ( 778.7502325331095108, -264.3510508353232353, -304.6391490659818828 ) ) ;
#41571=CARTESIAN_POINT ( 'NONE',  ( 814.2001403089898304, -281.3618753856923718, -347.4397851343538264 ) ) ;
#41575=CARTESIAN_POINT ( 'NONE',  ( 785.3141322388236176, -357.7255117493285184, -364.4286716492789537 ) ) ;
#41577=CARTESIAN_POINT ( 'NONE',  ( 781.2497674668890113, -36.35105083532390324, -375.3608509340180603 ) ) ;
#41578=CARTESIAN_POINT ( 'NONE',  ( 772.3691319403857278, -143.2601417444144829, -315.8894580844506663 ) ) ;
#41582=CARTESIAN_POINT ( 'NONE',  ( 759.9864689768902508, -50.08914811296584446, -354.9819416627836404 ) ) ;
#41583=CARTESIAN_POINT ( 'NONE',  ( 794.1144889064781864, -178.1692326535052473, -360.9840315886528401 ) ) ;
#41586=CARTESIAN_POINT ( 'NONE',  ( 764.3348316497523456, 1.285312801039623753, -308.6759233522265617 ) ) ;
#41593=CARTESIAN_POINT ( 'NONE',  ( 749.5768839229115201, -300.5545181178797520, -358.0661480581553064 ) ) ;
#41598=CARTESIAN_POINT ( 'NONE',  ( 804.8461984189677878, -146.1908817542438896, -336.9566956441385628 ) ) ;
#41599=CARTESIAN_POINT ( 'NONE',  ( 767.8955696845333705, -96.45278447660203369, -362.1676090361162323 ) ) ;
#41600=CARTESIAN_POINT ( 'NONE',  ( 801.9419747391806368, -306.4527844766013800, -351.9812246680014027 ) ) ;
#41604=CARTESIAN_POINT ( 'NONE',  ( 791.7608162188021197, 205.0000000000000568, -329.9999999999999432 ) ) ;
#41608=CARTESIAN_POINT ( 'NONE',  ( 807.2620300519052989, -384.0090635724249637, -318.0141637701419768 ) ) ;
#41609=DIRECTION ( 'NONE',  ( -1.000000000000000000, 0.000000000000000000, 0.000000000000000000 ) ) ;
#41612=CARTESIAN_POINT ( 'NONE',  ( 771.2633955100217236, -335.9073299311468190, -363.4237431249939618 ) ) ;
#41614=CARTESIAN_POINT ( 'NONE',  ( 787.4999999999992042, -512.9681489794448908, -370.0000000000000000 ) ) ;
#41615=CARTESIAN_POINT ( 'NONE',  ( 766.9102291470427417, -186.5545181178801215, -318.6633372737382501 ) ) ;
#41619=CARTESIAN_POINT ( 'NONE',  ( 751.6929314249750860, -390.9982390220556567, -318.8095938919659034 ) ) ;
#41624=CARTESIAN_POINT ( 'NONE',  ( 787.4397851343537695, -21.72551174932956641, -374.2001403089903988 ) ) ;
#41625=CARTESIAN_POINT ( 'NONE',  ( 804.6798772138708955, -231.7255117493288310, -334.6312213355107019 ) ) ;
#41629=CARTESIAN_POINT ( 'NONE',  ( 778.7629533639073998, -32.73633629969879877, -375.0009284576466371 ) ) ;
#41630=CARTESIAN_POINT ( 'NONE',  ( 803.2186876482843445, -55.98741447168748664, -350.0220218866286928 ) ) ;
#41640=CARTESIAN_POINT ( 'NONE',  ( 774.6312213355099630, -47.36187538569312494, -364.6798772138717482 ) ) ;
#41643=CARTESIAN_POINT ( 'NONE',  ( 787.6308680596127942, -371.2601417444136587, -364.1105419155492768 ) ) ;
#41647=CARTESIAN_POINT ( 'NONE',  ( 776.2433038121456548, -348.8965053807774552, -374.8207195650711014 ) ) ;
#41654=CARTESIAN_POINT ( 'NONE',  ( 777.5031285880264704, -214.8164208402380666, -374.9108240113588408 ) ) ;
#41658=CARTESIAN_POINT ( 'NONE',  ( 800.0135310231082713, -206.0891481129653471, -325.0180583372163028 ) ) ;
#41659=VECTOR ( 'NONE', #12480, 1000.000000000000000 ) ;
#41661=CARTESIAN_POINT ( 'NONE',  ( 768.0187753319979720, -320.6346026584195670, -318.0580252608186242 ) ) ;
#41662=CARTESIAN_POINT ( 'NONE',  ( 797.6776695296629214, -19.54369356751139364, -357.6776695296636603 ) ) ;
#41668=CARTESIAN_POINT ( 'NONE',  ( 804.4286716492782716, 6.638124614306706306, -345.3141322388244703 ) ) ;
#41670=FACE_OUTER_BOUND ( 'NONE', #30326, .T. ) ;
#41672=CARTESIAN_POINT ( 'NONE',  ( 802.2119215644370342, -246.0090635724253900, -367.5423716828165084 ) ) ;
#41676=CARTESIAN_POINT ( 'NONE',  ( 774.6858677611749044, -225.7255117493289163, -315.5713283507209894 ) ) ;
#41677=CARTESIAN_POINT ( 'NONE',  ( 798.7617431975189675, -387.6237781080499758, -323.0428371773161871 ) ) ;
#41681=CARTESIAN_POINT ( 'NONE',  ( 755.3028492785439312, -87.28179084515316788, -335.9200461376539693 ) ) ;
#41686=CARTESIAN_POINT ( 'NONE',  ( 759.8311093483677041, 25.83076734649409545, -310.9282345327691814 ) ) ;
#41687=CARTESIAN_POINT ( 'NONE',  ( 745.0891759886404770, -268.2709662947833067, -342.4968714119734159 ) ) ;
#41689=CARTESIAN_POINT ( 'NONE',  ( 764.8639956371174549, -80.08914811296574499, -319.7806653035542013 ) ) ;
#41691=CARTESIAN_POINT ( 'NONE',  ( 812.6845335610512393, -175.9874144716871172, -353.5525998758768651 ) ) ;
#41693=CARTESIAN_POINT ( 'NONE',  ( 782.4968714119720516, -418.8164208402374129, -305.0891759886411023 ) ) ;
#41694=DIRECTION ( 'NONE',  ( -0.000000000000000000, 1.110223024625155554E-15, 1.000000000000000000 ) ) ;
#41699=CARTESIAN_POINT ( 'NONE',  ( 802.1676090361156639, -422.6346026584192259, -327.8955696845344505 ) ) ;
#41703=CARTESIAN_POINT ( 'NONE',  ( 799.9999999999993179, -512.9681489794448908, -339.9999999999999432 ) ) ;
#41707=CARTESIAN_POINT ( 'NONE',  ( 765.8855110935204493, -262.1692326535049347, -319.0159684113471599 ) ) ;
#41709=CARTESIAN_POINT ( 'NONE',  ( 746.7653713866222915, -257.2601417444141134, -351.0478386215610271 ) ) ;
#41714=CARTESIAN_POINT ( 'NONE',  ( 773.3843516231979720, -37.44195992623299674, -364.4086373105754433 ) ) ;
#41715=CARTESIAN_POINT ( 'NONE',  ( 781.7834795799800531, -178.8164208402381519, -315.0636971347436202 ) ) ;
#41719=CARTESIAN_POINT ( 'NONE',  ( 751.9810565676468741, -122.0891481129656171, -360.9747183278973921 ) ) ;
#41720=CARTESIAN_POINT ( 'NONE',  ( 758.0580252608178853, -102.4527844766020337, -328.0187753319985404 ) ) ;
#41721=ORIENTED_EDGE ( 'NONE', *, *, #7796, .T. ) ;
#41722=CARTESIAN_POINT ( 'NONE',  ( 757.0176451133909268, -37.09997266333514432, -349.9200121543848354 ) ) ;
#41723=CARTESIAN_POINT ( 'NONE',  ( 759.0159684113467620, -352.9181544815159555, -325.8855110935213020 ) ) ;
#41728=DIRECTION ( 'NONE',  ( 0.000000000000000000, 0.000000000000000000, 1.000000000000000000 ) ) ;
#41730=CARTESIAN_POINT ( 'NONE',  ( 763.8424801807145741, -354.0090635724250774, -320.5453621957614700 ) ) ;
#41731=CARTESIAN_POINT ( 'NONE',  ( 785.3687786644884454, -347.3618753856922012, -315.3201227861279676 ) ) ;
#41732=CARTESIAN_POINT ( 'NONE',  ( 783.7953271457878373, -128.1908817542439465, -375.1787889125761239 ) ) ;
#41737=CARTESIAN_POINT ( 'NONE',  ( 758.6633372737375112, -308.5328690171412518, -326.9102291470432533 ) ) ;
#41738=CARTESIAN_POINT ( 'NONE',  ( 750.9282345327678740, -136.9181544815166376, -319.8311093483690115 ) ) ;
#41744=CARTESIAN_POINT ( 'NONE',  ( 801.1904061080338124, -164.0891481129654892, -368.3070685750236066 ) ) ;
#41748=CARTESIAN_POINT ( 'NONE',  ( 772.4837098697144029, -287.3618753856923718, -374.5518280994205611 ) ) ;
#41757=CARTESIAN_POINT ( 'NONE',  ( 781.2497674668890113, -372.3510508353228374, -375.3608509340180603 ) ) ;
#41758=CARTESIAN_POINT ( 'NONE',  ( 815.2698199232961542, -136.8164208402382371, -342.5225473063383106 ) ) ;
#41760=CARTESIAN_POINT ( 'NONE',  ( 804.7487373415286811, -379.5436935675102745, -364.7487373415288516 ) ) ;
#41764=CARTESIAN_POINT ( 'NONE',  ( 805.9055244015594326, -147.6237781080508285, -315.8990559732753240 ) ) ;
#41772=CARTESIAN_POINT ( 'NONE',  ( 787.4397851343537695, 2.274488250670355871, -374.2001403089903988 ) ) ;
#41778=CARTESIAN_POINT ( 'NONE',  ( 800.2193346964447755, -258.9982390220561115, -355.1360043628815788 ) ) ;
#41782=CARTESIAN_POINT ( 'NONE',  ( 800.9840315886518738, -268.9181544815162397, -354.1144889064786412 ) ) ;
#41783=CARTESIAN_POINT ( 'NONE',  ( 771.2633955100217236, -239.9073299311470748, -363.4237431249939618 ) ) ;
#41784=CARTESIAN_POINT ( 'NONE',  ( 791.9812246680005501, -404.6346026584193396, -361.9419747391813189 ) ) ;
#41785=CARTESIAN_POINT ( 'NONE',  ( 774.6858677611749044, -81.72551174932937101, -315.5713283507209894 ) ) ;
#41790=CARTESIAN_POINT ( 'NONE',  ( 766.4474001241216001, -43.09997266333511590, -307.3154664389482491 ) ) ;
#41796=CARTESIAN_POINT ( 'NONE',  ( 804.4086373105744769, -1.645427208789804308, -333.3843516231986541 ) ) ;
#41797=CARTESIAN_POINT ( 'NONE',  ( 812.7932403749906598, -87.18005720387481006, -327.7687537140311633 ) ) ;
#41799=AXIS2_PLACEMENT_3D ( 'NONE', #39816, #36320, #15754 ) ;
#41800=CARTESIAN_POINT ( 'NONE',  ( 768.0187753319979720, -440.6346026584191122, -318.0580252608186242 ) ) ;
#41801=CARTESIAN_POINT ( 'NONE',  ( 757.8323909638828582, -50.63460265842038410, -352.1044303154654358 ) ) ;
#41803=CARTESIAN_POINT ( 'NONE',  ( 759.0252816721024374, -192.9982390220562820, -368.0189434323527280 ) ) ;
#41807=LINE ( 'NONE', #30473, #35054 ) ;
#41809=CARTESIAN_POINT ( 'NONE',  ( 815.0009284576459549, -270.3510508353231216, -338.7629533639073429 ) ) ;
#41812=CARTESIAN_POINT ( 'NONE',  ( 805.0032342141412300, -277.5436935675105019, -314.9967657858571783 ) ) ;
#41816=CARTESIAN_POINT ( 'NONE',  ( 797.6776695296629214, -379.5436935675102745, -357.6776695296636603 ) ) ;
#41819=CARTESIAN_POINT ( 'NONE',  ( 751.2241431872005251, -64.16923265350563099, -359.9636004259367610 ) ) ;
#41820=CARTESIAN_POINT ( 'NONE',  ( 770.0799878456142551, -181.9874144716870887, -362.9823548866085616 ) ) ;
#41824=CARTESIAN_POINT ( 'NONE',  ( 778.2165204200184689, -46.81642084023858530, -364.9363028652563230 ) ) ;
#41825=CARTESIAN_POINT ( 'NONE',  ( 803.2186876482843445, -199.9874144716870603, -350.0220218866286928 ) ) ;
#41827=CARTESIAN_POINT ( 'NONE',  ( 756.1443688327750579, 2.376221891948710585, -314.3581564841659315 ) ) ;
#41832=CARTESIAN_POINT ( 'NONE',  ( 755.8990559732751535, -299.4636090269707438, -365.9055244015606831 ) ) ;
#41838=CARTESIAN_POINT ( 'NONE',  ( 761.4292242960306112, -137.4636090269711985, -323.2154366446414429 ) ) ;
#41839=CARTESIAN_POINT ( 'NONE',  ( 803.6646147819161570, -137.9073299311473875, -348.8264449731210561 ) ) ;
#41840=CARTESIAN_POINT ( 'NONE',  ( 792.1044303154646968, -300.4527844766013231, -317.8323909638837677 ) ) ;
#41848=CARTESIAN_POINT ( 'NONE',  ( 745.5313806188320314, -375.2817908451523294, -333.7943932421247268 ) ) ;
#41852=CARTESIAN_POINT ( 'NONE',  ( 757.8323909638827445, -314.6346026584194533, -352.1044303154654358 ) ) ;
#41854=CARTESIAN_POINT ( 'NONE',  ( 755.3028492785439312, -207.2817908451527842, -335.9200461376539693 ) ) ;
#41858=CARTESIAN_POINT ( 'NONE',  ( 814.5518280994195948, -423.7255117493282341, -332.4837098697145166 ) ) ;
#41863=CARTESIAN_POINT ( 'NONE',  ( 812.7932403749906598, -63.18005720387488822, -327.7687537140311633 ) ) ;
#41865=CARTESIAN_POINT ( 'NONE',  ( 759.7806653035534055, -270.9982390220561115, -324.8639956371180801 ) ) ;
#41869=CARTESIAN_POINT ( 'NONE',  ( 795.8262568251477660, -22.37269993606246743, -308.3538107759623585 ) ) ;
#41870=CARTESIAN_POINT ( 'NONE',  ( 773.3843516231979720, -37.44195992623299674, -364.4086373105754433 ) ) ;
#41877=CARTESIAN_POINT ( 'NONE',  ( 781.7834795799800531, -58.81642084023854267, -315.0636971347436202 ) ) ;
#41878=CARTESIAN_POINT ( 'NONE',  ( 756.1348686366196716, -353.2601417444137724, -347.5531968255698416 ) ) ;
#41881=CARTESIAN_POINT ( 'NONE',  ( 814.8230680027162407, -389.8055962898682765, -333.7305795820267917 ) ) ;
#41887=CARTESIAN_POINT ( 'NONE',  ( 772.4837098697144029, -215.3618753856925423, -374.5518280994205611 ) ) ;
#41890=CARTESIAN_POINT ( 'NONE',  ( 771.2633955100217236, -215.9073299311471317, -363.4237431249939618 ) ) ;
#41892=CARTESIAN_POINT ( 'NONE',  ( 804.9363028652555840, -352.2709662947830225, -338.2165204200192079 ) ) ;
#41893=CARTESIAN_POINT ( 'NONE',  ( 785.3141322388236176, -21.72551174932956641, -364.4286716492789537 ) ) ;
#41898=CARTESIAN_POINT ( 'NONE',  ( 774.6312213355099630, 0.6381246143067236254, -364.6798772138717482 ) ) ;
#41899=CARTESIAN_POINT ( 'NONE',  ( 791.4804426738954817, -453.0432664090020580, -367.7164109511201673 ) ) ;
#41902=CARTESIAN_POINT ( 'NONE',  ( 814.2805881961230625, -289.6454272087889308, -331.2368401574024119 ) ) ;
#41906=CARTESIAN_POINT ( 'NONE',  ( 781.8018195045266339, -214.2709662947834488, -365.1927285166406705 ) ) ;
#41908=CARTESIAN_POINT ( 'NONE',  ( 805.1016975059191054, -390.8965053807772279, -343.0745993439771837 ) ) ;
#41909=CARTESIAN_POINT ( 'NONE',  ( 779.9999999999992042, 126.4563064324884465, -339.9999999999999432 ) ) ;
#41910=CARTESIAN_POINT ( 'NONE',  ( 802.1676090361155502, 9.365397341579424051, -327.8955696845344505 ) ) ;
#41911=CARTESIAN_POINT ( 'NONE',  ( 763.0428371773158460, -107.4636090269713122, -358.7617431975195359 ) ) ;
#41915=CARTESIAN_POINT ( 'NONE',  ( 773.7943932421234194, 0.1944037101305369775, -305.5313806188329409 ) ) ;
#41916=CARTESIAN_POINT ( 'NONE',  ( 792.3570229623691148, -309.1800572038740711, -373.1304606946836770 ) ) ;
#41919=CARTESIAN_POINT ( 'NONE',  ( 781.8018195045266339, -70.27096629478397460, -365.1927285166406705 ) ) ;
#41921=CARTESIAN_POINT ( 'NONE',  ( 771.2368401574024119, -181.4419599262325278, -374.2805881961240857 ) ) ;
#41923=CARTESIAN_POINT ( 'NONE',  ( 807.2620300519052989, -0.009063572426172561425, -318.0141637701419768 ) ) ;
#41929=CARTESIAN_POINT ( 'NONE',  ( 755.0636971347428243, -436.2709662947827951, -341.7834795799807353 ) ) ;
#41935=CARTESIAN_POINT ( 'NONE',  ( 766.7756240680305382, -254.5328690171413655, -361.5560724626415663 ) ) ;
#41937=CARTESIAN_POINT ( 'NONE',  ( 805.9055244015594326, -243.6237781080504590, -315.8990559732753240 ) ) ;
#41945=CARTESIAN_POINT ( 'NONE',  ( 784.0799538623451781, -35.80559628986934229, -364.6971507214555572 ) ) ;
#41946=CARTESIAN_POINT ( 'NONE',  ( 797.8594530101008786, -157.5436935675108998, -322.1405469898980982 ) ) ;
#41947=CARTESIAN_POINT ( 'NONE',  ( 797.6776695296629214, -211.5436935675107861, -357.6776695296636603 ) ) ;
#41949=CARTESIAN_POINT ( 'NONE',  ( 746.8695393053150156, -125.9073299311474159, -327.6429770376306010 ) ) ;
#41950=CARTESIAN_POINT ( 'NONE',  ( 803.6646147819162707, -89.90732993114752958, -348.8264449731211130 ) ) ;
#41952=CARTESIAN_POINT ( 'NONE',  ( 801.5560724626406000, -48.55451811788057626, -326.7756240680316182 ) ) ;
#41953=CARTESIAN_POINT ( 'NONE',  ( 801.5560724626406000, -384.5545181178795247, -326.7756240680316182 ) ) ;
#41961=CARTESIAN_POINT ( 'NONE',  ( 776.9254006560222479, -356.1908817542432075, -314.8983024940802125 ) ) ;
#41962=CARTESIAN_POINT ( 'NONE',  ( 792.1044303154645831, -348.4527844766012663, -317.8323909638837677 ) ) ;
#41963=CARTESIAN_POINT ( 'NONE',  ( 749.5768839229115201, -156.5545181178802636, -358.0661480581553064 ) ) ;
#41969=CARTESIAN_POINT ( 'NONE',  ( 803.2186876482843445, -295.9874144716866908, -350.0220218866286928 ) ) ;
#41970=CARTESIAN_POINT ( 'NONE',  ( 764.8639956371174549, -440.0891481129644944, -319.7806653035542013 ) ) ;
#41971=CARTESIAN_POINT ( 'NONE',  ( 786.2694204179717872, -141.2817908451530400, -305.1769319972829067 ) ) ;
#41977=CARTESIAN_POINT ( 'NONE',  ( 751.9810565676468741, -170.0891481129654608, -360.9747183278973921 ) ) ;
#41981=CARTESIAN_POINT ( 'NONE',  ( 745.4481719005789273, -291.7255117493285752, -347.5162901302853129 ) ) ;
#41986=CARTESIAN_POINT ( 'NONE',  ( 778.7502325331095108, -384.3510508353227806, -304.6391490659818828 ) ) ;
#41987=CARTESIAN_POINT ( 'NONE',  ( 814.2001403089898304, -113.3618753856929260, -347.4397851343538264 ) ) ;
#41988=CARTESIAN_POINT ( 'NONE',  ( 808.3070685750230950, -378.9982390220555999, -361.1904061080339261 ) ) ;
#41992=CARTESIAN_POINT ( 'NONE',  ( 748.3538107759620743, -160.7146871989598651, -355.8262568251490165 ) ) ;
#41998=CARTESIAN_POINT ( 'NONE',  ( 811.0346526505616112, -14.63460265842049424, -323.0537975583477532 ) ) ;
#42001=CARTESIAN_POINT ( 'NONE',  ( 750.9282345327678740, -400.9181544815159555, -319.8311093483690115 ) ) ;
#42005=CARTESIAN_POINT ( 'NONE',  ( 795.1360043628807261, -260.0891481129650060, -360.2193346964456282 ) ) ;
#42008=CARTESIAN_POINT ( 'NONE',  ( 769.9779781133707957, -259.0999726633343698, -316.7813123517150871 ) ) ;
#42009=CARTESIAN_POINT ( 'NONE',  ( 804.4286716492782716, -257.3618753856924286, -345.3141322388244703 ) ) ;
#42010=CARTESIAN_POINT ( 'NONE',  ( 801.9419747391806368, -450.4527844766009821, -351.9812246680014027 ) ) ;
#42011=CARTESIAN_POINT ( 'NONE',  ( 765.0180583372156207, -96.99823902205660886, -360.0135310231089534 ) ) ;
#42015=CARTESIAN_POINT ( 'NONE',  ( 773.7305795820266212, -57.28179084515326736, -374.8230680027170365 ) ) ;
#42021=CARTESIAN_POINT ( 'NONE',  ( 804.1105419155481968, -3.827245390607979303, -347.6308680596136469 ) ) ;
#42022=CARTESIAN_POINT ( 'NONE',  ( 772.5602148656447525, -57.72551174932945628, -305.7998596910095443 ) ) ;
#42026=CARTESIAN_POINT ( 'NONE',  ( 804.7487373415286811, -211.5436935675107861, -364.7487373415288516 ) ) ;
#42030=CARTESIAN_POINT ( 'NONE',  ( 793.4146539503750546, -265.9874144716867477, -307.6481478633938877 ) ) ;
#42032=CARTESIAN_POINT ( 'NONE',  ( 745.7998596910086917, -269.3618753856924286, -332.5602148656461168 ) ) ;
#42036=CARTESIAN_POINT ( 'NONE',  ( 815.1787889125755555, -30.89650538077846065, -343.7953271457877804 ) ) ;
#42037=CARTESIAN_POINT ( 'NONE',  ( 755.3201227861273992, -387.7255117493283478, -345.3687786644892981 ) ) ;
#42039=CARTESIAN_POINT ( 'NONE',  ( 804.6798772138708955, -207.7255117493289447, -334.6312213355107019 ) ) ;
#42040=CARTESIAN_POINT ( 'NONE',  ( 811.6461892240364477, -52.71468719896020616, -324.1737431748509835 ) ) ;
#42041=CARTESIAN_POINT ( 'NONE',  ( 801.3366627262608972, -200.5328690171415644, -353.0897708529566899 ) ) ;
#42045=CARTESIAN_POINT ( 'NONE',  ( 787.6308680596127942, -203.2601417444143124, -364.1105419155492768 ) ) ;
#42047=CARTESIAN_POINT ( 'NONE',  ( 745.1769319972822814, -17.80559628986940979, -346.2694204179732083 ) ) ;
#42052=CARTESIAN_POINT ( 'NONE',  ( 766.4474001241216001, -307.0999726633343130, -307.3154664389482491 ) ) ;
#42056=CARTESIAN_POINT ( 'NONE',  ( 796.1575198192839480, -150.0090635724257027, -359.4546378042384163 ) ) ;
#42057=CARTESIAN_POINT ( 'NONE',  ( 757.8323909638827445, -146.6346026584200217, -352.1044303154654358 ) ) ;
#42058=CARTESIAN_POINT ( 'NONE',  ( 792.1044303154646968, -348.4527844766012095, -317.8323909638837677 ) ) ;
#42065=ORIENTED_EDGE ( 'NONE', *, *, #37315, .F. ) ;
#42066=CARTESIAN_POINT ( 'NONE',  ( 744.6391490659812007, -374.7363362996978253, -338.7502325331110455 ) ) ;
#42070=CARTESIAN_POINT ( 'NONE',  ( 797.8594530101008786, -325.5436935675105019, -322.1405469898980982 ) ) ;
#42072=CARTESIAN_POINT ( 'NONE',  ( 780.5236548040995785, -212.7363362996982232, -314.9735926884559944 ) ) ;
#42076=CARTESIAN_POINT ( 'NONE',  ( 763.0537975583476964, -408.4527844766009821, -371.0346526505628617 ) ) ;
#42081=CARTESIAN_POINT ( 'NONE',  ( 787.4397851343537695, -69.72551174932942786, -374.2001403089903988 ) ) ;
#42082=CARTESIAN_POINT ( 'NONE',  ( 788.7366044899766848, -299.9073299311468759, -316.5762568750059813 ) ) ;
#42086=CARTESIAN_POINT ( 'NONE',  ( 793.5525998758768083, -31.09997266333516919, -372.6845335610516941 ) ) ;
#42087=CARTESIAN_POINT ( 'NONE',  ( 789.9200121543843807, -73.98741447168741558, -317.0176451133914384 ) ) ;
#42092=CARTESIAN_POINT ( 'NONE',  ( 774.6858677611749044, -9.725511749329603717, -315.5713283507209894 ) ) ;
#42093=CARTESIAN_POINT ( 'NONE',  ( 783.0433043558608688, -96.89650538077825104, -315.1538015810313027 ) ) ;
#42095=CARTESIAN_POINT ( 'NONE',  ( 774.6858677611749044, -57.72551174932945628, -315.5713283507209894 ) ) ;
#42096=CARTESIAN_POINT ( 'NONE',  ( 755.0488828828309806, -377.8055962898682765, -344.1219089521771934 ) ) ;
#42100=CARTESIAN_POINT ( 'NONE',  ( 764.3348316497523456, -406.7146871989590409, -308.6759233522265617 ) ) ;
#42104=EDGE_LOOP ( 'NONE', ( #18675, #6018 ) ) ;
#42105=CARTESIAN_POINT ( 'NONE',  ( 804.7487373415286811, -235.5436935675107293, -364.7487373415288516 ) ) ;
#42108=CARTESIAN_POINT ( 'NONE',  ( 804.4286716492782716, -233.3618753856925423, -345.3141322388244703 ) ) ;
#42110=CARTESIAN_POINT ( 'NONE',  ( 758.0580252608178853, -366.4527844766012095, -328.0187753319985404 ) ) ;
#42111=CARTESIAN_POINT ( 'NONE',  ( 756.5762568750052424, -3.180057203875080063, -348.7366044899774238 ) ) ;
#42117=CARTESIAN_POINT ( 'NONE',  ( 759.7806653035534055, -30.99823902205680071, -324.8639956371180801 ) ) ;
#42121=CARTESIAN_POINT ( 'NONE',  ( 768.9521613784389729, -273.8272453906071746, -373.2346286133773106 ) ) ;
#42124=CARTESIAN_POINT ( 'NONE',  ( 788.8264449731200330, -237.1800572038742985, -363.6646147819171233 ) ) ;
#42125=CARTESIAN_POINT ( 'NONE',  ( 764.0069404352550464, -399.0783235625955285, -359.2566176426627180 ) ) ;
#42128=CARTESIAN_POINT ( 'NONE',  ( 772.4468031744293057, -105.8272453906076578, -363.8651313633793620 ) ) ;
#42131=CARTESIAN_POINT ( 'NONE',  ( 813.2346286133761168, 18.73985825558501972, -328.9521613784389160 ) ) ;
#42132=CARTESIAN_POINT ( 'NONE',  ( 814.9108240113580450, -304.2709662947832499, -337.5031285880265273 ) ) ;
#42135=CARTESIAN_POINT ( 'NONE',  ( 785.3141322388236176, -69.72551174932942786, -364.4286716492789537 ) ) ;
#42137=CARTESIAN_POINT ( 'NONE',  ( 749.8865473780648472, -188.5328690171416497, -322.1177392798429082 ) ) ;
#42139=CARTESIAN_POINT ( 'NONE',  ( 808.0189434323515343, -446.0891481129646081, -319.0252816721025511 ) ) ;
#42140=DIRECTION ( 'NONE',  ( 0.000000000000000000, -1.000000000000000000, 0.000000000000000000 ) ) ;
#42144=CARTESIAN_POINT ( 'NONE',  ( 789.5670355615794733, -453.0432664090020012, -363.0970091259334822 ) ) ;
#42150=CARTESIAN_POINT ( 'NONE',  ( 794.1144889064781864, -274.1692326535049915, -360.9840315886528401 ) ) ;
#42152=CARTESIAN_POINT ( 'NONE',  ( 745.1769319972822814, -281.8055962898686175, -346.2694204179732083 ) ) ;
#42157=CARTESIAN_POINT ( 'NONE',  ( 761.2382568024794409, -39.62377810805116951, -356.9571628226838129 ) ) ;
#42158=CARTESIAN_POINT ( 'NONE',  ( 759.7806653035534055, -198.9982390220562252, -324.8639956371180801 ) ) ;
#42161=CARTESIAN_POINT ( 'NONE',  ( 796.7737145352015204, -140.6346026584201070, -370.7187646348536987 ) ) ;
#42163=CARTESIAN_POINT ( 'NONE',  ( 757.8323909638828582, -98.63460265842023489, -352.1044303154654358 ) ) ;
#42165=CARTESIAN_POINT ( 'NONE',  ( 769.0155153010367712, -394.3726999360613377, -362.7791456095907279 ) ) ;
#42175=CARTESIAN_POINT ( 'NONE',  ( 755.1538015810308480, -350.1908817542433212, -343.0433043558613804 ) ) ;
#42176=CARTESIAN_POINT ( 'NONE',  ( 759.7806653035534055, -366.9982390220556567, -324.8639956371180801 ) ) ;
#42177=CARTESIAN_POINT ( 'NONE',  ( 766.4474001241216001, -163.0999726633347677, -307.3154664389482491 ) ) ;
#42181=CARTESIAN_POINT ( 'NONE',  ( 757.2208543904082489, -280.7146871989594956, -350.9844846989624330 ) ) ;
#42182=CARTESIAN_POINT ( 'NONE',  ( 771.1735550268778070, -441.1800572038735027, -316.3353852180827630 ) ) ;
#42183=CARTESIAN_POINT ( 'NONE',  ( 746.4236121716829757, -159.8272453906075157, -328.8385539511384650 ) ) ;
#42184=FACE_OUTER_BOUND ( 'NONE', #42104, .T. ) ;
#42188=CARTESIAN_POINT ( 'NONE',  ( 814.9108240113580450, -208.2709662947835341, -337.5031285880265273 ) ) ;
#42194=CARTESIAN_POINT ( 'NONE',  ( 754.0944755984390895, -111.6237781080509279, -364.1009440267246760 ) ) ;
#42195=CARTESIAN_POINT ( 'NONE',  ( 767.7687537140311633, -335.9073299311468190, -372.7932403749916830 ) ) ;
#42202=CARTESIAN_POINT ( 'NONE',  ( 758.0141637701419768, -375.0783235625955285, -367.2620300519063790 ) ) ;
#42203=CARTESIAN_POINT ( 'NONE',  ( 745.4481719005789273, -147.7255117493291152, -347.5162901302853129 ) ) ;
#42204=CARTESIAN_POINT ( 'NONE',  ( 749.2812353651451076, -438.4527844766009821, -323.2262854647983090 ) ) ;
#42208=CARTESIAN_POINT ( 'NONE',  ( 744.8212110874229666, -186.8965053807779668, -336.2046728542121627 ) ) ;
#42216=CARTESIAN_POINT ( 'NONE',  ( 813.1304606946830518, -17.90732993114776406, -352.3570229623690580 ) ) ;
#42220=CARTESIAN_POINT ( 'NONE',  ( 814.8207195650702488, -410.1908817542430370, -336.2433038121456548 ) ) ;
#42222=CARTESIAN_POINT ( 'NONE',  ( 785.3687786644884454, -275.3618753856923149, -315.3201227861279676 ) ) ;
#42226=EDGE_CURVE ( 'NONE', #43683, #34870, #45188, .T. ) ;
#42227=CARTESIAN_POINT ( 'NONE',  ( 755.5913626894240451, -253.6454272087889876, -346.6156483768012890 ) ) ;
#42228=CARTESIAN_POINT ( 'NONE',  ( 788.8264449731200330, -237.1800572038742985, -363.6646147819171233 ) ) ;
#42230=CARTESIAN_POINT ( 'NONE',  ( 758.0580252608178853, -102.4527844766020337, -328.0187753319985404 ) ) ;
#42234=DIRECTION ( 'NONE',  ( 0.000000000000000000, -1.000000000000000000, 0.000000000000000000 ) ) ;
#42235=CARTESIAN_POINT ( 'NONE',  ( 797.8822607201568644, -54.55451811788054783, -370.1134526219340160 ) ) ;
#42241=CARTESIAN_POINT ( 'NONE',  ( 804.4086373105744769, -25.64542720878973014, -333.3843516231986541 ) ) ;
#42242=CARTESIAN_POINT ( 'NONE',  ( 800.9747183278959710, -108.9982390220565804, -311.9810565676471583 ) ) ;
#42244=CARTESIAN_POINT ( 'NONE',  ( 801.9419747391806368, -450.4527844766009821, -351.9812246680014027 ) ) ;
#42246=CARTESIAN_POINT ( 'NONE',  ( 782.4968714119720516, -250.8164208402379245, -305.0891759886411023 ) ) ;
#42251=CARTESIAN_POINT ( 'NONE',  ( 771.2368401574024119, -277.4419599262322436, -374.2805881961240857 ) ) ;
#42253=CARTESIAN_POINT ( 'NONE',  ( 787.4397851343537695, -333.7255117493286320, -374.2001403089903988 ) ) ;
#42257=CARTESIAN_POINT ( 'NONE',  ( 788.8264449731200330, -381.1800572038737869, -363.6646147819171233 ) ) ;
#42259=CARTESIAN_POINT ( 'NONE',  ( 798.0661480581538854, -50.53286901714203339, -309.5768839229118043 ) ) ;
#42264=CARTESIAN_POINT ( 'NONE',  ( 795.9930595647434757, -195.0783235625961538, -320.7433823573372820 ) ) ;
#42266=CARTESIAN_POINT ( 'NONE',  ( 776.2433038121456548, -36.89650538077844288, -374.8207195650711014 ) ) ;
#42271=CARTESIAN_POINT ( 'NONE',  ( 814.2805881961230625, -313.6454272087888171, -331.2368401574024119 ) ) ;
#42274=CARTESIAN_POINT ( 'NONE',  ( 755.1538015810308480, -158.1908817542438612, -343.0433043558613804 ) ) ;
#42275=CARTESIAN_POINT ( 'NONE',  ( 767.8955696845333705, -144.4527844766018632, -362.1676090361162323 ) ) ;
#42277=CARTESIAN_POINT ( 'NONE',  ( 771.2633955100217236, -335.9073299311468190, -363.4237431249939618 ) ) ;
#42286=CARTESIAN_POINT ( 'NONE',  ( 813.5763878283155464, -363.8272453906068336, -351.1614460488615350 ) ) ;
#42287=CARTESIAN_POINT ( 'NONE',  ( 782.4968714119720516, -10.81642084023869543, -305.0891759886411023 ) ) ;
#42290=CARTESIAN_POINT ( 'NONE',  ( 794.9819416627830151, -372.9982390220557704, -319.9864689768909898 ) ) ;
#42293=CARTESIAN_POINT ( 'NONE',  ( 759.0159684113467620, -232.9181544815163249, -325.8855110935213020 ) ) ;
#42297=CARTESIAN_POINT ( 'NONE',  ( 746.8695393053151292, -413.9073299311465348, -327.6429770376306578 ) ) ;
#42302=CARTESIAN_POINT ( 'NONE',  ( 754.9967657858570647, -49.54369356751129061, -365.0032342141425374 ) ) ;
#42303=CARTESIAN_POINT ( 'NONE',  ( 802.1676090361156639, -278.6346026584196807, -327.8955696845344505 ) ) ;
#42307=CARTESIAN_POINT ( 'NONE',  ( 745.1792804349281596, -14.19088175424431242, -343.7566961878542884 ) ) ;
#42308=CARTESIAN_POINT ( 'NONE',  ( 758.6633372737375112, -68.53286901714197654, -326.9102291470432533 ) ) ;
#42313=CARTESIAN_POINT ( 'NONE',  ( 800.2193346964447755, 5.001760977943074948, -355.1360043628815788 ) ) ;
#42314=ORIENTED_EDGE ( 'NONE', *, *, #44997, .T. ) ;
#42315=CARTESIAN_POINT ( 'NONE',  ( 800.2193346964447755, -90.99823902205663728, -355.1360043628815788 ) ) ;
#42316=CARTESIAN_POINT ( 'NONE',  ( 770.0799878456142551, -397.9874144716864066, -362.9823548866085616 ) ) ;
#42319=CARTESIAN_POINT ( 'NONE',  ( 761.9338519418445230, -398.5328690171409107, -370.4231160770881957 ) ) ;
#42326=CARTESIAN_POINT ( 'NONE',  ( 763.2262854647970016, -248.6346026584197659, -309.2812353651462445 ) ) ;
#42329=CARTESIAN_POINT ( 'NONE',  ( 762.3223304703356007, -247.5436935675106724, -322.3223304703362828 ) ) ;
#42331=CARTESIAN_POINT ( 'NONE',  ( 755.0636971347428243, -364.2709662947830793, -341.7834795799807353 ) ) ;
#42332=CARTESIAN_POINT ( 'NONE',  ( 765.0180583372156207, -24.99823902205683268, -360.0135310231089534 ) ) ;
#42337=CARTESIAN_POINT ( 'NONE',  ( 755.3201227861273992, -27.72551174932954510, -345.3687786644892981 ) ) ;
#42342=CARTESIAN_POINT ( 'NONE',  ( 747.6481478633932056, -277.0999726633344267, -353.4146539503763620 ) ) ;
#42346=CARTESIAN_POINT ( 'NONE',  ( 768.0187753319979720, -248.6346026584197659, -318.0580252608186242 ) ) ;
#42347=CARTESIAN_POINT ( 'NONE',  ( 756.1348686366196716, -401.2601417444137155, -347.5531968255698416 ) ) ;
#42348=DIRECTION ( 'NONE',  ( 0.000000000000000000, 0.000000000000000000, 1.000000000000000000 ) ) ;
#42349=CARTESIAN_POINT ( 'NONE',  ( 775.8780910478218402, -105.2817908451530968, -364.9511171171680530 ) ) ;
#42352=CARTESIAN_POINT ( 'NONE',  ( 764.3348316497523456, 1.285312801039623753, -308.6759233522265617 ) ) ;
#42353=CARTESIAN_POINT ( 'NONE',  ( 812.7932403749906598, -327.1800572038741279, -327.7687537140311633 ) ) ;
#42356=CARTESIAN_POINT ( 'NONE',  ( 804.6798772138708955, -87.72551174932937101, -334.6312213355107019 ) ) ;
#42359=CARTESIAN_POINT ( 'NONE',  ( 800.1688906516307043, -202.1692326535051905, -369.0717654672308186 ) ) ;
#42361=CARTESIAN_POINT ( 'NONE',  ( 786.2694204179717872, 2.718209154846545683, -305.1769319972829067 ) ) ;
#42366=CARTESIAN_POINT ( 'NONE',  ( 804.9363028652555840, -448.2709662947827951, -338.2165204200192079 ) ) ;
#42372=CARTESIAN_POINT ( 'NONE',  ( 799.4546378042377910, -297.0783235625957559, -356.1575198192848006 ) ) ;
#42376=CARTESIAN_POINT ( 'NONE',  ( 788.7631598425961101, -289.4419599262321299, -305.7194118038759143 ) ) ;
#42381=CARTESIAN_POINT ( 'NONE',  ( 801.3366627262608972, -56.53286901714201917, -353.0897708529566899 ) ) ;
#42382=CARTESIAN_POINT ( 'NONE',  ( 771.2633955100217236, -167.9073299311473022, -363.4237431249939618 ) ) ;
#42383=CARTESIAN_POINT ( 'NONE',  ( 771.2633955100217236, -215.9073299311471317, -363.4237431249939618 ) ) ;
#42385=CARTESIAN_POINT ( 'NONE',  ( 815.2698199232961542, -160.8164208402382371, -342.5225473063383106 ) ) ;
#42386=CARTESIAN_POINT ( 'NONE',  ( 797.8594530101009923, -133.5436935675110419, -322.1405469898982119 ) ) ;
#42388=CARTESIAN_POINT ( 'NONE',  ( 763.0428371773158460, -395.4636090269705164, -358.7617431975195359 ) ) ;
#42398=CARTESIAN_POINT ( 'NONE',  ( 800.9840315886518738, -388.9181544815158986, -354.1144889064786412 ) ) ;
#42399=CARTESIAN_POINT ( 'NONE',  ( 755.0636971347428243, -364.2709662947830793, -341.7834795799807353 ) ) ;
#42400=CARTESIAN_POINT ( 'NONE',  ( 815.3608509340175488, -170.7363362996983938, -341.2497674668889545 ) ) ;
#42404=CARTESIAN_POINT ( 'NONE',  ( 802.1676090361156639, -446.6346026584189985, -327.8955696845344505 ) ) ;
#42405=CARTESIAN_POINT ( 'NONE',  ( 745.5313806188320314, -159.2817908451529547, -333.7943932421247268 ) ) ;
#42406=DIRECTION ( 'NONE',  ( 0.000000000000000000, -0.000000000000000000, -1.000000000000000000 ) ) ;
#42409=AXIS2_PLACEMENT_3D ( 'NONE', #26613, #43948, #2138 ) ;
#42411=AXIS2_PLACEMENT_3D ( 'NONE', #20544, #9695, #34854 ) ;
#42412=CARTESIAN_POINT ( 'NONE',  ( 754.9967657858570647, -193.5436935675108714, -365.0032342141425943 ) ) ;
#42414=CARTESIAN_POINT ( 'NONE',  ( 771.1735550268778070, 14.81994279612486309, -316.3353852180827630 ) ) ;
#42417=CARTESIAN_POINT ( 'NONE',  ( 744.9990715423526808, -114.3510508353236617, -341.2370466360926002 ) ) ;
#42419=CARTESIAN_POINT ( 'NONE',  ( 800.9747183278959710, -324.9982390220559409, -311.9810565676471583 ) ) ;
#42420=EDGE_CURVE ( 'NONE', #37557, #26190, #44507, .T. ) ;
#42425=CARTESIAN_POINT ( 'NONE',  ( 744.8212110874229666, -426.8965053807771142, -336.2046728542121627 ) ) ;
#42427=CARTESIAN_POINT ( 'NONE',  ( 763.0537975583475827, -432.4527844766008684, -371.0346526505627480 ) ) ;
#42433=CARTESIAN_POINT ( 'NONE',  ( 803.8556311672234642, -177.6237781080507148, -365.6418435158340117 ) ) ;
#42438=CARTESIAN_POINT ( 'NONE',  ( 759.9864689768902508, -146.0891481129655176, -354.9819416627836404 ) ) ;
#42440=CARTESIAN_POINT ( 'NONE',  ( 749.2812353651451076, -30.45278447660226817, -323.2262854647983090 ) ) ;
#42444=CARTESIAN_POINT ( 'NONE',  ( 813.5763878283155464, -459.8272453906066062, -351.1614460488615350 ) ) ;
#42450=CARTESIAN_POINT ( 'NONE',  ( 794.9819416627830151, -300.9982390220559409, -319.9864689768909898 ) ) ;
#42456=CARTESIAN_POINT ( 'NONE',  ( 801.5560724626406000, -288.5545181178798657, -326.7756240680316182 ) ) ;
#42457=CARTESIAN_POINT ( 'NONE',  ( 781.8018195045266339, -238.2709662947833920, -365.1927285166406705 ) ) ;
#42458=CARTESIAN_POINT ( 'NONE',  ( 771.1735550268780344, -441.1800572038736163, -316.3353852180828198 ) ) ;
#42459=CARTESIAN_POINT ( 'NONE',  ( 756.3353852180819104, -125.9073299311474159, -331.1735550268788302 ) ) ;
#42465=CARTESIAN_POINT ( 'NONE',  ( 757.7880784355613741, -42.00906357242603661, -312.4576283171834916 ) ) ;
#42468=CIRCLE ( 'NONE', #28450, 30.00000000000008171 ) ;
#42471=ORIENTED_EDGE ( 'NONE', *, *, #45593, .T. ) ;
#42472=CARTESIAN_POINT ( 'NONE',  ( 802.9823548866075953, -1.099972663335260226, -330.0799878456151077 ) ) ;
#42473=CARTESIAN_POINT ( 'NONE',  ( 814.5518280994195948, -87.72551174932935680, -332.4837098697145166 ) ) ;
#42478=CARTESIAN_POINT ( 'NONE',  ( 744.7301800767019131, -244.8164208402378961, -337.4774526936615757 ) ) ;
#42483=CARTESIAN_POINT ( 'NONE',  ( 793.4146539503750546, -289.9874144716866908, -307.6481478633938877 ) ) ;
#42484=AXIS2_PLACEMENT_3D ( 'NONE', #30339, #11893, #15803 ) ;
#42486=CARTESIAN_POINT ( 'NONE',  ( 763.0537975583475827, -312.4527844766012663, -371.0346526505627480 ) ) ;
#42491=CARTESIAN_POINT ( 'NONE',  ( 802.1676090361156639, -398.6346026584193396, -327.8955696845344505 ) ) ;
#42494=CARTESIAN_POINT ( 'NONE',  ( 773.7943932421234194, -71.80559628986922860, -305.5313806188329409 ) ) ;
#42499=CARTESIAN_POINT ( 'NONE',  ( 789.9200121543843807, -217.9874144716870035, -317.0176451133914384 ) ) ;
#42503=CARTESIAN_POINT ( 'NONE',  ( 793.4146539503750546, -49.98741447168749374, -307.6481478633938877 ) ) ;
#42505=CARTESIAN_POINT ( 'NONE',  ( 792.6815175455323015, -452.9681489794447202, -361.6124358662449367 ) ) ;
#42509=CARTESIAN_POINT ( 'NONE',  ( 766.4474001241216001, -355.0999726633341993, -307.3154664389482491 ) ) ;
#42513=CARTESIAN_POINT ( 'NONE',  ( 775.8780910478218402, -153.2817908451529831, -364.9511171171680530 ) ) ;
#42514=CARTESIAN_POINT ( 'NONE',  ( 771.2633955100217236, -143.9073299311473590, -363.4237431249939618 ) ) ;
#42515=CARTESIAN_POINT ( 'NONE',  ( 768.0187753319979720, -344.6346026584195101, -318.0580252608186242 ) ) ;
#42526=CARTESIAN_POINT ( 'NONE',  ( 755.8990559732751535, -395.4636090269705164, -365.9055244015606831 ) ) ;
#42527=CARTESIAN_POINT ( 'NONE',  ( 777.4774526936600978, 13.72903370521577315, -304.7301800767028226 ) ) ;
#42531=CARTESIAN_POINT ( 'NONE',  ( 795.1360043628807261, -356.0891481129647218, -360.2193346964456282 ) ) ;
#42535=CARTESIAN_POINT ( 'NONE',  ( 799.2566176426618085, -216.0090635724255037, -324.0069404352559559 ) ) ;
#42541=CARTESIAN_POINT ( 'NONE',  ( 804.7487373415286811, -427.5436935675101040, -364.7487373415288516 ) ) ;
#42542=DIRECTION ( 'NONE',  ( -1.000000000000000000, 0.000000000000000000, 0.000000000000000000 ) ) ;
#42546=CARTESIAN_POINT ( 'NONE',  ( 792.3570229623688874, -45.18005720387493085, -373.1304606946836202 ) ) ;
#42548=CARTESIAN_POINT ( 'NONE',  ( 778.1981804954714335, -274.2709662947833067, -314.8072714833589885 ) ) ;
#42553=CARTESIAN_POINT ( 'NONE',  ( 813.5763878283155464, -75.82724539060775726, -351.1614460488615350 ) ) ;
#42554=CARTESIAN_POINT ( 'NONE',  ( 804.9511171171677688, -77.80559628986920018, -335.8780910478229202 ) ) ;
#42557=CARTESIAN_POINT ( 'NONE',  ( 788.8264449731200330, 2.819942796124898177, -363.6646147819171233 ) ) ;
#42558=CARTESIAN_POINT ( 'NONE',  ( 804.1601925771018387, -103.4419599262327836, -346.5483106153029098 ) ) ;
#42560=CARTESIAN_POINT ( 'NONE',  ( 800.2193346964447755, -114.9982390220565236, -355.1360043628815788 ) ) ;
#42562=CARTESIAN_POINT ( 'NONE',  ( 779.4709603349208464, -408.3510508353227806, -314.7162404726379918 ) ) ;
#42567=CARTESIAN_POINT ( 'NONE',  ( 805.9055244015594326, -411.6237781080499758, -315.8990559732753240 ) ) ;
#42574=CARTESIAN_POINT ( 'NONE',  ( 792.3570229623688874, -237.1800572038742985, -373.1304606946836202 ) ) ;
#42579=CARTESIAN_POINT ( 'NONE',  ( 804.4286716492782716, -257.3618753856924286, -345.3141322388244703 ) ) ;
#42581=CARTESIAN_POINT ( 'NONE',  ( 792.1044303154645831, -348.4527844766012663, -317.8323909638837677 ) ) ;
#42582=CARTESIAN_POINT ( 'NONE',  ( 768.0187753319979720, -8.634602658420517329, -318.0580252608186242 ) ) ;
#42585=DIRECTION ( 'NONE',  ( -1.000000000000000000, -0.000000000000000000, -0.000000000000000000 ) ) ;
#42587=CARTESIAN_POINT ( 'NONE',  ( 756.3353852180819104, -29.90732993114771787, -331.1735550268788302 ) ) ;
#42591=CARTESIAN_POINT ( 'NONE',  ( 802.2119215644370342, -270.0090635724253048, -367.5423716828165084 ) ) ;
#42594=CARTESIAN_POINT ( 'NONE',  ( 797.6776695296629214, -259.5436935675106156, -357.6776695296636603 ) ) ;
#42595=CARTESIAN_POINT ( 'NONE',  ( 754.9735926884551418, -402.3510508353228374, -340.5236548041000333 ) ) ;
#42597=CARTESIAN_POINT ( 'NONE',  ( 769.0155153010367712, -130.3726999360621619, -362.7791456095907279 ) ) ;
#42600=CARTESIAN_POINT ( 'NONE',  ( 795.6651683502461765, 13.28531280103958423, -371.3240766477733814 ) ) ;
#42601=CARTESIAN_POINT ( 'NONE',  ( 754.9967657858570647, -313.5436935675103882, -365.0032342141425943 ) ) ;
#42606=CARTESIAN_POINT ( 'NONE',  ( 759.8311093483677041, -190.1692326535052189, -310.9282345327691814 ) ) ;
#42608=CARTESIAN_POINT ( 'NONE',  ( 763.2262854647970016, -440.6346026584191122, -309.2812353651462445 ) ) ;
#42613=CARTESIAN_POINT ( 'NONE',  ( 756.7813123517142913, 4.012585528312341054, -329.9779781133712504 ) ) ;
#42619=CARTESIAN_POINT ( 'NONE',  ( 789.9200121543843807, -289.9874144716866908, -317.0176451133914384 ) ) ;
#42621=CARTESIAN_POINT ( 'NONE',  ( 813.2346286133761168, -293.2601417444139429, -328.9521613784389160 ) ) ;
#42626=CARTESIAN_POINT ( 'NONE',  ( 766.7756240680305382, -86.53286901714194812, -361.5560724626415663 ) ) ;
#42627=CARTESIAN_POINT ( 'NONE',  ( 755.0636971347428243, -148.2709662947837330, -341.7834795799807353 ) ) ;
#42628=CARTESIAN_POINT ( 'NONE',  ( 762.1405469898971887, -217.5436935675107293, -357.8594530101015607 ) ) ;
#42630=CARTESIAN_POINT ( 'NONE',  ( 810.7187646348534145, -162.4527844766018632, -356.7737145352016341 ) ) ;
#42632=CARTESIAN_POINT ( 'NONE',  ( 759.7806653035535192, -150.9982390220564241, -324.8639956371181370 ) ) ;
#42635=CARTESIAN_POINT ( 'NONE',  ( 780.5236548040995785, -380.7363362996977116, -314.9735926884559944 ) ) ;
#42642=CARTESIAN_POINT ( 'NONE',  ( 757.4527132478984868, -400.3726999360612808, -329.1273215169538844 ) ) ;
#42644=CARTESIAN_POINT ( 'NONE',  ( 747.6481478633932056, -181.0999726633347109, -353.4146539503763620 ) ) ;
#42649=CARTESIAN_POINT ( 'NONE',  ( 786.2694204179717872, -189.2817908451528979, -305.1769319972829067 ) ) ;
#42654=CARTESIAN_POINT ( 'NONE',  ( 751.9810565676468741, -218.0891481129653187, -360.9747183278973921 ) ) ;
#42656=CARTESIAN_POINT ( 'NONE',  ( 788.7366044899766848, 12.09267006885214180, -316.5762568750059813 ) ) ;
#42658=CARTESIAN_POINT ( 'NONE',  ( 747.3154664389472828, -91.98741447168737295, -326.4474001241230781 ) ) ;
#42660=CARTESIAN_POINT ( 'NONE',  ( 814.5518280994195948, -327.7255117493285184, -332.4837098697145734 ) ) ;
#42665=CARTESIAN_POINT ( 'NONE',  ( 759.8311093483677041, -406.1692326535045368, -310.9282345327691814 ) ) ;
#42667=CARTESIAN_POINT ( 'NONE',  ( 758.8095938919642549, -416.0891481129645513, -311.6929314249763365 ) ) ;
#42671=CARTESIAN_POINT ( 'NONE',  ( 766.5853460496234675, -181.9874144716870887, -372.3518521366060554 ) ) ;
#42676=CARTESIAN_POINT ( 'NONE',  ( 744.7301800767019131, -28.81642084023863148, -337.4774526936615757 ) ) ;
#42679=CARTESIAN_POINT ( 'NONE',  ( 815.3608509340175488, -434.7363362996975980, -341.2497674668889545 ) ) ;
#42685=CARTESIAN_POINT ( 'NONE',  ( 772.4468031744293057, -273.8272453906071746, -363.8651313633793620 ) ) ;
#42686=CARTESIAN_POINT ( 'NONE',  ( 762.1405469898971887, -289.5436935675103882, -357.8594530101015607 ) ) ;
#42687=CARTESIAN_POINT ( 'NONE',  ( 754.8072714833583632, -436.8164208402372992, -338.1981804954721156 ) ) ;
#42694=CARTESIAN_POINT ( 'NONE',  ( 776.2046728542105711, -68.19088175424413123, -304.8212110874238761 ) ) ;
#42701=CARTESIAN_POINT ( 'NONE',  ( 757.4527132478984868, -64.37269993606231822, -329.1273215169538844 ) ) ;
#42702=CARTESIAN_POINT ( 'NONE',  ( 767.6429770376291799, -105.1800572038747390, -306.8695393053162093 ) ) ;
#42706=CARTESIAN_POINT ( 'NONE',  ( 805.0032342141412300, -229.5436935675106440, -314.9967657858571783 ) ) ;
#42709=CARTESIAN_POINT ( 'NONE',  ( 758.0141637701419768, -303.0783235625957559, -367.2620300519063790 ) ) ;
#42711=CARTESIAN_POINT ( 'NONE',  ( 808.3070685750230950, -306.9982390220558273, -361.1904061080339261 ) ) ;
#42715=CARTESIAN_POINT ( 'NONE',  ( 797.8594530101008786, -373.5436935675101040, -322.1405469898980982 ) ) ;
#42717=CARTESIAN_POINT ( 'NONE',  ( 747.3154664389472828, -67.98741447168742980, -326.4474001241230781 ) ) ;
#42722=CARTESIAN_POINT ( 'NONE',  ( 805.0264073115434940, -198.3510508353234059, -339.4763451958999099 ) ) ;
#42724=CARTESIAN_POINT ( 'NONE',  ( 744.8212110874229666, -18.89650538077849617, -336.2046728542121627 ) ) ;
#42726=CARTESIAN_POINT ( 'NONE',  ( 802.3178104526313064, -452.9681489794448339, -352.6268974387025423 ) ) ;
#42730=CARTESIAN_POINT ( 'NONE',  ( 776.2046728542105711, -332.1908817542433781, -304.8212110874238761 ) ) ;
#42734=CARTESIAN_POINT ( 'NONE',  ( 805.2837595273609850, -194.7363362996982517, -340.5290396650784714 ) ) ;
#42735=CARTESIAN_POINT ( 'NONE',  ( 771.1735550268778070, -153.1800572038746395, -316.3353852180827630 ) ) ;
#42736=CARTESIAN_POINT ( 'NONE',  ( 805.1927285166399315, -352.8164208402375266, -341.8018195045277707 ) ) ;
#42742=DIRECTION ( 'NONE',  ( -0.000000000000000000, -1.110223024625155554E-15, -1.000000000000000000 ) ) ;
#42747=CARTESIAN_POINT ( 'NONE',  ( 778.7629533639073998, -416.7363362996975980, -375.0009284576466371 ) ) ;
#42748=CARTESIAN_POINT ( 'NONE',  ( 759.0252816721024374, -0.9982390220569063999, -368.0189434323527280 ) ) ;
#42752=CARTESIAN_POINT ( 'NONE',  ( 754.8072714833581358, -364.8164208402374697, -338.1981804954720587 ) ) ;
#42754=CARTESIAN_POINT ( 'NONE',  ( 793.9708237608222134, -238.9181544815163534, -319.2295555964448681 ) ) ;
#42758=CARTESIAN_POINT ( 'NONE',  ( 792.3570229623691148, -405.1800572038737869, -373.1304606946836770 ) ) ;
#42765=CARTESIAN_POINT ( 'NONE',  ( 814.9108240113580450, -40.27096629478405987, -337.5031285880265273 ) ) ;
#42766=CARTESIAN_POINT ( 'NONE',  ( 768.0187753319979720, -296.6346026584195670, -318.0580252608186242 ) ) ;
#42771=CARTESIAN_POINT ( 'NONE',  ( 755.8990559732751535, -59.46360902697142592, -365.9055244015606831 ) ) ;
#42772=CARTESIAN_POINT ( 'NONE',  ( 754.9735926884551418, -90.35105083532373271, -340.5236548041000333 ) ) ;
#42775=CARTESIAN_POINT ( 'NONE',  ( 804.9363028652555840, 7.729033705215793582, -338.2165204200192079 ) ) ;
#42776=CARTESIAN_POINT ( 'NONE',  ( 794.1144889064781864, -106.1692326535054889, -360.9840315886528401 ) ) ;
#42778=CARTESIAN_POINT ( 'NONE',  ( 788.7366044899766848, -83.90732993114754379, -316.5762568750059813 ) ) ;
#42779=CARTESIAN_POINT ( 'NONE',  ( 802.7791456095903868, -412.7146871989590409, -329.0155153010375102 ) ) ;
#42782=CARTESIAN_POINT ( 'NONE',  ( 747.3154664389472828, -403.9874144716863498, -326.4474001241230781 ) ) ;
#42788=( NAMED_UNIT ( * ) SI_UNIT ( $, .STERADIAN. ) SOLID_ANGLE_UNIT ( ) );
#42789=CARTESIAN_POINT ( 'NONE',  ( 767.7687537140311633, -263.9073299311469327, -372.7932403749916830 ) ) ;
#42791=EDGE_CURVE ( 'NONE', #5020, #25862, #34118, .T. ) ;
#42795=CARTESIAN_POINT ( 'NONE',  ( 801.5560724626406000, -72.55451811788049099, -326.7756240680316182 ) ) ;
#42797=CARTESIAN_POINT ( 'NONE',  ( 797.8594530101009923, -229.5436935675107009, -322.1405469898982119 ) ) ;
#42799=CARTESIAN_POINT ( 'NONE',  ( 759.7806653035534055, -342.9982390220557136, -324.8639956371180801 ) ) ;
#42800=CARTESIAN_POINT ( 'NONE',  ( 762.1405469898971887, -49.54369356751129061, -357.8594530101015607 ) ) ;
#42805=ORIENTED_EDGE ( 'NONE', *, *, #11198, .F. ) ;
#42806=CARTESIAN_POINT ( 'NONE',  ( 754.8072714833581358, -4.816420840238714085, -338.1981804954720587 ) ) ;
#42810=CARTESIAN_POINT ( 'NONE',  ( 795.8262568251477660, -286.3726999360617356, -308.3538107759623585 ) ) ;
#42813=CARTESIAN_POINT ( 'NONE',  ( 762.3223304703356007, -247.5436935675106724, -322.3223304703362828 ) ) ;
#42815=CARTESIAN_POINT ( 'NONE',  ( 804.8461984189677878, -122.1908817542439749, -336.9566956441385628 ) ) ;
#42818=CARTESIAN_POINT ( 'NONE',  ( 766.5853460496234675, -13.98741447168760033, -372.3518521366060554 ) ) ;
#42819=CARTESIAN_POINT ( 'NONE',  ( 751.6929314249750860, -294.9982390220559978, -318.8095938919659034 ) ) ;
#42823=CARTESIAN_POINT ( 'NONE',  ( 752.4576283171824116, -213.0783235625960401, -317.7880784355627952 ) ) ;
#42825=CARTESIAN_POINT ( 'NONE',  ( 754.3581564841646241, 6.536390973028352924, -316.1443688327762516 ) ) ;
#42830=CARTESIAN_POINT ( 'NONE',  ( 772.3691319403857278, 24.73985825558500551, -315.8894580844506663 ) ) ;
#42831=DIRECTION ( 'NONE',  ( 0.000000000000000000, -0.000000000000000000, 1.000000000000000000 ) ) ;
#42836=CARTESIAN_POINT ( 'NONE',  ( 804.1601925771018387, -295.4419599262320730, -346.5483106153029098 ) ) ;
#42838=CARTESIAN_POINT ( 'NONE',  ( 805.9055244015594326, -291.6237781080503169, -315.8990559732753240 ) ) ;
#42843=CARTESIAN_POINT ( 'NONE',  ( 793.2243759319678702, -74.53286901714196233, -318.4439275373583200 ) ) ;
#42844=CARTESIAN_POINT ( 'NONE',  ( 804.9363028652555840, -160.2709662947836762, -338.2165204200192079 ) ) ;
#42846=CARTESIAN_POINT ( 'NONE',  ( 801.1904061080336987, -140.0891481129654892, -368.3070685750235498 ) ) ;
#42848=CARTESIAN_POINT ( 'NONE',  ( 781.7834795799800531, -154.8164208402382371, -315.0636971347436202 ) ) ;
#42850=CARTESIAN_POINT ( 'NONE',  ( 755.3028492785439312, -375.2817908451523294, -335.9200461376539693 ) ) ;
#42857=CARTESIAN_POINT ( 'NONE',  ( 755.1538015810308480, -398.1908817542431507, -343.0433043558613804 ) ) ;
#42859=CARTESIAN_POINT ( 'NONE',  ( 814.2805881961230625, -169.6454272087892718, -331.2368401574024119 ) ) ;
#42863=CARTESIAN_POINT ( 'NONE',  ( 766.7756240680305382, -326.5328690171411381, -361.5560724626415663 ) ) ;
#42864=CARTESIAN_POINT ( 'NONE',  ( 797.8594530101008786, -445.5436935675098766, -322.1405469898980982 ) ) ;
#42865=CARTESIAN_POINT ( 'NONE',  ( 813.5763878283155464, -195.8272453906074304, -351.1614460488615350 ) ) ;
#42870=CARTESIAN_POINT ( 'NONE',  ( 748.9653473494365699, -218.6346026584198228, -356.9462024416520762 ) ) ;
#42872=CARTESIAN_POINT ( 'NONE',  ( 781.7834795799800531, -10.81642084023869543, -315.0636971347436202 ) ) ;
#42874=CARTESIAN_POINT ( 'NONE',  ( 771.2368401574024119, -85.44195992623282621, -374.2805881961240857 ) ) ;
#42876=CARTESIAN_POINT ( 'NONE',  ( 787.4397851343537695, -333.7255117493286320, -374.2001403089903988 ) ) ;
#42881=CARTESIAN_POINT ( 'NONE',  ( 812.6845335610512393, -415.9874144716862361, -353.5525998758768651 ) ) ;
#42882=CARTESIAN_POINT ( 'NONE',  ( 787.5162901302840055, -419.3618753856918033, -305.4481719005792684 ) ) ;
#42886=CARTESIAN_POINT ( 'NONE',  ( 772.3691319403857278, -191.2601417444143976, -315.8894580844506663 ) ) ;
#42887=CARTESIAN_POINT ( 'NONE',  ( 774.6312213355099630, -119.3618753856928691, -364.6798772138717482 ) ) ;
#42889=CARTESIAN_POINT ( 'NONE',  ( 781.2497674668890113, -204.3510508353233774, -375.3608509340180603 ) ) ;
#42895=CARTESIAN_POINT ( 'NONE',  ( 748.9653473494363425, -50.63460265842036989, -356.9462024416521331 ) ) ;
#42898=CARTESIAN_POINT ( 'NONE',  ( 802.2119215644370342, -438.0090635724247932, -367.5423716828165084 ) ) ;
#42903=CARTESIAN_POINT ( 'NONE',  ( 759.7806653035534055, -294.9982390220560546, -324.8639956371180801 ) ) ;
#42907=CARTESIAN_POINT ( 'NONE',  ( 755.5913626894240451, -301.6454272087889308, -346.6156483768012890 ) ) ;
#42908=CARTESIAN_POINT ( 'NONE',  ( 759.7806653035534055, -294.9982390220560546, -324.8639956371180801 ) ) ;
#42910=CARTESIAN_POINT ( 'NONE',  ( 805.1927285166397041, -112.8164208402383508, -341.8018195045277707 ) ) ;
#42916=CARTESIAN_POINT ( 'NONE',  ( 810.4231160770870019, -72.55451811788049099, -321.9338519418446936 ) ) ;
#42922=CARTESIAN_POINT ( 'NONE',  ( 804.8461984189677878, -50.19088175424420939, -336.9566956441385628 ) ) ;
#42923=CARTESIAN_POINT ( 'NONE',  ( 751.6929314249750860, -102.9982390220565662, -318.8095938919659034 ) ) ;
#42928=CARTESIAN_POINT ( 'NONE',  ( 787.4397851343537695, -237.7255117493289163, -374.2001403089903988 ) ) ;
#42932=CARTESIAN_POINT ( 'NONE',  ( 791.1614460488616487, -323.2601417444138860, -373.5763878283158874 ) ) ;
#42934=CARTESIAN_POINT ( 'NONE',  ( 808.3070685750230950, -330.9982390220558273, -361.1904061080339261 ) ) ;
#42938=CARTESIAN_POINT ( 'NONE',  ( 764.8639956371174549, -416.0891481129645513, -319.7806653035542013 ) ) ;
#42940=CARTESIAN_POINT ( 'NONE',  ( 758.0580252608178853, -198.4527844766017495, -328.0187753319985404 ) ) ;
#42941=CARTESIAN_POINT ( 'NONE',  ( 754.0944755984390895, -87.62377810805102740, -364.1009440267246760 ) ) ;
#42945=CARTESIAN_POINT ( 'NONE',  ( 779.4709603349208464, -240.3510508353232069, -314.7162404726379918 ) ) ;
#42947=CARTESIAN_POINT ( 'NONE',  ( 805.9055244015594326, -27.62377810805120149, -315.8990559732753240 ) ) ;
#42954=CARTESIAN_POINT ( 'NONE',  ( 811.3240766477731540, -340.3726999360615082, -355.6651683502462902 ) ) ;
#42957=CARTESIAN_POINT ( 'NONE',  ( 802.9823548866075953, -193.0999726633346256, -330.0799878456151077 ) ) ;
#42958=CARTESIAN_POINT ( 'NONE',  ( 804.6798772138708955, -183.7255117493290015, -334.6312213355107019 ) ) ;
#42959=CARTESIAN_POINT ( 'NONE',  ( 758.0580252608178853, -366.4527844766012095, -328.0187753319985404 ) ) ;
#42961=CARTESIAN_POINT ( 'NONE',  ( 789.9200121543843807, 22.01258552831228599, -317.0176451133914384 ) ) ;
#42971=CARTESIAN_POINT ( 'NONE',  ( 755.8990559732751535, -419.4636090269702891, -365.9055244015606831 ) ) ;
#42973=CARTESIAN_POINT ( 'NONE',  ( 767.6429770376291799, 14.81994279612486309, -306.8695393053162093 ) ) ;
#42976=CARTESIAN_POINT ( 'NONE',  ( 762.1405469898971887, -361.5436935675103882, -357.8594530101015607 ) ) ;
#42977=CARTESIAN_POINT ( 'NONE',  ( 762.3223304703356007, 16.45630643248849267, -322.3223304703362828 ) ) ;
#42980=CARTESIAN_POINT ( 'NONE',  ( 775.8780910478218402, -273.2817908451526137, -364.9511171171680530 ) ) ;
#42990=CARTESIAN_POINT ( 'NONE',  ( 791.9812246680005501, -332.6346026584195101, -361.9419747391813189 ) ) ;
#42995=CARTESIAN_POINT ( 'NONE',  ( 799.9636004259356241, -70.91815448151683654, -311.2241431872006956 ) ) ;
#42996=CARTESIAN_POINT ( 'NONE',  ( 759.2295555964440155, -88.16923265350555994, -353.9708237608231229 ) ) ;
#42999=CARTESIAN_POINT ( 'NONE',  ( 758.0580252608178853, -6.452784476602343666, -328.0187753319985404 ) ) ;
#43000=CARTESIAN_POINT ( 'NONE',  ( 759.2295555964440155, -112.1692326535054889, -353.9708237608231229 ) ) ;
#43002=CARTESIAN_POINT ( 'NONE',  ( 768.0187753319979720, -104.6346026584202207, -318.0580252608186242 ) ) ;
#43004=CARTESIAN_POINT ( 'NONE',  ( 783.0433043558608688, -408.8965053807772847, -315.1538015810313027 ) ) ;
#43015=CARTESIAN_POINT ( 'NONE',  ( 766.0291762391763086, -82.91815448151682233, -360.7704444035551319 ) ) ;
#43017=CARTESIAN_POINT ( 'NONE',  ( 755.3201227861273992, -243.7255117493288310, -345.3687786644892981 ) ) ;
#43018=ORIENTED_EDGE ( 'NONE', *, *, #9907, .T. ) ;
#43020=CARTESIAN_POINT ( 'NONE',  ( 804.4286716492782716, -377.3618753856920875, -345.3141322388244703 ) ) ;
#43021=CARTESIAN_POINT ( 'NONE',  ( 804.4286716492782716, -41.36187538569314626, -345.3141322388244703 ) ) ;
#43023=EDGE_CURVE ( 'NONE', #21713, #23858, #23067, .T. ) ;
#43026=CYLINDRICAL_SURFACE ( 'NONE', #33170, 10.00000000000000888 ) ;
#43027=CARTESIAN_POINT ( 'NONE',  ( 757.8323909638827445, -26.63460265842045871, -352.1044303154654358 ) ) ;
#43028=CARTESIAN_POINT ( 'NONE',  ( 799.9999999999993179, 205.0000000000000568, -339.9999999999999432 ) ) ;
#43030=CARTESIAN_POINT ( 'NONE',  ( 813.5763878283155464, -315.8272453906070609, -351.1614460488615350 ) ) ;
#43033=CARTESIAN_POINT ( 'NONE',  ( 755.0636971347428243, -268.2709662947833067, -341.7834795799807353 ) ) ;
#43034=( BOUNDED_SURFACE ( )  B_SPLINE_SURFACE ( 3, 2, ( 
 ( #14487, #7549, #5985, #42414, #14027, #3853, #23532, #28567, #42656, #11018, #10785, #45037, #24861, #35709, #23753, #13168, #27018, #37868, #38978, #21626, #17944, #6215, #25085, #41117, #9470, #26224, #11239, #11701, #43334, #32486, #18183, #15166, #35949, #29257, #21857, #29472, #40090, #43762, #36173, #32259, #25773, #12142, #836, #36392, #25551, #14935, #8014, #22522, #18858, #40339, #42872, #43546, #8227, #11471, #36633, #29018, #4987, #43101, #4315, #39665, #617, #22082, #15393, #4533, #18406, #8452, #39885, #32948, #8691, #18626, #4755, #32712, #1059, #22296, #19080, #1295, #22755, #25312, #11912, #25983, #33169, #1505, #15602, #29686, #36850, #14719, #28794, #39425, #7780, #2414, #19510, #22968, #27144, #44457, #19979, #1720, #34280, #15824, #30832, #20199, #44926, #44696, #12375, #2192, #2652, #23875, #16284, #23190, #13056, #19289, #16514, #30596, #27361, #44001, #12813, #41231, #40765, #37063, #9590, #23650, #37531, #44232, #34055, #5890, #16750, #5416, #8901, #40550, #26452, #9122, #29916, #33608, #12590, #37298, #37761, #41001, #6110, #1960, #16060, #13284, #26894, #5659, #19752, #41456, #26668, #9808, #30143, #33838, #5202, #33375, #30364, #9361, #23430, #10263, #6795, #17667, #24804, #31051, #42135, #41919, #21121, #16975, #97, #31729, #14189, #24340, #27822, #20872, #38924, #34742, #45150, #37995, #17192, #31279, #7276, #38444, #27584, #41689, #34525, #28257, #6348, #13511, #34970, #3344, #6571, #20432, #17437, #38225, #31517, #24113, #7035, #42356, #2883, #45620, #10043, #35204, #13968, #45383, #20650, #28041, #10486, #3102, #3581, #24560, #38676, #10725, #13745, #41599, #26586, #27062, #12972, #2111, #33526, #30508, #5574, #44611, #37210, #44847, #9728, #13430, #5812, #1874, #41157, #27500, #16200, #6026, #40914, #30280, #23351, #37904, #34193, #9956, #12510, #13209, #23572, #26808, #6258, #44373, #20345, #12728, #19666, #9281, #15982, #37453, #30754, #19900, #33759, #23792, #9508, #2563, #30065, #16896, #44146, #24026, #2805, #38145, #27286, #40684, #37677, #30977, #6496, #20117, #33977, #41379, #9038, #34440, #45075, #23108, #2328, #16668, #16427, #10405, #38368, #24947, #14338, #7188, #13887, #3717, #21262, #18032, #20791, #24260, #10184, #41839, #24482, #17116, #34886, #27961, #38588, #35341, #10636, #17804, #6714, #17342, #42514, #42275, #6944, #35115, #478, #42057, #39062, #31428, #3250, #10879, #20574, #7410, #27735, #28416, #17580, #14109, #35562, #42735, #45534, #31871, #3492, #21485, #13654, #32113, #3937, #14583, #31650, #21027, #28183, #25169, #18, #24717, #38835, #31197, #241, #28657, #11099, #39279, #34670, #3029, #45295, #4405, #29563, #29347, #11561, #22166, #33248, #917, #26070, #18495, #25403, #43637, #7633, #40184, #14804, #15483, #4613, #1153, #22613, #29775, #28878, #18946, #36255, #12007, #707, #5073, #36713, #19164, #18709, #8105, #15258, #12235, #15019, #42958, #21711, #29108, #43192, #43852, #32799, #11325, #39525, #35808, #1593, #15692, #7880, #43420, #11787, #21956, #4184, #25858, #36042, #39968, #32573, #33042, #8549, #26314, #25643, #18279, #8313, #32353, #39757, #22377, #36482, #4847, #1380, #44793, #41094, #2749, #19380, #5967, #30447, #33700, #13148, #8984, #27229, #5511, #12455, #37151, #22840, #19607, #37614, #23053, #26534, #16609, #33920, #9449, #36933, #23736, #5287, #20287, #9671, #34380, #34134, #1812, #37395, #37847, #13372, #5749, #12673, #2502, #8772, #20056, #30697, #16844, #33464, #2271, #41321, #30227, #40632, #6195, #30923, #26998, #2050, #23513, #45019, #40420, #16144, #44090, #44318, #16369, #9219, #15919, #30003, #26753, #40856, #23294, #12910, #44549, #19838, #38532, #35061, #42228, #38316, #42457, #192, #20963, #41783, #17757, #28353, #21211, #13595, #2972, #14284, #31137, #7361, #31371, #23967, #10824, #45709, #24659, #3670, #10581, #31605, #28133, #17061, #24896, #31821, #21437, #9893, #17982, #6886, #6663, #6444, #32052, #3435, #17532, #423, #34829, #42009, #35513, #38775, #38089, #45479, #14061, #27444, #39010, #27678, #7133, #20736, #41542, #35292, #3888, #20523, #34617, #45235, #24429, #10133, #24206, #13835, #10353, #3193, #27912, #17282, #36206, #35988, #25596, #36670, #28604, #5030, #21662, #870, #39465, #14973, #11510, #18661, #32751, #39232, #11741, #25118, #4131, #43585, #43144, #4570, #19120, #18897, #26021, #29058, #28828, #11953, #7825, #21904, #18223, #40131, #8264, #4354, #8053, #18444, #42686, #1098, #39706, #32522, #22118, #15212, #29300, #43375, #8495, #35752, #42908, #14528, #32299, #25808, #39921, #22329, #36430, #4794, #32993, #653, #15435, #1331, #22566, #11053, #33209, #29513, #7585, #14754, #11275, #25351, #9163, #6149, #8937, #16097, #41271, #2227, #43802, #19553, #23236, #20239, #5923, #33415, #12858, #12410, #1546, #19791, #26939, #16322, #37342, #26265, #44272, #41039, #33874, #33649, #30181, #29724, #2001, #12184, #5704, #23008, #12629, #23689, #15641, #37800, #8730, #26707, #26490, #40806, #30403, #9400, #23467, #40379, #37566, #22795, #5242, #30643, #20013, #34089, #19332, #2455, #13099, #16558, #15867, #44741, #40591, #37102, #1759, #27183, #9626, #5458, #29956, #44040, #2697, #38482, #3142, #6614, #20689, #35010, #6833, #10085, #14230, #41494, #2923, #34326, #6394, #24158, #41731, #45426, #41962, #17233, #10305, #17012, #24378, #31320, #31770, #31560, #27623, #7079, #10768, #20913, #3386, #28299, #13788, #17479, #45660, #45187, #3621, #21160, #27867, #31089, #24601, #35243, #28080, #20478, #9847, #17709, #38038, #42399, #38268, #30871, #141, #14010, #42176, #10525, #38719, #24845, #38964, #7314, #16794, #44967, #23917, #13323, #27399, #34565, #13549, #34780, #23198, #19760, #36860, #8700, #1728, #12823, #1516, #1306, #8236, #15611, #43771, #30374, #22765, #43555, #11921, #36402, #37307, #16292, #15403, #15833, #33384, #22533, #22305, #5211, #25992, #19299, #40100, #19520, #30151, #33846, #26235, #4765, #29925, #2200, #36643, #26460, #29696, #4998, #12152, #12600, #8910, #44467, #32960, #33618, #44010, #40348, #26678, #19091, #40774, #33180, #8463, #12383, #18868, #40562, #5425, #22977, #37073, #44241, #1970, #16068, #29484, #5669, #9131, #26903, #10272, #20881, #34750, #2424, #38006, #38452, #13978, #6360, #13293, #3111, #9371, #6580, #38234, #17446, #34063, #2891, #17200, #30840, #13066, #45392, #31288, #27593, #34292, #24125, #41699, #6803, #41240, #44705, #30607, #16525, #44935, #37539, #9598, #2663, #27369, #10055, #31060, #20658, #27152, #37769, #13754, #16983, #41464, #9817, #3354, #16760, #27834, #6118, #23658, #41929, #41010, #24348, #20209, #31527, #20443, #45630, #23884, #34533, #23438, #45158, #13520, #5898, #19987, #17677, #31738, #10495, #11417, #36129, #21130, #21576, #7504, #42366, #28050, #25042, #106, #39152, #14199, #39373, #4274, #7971, #333, #42144 ),
 ( #28266, #18366, #35658, #42830, #24569, #25503, #38687, #22038, #43055, #4492, #21805, #35214, #4032, #39616, #1011, #18131, #14436, #35901, #7045, #7727, #25264, #18584, #3589, #32210, #32446, #17895, #10734, #794, #14894, #14673, #21355, #11191, #28749, #32668, #24813, #38933, #7284, #35433, #31962, #3804, #28517, #42613, #10973, #28974, #572, #15779, #18809, #11868, #37015, #36803, #19034, #29641, #40715, #8405, #33558, #25941, #32899, #5369, #15116, #1906, #22250, #22923, #12096, #8643, #30096, #37243, #36348, #26403, #43721, #19463, #8185, #12542, #44178, #26617, #26175, #15561, #22705, #40287, #5159, #29868, #40048, #9071, #16015, #19243, #29428, #23137, #5606, #8856, #1245, #4706, #19700, #15348, #33790, #33125, #11654, #29205, #33330, #12330, #43284, #43951, #1675, #40505, #43501, #25730, #39843, #22474, #36581, #4938, #1461, #27091, #26837, #38397, #9758, #23823, #6747, #9537, #16699, #41870, #2834, #44403, #20147, #37934, #20821, #6524, #34004, #45104, #13003, #2141, #20377, #13461, #16926, #6292, #40946, #44875, #27530, #34474, #34223, #30784, #30309, #2598, #12758, #31006, #23601, #13237, #24291, #16230, #9309, #23379, #27315, #41183, #41408, #41630, #9989, #24058, #37482, #38176, #5843, #19929, #31231, #20603, #34698, #2358, #3057, #13689, #17146, #16457, #45327, #37707, #6056, #30540, #27768, #10214, #44642, #28455, #42308, #3286, #39095, #3750, #7226, #21297, #35597, #7445, #10672, #14842, #42087, #3527, #34922, #6982, #24756, #38871, #277, #42554, #17838, #10916, #17613, #24985, #31905, #32392, #32150, #28214, #7670, #11362, #21520, #3974, #28915, #18068, #513, #39562, #35375, #14374, #42996, #14621, #31463, #28693, #42772, #7917, #39314, #21067, #11132, #49, #17381, #25204, #21748, #35845, #4220, #13920, #18313, #743, #25441, #45568, #27992, #10438, #24513, #38622, #35150, #31682, #14143, #44122, #36076, #12488, #29144, #8348, #1188, #22416, #18982, #26112, #40227, #952, #19194, #32611, #11599, #5318, #4880, #12043, #26565, #26347, #33503, #36519, #36294, #19413, #15296, #29380, #25677, #1851, #15725, #43452, #15514, #11819, #4443, #8586, #33072, #40000, #1411, #22650, #36748, #25887, #15957, #43228, #4652, #21987, #39790, #29594, #43672, #5106, #33281, #1626, #29813, #18749, #43892, #12272, #30041, #40451, #8805, #22872, #40663, #36964, #18529, #15058, #8138, #22202, #32837, #19878, #24005, #27480, #2542, #23329, #45054, #9932, #2785, #40892, #30259, #41578, #12708, #34651, #12950, #5551, #38127, #27268, #6233, #30960, #23770, #13186, #9707, #44351, #6478, #13408, #3010, #37187, #45273, #20094, #33955, #33737, #13632, #31177, #41356, #30733, #17098, #34169, #16646, #37883, #2306, #20555, #27715, #44827, #37432, #9017, #23087, #16877, #9260, #26787, #19645, #5788, #2087, #27036, #16178, #16405, #20323, #34418, #30485, #44590, #41135, #9487, #23549, #37653, #6001, #22310, #24241, #32966, #7800, #21004, #20774, #1311, #4332, #18421, #15410, #3472, #11254, #36408, #43120, #38350, #14093, #32501, #41820, #1075, #27944, #39682, #6924, #10165, #14950, #8030, #11489, #850, #34867, #39443, #22097, #29033, #28167, #25328, #6695, #42886, #3229, #25569, #17563, #21875, #18875, #17319, #31409, #45516, #35965, #35096, #36187, #4547, #18640, #32727, #13869, #15187, #42041, #10387, #25788, #29273, #43350, #24462, #11716, #8241, #39902, #38570, #4770, #31635, #2, #33186, #41018, #23206, #8706, #22984, #36867, #43561, #33625, #44016, #1736, #15841, #30158, #1976, #5218, #9377, #36648, #43777, #29489, #1522, #19306, #33392, #40569, #37079, #12389, #5432, #12159, #19527, #26468, #26909, #26684, #22773, #2206, #40354, #44472, #16298, #16074, #26243, #19766, #30381, #37317, #15619, #5006, #12829, #29703, #23443, #29933, #25997, #37545, #44248, #40781, #5675, #12608, #9137, #33853, #19097, #5903, #19992, #34069, #11928, #2431, #8916, #40106, #8470, #22540, #24131, #38241, #21137, #23891, #31066, #10501, #17207, #13073, #34539, #6587, #35220, #20888, #2671, #13764, #27375, #16531, #34756, #27841, #31294, #20665, #41247, #13526, #41935, #3117, #2899, #45164, #44713, #16990, #27159, #45399, #38014, #27599, #38694, #30615, #7053, #23664, #41707, #41470, #10063, #10280, #24354, #38458, #9603, #6809, #37776, #6125, #45637, #34984, #3361, #20215, #17453, #28057, #31536, #30847, #13985, #9823, #6368, #34299, #42150, #24576, #20450, #16766, #44943, #13299, #7735, #18138, #21582, #35665, #4280, #21813, #25049, #29212, #10741, #17902, #3598, #21365, #39161, #10980, #14679, #11199, #32217, #25272, #31969, #39381, #578, #1020, #800, #42619, #22044, #25736, #35908, #18372, #43292, #28756, #32452, #14900, #4039, #42836, #8191, #7511, #42372, #17685, #28982, #43062, #39849, #11424, #38939, #7290, #31744, #32674, #11660, #24820, #25510, #39624, #340, #113, #7977, #35441, #36136, #3810, #4498, #18590, #22258, #15123, #14205, #28273, #14444, #28524, #8861, #43726, #4948, #26182, #40720, #37021, #44410, #15355, #1915, #26410, #29647, #9078, #19039, #23144, #1466, #8413, #33130, #18817, #15566, #33565, #12103, #22480, #12548, #29874, #5376, #32909, #19710, #1253, #16240, #5614, #30319, #30101, #43507, #33336, #33796, #9317, #1681, #8651, #44187, #4714, #16022, #26623, #12765, #29434, #43959, #37251, #40296, #36590, #2148, #26846, #22928, #22714, #19469, #40955, #36355, #36809, #40053, #25946, #11874, #5164, #19249, #15785, #12337, #40511, #38185, #13469, #24068, #27101, #20156, #45336, #45112, #27323, #37947, #3296, #16707, #41878, #34232, #41192, #13698, #23388, #10222, #30549, #31240, #20385, #16935, #38406, #45579, #44649, #34706, #6301, #27778, #16466, #20830, #6757, #34930, #34483, #13011, #41416, #19937, #37716, #30792, #9765, #6531, #27539, #20611, #9546, #2606, #24300, #41643, #23832, #2842, #17390, #44884, #31475, #13245, #23609, #13927, #37489, #28001, #6066, #42096, #31014, #9998, #5849, #34013, #3064, #17154, #2368, #14849, #3539, #7925, #25451, #21995, #39103, #10924, #3980, #15066, #3756, #17625, #10447, #17845, #284, #32618, #24992, #58, #14151, #38633, #39570, #18538, #31691, #18077, #35605, #24763, #24523, #7453, #28221, #21527, #42316, #21758, #32401, #36084, #28462, #6993, #32157, #4450, #38880, #28700, #31912, #7235, #14384, #28926, #11141, #961, #35160, #35852, #522, #42562, #43004, #21306, #11368, #35383, #10681, #14628, #21076, #42779, #7677, #25211, #39322, #751, #4229, #18321, #29153, #26572, #39797, #23094, #12496, #37194, #36972, #4658, #40237, #40669, #16186, #8594, #15521, #5325, #11607, #8812, #40460, #19652, #36301, #5112, #19420, #33081, #15303, #1860, #33512, #29821, #36531, #26356, #43903, #9024, #43458, #1195, #32847, #12050, #25685, #29601, #8145, #19201, #18989, #22660, #33746, #22208, #2096, #18757, #43679, #22422, #26122, #36757, #1633, #15732, #29386 ),
 ( #33288, #12280, #22880, #1419, #5561, #11825, #25895, #43235, #40006, #15967, #4888, #30048, #44131, #8356, #37892, #12959, #6243, #44834, #27725, #27488, #23558, #3019, #6704, #2793, #20333, #24250, #41367, #34426, #45063, #41142, #45281, #17105, #23779, #44597, #20565, #31187, #24014, #16412, #5798, #13641, #33963, #10172, #34177, #26794, #41827, #16885, #41586, #6485, #13418, #30967, #9942, #19884, #38358, #34659, #20781, #12714, #34875, #9714, #9495, #9268, #3238, #38134, #30267, #44358, #37661, #13195, #40899, #23334, #37438, #2549, #2314, #30492, #27044, #6010, #20103, #16655, #30740, #27275, #28646, #18022, #7400, #42047, #14326, #42724, #35551, #35331, #32099, #28173, #32341, #35795, #10869, #31641, #7623, #18269, #11088, #3480, #38577, #4174, #21014, #42947, #21251, #13875, #697, #3927, #14570, #39267, #468, #21474, #25158, #6931, #14793, #21699, #11315, #45523, #7869, #28403, #42266, #10395, #21947, #24935, #39051, #36033, #24703, #31860, #25392, #28867, #27951, #3708, #39512, #17328, #31417, #17570, #24470, #10626, #35104, #9, #14100, #38825, #7177, #17795, #42503, #231, #29554, #11779, #39958, #18486, #25850, #32563, #33032, #15251, #36472, #22830, #907, #5278, #43184, #8304, #32790, #22368, #4835, #15475, #43629, #15011, #40173, #29099, #11554, #12224, #18938, #1371, #36924, #33241, #26303, #11996, #36247, #40413, #1142, #29339, #25635, #8763, #22603, #43411, #26062, #8537, #39747, #36705, #5063, #19155, #1583, #15683, #29763, #43840, #19372, #8097, #4605, #4395, #22157, #18700, #7330, #11021, #7552, #28569, #21628, #28317, #35711, #14490, #43105, #42874, #38980, #18409, #22085, #18186, #4090, #39668, #25087, #32261, #21861, #619, #3855, #42658, #25554, #21406, #32488, #10788, #17725, #35951, #45677, #838, #7099, #7783, #39201, #14722, #14937, #36175, #21179, #11241, #28796, #4317, #38739, #11474, #29021, #8016, #25315, #388, #39427, #4535, #35481, #35259, #14029, #17946, #32016, #18628, #28098, #3638, #31788, #42194, #10542, #24618, #158, #14249, #42417, #24863, #32715, #29688, #4757, #43764, #36395, #44003, #8903, #12593, #4990, #1061, #12144, #26670, #15395, #5204, #40093, #1297, #22525, #37066, #33377, #40767, #11704, #12377, #22758, #25985, #5419, #29476, #19512, #43548, #18861, #11914, #15170, #8454, #29918, #36635, #32951, #22970, #26227, #1722, #29259, #16062, #43336, #9125, #1963, #23192, #26454, #39887, #40341, #30145, #5662, #8693, #19082, #40555, #25776, #33611, #44235, #37301, #8229, #36853, #22298, #33172, #1509, #15604, #19292, #15826, #13059, #2885, #6351, #17194, #19981, #23432, #9364, #41004, #23652, #16286, #34057, #27146, #37763, #34527, #9811, #20435, #37533, #16517, #45385, #2194, #10265, #30834, #44698, #44459, #24342, #27363, #41458, #38446, #41233, #34282, #13748, #16977, #30367, #6112, #23878, #19754, #24116, #5892, #31053, #30598, #33840, #37998, #45152, #13514, #27587, #12816, #16753, #41691, #10047, #20202, #2655, #26896, #44928, #2417, #38227, #9592, #13286, #41921, #6573, #20652, #34744, #3104, #31282, #27826, #3796, #10966, #25035, #31520, #4022, #17439, #42137, #35892, #35425, #42606, #43047, #11184, #18358, #38927, #21123, #4267, #99, #14191, #10488, #32439, #564, #31731, #325, #28260, #20875, #39145, #21348, #24806, #7278, #7496, #21567, #42359, #787, #13970, #35207, #6797, #24563, #10727, #17887, #31955, #14428, #28508, #35651, #3583, #18123, #32201, #14887, #14666, #28742, #25255, #28965, #42823, #39365, #11408, #7719, #21799, #25495, #17670, #34972, #3346, #45623, #28043, #38679, #7037, #33947, #25723, #15107, #12939, #43275, #20085, #43494, #36120, #23539, #12700, #37423, #16396, #9250, #44344, #40885, #29195, #41124, #30475, #34159, #22243, #26779, #1234, #8178, #29422, #44579, #23319, #2531, #18577, #5780, #30252, #32890, #27026, #36340, #9477, #4699, #11646, #18800, #22031, #15341, #19867, #11861, #39836, #37642, #33118, #2298, #4485, #5992, #32660, #16636, #30724, #44818, #13175, #1003, #36574, #39607, #7964, #4929, #25934, #40041, #8398, #22466, #19026, #1454, #16170, #34855, #3460, #17087, #45044, #31626, #20993, #13858, #20545, #10376, #27934, #24685, #27470, #30949, #16868, #2776, #31166, #23761, #41568, #34641, #45261, #42030, #17309, #24452, #13399, #23993, #17554, #3218, #13622, #41809, #7159, #2998, #24561, #38116, #9921, #14083, #27256, #28158, #34407, #35086, #24232, #20763, #42251, #3692, #6469, #38558, #10156, #10608, #20313, #38803, #21234, #35314, #38340, #27705, #31399, #31844, #6686, #45504, #41347, #6912, #17779, #216, #9696, #37874, #6222, #42483, #43398, #22353, #7383, #7850, #39494, #28631, #14309, #11298, #32079, #25376, #18006, #25618, #36230, #39944, #32325, #28381, #21928, #36457, #39034, #39730, #4377, #7607, #18685, #42709, #32774, #25141, #447, #11073, #10850, #39254, #11536, #21684, #14552, #4591, #36013, #29081, #24920, #11764, #21459, #8289, #29324, #4820, #8078, #35537, #18467, #25831, #33016, #32546, #679, #22141, #3912, #1122, #15234, #18921, #35778, #892, #4155, #18249, #14779, #28851, #42932, #14995, #43169, #30203, #33672, #44523, #1566, #5048, #36688, #22585, #5260, #43609, #15663, #8748, #19352, #16117, #37123, #2022, #19139, #43821, #23263, #23029, #33436, #15891, #26967, #40397, #19812, #12206, #33226, #37364, #1355, #33895, #8520, #9188, #44063, #40609, #16344, #23489, #29743, #12648, #29977, #5725, #40154, #12881, #30424, #41063, #12429, #1780, #8960, #5943, #22814, #26285, #15458, #36906, #26508, #37589, #5479, #19578, #44293, #29535, #9421, #20034, #26728, #40830, #2249, #11976, #26043, #31112, #6172, #45208, #37822, #45451, #10328, #14037, #6417, #34111, #13571, #28105, #16817, #6637, #41518, #2722, #23940, #38504, #34804, #24628, #27646, #13346, #13122, #38748, #41757, #10107, #7107, #9870, #2945, #42202, #3166, #30668, #20499, #24183, #2478, #6856, #20261, #31343, #44990, #16585, #20710, #13811, #17257, #38290, #27202, #27888, #41986, #24402, #34589, #17034, #44765, #20938, #41296, #35033, #38061, #3410, #10549, #9646, #23711, #34353, #17503, #27421, #31581, #45684, #30895, #39438, #166, #18416, #31796, #10797, #4542, #4098, #11249, #11711, #25563, #32722, #7560, #35489, #18636, #14500, #28577, #24870, #1070, #14945, #395, #14729, #42665, #35266, #25323, #35721, #39208, #18194, #21870, #7792, #11028, #15178, #28325, #3864, #21187, #38987, #25094, #32269, #627, #28803, #42881, #35958, #17954, #4325, #32495, #29267, #845, #29028, #39676, #43344, #43115, #11483, #39894, #8023, #22092, #36182, #32025, #3645, #17732, #14257, #42425, #7337, #21413, #12091, #4487, #39609, #36797, #22033, #43946, #22245, #14889, #1669, #36576, #15556, #40282, #33120, #22468, #19028, #7966, #19238, #8636, #12324, #789, #1456, #8400, #43049, #15343, #29636, #4931, #36342, #32892, #28967 ),
 ( #29861, #4701, #32662, #15774, #11648, #25725, #36122, #26398, #26169, #43277, #11863, #39838, #32441, #43715, #1237, #18802, #43496, #22699, #5154, #8180, #40499, #25497, #1005, #18360, #18579, #25936, #40043, #33325, #8850, #22918, #37009, #15109, #11410, #29197, #2828, #2592, #44397, #23817, #27524, #23596, #27085, #45097, #16451, #12998, #20140, #16225, #20372, #37928, #44634, #19693, #41403, #6285, #44870, #37236, #26610, #34467, #9064, #31000, #9304, #1900, #16920, #37702, #16693, #27309, #34217, #9532, #6051, #40710, #13455, #9753, #41624, #33551, #9981, #30535, #30303, #30091, #24051, #41178, #30779, #5363, #12752, #19924, #19458, #13232, #16009, #23373, #44173, #12536, #23132, #5601, #33785, #26832, #2136, #40939, #37477, #5838, #33999, #2352, #3521, #17374, #17140, #28687, #43, #14136, #42765, #45560, #6975, #32143, #38865, #34692, #10430, #28208, #11126, #42546, #24284, #35368, #3280, #38170, #10666, #3743, #7219, #42302, #31224, #35144, #17831, #24749, #24507, #21060, #20597, #38615, #3050, #21291, #13913, #17606, #14614, #6519, #45321, #13682, #31675, #31458, #31899, #271, #14368, #28448, #27761, #10910, #41863, #10208, #21511, #24978, #39089, #38391, #7438, #3967, #35591, #6740, #18062, #27986, #42081, #20815, #507, #34914, #5049, #19353, #33227, #39308, #29978, #40399, #43822, #12207, #26509, #44065, #1567, #5727, #32385, #40155, #25195, #43610, #15664, #29745, #36907, #33438, #8749, #1781, #8521, #15892, #22815, #23264, #23030, #19140, #44294, #2250, #12430, #40610, #19813, #5261, #8961, #37125, #36690, #40832, #12649, #5480, #22586, #16118, #26729, #19579, #11977, #737, #9189, #29536, #33896, #26286, #21741, #37365, #33674, #2024, #30204, #16345, #30425, #44525, #14836, #7663, #35838, #4214, #18307, #26045, #6419, #17505, #6174, #5944, #12882, #20262, #2723, #35034, #13347, #2479, #16586, #41064, #41987, #20939, #20035, #20501, #38062, #27203, #26968, #9871, #30669, #23941, #44766, #24185, #34805, #38505, #30896, #9423, #34590, #6857, #41297, #31113, #34354, #9647, #16819, #17258, #13572, #3411, #37590, #38291, #2946, #44991, #31344, #23712, #45452, #37823, #13124, #27422, #23490, #41519, #10108, #17035, #45209, #3167, #27647, #41758, #34112, #10329, #6638, #31583, #27890, #20711, #13812, #24403, #24629, #3646, #17733, #38749, #10550, #21188, #45685, #35268, #14038, #28106, #7108, #42203, #19630, #33270, #15503, #2073, #37175, #30027, #36736, #26555, #44112, #40880, #43659, #1399, #33062, #18968, #1616, #39988, #12030, #5094, #15715, #12476, #33489, #40653, #29583, #40210, #33724, #19403, #29800, #12257, #23314, #19184, #16165, #8573, #26098, #30247, #43439, #44339, #4867, #5533, #40441, #36954, #12694, #19861, #22638, #9006, #26337, #26774, #36503, #9243, #37417, #15945, #23076, #5774, #33941, #1835, #2293, #43878, #16391, #11807, #25876, #8336, #22400, #8793, #22861, #5307, #20987, #38108, #6464, #35081, #37869, #45038, #24448, #31159, #27020, #2771, #20542, #3454, #34848, #16630, #27699, #41341, #30470, #2993, #41803, #45256, #34636, #9472, #27464, #10152, #17081, #16863, #13393, #12933, #30944, #41119, #13616, #6216, #41562, #6907, #44573, #23534, #37636, #9916, #9691, #23987, #24227, #38335, #6681, #5987, #20757, #20079, #34154, #13854, #3212, #17303, #2525, #31392, #42026, #45497, #44813, #27931, #23755, #20308, #30717, #10372, #38552, #34400, #13170, #27250, #31623, #21681, #32073, #35533, #3907, #18245, #35772, #39029, #43165, #24680, #31841, #17550, #35311, #7379, #24916, #28626, #25137, #14547, #39251, #211, #7603, #42706, #14991, #14776, #10843, #36010, #39726, #4151, #32320, #11531, #11070, #674, #28847, #28376, #32542, #4373, #42928, #14305, #7846, #18462, #11293, #3688, #38797, #889, #21231, #25614, #21455, #14079, #29078, #42478, #21923, #18002, #17775, #25372, #39330, #39487, #8074, #22137, #36225, #28154, #42246, #10604, #7154, #33668, #1117, #30198, #19572, #44288, #44057, #11761, #1562, #2017, #23257, #15660, #22582, #12425, #18680, #15886, #1775, #26724, #43394, #12202, #26504, #40151, #22348, #8956, #40605, #36903, #43605, #33431, #5256, #16113, #4814, #8284, #39940, #25827, #8515, #15231, #18917, #11971, #36684, #19348, #40393, #29973, #36451, #1352, #23025, #26281, #5044, #19135, #12644, #26038, #37118, #15455, #33012, #5476, #4589, #40825, #29531, #9183, #29737, #43816, #32771, #29318, #33223, #8744, #22811, #41748, #30419, #34796, #6631, #3159, #20255, #37816, #30889, #41981, #30660, #44516, #37358, #44759, #27195, #13805, #6165, #26960, #41058, #19807, #20704, #45444, #12876, #44983, #16810, #5938, #5719, #34346, #9415, #2715, #23483, #2939, #13564, #17250, #9640, #33890, #13338, #31337, #20028, #9862, #13116, #34105, #41288, #10101, #38053, #27883, #16338, #17026, #27415, #23704, #24176, #10322, #41512, #37584, #2471, #2243, #16578, #23934, #6411, #20493, #34582, #31103, #45202, #27640, #38284, #35483, #28099, #35713, #621, #4319, #42419, #24395, #21408, #18411, #7100, #42660, #31790, #38740, #14251, #28798, #25089, #32490, #3403, #4092, #14492, #17727, #42876, #21181, #11243, #35261, #42195, #3640, #6849, #160, #21630, #28319, #10543, #14724, #17948, #39203, #20929, #7785, #35027, #840, #39429, #14939, #18188, #31575, #3857, #21863, #43107, #32018, #10790, #32263, #38497, #25317, #35953, #29023, #17497, #390, #45678, #24865, #24619, #14030, #38982, #11023, #7332, #7554, #28571, #8905, #11706, #15172, #1063, #32717, #15397, #8018, #25778, #18863, #29478, #26229, #1511, #12146, #29261, #8231, #33379, #33174, #43550, #25987, #37068, #4759, #29920, #22300, #43338, #1724, #11476, #44005, #18630, #19294, #8456, #4992, #26456, #33613, #39889, #22760, #40095, #15828, #4537, #22972, #40557, #5421, #22527, #11916, #19084, #16064, #32953, #36397, #25556, #1299, #36637, #15606, #19514, #1965, #30147, #29690, #43766, #40343, #39670, #8695, #36855, #22087, #5206, #12379, #36177, #44700, #33842, #2196, #26672, #27589, #6575, #37303, #37765, #23654, #12818, #44237, #41235, #16288, #9594, #30369, #9813, #20437, #24118, #16519, #12595, #6114, #38229, #26898, #16755, #5894, #41006, #34059, #2887, #44930, #20654, #23194, #23880, #34284, #37535, #16979, #9366, #31055, #23434, #44461, #19983, #40769, #2419, #41460, #30600, #13061, #34529, #20204, #13288, #9127, #41693, #5664, #34746, #13516, #3106, #38000, #19756, #2658, #10050, #17196, #30836, #27148, #6354, #27365, #45154, #28510, #7721, #24344, #38929, #7498, #21125, #3348, #35653, #25037, #17889, #24565, #14430, #31957, #28744, #31522, #34974, #20877, #6799, #35209, #27828, #45625, #38681, #3585, #327, #21350, #42608, #17441, #28045, #21569, #7280, #17672, #101, #11186, #7039, #4024, #42139, #13972, #18125, #31284, #32203, #38448, #39147, #28262, #24808, #566, #21801, #10490, #10968, #14193, #14668 ),
 ( #42825, #25257, #35427, #31733, #39367, #35894, #4269, #42361, #10729, #45387, #3798, #13750, #41923, #10267, #13156, #1654, #26379, #20064, #43928, #33309, #29844, #18780, #30703, #2510, #37853, #11628, #20294, #40264, #8381, #8164, #34386, #36779, #5135, #2756, #36554, #43699, #6202, #12307, #25706, #1439, #19222, #29175, #44799, #15324, #40481, #40027, #43258, #15756, #22901, #37621, #27235, #22227, #26148, #41327, #39818, #15540, #12072, #36323, #8618, #4684, #32870, #4912, #22683, #1217, #29406, #43478, #11846, #25917, #22450, #19009, #33101, #20972, #35068, #41549, #14068, #27451, #6451, #199, #45485, #6893, #7368, #21219, #28364, #3199, #31145, #14291, #10140, #24215, #20530, #42465, #10591, #41790, #10360, #38323, #30931, #3442, #31380, #34836, #17290, #17538, #31612, #6669, #10831, #23974, #38096, #20744, #13378, #45242, #13841, #27920, #45715, #28140, #42235, #34624, #13603, #38783, #38541, #42015, #24436, #24903, #24667, #35300, #27686, #2981, #7140, #16851, #3677, #17068, #17764, #31829, #39018, #21444, #35520, #45025, #9902, #32531, #8271, #42694, #1339, #18906, #15443, #878, #4362, #43154, #8504, #42916, #11059, #3896, #11282, #39476, #26028, #18452, #39239, #7592, #32061, #33000, #11960, #25126, #11520, #29066, #18232, #17988, #14981, #21668, #25604, #35760, #15220, #25816, #29520, #21911, #432, #39714, #43594, #32307, #22126, #25359, #662, #7834, #22336, #4578, #40139, #28612, #29308, #8064, #35998, #36438, #14763, #4802, #28836, #4139, #36214, #14535, #18670, #1106, #32759, #43381, #39928, #11749, #22572, #33214, #20019, #1551, #16566, #5928, #30649, #30410, #43807, #33656, #34095, #9631, #2007, #8945, #44505, #5035, #2233, #33880, #13106, #29729, #44278, #12864, #26496, #8735, #41047, #26947, #23245, #29963, #19796, #37348, #2462, #5247, #40384, #26271, #12191, #9405, #22801, #44747, #40596, #15649, #27187, #9168, #16328, #23473, #5709, #40813, #37573, #19337, #41278, #36675, #19127, #33422, #1764, #16104, #15874, #44047, #12415, #12635, #26714, #23013, #37108, #5466, #19561, #30188, #20244, #41738, #45434, #28307, #28087, #9853, #20921, #34571, #23695, #41971, #35017, #24385, #13797, #2703, #20696, #3395, #10313, #10091, #38274, #6156, #24167, #34335, #27874, #45194, #34787, #148, #37807, #14238, #30878, #6621, #2931, #3150, #17241, #38489, #6841, #16799, #17488, #44974, #13328, #7088, #31327, #31567, #42405, #42183, #35250, #45667, #38044, #21169, #17018, #31095, #27405, #3628, #14019, #13556, #10533, #27629, #41502, #24609, #38726, #17715, #31778, #23923, #6402, #20484, #36385, #17936, #25078, #10776, #28558, #610, #18175, #21847, #18400, #39417, #32480, #39192, #830, #25305, #8220, #8009, #4076, #29249, #32941, #29012, #14929, #4747, #35940, #43095, #25544, #21618, #25767, #43326, #4308, #7542, #1052, #11694, #4527, #42649, #376, #32005, #14711, #7321, #35700, #32251, #28787, #39657, #11461, #22075, #14478, #42865, #32706, #36166, #11232, #7769, #18851, #18619, #39879, #15158, #11011, #22289, #24853, #1287, #15386, #29465, #38971, #21397, #35471, #3845, #19072, #9111, #26443, #2182, #36624, #40990, #12801, #9350, #40542, #43990, #37053, #2402, #36842, #4979, #43538, #5192, #33366, #19970, #12367, #33160, #1497, #25976, #26883, #5880, #15595, #5405, #22957, #12133, #11905, #8892, #29677, #19501, #43755, #23180, #19742, #23420, #15815, #40084, #33598, #37521, #26215, #16051, #19279, #40330, #1711, #16274, #44221, #34045, #22514, #37288, #1949, #29905, #30353, #8683, #44445, #22747, #30133, #12579, #8444, #26656, #40752, #5648, #33829, #16503, #30822, #27352, #44685, #20419, #13043, #2873, #34514, #16964, #23865, #27133, #16739, #31041, #30583, #41446, #44916, #41222, #9579, #23639, #37750, #6099, #2642, #20189, #34269, #13274, #9797, #37982, #6337, #12720, #19427, #9274, #26801, #23564, #26362, #29827, #22666, #44137, #2101, #30745, #30500, #12286, #23341, #36978, #26128, #44365, #37444, #40904, #16191, #5119, #23101, #5804, #19890, #12502, #40676, #8600, #26578, #36763, #30272, #1866, #37200, #2554, #40243, #16661, #33294, #9030, #5331, #5566, #19658, #33968, #2320, #19207, #16418, #1639, #15740, #9500, #33751, #44602, #44839, #12964, #37667, #27050, #40466, #6017, #33517, #15972, #43909, #20108, #41148, #30054, #34184, #8818, #22887, #17333, #27730, #31192, #45288, #13880, #31422, #34664, #38831, #20339, #27493, #13202, #30972, #3024, #20569, #24255, #20786, #41832, #34880, #41593, #3245, #10178, #10632, #10400, #6490, #31646, #35336, #45528, #27956, #7181, #38363, #42052, #24476, #24021, #28179, #14, #6709, #9948, #3485, #14105, #6938, #45069, #34432, #42271, #16891, #21256, #17110, #9720, #24709, #38583, #21019, #35109, #17575, #3713, #17800, #2799, #31866, #27280, #41373, #23785, #37899, #6249, #38139, #13424, #13646, #7875, #21952, #4840, #7629, #14799, #39963, #912, #18275, #15015, #36037, #29104, #3933, #42730, #22161, #4400, #4180, #28873, #25854, #39274, #18704, #11094, #18028, #36251, #237, #32795, #7406, #8100, #42954, #39519, #15254, #22372, #21480, #11557, #11321, #4608, #39057, #43415, #29343, #11783, #25399, #703, #18491, #18942, #21707, #35558, #14333, #35802, #32348, #36477, #32567, #32106, #474, #28411, #8309, #42509, #14577, #43187, #25638, #28652, #10875, #39750, #25165, #1147, #24941, #44313, #9211, #12904, #5282, #33036, #29997, #26990, #15687, #5505, #8766, #1587, #22834, #37388, #33695, #41090, #12001, #12667, #23047, #26308, #5744, #29768, #19831, #43846, #5067, #12228, #15479, #36928, #30222, #19376, #19159, #23286, #26529, #2043, #29558, #16363, #43633, #9443, #2266, #23507, #26748, #40178, #44084, #30443, #5962, #12449, #33459, #40849, #1375, #33914, #44544, #37609, #26066, #40628, #8541, #1805, #33244, #22608, #36709, #19599, #15911, #16136, #8979, #37146, #20281, #23730, #9665, #41316, #23961, #16604, #34373, #27438, #20729, #37843, #16839, #42001, #10126, #38082, #34608, #45700, #13365, #38524, #30916, #6190, #10344, #20052, #6876, #27222, #27905, #17053, #13589, #35053, #42220, #2743, #31363, #2966, #24419, #13143, #17523, #3426, #31597, #31131, #20517, #27671, #24648, #41537, #45011, #34130, #9888, #6439, #10571, #45228, #24200, #38307, #2498, #14053, #28123, #6655, #34822, #3185, #17273, #30688, #45470, #13828, #20955, #38765, #44789, #29047, #32741, #25109, #7123, #4118, #1087, #35504, #25340, #14517, #21428, #42679, #11500, #7812, #15200, #31812, #18433, #42898, #414, #25582, #3879, #39696, #17971, #24887, #32043, #35283, #28595, #4342, #11043, #39001, #43133, #643, #21891, #3660, #36198, #17748, #29287, #22108, #43364, #860, #14274, #18213, #4561, #25799, #32287, #39223, #14963, #21202, #32512, #8043, #11729, #181, #14744, #18652, #7576, #7351, #28344, #42444, #39456, #21652, #35978, #10814, #35739, #28818, #11265 ),
 ( #33405, #19321, #8484, #39912, #36880, #11942, #5230, #43574, #5447, #16087, #19780, #12173, #8254, #1749, #33865, #22554, #12400, #1534, #36659, #29714, #44262, #40581, #2218, #18886, #19542, #29944, #33197, #12620, #5019, #26698, #19110, #26010, #15631, #22320, #43791, #37092, #26254, #40119, #30171, #15856, #8927, #36420, #23225, #4784, #16312, #9153, #30394, #33637, #1321, #44028, #37330, #12843, #26479, #40367, #1990, #32981, #40795, #5692, #44487, #15424, #22997, #29502, #8719, #22785, #31308, #20680, #13539, #20229, #10076, #27613, #25007, #27173, #30632, #16547, #2445, #30863, #23457, #41261, #34317, #44957, #41722, #17003, #24147, #44727, #23679, #3133, #2913, #13314, #41485, #7467, #2686, #45416, #37790, #13090, #17222, #26927, #13777, #34081, #34770, #23908, #20465, #41952, #3993, #9617, #38256, #9839, #27856, #20004, #39118, #10293, #21539, #38029, #27390, #6139, #16783, #35621, #41030, #18091, #6384, #32173, #34554, #31080, #536, #9389, #45178, #6602, #37556, #5914, #7691, #12063, #29613, #26137, #43248, #15077, #8155, #19214, #7938, #21771, #14641, #22005, #4460, #36771, #29164, #4242, #18332, #42795, #43690, #22674, #35865, #22218, #39808, #28938, #28714, #11619, #32412, #25697, #761, #25908, #36543, #40252, #32631, #11155, #36311, #8609, #43015, #32857, #36095, #11380, #18549, #19001, #15315, #5126, #39337, #40017, #4673, #974, #33093, #25462, #1430, #39581, #14862, #18771, #25225, #1207, #11837, #29397, #43469, #4902, #8369, #22438, #15532, #33301, #43916, #27285, #16667, #41378, #41156, #8825, #44372, #44846, #20344, #12727, #19665, #9507, #15747, #12971, #44610, #23791, #40473, #9280, #23571, #37209, #19433, #6025, #37676, #33976, #40683, #30507, #2327, #13208, #1873, #5338, #36985, #22893, #5573, #12295, #15980, #9037, #33758, #16426, #37452, #27060, #33525, #44145, #20116, #23349, #2110, #16199, #9727, #23107, #34192, #29835, #37903, #30064, #30279, #26585, #26807, #40913, #5811, #19899, #26371, #2562, #12509, #30752, #6257, #1646, #24481, #24946, #38834, #240, #20790, #3028, #31870, #27734, #41838, #38144, #14337, #28182, #13653, #27960, #10183, #2804, #38587, #3249, #6713, #34885, #35114, #6943, #24259, #28415, #41598, #17115, #34438, #6495, #38367, #17341, #45533, #42056, #31427, #10404, #31196, #21026, #13886, #42513, #31649, #3491, #7187, #10878, #17579, #17, #39061, #14108, #42274, #10635, #45294, #3716, #21261, #24716, #35340, #17803, #7409, #16895, #20573, #9955, #30976, #34669, #45074, #13429, #27499, #24025, #39756, #18708, #43419, #36254, #25642, #22165, #11098, #22376, #11786, #1379, #3936, #12006, #32572, #706, #477, #26069, #29107, #43191, #40183, #28877, #36041, #15482, #4612, #18031, #39524, #11560, #21484, #25857, #7632, #32798, #32352, #35561, #8104, #1152, #15257, #29346, #14582, #18494, #39967, #8312, #7879, #4404, #32112, #21955, #28656, #36481, #42957, #916, #43636, #42734, #25168, #15018, #14803, #39278, #21710, #4846, #18945, #35807, #11324, #33041, #29562, #4183, #18278, #25402, #30226, #13147, #12909, #40419, #5748, #19379, #8548, #26752, #19837, #9218, #44317, #33247, #5510, #33919, #40855, #26533, #23052, #36712, #40631, #5072, #12672, #30002, #19606, #30696, #22612, #44792, #15691, #8983, #33463, #37150, #33699, #23293, #37394, #1592, #2270, #19163, #43851, #37613, #2049, #16368, #27228, #26997, #20055, #16143, #22839, #5966, #1811, #15918, #12234, #34133, #30446, #44089, #44548, #12454, #29774, #41093, #9448, #23512, #2501, #16608, #26313, #8771, #36932, #5286, #9892, #41320, #13371, #31136, #2971, #6662, #3192, #24205, #17281, #23966, #31370, #10132, #38774, #38531, #34616, #14060, #17756, #13834, #45478, #35291, #20735, #27911, #10352, #6443, #10580, #28132, #34828, #38088, #31604, #42227, #35060, #27443, #16843, #24658, #45018, #21210, #45234, #37846, #7132, #42008, #6885, #17531, #24428, #20962, #3434, #30922, #3669, #31820, #191, #13594, #9670, #38315, #14283, #20522, #23735, #17060, #27677, #41782, #6194, #20286, #34379, #2748, #41541, #18443, #21661, #32750, #42685, #1097, #39231, #422, #25117, #10823, #7584, #25595, #11052, #14527, #4569, #21903, #43143, #24895, #11740, #39009, #8263, #43374, #22328, #22117, #35512, #25350, #25807, #1330, #39464, #652, #36205, #42456, #39705, #8052, #4793, #21436, #35987, #18660, #18222, #28603, #15211, #29299, #14972, #35751, #11509, #29057, #39920, #4130, #32051, #17981, #3887, #32298, #7360, #14753, #28827, #42907, #36429, #32521, #18896, #11274, #7824, #32992, #4353, #869, #28352, #41038, #8729, #33873, #26264, #33208, #37341, #15434, #2226, #22565, #23235, #12409, #8936, #30402, #37565, #36669, #26706, #44039, #19790, #8494, #12857, #44496, #26938, #26489, #15866, #23007, #20012, #22794, #5029, #29512, #36889, #5241, #5922, #29955, #19119, #1545, #43584, #9399, #23466, #15640, #37101, #40590, #29723, #11952, #5457, #43801, #19552, #12183, #40805, #5703, #34088, #26020, #33648, #2000, #33414, #1758, #16096, #30180, #19331, #40130, #40378, #44271, #12628, #9162, #16321, #9846, #13548, #10084, #31088, #24157, #30870, #38267, #17011, #45659, #45425, #41493, #20912, #24600, #20688, #6613, #42175, #27622, #34779, #17232, #13322, #17478, #35009, #41730, #16793, #38481, #3385, #41961, #34325, #23688, #31559, #6148, #28079, #6393, #44740, #14009, #3141, #13787, #24377, #31319, #27866, #10304, #37799, #10524, #6832, #38718, #30642, #7078, #21159, #27398, #27182, #2454, #16557, #13098, #41270, #23916, #45186, #9625, #20238, #2696, #20477, #44966, #38037, #34564, #2922, #32472, #368, #35242, #7761, #821, #35931, #25295, #14229, #32242, #14921, #21838, #7534, #4068, #17708, #21608, #31769, #11224, #11003, #602, #11686, #3620, #25759, #42398, #35691, #14469, #18166, #14703, #39407, #4301, #28298, #29002, #140, #24844, #18611, #28779, #18392, #39871, #39648, #1043, #42857, #3836, #32696, #28548, #42642, #38963, #15150, #43086, #25070, #11452, #39184, #25535, #17926, #7313, #8001, #22067, #36157, #10767, #29239, #21390, #43317, #4519, #8212, #35463, #31996, #19270, #19731, #40981, #33358, #40321, #16042, #36376, #33589, #19491, #44434, #15378, #29896, #44212, #12124, #40074, #26646, #30124, #8883, #15587, #5396, #22948, #33819, #22506, #25968, #11896, #43530, #26207, #18843, #36615, #29670, #8674, #37045, #12357, #1939, #8436, #19063, #12571, #43981, #22739, #36832, #2172, #43745, #40743, #33152, #4970, #9100, #22281, #23169, #29457, #37279, #1701, #15806, #5637, #12789, #1489, #16264, #5184, #30342, #26434, #26871, #4739, #32933, #40534, #1278, #2864, #13948, #2633, #2392, #9340, #16730, #44907, #31497, #9789, #44676, #13033, #37512, #38427, #17419, #16491, #16955, #34505, #23630, #23410, #6328, #27123, #20409, #41214, #20632, #31262, #34951, #27344, #5871, #31033, #3322, #37739, #27563 ),
 ( #20853, #37971, #23855, #45132, #28023, #30813, #30573, #19961, #13266, #41437, #45601, #13490, #9570, #6091, #34035, #6777, #20179, #34258, #41668, #10025, #24091, #38206, #6554, #34725, #3084, #17175, #45364, #13726, #27803, #41898, #10244, #24323, #22014, #24788, #14650, #3777, #10705, #31936, #772, #42806, #4469, #21105, #7701, #32185, #35406, #14872, #38905, #28946, #7258, #14172, #21329, #24543, #17868, #39347, #306, #28242, #18341, #35631, #11165, #38656, #25474, #7014, #36105, #11390, #18560, #35876, #3563, #39127, #39592, #15089, #7479, #14408, #4251, #10467, #21781, #32422, #32642, #35187, #4003, #43027, #28489, #42337, #7947, #984, #28726, #42587, #25237, #42117, #17651, #10947, #81, #31712, #25019, #21548, #18103, #546, #39380, #22257, #4713, #21363, #10979, #39159, #22711, #30316, #33563, #1913, #16021, #8412, #44185, #4944, #36808, #26180, #40294, #37249, #19708, #6064, #6756, #41640, #38184, #13926, #21075, #20153, #28000, #17389, #6530, #13244, #34929, #45576, #38405, #30791, #34230, #31472, #2605, #24522, #2841, #41191, #42095, #17153, #41877, #20829, #13696, #3063, #45334, #16705, #10446, #3294, #38632, #27100, #35158, #9996, #37943, #23608, #3537, #20610, #34705, #17622, #6300, #13468, #6991, #27774, #9545, #16934, #31239, #44648, #13010, #44883, #10221, #9764, #37715, #24299, #27322, #41415, #20383, #34482, #24066, #31013, #45111, #27538, #519, #14150, #3979, #28220, #7676, #7451, #42778, #8144, #57, #22207, #38878, #18074, #10923, #32156, #28699, #35851, #4227, #10679, #28924, #42315, #21304, #15064, #14627, #21755, #36300, #36082, #43234, #11139, #283, #29151, #24991, #39101, #35380, #11605, #25448, #21526, #25209, #35604, #24762, #18320, #39321, #32400, #750, #14848, #43002, #11367, #25684, #7234, #14382, #31690, #3755, #39569, #7923, #21994, #4449, #18537, #32617, #28461, #959, #39796, #4657, #17844, #31911, #42560, #40897, #36970, #40457, #26792, #29819, #26353, #33509, #29599, #18755, #23092, #30264, #19199, #33079, #16183, #12048, #26120, #22421, #44356, #12493, #43677, #12278, #40234, #32843, #22878, #33286, #36755, #1631, #19418, #1857, #8591, #1194, #25894, #1416, #15301, #36526, #22657, #15730, #43900, #8810, #15965, #44128, #15519, #26570, #9022, #43457, #37192, #5558, #2094, #11824, #40005, #8355, #4885, #35046, #3421, #17516, #31807, #42438, #25057, #123, #20896, #42627, #7519, #349, #38465, #27849, #39169, #24362, #32226, #10509, #3126, #35673, #24828, #3820, #28532, #21373, #10751, #7298, #41946, #21593, #10989, #586, #34764, #42844, #17693, #45646, #31302, #11208, #14213, #28282, #25280, #13995, #21145, #14688, #35449, #17215, #24585, #42382, #6595, #4049, #6818, #17910, #17461, #20673, #38948, #31978, #14454, #18147, #45409, #31754, #28764, #13771, #38702, #34994, #3370, #7062, #30442, #38081, #23729, #45010, #6875, #9442, #2497, #30687, #20280, #41315, #34372, #2965, #17052, #31130, #37842, #45227, #16838, #10125, #45469, #3184, #24003, #16644, #3227, #38125, #35786, #21001, #25149, #28392, #10860, #32334, #39503, #35094, #7616, #224, #687, #10385, #28859, #42940, #11307, #24928, #17787, #39042, #45514, #10618, #14091, #13867, #21242, #3700, #7860, #31852, #7391, #3920, #27942, #25385, #42039, #18015, #32087, #29544, #1130, #18476, #15466, #22149, #43620, #8087, #15672, #36914, #12436, #18930, #32555, #11986, #26515, #15243, #22593, #25840, #29332, #39952, #5268, #29753, #8967, #29089, #43830, #8528, #33025, #19360, #26053, #33446, #12213, #36237, #899, #11544, #25627, #39737, #4598, #12891, #3596, #41074, #27311, #9065, #41625, #23133, #38171, #27525, #6520, #6287, #19696, #9533, #9982, #31225, #23597, #30536, #20373, #26612, #23818, #9754, #34693, #5602, #20141, #34469, #2353, #30304, #16921, #2829, #44871, #5839, #41404, #13233, #24053, #12753, #16226, #2137, #33786, #16453, #37237, #26833, #19925, #44635, #37929, #2593, #31001, #44399, #9305, #45099, #34219, #12999, #27087, #20598, #34000, #13456, #23375, #3051, #17141, #16694, #12537, #40940, #40711, #37478, #41179, #37703, #6052, #30780, #24508, #24285, #35839, #7220, #21292, #4215, #6976, #14137, #39310, #272, #41865, #17607, #35369, #18308, #3968, #31459, #42548, #10431, #45322, #17832, #10911, #14369, #3745, #38392, #42303, #24979, #31900, #31677, #28209, #27762, #44, #10209, #28449, #21061, #10667, #21742, #13683, #6741, #20816, #24750, #38616, #38866, #39090, #7439, #21513, #34915, #35592, #3281, #17375, #28688, #18063, #32144, #45561, #508, #11127, #14616, #13915, #42766, #35145, #3522, #27987, #25196, #7664, #42082, #25884, #39785, #738, #36515, #1183, #4648, #18743, #33069, #4876, #8134, #12267, #39557, #947, #32387, #4437, #22197, #36289, #43448, #39996, #15292, #8345, #15050, #22411, #29376, #29808, #29591, #25672, #5103, #8802, #18979, #1408, #26344, #11815, #15511, #43668, #43221, #1623, #19191, #12040, #29139, #22646, #33277, #26107, #18524, #7912, #15722, #36071, #40447, #32832, #28909, #43888, #40223, #8582, #36745, #11594, #22869, #36961, #5314, #14837, #42990, #11355, #25435, #21982, #32605, #13405, #30482, #27032, #34166, #30256, #34414, #37880, #12946, #33734, #9703, #20320, #13182, #5546, #40660, #6228, #23084, #45050, #23324, #15954, #2782, #37649, #16642, #41353, #2537, #23546, #20091, #9013, #16874, #23767, #27477, #1847, #9927, #44585, #44348, #44119, #24000, #41131, #9483, #38122, #26784, #33952, #41575, #30730, #30037, #37428, #5998, #19410, #30956, #19640, #44824, #12704, #33497, #27264, #12484, #26562, #37182, #2083, #16402, #16175, #40889, #5785, #2303, #9256, #19874, #34648, #28164, #27940, #17560, #28636, #20552, #42715, #13628, #38566, #31406, #6920, #3468, #10615, #24692, #31173, #3698, #17094, #41816, #35543, #35092, #42257, #11079, #10857, #18013, #20999, #20770, #3918, #45511, #13865, #10162, #32085, #222, #42037, #5370, #10383, #3006, #38810, #31632, #24459, #14089, #7166, #21240, #35320, #456, #27712, #34863, #6475, #24238, #17785, #31850, #14316, #28388, #42491, #45269, #14560, #38347, #25147, #21465, #6692, #24926, #3225, #39040, #17315, #7389, #25625, #898, #11770, #7614, #43404, #29330, #11984, #18257, #22147, #39950, #32553, #28857, #22359, #25838, #32781, #36021, #15241, #1128, #1362, #11305, #42938, #14785, #32331, #15001, #21691, #25383, #4384, #29088, #8295, #4597, #36464, #39500, #7858, #4826, #36236, #43175, #11543, #29543, #18474, #18928, #21936, #39736, #33024, #39259, #15465, #8085, #43618, #18692, #26052, #40163, #35784, #8527, #4163, #685, #39191, #27873, #32250, #4075, #609, #17714, #35249, #28306, #39416, #28086, #41970, #34786, #42182, #24608, #11231, #3627, #24384, #38488, #17240, #18174, #42864, #10312, #42404, #14237, #3394, #3149, #31777, #6840, #147, #20920, #375, #11010, #14710, #7087, #31326, #10775 ) ),
 .UNSPECIFIED., .T., .F., .T. ) 
 B_SPLINE_SURFACE_WITH_KNOTS ( ( 4, 3, 4 ),
 ( 3, 2, 2, 2, 2, 2, 2, 2, 2, 2, 2, 2, 2, 2, 2, 2, 2, 2, 2, 2, 2, 2, 2, 2, 2, 2, 2, 2, 2, 2, 2, 2, 2, 2, 2, 2, 2, 2, 2, 2, 2, 2, 2, 2, 2, 2, 2, 2, 2, 2, 2, 2, 2, 2, 2, 2, 2, 2, 2, 2, 2, 2, 2, 2, 2, 2, 2, 2, 2, 2, 2, 2, 2, 2, 2, 2, 2, 2, 2, 2, 2, 2, 2, 2, 2, 2, 2, 2, 2, 2, 2, 2, 2, 2, 2, 2, 2, 2, 2, 2, 2, 2, 2, 2, 2, 2, 2, 2, 2, 2, 2, 2, 2, 2, 2, 2, 2, 2, 2, 2, 2, 2, 2, 2, 2, 2, 2, 2, 2, 2, 2, 2, 2, 2, 2, 2, 2, 2, 2, 2, 2, 2, 2, 2, 2, 2, 2, 2, 2, 2, 2, 2, 2, 2, 2, 2, 2, 2, 2, 2, 2, 2, 2, 2, 2, 2, 2, 2, 2, 2, 2, 2, 2, 2, 2, 2, 2, 2, 2, 2, 2, 2, 2, 2, 2, 2, 2, 2, 2, 2, 2, 2, 2, 2, 2, 2, 2, 2, 2, 2, 2, 2, 2, 2, 2, 2, 2, 2, 2, 2, 2, 2, 2, 2, 2, 2, 2, 2, 2, 2, 2, 2, 2, 2, 2, 2, 2, 2, 2, 2, 2, 2, 2, 2, 2, 2, 2, 2, 2, 2, 2, 2, 2, 2, 2, 2, 2, 2, 2, 2, 2, 2, 2, 2, 2, 2, 2, 2, 2, 2, 2, 2, 2, 2, 2, 2, 2, 2, 2, 2, 2, 2, 2, 2, 2, 2, 2, 2, 2, 2, 2, 2, 2, 2, 2, 2, 2, 2, 2, 2, 2, 2, 2, 2, 2, 2, 2, 2, 2, 2, 2, 2, 2, 2, 2, 2, 2, 2, 2, 2, 2, 2, 2, 2, 2, 2, 2, 2, 2, 2, 2, 2, 2, 2, 2, 2, 2, 2, 2, 2, 2, 2, 2, 2, 2, 2, 2, 2, 2, 2, 2, 2, 2, 2, 2, 2, 2, 2, 2, 2, 2, 2, 2, 2, 2, 2, 2, 2, 2, 2, 2, 2, 2, 2, 2, 2, 2, 2, 2, 2, 2, 2, 2, 2, 2, 2, 2, 2, 2, 2, 2, 2, 2, 2, 2, 2, 2, 2, 2, 2, 2, 2, 2, 2, 2, 2, 2, 2, 2, 2, 2, 2, 2, 2, 2, 2, 2, 2, 2, 2, 2, 2, 2, 2, 2, 2, 2, 2, 2, 2, 2, 2, 2, 2, 2, 2, 2, 2, 2, 2, 2, 3 ),
 ( 0.000000000000000000, 0.5000000000000000000, 1.000000000000000000 ),
 ( 0.000000000000000000, 0.002272727272727272617, 0.004545454545454545234, 0.006818181818181817851, 0.009090909090909090468, 0.01136363636363636395, 0.01363636363636363570, 0.01590909090909090745, 0.01818181818181818094, 0.02045454545454545442, 0.02272727272727272790, 0.02500000000000000139, 0.02727272727272727140, 0.02954545454545454489, 0.03181818181818181490, 0.03409090909090908839, 0.03636363636363636187, 0.03863636363636363535, 0.04090909090909090884, 0.04318181818181818232, 0.04545454545454545581, 0.04772727272727272929, 0.05000000000000000278, 0.05227272727272726932, 0.05454545454545454281, 0.05681818181818181629, 0.05909090909090908977, 0.06136363636363636326, 0.06363636363636362980, 0.06590909090909090329, 0.06818181818181817677, 0.07045454545454545026, 0.07272727272727272374, 0.07499999999999999722, 0.07727272727272727071, 0.07954545454545454419, 0.08181818181818181768, 0.08409090909090909116, 0.08636363636363636465, 0.08863636363636363813, 0.09090909090909091161, 0.09318181818181818510, 0.09545454545454545858, 0.09772727272727273207, 0.1000000000000000056, 0.1022727272727272790, 0.1045454545454545386, 0.1068181818181818121, 0.1090909090909090856, 0.1113636363636363591, 0.1136363636363636326, 0.1159090909090909061, 0.1181818181818181795, 0.1204545454545454530, 0.1227272727272727265, 0.1250000000000000000, 0.1272727272727272596, 0.1295454545454545470, 0.1318181818181818066, 0.1340909090909090939, 0.1363636363636363535, 0.1386363636363636409, 0.1409090909090909005, 0.1431818181818181879, 0.1454545454545454475, 0.1477272727272727348, 0.1499999999999999944, 0.1522727272727272818, 0.1545454545454545414, 0.1568181818181818288, 0.1590909090909090884, 0.1613636363636363757, 0.1636363636363636354, 0.1659090909090909227, 0.1681818181818181823, 0.1704545454545454419, 0.1727272727272727293, 0.1749999999999999889, 0.1772727272727272763, 0.1795454545454545359, 0.1818181818181818232, 0.1840909090909090828, 0.1863636363636363702, 0.1886363636363636298, 0.1909090909090909172, 0.1931818181818181768, 0.1954545454545454641, 0.1977272727272727237, 0.2000000000000000111, 0.2022727272727272707, 0.2045454545454545581, 0.2068181818181818177, 0.2090909090909090773, 0.2113636363636363646, 0.2136363636363636243, 0.2159090909090909116, 0.2181818181818181712, 0.2204545454545454586, 0.2227272727272727182, 0.2250000000000000056, 0.2272727272727272652, 0.2295454545454545525, 0.2318181818181818121, 0.2340909090909090995, 0.2363636363636363591, 0.2386363636363636465, 0.2409090909090909061, 0.2431818181818181934, 0.2454545454545454530, 0.2477272727272727404, 0.2500000000000000000, 0.2522727272727272596, 0.2545454545454545192, 0.2568181818181818343, 0.2590909090909090939, 0.2613636363636363535, 0.2636363636363636131, 0.2659090909090909283, 0.2681818181818181879, 0.2704545454545454475, 0.2727272727272727071, 0.2750000000000000222, 0.2772727272727272818, 0.2795454545454545414, 0.2818181818181818010, 0.2840909090909091161, 0.2863636363636363757, 0.2886363636363636354, 0.2909090909090908950, 0.2931818181818181546, 0.2954545454545454697, 0.2977272727272727293, 0.2999999999999999889, 0.3022727272727272485, 0.3045454545454545636, 0.3068181818181818232, 0.3090909090909090828, 0.3113636363636363424, 0.3136363636363636576, 0.3159090909090909172, 0.3181818181818181768, 0.3204545454545454364, 0.3227272727272727515, 0.3250000000000000111, 0.3272727272727272707, 0.3295454545454545303, 0.3318181818181818454, 0.3340909090909091050, 0.3363636363636363646, 0.3386363636363636243, 0.3409090909090908839, 0.3431818181818181990, 0.3454545454545454586, 0.3477272727272727182, 0.3499999999999999778, 0.3522727272727272929, 0.3545454545454545525, 0.3568181818181818121, 0.3590909090909090717, 0.3613636363636363869, 0.3636363636363636465, 0.3659090909090909061, 0.3681818181818181657, 0.3704545454545454808, 0.3727272727272727404, 0.3750000000000000000, 0.3772727272727272596, 0.3795454545454545192, 0.3818181818181818343, 0.3840909090909090939, 0.3863636363636363535, 0.3886363636363636131, 0.3909090909090909283, 0.3931818181818181879, 0.3954545454545454475, 0.3977272727272727071, 0.4000000000000000222, 0.4022727272727272818, 0.4045454545454545414, 0.4068181818181818010, 0.4090909090909091161, 0.4113636363636363757, 0.4136363636363636354, 0.4159090909090908950, 0.4181818181818181546, 0.4204545454545454697, 0.4227272727272727293, 0.4249999999999999889, 0.4272727272727272485, 0.4295454545454545636, 0.4318181818181818232, 0.4340909090909090828, 0.4363636363636363424, 0.4386363636363636576, 0.4409090909090909172, 0.4431818181818181768, 0.4454545454545454364, 0.4477272727272727515, 0.4500000000000000111, 0.4522727272727272707, 0.4545454545454545303, 0.4568181818181818454, 0.4590909090909091050, 0.4613636363636363646, 0.4636363636363636243, 0.4659090909090908839, 0.4681818181818181990, 0.4704545454545454586, 0.4727272727272727182, 0.4749999999999999778, 0.4772727272727272929, 0.4795454545454545525, 0.4818181818181818121, 0.4840909090909090717, 0.4863636363636363869, 0.4886363636363636465, 0.4909090909090909061, 0.4931818181818181657, 0.4954545454545454808, 0.4977272727272727404, 0.5000000000000000000, 0.5022727272727273151, 0.5045454545454545192, 0.5068181818181818343, 0.5090909090909090384, 0.5113636363636363535, 0.5136363636363636687, 0.5159090909090908728, 0.5181818181818181879, 0.5204545454545455030, 0.5227272727272727071, 0.5250000000000000222, 0.5272727272727272263, 0.5295454545454545414, 0.5318181818181818565, 0.5340909090909090606, 0.5363636363636363757, 0.5386363636363636909, 0.5409090909090908950, 0.5431818181818182101, 0.5454545454545454142, 0.5477272727272727293, 0.5500000000000000444, 0.5522727272727272485, 0.5545454545454545636, 0.5568181818181817677, 0.5590909090909090828, 0.5613636363636363980, 0.5636363636363636020, 0.5659090909090909172, 0.5681818181818182323, 0.5704545454545454364, 0.5727272727272727515, 0.5749999999999999556, 0.5772727272727272707, 0.5795454545454545858, 0.5818181818181817899, 0.5840909090909091050, 0.5863636363636363091, 0.5886363636363636243, 0.5909090909090909394, 0.5931818181818181435, 0.5954545454545454586, 0.5977272727272727737, 0.5999999999999999778, 0.6022727272727272929, 0.6045454545454544970, 0.6068181818181818121, 0.6090909090909091272, 0.6113636363636363313, 0.6136363636363636465, 0.6159090909090909616, 0.6181818181818181657, 0.6204545454545454808, 0.6227272727272726849, 0.6250000000000000000, 0.6272727272727273151, 0.6295454545454545192, 0.6318181818181818343, 0.6340909090909090384, 0.6363636363636363535, 0.6386363636363636687, 0.6409090909090908728, 0.6431818181818181879, 0.6454545454545455030, 0.6477272727272727071, 0.6500000000000000222, 0.6522727272727272263, 0.6545454545454545414, 0.6568181818181818565, 0.6590909090909090606, 0.6613636363636363757, 0.6636363636363636909, 0.6659090909090908950, 0.6681818181818182101, 0.6704545454545454142, 0.6727272727272727293, 0.6750000000000000444, 0.6772727272727272485, 0.6795454545454545636, 0.6818181818181817677, 0.6840909090909090828, 0.6863636363636363980, 0.6886363636363636020, 0.6909090909090909172, 0.6931818181818182323, 0.6954545454545454364, 0.6977272727272727515, 0.6999999999999999556, 0.7022727272727272707, 0.7045454545454545858, 0.7068181818181817899, 0.7090909090909091050, 0.7113636363636363091, 0.7136363636363636243, 0.7159090909090909394, 0.7181818181818181435, 0.7204545454545454586, 0.7227272727272727737, 0.7249999999999999778, 0.7272727272727272929, 0.7295454545454544970, 0.7318181818181818121, 0.7340909090909091272, 0.7363636363636363313, 0.7386363636363636465, 0.7409090909090909616, 0.7431818181818181657, 0.7454545454545454808, 0.7477272727272726849, 0.7500000000000000000, 0.7522727272727273151, 0.7545454545454545192, 0.7568181818181818343, 0.7590909090909090384, 0.7613636363636363535, 0.7636363636363636687, 0.7659090909090908728, 0.7681818181818181879, 0.7704545454545455030, 0.7727272727272727071, 0.7750000000000000222, 0.7772727272727272263, 0.7795454545454545414, 0.7818181818181818565, 0.7840909090909090606, 0.7863636363636363757, 0.7886363636363636909, 0.7909090909090908950, 0.7931818181818182101, 0.7954545454545454142, 0.7977272727272727293, 0.8000000000000000444, 0.8022727272727272485, 0.8045454545454545636, 0.8068181818181817677, 0.8090909090909090828, 0.8113636363636363980, 0.8136363636363636020, 0.8159090909090909172, 0.8181818181818182323, 0.8204545454545454364, 0.8227272727272727515, 0.8249999999999999556, 0.8272727272727272707, 0.8295454545454545858, 0.8318181818181817899, 0.8340909090909091050, 0.8363636363636363091, 0.8386363636363636243, 0.8409090909090909394, 0.8431818181818181435, 0.8454545454545454586, 0.8477272727272727737, 0.8499999999999999778, 0.8522727272727272929, 0.8545454545454544970, 0.8568181818181818121, 0.8590909090909091272, 0.8613636363636363313, 0.8636363636363636465, 0.8659090909090909616, 0.8681818181818181657, 0.8704545454545454808, 0.8727272727272726849, 0.8750000000000000000, 0.8772727272727273151, 0.8795454545454545192, 0.8818181818181818343, 0.8840909090909090384, 0.8863636363636363535, 0.8886363636363636687, 0.8909090909090908728, 0.8931818181818181879, 0.8954545454545455030, 0.8977272727272727071, 0.9000000000000000222, 0.9022727272727272263, 0.9045454545454545414, 0.9068181818181818565, 0.9090909090909090606, 0.9113636363636363757, 0.9136363636363636909, 0.9159090909090908950, 0.9181818181818182101, 0.9204545454545454142, 0.9227272727272727293, 0.9250000000000000444, 0.9272727272727272485, 0.9295454545454545636, 0.9318181818181817677, 0.9340909090909090828, 0.9363636363636363980, 0.9386363636363636020, 0.9409090909090909172, 0.9431818181818182323, 0.9454545454545454364, 0.9477272727272727515, 0.9499999999999999556, 0.9522727272727272707, 0.9545454545454545858, 0.9568181818181817899, 0.9590909090909091050, 0.9613636363636363091, 0.9636363636363636243, 0.9659090909090909394, 0.9681818181818181435, 0.9704545454545454586, 0.9727272727272727737, 0.9749999999999999778, 0.9772727272727272929, 0.9781254700864303597 ),
 .UNSPECIFIED. ) 
 GEOMETRIC_REPRESENTATION_ITEM ( )  RATIONAL_B_SPLINE_SURFACE ( (
 ( 1.000000000000000000, 0.9898214418809326842, 1.000000000000000000, 0.9898214418809326842, 1.000000000000000000, 0.9898214418809326842, 1.000000000000000000, 0.9898214418809326842, 1.000000000000000000, 0.9898214418809326842, 1.000000000000000000, 0.9898214418809326842, 1.000000000000000000, 0.9898214418809326842, 1.000000000000000000, 0.9898214418809326842, 1.000000000000000000, 0.9898214418809326842, 1.000000000000000000, 0.9898214418809326842, 1.000000000000000000, 0.9898214418809326842, 1.000000000000000000, 0.9898214418809326842, 1.000000000000000000, 0.9898214418809326842, 1.000000000000000000, 0.9898214418809326842, 1.000000000000000000, 0.9898214418809326842, 1.000000000000000000, 0.9898214418809326842, 1.000000000000000000, 0.9898214418809326842, 1.000000000000000000, 0.9898214418809326842, 1.000000000000000000, 0.9898214418809326842, 1.000000000000000000, 0.9898214418809326842, 1.000000000000000000, 0.9898214418809326842, 1.000000000000000000, 0.9898214418809326842, 1.000000000000000000, 0.9898214418809326842, 1.000000000000000000, 0.9898214418809326842, 1.000000000000000000, 0.9898214418809326842, 1.000000000000000000, 0.9898214418809326842, 1.000000000000000000, 0.9898214418809326842, 1.000000000000000000, 0.9898214418809326842, 1.000000000000000000, 0.9898214418809326842, 1.000000000000000000, 0.9898214418809326842, 1.000000000000000000, 0.9898214418809326842, 1.000000000000000000, 0.9898214418809326842, 1.000000000000000000, 0.9898214418809326842, 1.000000000000000000, 0.9898214418809326842, 1.000000000000000000, 0.9898214418809326842, 1.000000000000000000, 0.9898214418809326842, 1.000000000000000000, 0.9898214418809326842, 1.000000000000000000, 0.9898214418809326842, 1.000000000000000000, 0.9898214418809326842, 1.000000000000000000, 0.9898214418809326842, 1.000000000000000000, 0.9898214418809326842, 1.000000000000000000, 0.9898214418809326842, 1.000000000000000000, 0.9898214418809326842, 1.000000000000000000, 0.9898214418809326842, 1.000000000000000000, 0.9898214418809326842, 1.000000000000000000, 0.9898214418809326842, 1.000000000000000000, 0.9898214418809326842, 1.000000000000000000, 0.9898214418809326842, 1.000000000000000000, 0.9898214418809326842, 1.000000000000000000, 0.9898214418809326842, 1.000000000000000000, 0.9898214418809326842, 1.000000000000000000, 0.9898214418809326842, 1.000000000000000000, 0.9898214418809326842, 1.000000000000000000, 0.9898214418809326842, 1.000000000000000000, 0.9898214418809326842, 1.000000000000000000, 0.9898214418809326842, 1.000000000000000000, 0.9898214418809326842, 1.000000000000000000, 0.9898214418809326842, 1.000000000000000000, 0.9898214418809326842, 1.000000000000000000, 0.9898214418809326842, 1.000000000000000000, 0.9898214418809326842, 1.000000000000000000, 0.9898214418809326842, 1.000000000000000000, 0.9898214418809326842, 1.000000000000000000, 0.9898214418809326842, 1.000000000000000000, 0.9898214418809326842, 1.000000000000000000, 0.9898214418809326842, 1.000000000000000000, 0.9898214418809326842, 1.000000000000000000, 0.9898214418809326842, 1.000000000000000000, 0.9898214418809326842, 1.000000000000000000, 0.9898214418809326842, 1.000000000000000000, 0.9898214418809326842, 1.000000000000000000, 0.9898214418809326842, 1.000000000000000000, 0.9898214418809326842, 1.000000000000000000, 0.9898214418809326842, 1.000000000000000000, 0.9898214418809326842, 1.000000000000000000, 0.9898214418809326842, 1.000000000000000000, 0.9898214418809326842, 1.000000000000000000, 0.9898214418809326842, 1.000000000000000000, 0.9898214418809326842, 1.000000000000000000, 0.9898214418809326842, 1.000000000000000000, 0.9898214418809326842, 1.000000000000000000, 0.9898214418809326842, 1.000000000000000000, 0.9898214418809326842, 1.000000000000000000, 0.9898214418809326842, 1.000000000000000000, 0.9898214418809326842, 1.000000000000000000, 0.9898214418809326842, 1.000000000000000000, 0.9898214418809326842, 1.000000000000000000, 0.9898214418809326842, 1.000000000000000000, 0.9898214418809326842, 1.000000000000000000, 0.9898214418809326842, 1.000000000000000000, 0.9898214418809326842, 1.000000000000000000, 0.9898214418809326842, 1.000000000000000000, 0.9898214418809326842, 1.000000000000000000, 0.9898214418809326842, 1.000000000000000000, 0.9898214418809326842, 1.000000000000000000, 0.9898214418809326842, 1.000000000000000000, 0.9898214418809326842, 1.000000000000000000, 0.9898214418809326842, 1.000000000000000000, 0.9898214418809326842, 1.000000000000000000, 0.9898214418809326842, 1.000000000000000000, 0.9898214418809326842, 1.000000000000000000, 0.9898214418809326842, 1.000000000000000000, 0.9898214418809326842, 1.000000000000000000, 0.9898214418809326842, 1.000000000000000000, 0.9898214418809326842, 1.000000000000000000, 0.9898214418809326842, 1.000000000000000000, 0.9898214418809326842, 1.000000000000000000, 0.9898214418809326842, 1.000000000000000000, 0.9898214418809326842, 1.000000000000000000, 0.9898214418809326842, 1.000000000000000000, 0.9898214418809326842, 1.000000000000000000, 0.9898214418809326842, 1.000000000000000000, 0.9898214418809326842, 1.000000000000000000, 0.9898214418809326842, 1.000000000000000000, 0.9898214418809326842, 1.000000000000000000, 0.9898214418809326842, 1.000000000000000000, 0.9898214418809326842, 1.000000000000000000, 0.9898214418809326842, 1.000000000000000000, 0.9898214418809326842, 1.000000000000000000, 0.9898214418809326842, 1.000000000000000000, 0.9898214418809326842, 1.000000000000000000, 0.9898214418809326842, 1.000000000000000000, 0.9898214418809326842, 1.000000000000000000, 0.9898214418809326842, 1.000000000000000000, 0.9898214418809326842, 1.000000000000000000, 0.9898214418809326842, 1.000000000000000000, 0.9898214418809326842, 1.000000000000000000, 0.9898214418809326842, 1.000000000000000000, 0.9898214418809326842, 1.000000000000000000, 0.9898214418809326842, 1.000000000000000000, 0.9898214418809326842, 1.000000000000000000, 0.9898214418809326842, 1.000000000000000000, 0.9898214418809326842, 1.000000000000000000, 0.9898214418809326842, 1.000000000000000000, 0.9898214418809326842, 1.000000000000000000, 0.9898214418809326842, 1.000000000000000000, 0.9898214418809326842, 1.000000000000000000, 0.9898214418809326842, 1.000000000000000000, 0.9898214418809326842, 1.000000000000000000, 0.9898214418809326842, 1.000000000000000000, 0.9898214418809326842, 1.000000000000000000, 0.9898214418809326842, 1.000000000000000000, 0.9898214418809326842, 1.000000000000000000, 0.9898214418809326842, 1.000000000000000000, 0.9898214418809326842, 1.000000000000000000, 0.9898214418809326842, 1.000000000000000000, 0.9898214418809326842, 1.000000000000000000, 0.9898214418809326842, 1.000000000000000000, 0.9898214418809326842, 1.000000000000000000, 0.9898214418809326842, 1.000000000000000000, 0.9898214418809326842, 1.000000000000000000, 0.9898214418809326842, 1.000000000000000000, 0.9898214418809326842, 1.000000000000000000, 0.9898214418809326842, 1.000000000000000000, 0.9898214418809326842, 1.000000000000000000, 0.9898214418809326842, 1.000000000000000000, 0.9898214418809326842, 1.000000000000000000, 0.9898214418809326842, 1.000000000000000000, 0.9898214418809326842, 1.000000000000000000, 0.9898214418809326842, 1.000000000000000000, 0.9898214418809326842, 1.000000000000000000, 0.9898214418809326842, 1.000000000000000000, 0.9898214418809326842, 1.000000000000000000, 0.9898214418809326842, 1.000000000000000000, 0.9898214418809326842, 1.000000000000000000, 0.9898214418809326842, 1.000000000000000000, 0.9898214418809326842, 1.000000000000000000, 0.9898214418809326842, 1.000000000000000000, 0.9898214418809326842, 1.000000000000000000, 0.9898214418809326842, 1.000000000000000000, 0.9898214418809326842, 1.000000000000000000, 0.9898214418809326842, 1.000000000000000000, 0.9898214418809326842, 1.000000000000000000, 0.9898214418809326842, 1.000000000000000000, 0.9898214418809326842, 1.000000000000000000, 0.9898214418809326842, 1.000000000000000000, 0.9898214418809326842, 1.000000000000000000, 0.9898214418809326842, 1.000000000000000000, 0.9898214418809326842, 1.000000000000000000, 0.9898214418809326842, 1.000000000000000000, 0.9898214418809326842, 1.000000000000000000, 0.9898214418809326842, 1.000000000000000000, 0.9898214418809326842, 1.000000000000000000, 0.9898214418809326842, 1.000000000000000000, 0.9898214418809326842, 1.000000000000000000, 0.9898214418809326842, 1.000000000000000000, 0.9898214418809326842, 1.000000000000000000, 0.9898214418809326842, 1.000000000000000000, 0.9898214418809326842, 1.000000000000000000, 0.9898214418809326842, 1.000000000000000000, 0.9898214418809326842, 1.000000000000000000, 0.9898214418809326842, 1.000000000000000000, 0.9898214418809326842, 1.000000000000000000, 0.9898214418809326842, 1.000000000000000000, 0.9898214418809326842, 1.000000000000000000, 0.9898214418809326842, 1.000000000000000000, 0.9898214418809326842, 1.000000000000000000, 0.9898214418809326842, 1.000000000000000000, 0.9898214418809326842, 1.000000000000000000, 0.9898214418809326842, 1.000000000000000000, 0.9898214418809326842, 1.000000000000000000, 0.9898214418809326842, 1.000000000000000000, 0.9898214418809326842, 1.000000000000000000, 0.9898214418809326842, 1.000000000000000000, 0.9898214418809326842, 1.000000000000000000, 0.9898214418809326842, 1.000000000000000000, 0.9898214418809326842, 1.000000000000000000, 0.9898214418809326842, 1.000000000000000000, 0.9898214418809326842, 1.000000000000000000, 0.9898214418809326842, 1.000000000000000000, 0.9898214418809326842, 1.000000000000000000, 0.9898214418809326842, 1.000000000000000000, 0.9898214418809326842, 1.000000000000000000, 0.9898214418809326842, 1.000000000000000000, 0.9898214418809326842, 1.000000000000000000, 0.9898214418809326842, 1.000000000000000000, 0.9898214418809326842, 1.000000000000000000, 0.9898214418809326842, 1.000000000000000000, 0.9898214418809326842, 1.000000000000000000, 0.9898214418809326842, 1.000000000000000000, 0.9898214418809326842, 1.000000000000000000, 0.9898214418809326842, 1.000000000000000000, 0.9898214418809326842, 1.000000000000000000, 0.9898214418809326842, 1.000000000000000000, 0.9898214418809326842, 1.000000000000000000, 0.9898214418809326842, 1.000000000000000000, 0.9898214418809326842, 1.000000000000000000, 0.9898214418809326842, 1.000000000000000000, 0.9898214418809326842, 1.000000000000000000, 0.9898214418809326842, 1.000000000000000000, 0.9898214418809326842, 1.000000000000000000, 0.9898214418809326842, 1.000000000000000000, 0.9898214418809326842, 1.000000000000000000, 0.9898214418809326842, 1.000000000000000000, 0.9898214418809326842, 1.000000000000000000, 0.9898214418809326842, 1.000000000000000000, 0.9898214418809326842, 1.000000000000000000, 0.9898214418809326842, 1.000000000000000000, 0.9898214418809326842, 1.000000000000000000, 0.9898214418809326842, 1.000000000000000000, 0.9898214418809326842, 1.000000000000000000, 0.9898214418809326842, 1.000000000000000000, 0.9898214418809326842, 1.000000000000000000, 0.9898214418809326842, 1.000000000000000000, 0.9898214418809326842, 1.000000000000000000, 0.9898214418809326842, 1.000000000000000000, 0.9898214418809326842, 1.000000000000000000, 0.9898214418809326842, 1.000000000000000000, 0.9898214418809326842, 1.000000000000000000, 0.9898214418809326842, 1.000000000000000000, 0.9898214418809326842, 1.000000000000000000, 0.9898214418809326842, 1.000000000000000000, 0.9898214418809326842, 1.000000000000000000, 0.9898214418809326842, 1.000000000000000000, 0.9898214418809326842, 1.000000000000000000, 0.9898214418809326842, 1.000000000000000000, 0.9898214418809326842, 1.000000000000000000, 0.9898214418809326842, 1.000000000000000000, 0.9898214418809326842, 1.000000000000000000, 0.9898214418809326842, 1.000000000000000000, 0.9898214418809326842, 1.000000000000000000, 0.9898214418809326842, 1.000000000000000000, 0.9898214418809326842, 1.000000000000000000, 0.9898214418809326842, 1.000000000000000000, 0.9898214418809326842, 1.000000000000000000, 0.9898214418809326842, 1.000000000000000000, 0.9898214418809326842, 1.000000000000000000, 0.9898214418809326842, 1.000000000000000000, 0.9898214418809326842, 1.000000000000000000, 0.9898214418809326842, 1.000000000000000000, 0.9898214418809326842, 1.000000000000000000, 0.9898214418809326842, 1.000000000000000000, 0.9898214418809326842, 1.000000000000000000, 0.9898214418809326842, 1.000000000000000000, 0.9898214418809326842, 1.000000000000000000, 0.9898214418809326842, 1.000000000000000000, 0.9898214418809326842, 1.000000000000000000, 0.9898214418809326842, 1.000000000000000000, 0.9898214418809326842, 1.000000000000000000, 0.9898214418809326842, 1.000000000000000000, 0.9898214418809326842, 1.000000000000000000, 0.9898214418809326842, 1.000000000000000000, 0.9898214418809326842, 1.000000000000000000, 0.9898214418809326842, 1.000000000000000000, 0.9898214418809326842, 1.000000000000000000, 0.9898214418809326842, 1.000000000000000000, 0.9898214418809326842, 1.000000000000000000, 0.9898214418809326842, 1.000000000000000000, 0.9898214418809326842, 1.000000000000000000, 0.9898214418809326842, 1.000000000000000000, 0.9898214418809326842, 1.000000000000000000, 0.9898214418809326842, 1.000000000000000000, 0.9898214418809326842, 1.000000000000000000, 0.9898214418809326842, 1.000000000000000000, 0.9898214418809326842, 1.000000000000000000, 0.9898214418809326842, 1.000000000000000000, 0.9898214418809326842, 1.000000000000000000, 0.9898214418809326842, 1.000000000000000000, 0.9898214418809326842, 1.000000000000000000, 0.9898214418809326842, 1.000000000000000000, 0.9898214418809326842, 1.000000000000000000, 0.9898214418809326842, 1.000000000000000000, 0.9898214418809326842, 1.000000000000000000, 0.9898214418809326842, 1.000000000000000000, 0.9898214418809326842, 1.000000000000000000, 0.9898214418809326842, 1.000000000000000000, 0.9898214418809326842, 1.000000000000000000, 0.9898214418809326842, 1.000000000000000000, 0.9898214418809326842, 1.000000000000000000, 0.9898214418809326842, 1.000000000000000000, 0.9898214418809326842, 1.000000000000000000, 0.9898214418809326842, 1.000000000000000000, 0.9898214418809326842, 1.000000000000000000, 0.9898214418809326842, 1.000000000000000000, 0.9898214418809326842, 1.000000000000000000, 0.9898214418809326842, 1.000000000000000000, 0.9898214418809326842, 1.000000000000000000, 0.9898214418809326842, 1.000000000000000000, 0.9898214418809326842, 1.000000000000000000, 0.9898214418809326842, 1.000000000000000000, 0.9898214418809326842, 1.000000000000000000, 0.9898214418809326842, 1.000000000000000000, 0.9898214418809326842, 1.000000000000000000, 0.9898214418809326842, 1.000000000000000000, 0.9898214418809326842, 1.000000000000000000, 0.9898214418809326842, 1.000000000000000000, 0.9898214418809326842, 1.000000000000000000, 0.9898214418809326842, 1.000000000000000000, 0.9898214418809326842, 1.000000000000000000, 0.9898214418809326842, 1.000000000000000000, 0.9898214418809326842, 1.000000000000000000, 0.9898214418809326842, 1.000000000000000000, 0.9898214418809326842, 1.000000000000000000, 0.9898214418809326842, 1.000000000000000000, 0.9898214418809326842, 1.000000000000000000, 0.9898214418809326842, 1.000000000000000000, 0.9898214418809326842, 1.000000000000000000, 0.9898214418809326842, 1.000000000000000000, 0.9898214418809326842, 1.000000000000000000, 0.9898214418809326842, 1.000000000000000000, 0.9898214418809326842, 1.000000000000000000, 0.9898214418809326842, 1.000000000000000000, 0.9898214418809326842, 1.000000000000000000, 0.9898214418809326842, 1.000000000000000000, 0.9898214418809326842, 1.000000000000000000, 0.9898214418809326842, 1.000000000000000000, 0.9898214418809326842, 1.000000000000000000, 0.9898214418809326842, 1.000000000000000000, 0.9898214418809326842, 1.000000000000000000, 0.9898214418809326842, 1.000000000000000000, 0.9898214418809326842, 1.000000000000000000, 0.9898214418809326842, 1.000000000000000000, 0.9898214418809326842, 1.000000000000000000, 0.9898214418809326842, 1.000000000000000000, 0.9898214418809326842, 1.000000000000000000, 0.9898214418809326842, 1.000000000000000000, 0.9898214418809326842, 1.000000000000000000, 0.9898214418809326842, 1.000000000000000000, 0.9898214418809326842, 1.000000000000000000, 0.9898214418809326842, 1.000000000000000000, 0.9898214418809326842, 1.000000000000000000, 0.9898214418809326842, 1.000000000000000000, 0.9898214418809326842, 1.000000000000000000, 0.9898214418809326842, 1.000000000000000000, 0.9898214418809326842, 1.000000000000000000, 0.9898214418809326842, 1.000000000000000000, 0.9898214418809326842, 1.000000000000000000, 0.9898214418809326842, 1.000000000000000000, 0.9898214418809326842, 1.000000000000000000, 0.9898214418809326842, 1.000000000000000000, 0.9898214418809326842, 1.000000000000000000, 0.9898214418809326842, 1.000000000000000000, 0.9898214418809326842, 1.000000000000000000, 0.9898214418809326842, 1.000000000000000000, 0.9898214418809326842, 1.000000000000000000, 0.9898214418809326842, 1.000000000000000000, 0.9898214418809326842, 1.000000000000000000, 0.9898214418809326842, 1.000000000000000000, 0.9898214418809326842, 1.000000000000000000, 0.9898214418809326842, 1.000000000000000000, 0.9898214418809326842, 1.000000000000000000, 0.9898214418809326842, 1.000000000000000000, 0.9898214418809326842, 1.000000000000000000, 0.9898214418809326842, 1.000000000000000000, 0.9898214418809326842, 1.000000000000000000, 0.9898214418809326842, 1.000000000000000000, 0.9898214418809326842, 1.000000000000000000, 0.9898214418809326842, 1.000000000000000000, 0.9898214418809326842, 1.000000000000000000, 0.9898214418809326842, 1.000000000000000000, 0.9898214418809326842, 1.000000000000000000, 0.9898214418809326842, 1.000000000000000000, 0.9898214418809326842, 1.000000000000000000, 0.9898214418809326842, 1.000000000000000000, 0.9898214418809326842, 1.000000000000000000, 0.9898214418809326842, 1.000000000000000000, 0.9898214418809326842, 1.000000000000000000, 0.9898214418809326842, 1.000000000000000000, 0.9898214418809326842, 1.000000000000000000, 0.9898214418809326842, 1.000000000000000000, 0.9898214418809326842, 1.000000000000000000, 0.9898214418809326842, 1.000000000000000000, 0.9898214418809326842, 1.000000000000000000, 0.9898214418809326842, 1.000000000000000000, 0.9898214418809326842, 1.000000000000000000, 0.9898214418809326842, 1.000000000000000000, 0.9898214418809326842, 1.000000000000000000, 0.9898214418809326842, 1.000000000000000000, 0.9898214418809326842, 1.000000000000000000, 0.9898214418809326842, 1.000000000000000000, 0.9898214418809326842, 1.000000000000000000, 0.9898214418809326842, 1.000000000000000000, 0.9898214418809326842, 1.000000000000000000, 0.9898214418809326842, 1.000000000000000000, 0.9898214418809326842, 1.000000000000000000, 0.9898214418809326842, 1.000000000000000000, 0.9898214418809326842, 1.000000000000000000, 0.9898214418809326842, 1.000000000000000000, 0.9898214418809326842, 1.000000000000000000, 0.9898214418809326842, 1.000000000000000000, 0.9898214418809326842, 1.000000000000000000, 0.9898214418809326842, 1.000000000000000000, 0.9898214418809326842, 1.000000000000000000, 0.9898214418809326842, 1.000000000000000000, 0.9898214418809326842, 1.000000000000000000, 0.9898214418809326842, 1.000000000000000000, 0.9898214418809326842, 1.000000000000000000, 0.9898214418809326842, 1.000000000000000000, 0.9898214418809326842, 1.000000000000000000, 0.9898214418809326842, 1.000000000000000000, 0.9961809353924466759, 0.9952277490961531914),
 ( 0.3333333333333333703, 0.3299404806269776169, 0.3333333333333333703, 0.3299404806269776169, 0.3333333333333333703, 0.3299404806269776169, 0.3333333333333333703, 0.3299404806269776169, 0.3333333333333333703, 0.3299404806269776169, 0.3333333333333333703, 0.3299404806269776169, 0.3333333333333333703, 0.3299404806269776169, 0.3333333333333333703, 0.3299404806269776169, 0.3333333333333333703, 0.3299404806269776169, 0.3333333333333333703, 0.3299404806269776169, 0.3333333333333333703, 0.3299404806269776169, 0.3333333333333333703, 0.3299404806269776169, 0.3333333333333333703, 0.3299404806269776169, 0.3333333333333333703, 0.3299404806269776169, 0.3333333333333333703, 0.3299404806269776169, 0.3333333333333333703, 0.3299404806269776169, 0.3333333333333333703, 0.3299404806269776169, 0.3333333333333333703, 0.3299404806269776169, 0.3333333333333333703, 0.3299404806269776169, 0.3333333333333333703, 0.3299404806269776169, 0.3333333333333333703, 0.3299404806269776169, 0.3333333333333333703, 0.3299404806269776169, 0.3333333333333333703, 0.3299404806269776169, 0.3333333333333333703, 0.3299404806269776169, 0.3333333333333333703, 0.3299404806269776169, 0.3333333333333333703, 0.3299404806269776169, 0.3333333333333333703, 0.3299404806269776169, 0.3333333333333333703, 0.3299404806269776169, 0.3333333333333333703, 0.3299404806269776169, 0.3333333333333333703, 0.3299404806269776169, 0.3333333333333333703, 0.3299404806269776169, 0.3333333333333333703, 0.3299404806269776169, 0.3333333333333333703, 0.3299404806269776169, 0.3333333333333333703, 0.3299404806269776169, 0.3333333333333333703, 0.3299404806269776169, 0.3333333333333333703, 0.3299404806269776169, 0.3333333333333333703, 0.3299404806269776169, 0.3333333333333333703, 0.3299404806269776169, 0.3333333333333333703, 0.3299404806269776169, 0.3333333333333333703, 0.3299404806269776169, 0.3333333333333333703, 0.3299404806269776169, 0.3333333333333333703, 0.3299404806269776169, 0.3333333333333333703, 0.3299404806269776169, 0.3333333333333333703, 0.3299404806269776169, 0.3333333333333333703, 0.3299404806269776169, 0.3333333333333333703, 0.3299404806269776169, 0.3333333333333333703, 0.3299404806269776169, 0.3333333333333333703, 0.3299404806269776169, 0.3333333333333333703, 0.3299404806269776169, 0.3333333333333333703, 0.3299404806269776169, 0.3333333333333333703, 0.3299404806269776169, 0.3333333333333333703, 0.3299404806269776169, 0.3333333333333333703, 0.3299404806269776169, 0.3333333333333333703, 0.3299404806269776169, 0.3333333333333333703, 0.3299404806269776169, 0.3333333333333333703, 0.3299404806269776169, 0.3333333333333333703, 0.3299404806269776169, 0.3333333333333333703, 0.3299404806269776169, 0.3333333333333333703, 0.3299404806269776169, 0.3333333333333333703, 0.3299404806269776169, 0.3333333333333333703, 0.3299404806269776169, 0.3333333333333333703, 0.3299404806269776169, 0.3333333333333333703, 0.3299404806269776169, 0.3333333333333333703, 0.3299404806269776169, 0.3333333333333333703, 0.3299404806269776169, 0.3333333333333333703, 0.3299404806269776169, 0.3333333333333333703, 0.3299404806269776169, 0.3333333333333333703, 0.3299404806269776169, 0.3333333333333333703, 0.3299404806269776169, 0.3333333333333333703, 0.3299404806269776169, 0.3333333333333333703, 0.3299404806269776169, 0.3333333333333333703, 0.3299404806269776169, 0.3333333333333333703, 0.3299404806269776169, 0.3333333333333333703, 0.3299404806269776169, 0.3333333333333333703, 0.3299404806269776169, 0.3333333333333333703, 0.3299404806269776169, 0.3333333333333333703, 0.3299404806269776169, 0.3333333333333333703, 0.3299404806269776169, 0.3333333333333333703, 0.3299404806269776169, 0.3333333333333333703, 0.3299404806269776169, 0.3333333333333333703, 0.3299404806269776169, 0.3333333333333333703, 0.3299404806269776169, 0.3333333333333333703, 0.3299404806269776169, 0.3333333333333333703, 0.3299404806269776169, 0.3333333333333333703, 0.3299404806269776169, 0.3333333333333333703, 0.3299404806269776169, 0.3333333333333333703, 0.3299404806269776169, 0.3333333333333333703, 0.3299404806269776169, 0.3333333333333333703, 0.3299404806269776169, 0.3333333333333333703, 0.3299404806269776169, 0.3333333333333333703, 0.3299404806269776169, 0.3333333333333333703, 0.3299404806269776169, 0.3333333333333333703, 0.3299404806269776169, 0.3333333333333333703, 0.3299404806269776169, 0.3333333333333333703, 0.3299404806269776169, 0.3333333333333333703, 0.3299404806269776169, 0.3333333333333333703, 0.3299404806269776169, 0.3333333333333333703, 0.3299404806269776169, 0.3333333333333333703, 0.3299404806269776169, 0.3333333333333333703, 0.3299404806269776169, 0.3333333333333333703, 0.3299404806269776169, 0.3333333333333333703, 0.3299404806269776169, 0.3333333333333333703, 0.3299404806269776169, 0.3333333333333333703, 0.3299404806269776169, 0.3333333333333333703, 0.3299404806269776169, 0.3333333333333333703, 0.3299404806269776169, 0.3333333333333333703, 0.3299404806269776169, 0.3333333333333333703, 0.3299404806269776169, 0.3333333333333333703, 0.3299404806269776169, 0.3333333333333333703, 0.3299404806269776169, 0.3333333333333333703, 0.3299404806269776169, 0.3333333333333333703, 0.3299404806269776169, 0.3333333333333333703, 0.3299404806269776169, 0.3333333333333333703, 0.3299404806269776169, 0.3333333333333333703, 0.3299404806269776169, 0.3333333333333333703, 0.3299404806269776169, 0.3333333333333333703, 0.3299404806269776169, 0.3333333333333333703, 0.3299404806269776169, 0.3333333333333333703, 0.3299404806269776169, 0.3333333333333333703, 0.3299404806269776169, 0.3333333333333333703, 0.3299404806269776169, 0.3333333333333333703, 0.3299404806269776169, 0.3333333333333333703, 0.3299404806269776169, 0.3333333333333333703, 0.3299404806269776169, 0.3333333333333333703, 0.3299404806269776169, 0.3333333333333333703, 0.3299404806269776169, 0.3333333333333333703, 0.3299404806269776169, 0.3333333333333333703, 0.3299404806269776169, 0.3333333333333333703, 0.3299404806269776169, 0.3333333333333333703, 0.3299404806269776169, 0.3333333333333333703, 0.3299404806269776169, 0.3333333333333333703, 0.3299404806269776169, 0.3333333333333333703, 0.3299404806269776169, 0.3333333333333333703, 0.3299404806269776169, 0.3333333333333333703, 0.3299404806269776169, 0.3333333333333333703, 0.3299404806269776169, 0.3333333333333333703, 0.3299404806269776169, 0.3333333333333333703, 0.3299404806269776169, 0.3333333333333333703, 0.3299404806269776169, 0.3333333333333333703, 0.3299404806269776169, 0.3333333333333333703, 0.3299404806269776169, 0.3333333333333333703, 0.3299404806269776169, 0.3333333333333333703, 0.3299404806269776169, 0.3333333333333333703, 0.3299404806269776169, 0.3333333333333333703, 0.3299404806269776169, 0.3333333333333333703, 0.3299404806269776169, 0.3333333333333333703, 0.3299404806269776169, 0.3333333333333333703, 0.3299404806269776169, 0.3333333333333333703, 0.3299404806269776169, 0.3333333333333333703, 0.3299404806269776169, 0.3333333333333333703, 0.3299404806269776169, 0.3333333333333333703, 0.3299404806269776169, 0.3333333333333333703, 0.3299404806269776169, 0.3333333333333333703, 0.3299404806269776169, 0.3333333333333333703, 0.3299404806269776169, 0.3333333333333333703, 0.3299404806269776169, 0.3333333333333333703, 0.3299404806269776169, 0.3333333333333333703, 0.3299404806269776169, 0.3333333333333333703, 0.3299404806269776169, 0.3333333333333333703, 0.3299404806269776169, 0.3333333333333333703, 0.3299404806269776169, 0.3333333333333333703, 0.3299404806269776169, 0.3333333333333333703, 0.3299404806269776169, 0.3333333333333333703, 0.3299404806269776169, 0.3333333333333333703, 0.3299404806269776169, 0.3333333333333333703, 0.3299404806269776169, 0.3333333333333333703, 0.3299404806269776169, 0.3333333333333333703, 0.3299404806269776169, 0.3333333333333333703, 0.3299404806269776169, 0.3333333333333333703, 0.3299404806269776169, 0.3333333333333333703, 0.3299404806269776169, 0.3333333333333333703, 0.3299404806269776169, 0.3333333333333333703, 0.3299404806269776169, 0.3333333333333333703, 0.3299404806269776169, 0.3333333333333333703, 0.3299404806269776169, 0.3333333333333333703, 0.3299404806269776169, 0.3333333333333333703, 0.3299404806269776169, 0.3333333333333333703, 0.3299404806269776169, 0.3333333333333333703, 0.3299404806269776169, 0.3333333333333333703, 0.3299404806269776169, 0.3333333333333333703, 0.3299404806269776169, 0.3333333333333333703, 0.3299404806269776169, 0.3333333333333333703, 0.3299404806269776169, 0.3333333333333333703, 0.3299404806269776169, 0.3333333333333333703, 0.3299404806269776169, 0.3333333333333333703, 0.3299404806269776169, 0.3333333333333333703, 0.3299404806269776169, 0.3333333333333333703, 0.3299404806269776169, 0.3333333333333333703, 0.3299404806269776169, 0.3333333333333333703, 0.3299404806269776169, 0.3333333333333333703, 0.3299404806269776169, 0.3333333333333333703, 0.3299404806269776169, 0.3333333333333333703, 0.3299404806269776169, 0.3333333333333333703, 0.3299404806269776169, 0.3333333333333333703, 0.3299404806269776169, 0.3333333333333333703, 0.3299404806269776169, 0.3333333333333333703, 0.3299404806269776169, 0.3333333333333333703, 0.3299404806269776169, 0.3333333333333333703, 0.3299404806269776169, 0.3333333333333333703, 0.3299404806269776169, 0.3333333333333333703, 0.3299404806269776169, 0.3333333333333333703, 0.3299404806269776169, 0.3333333333333333703, 0.3299404806269776169, 0.3333333333333333703, 0.3299404806269776169, 0.3333333333333333703, 0.3299404806269776169, 0.3333333333333333703, 0.3299404806269776169, 0.3333333333333333703, 0.3299404806269776169, 0.3333333333333333703, 0.3299404806269776169, 0.3333333333333333703, 0.3299404806269776169, 0.3333333333333333703, 0.3299404806269776169, 0.3333333333333333703, 0.3299404806269776169, 0.3333333333333333703, 0.3299404806269776169, 0.3333333333333333703, 0.3299404806269776169, 0.3333333333333333703, 0.3299404806269776169, 0.3333333333333333703, 0.3299404806269776169, 0.3333333333333333703, 0.3299404806269776169, 0.3333333333333333703, 0.3299404806269776169, 0.3333333333333333703, 0.3299404806269776169, 0.3333333333333333703, 0.3299404806269776169, 0.3333333333333333703, 0.3299404806269776169, 0.3333333333333333703, 0.3299404806269776169, 0.3333333333333333703, 0.3299404806269776169, 0.3333333333333333703, 0.3299404806269776169, 0.3333333333333333703, 0.3299404806269776169, 0.3333333333333333703, 0.3299404806269776169, 0.3333333333333333703, 0.3299404806269776169, 0.3333333333333333703, 0.3299404806269776169, 0.3333333333333333703, 0.3299404806269776169, 0.3333333333333333703, 0.3299404806269776169, 0.3333333333333333703, 0.3299404806269776169, 0.3333333333333333703, 0.3299404806269776169, 0.3333333333333333703, 0.3299404806269776169, 0.3333333333333333703, 0.3299404806269776169, 0.3333333333333333703, 0.3299404806269776169, 0.3333333333333333703, 0.3299404806269776169, 0.3333333333333333703, 0.3299404806269776169, 0.3333333333333333703, 0.3299404806269776169, 0.3333333333333333703, 0.3299404806269776169, 0.3333333333333333703, 0.3299404806269776169, 0.3333333333333333703, 0.3299404806269776169, 0.3333333333333333703, 0.3299404806269776169, 0.3333333333333333703, 0.3299404806269776169, 0.3333333333333333703, 0.3299404806269776169, 0.3333333333333333703, 0.3299404806269776169, 0.3333333333333333703, 0.3299404806269776169, 0.3333333333333333703, 0.3299404806269776169, 0.3333333333333333703, 0.3299404806269776169, 0.3333333333333333703, 0.3299404806269776169, 0.3333333333333333703, 0.3299404806269776169, 0.3333333333333333703, 0.3299404806269776169, 0.3333333333333333703, 0.3299404806269776169, 0.3333333333333333703, 0.3299404806269776169, 0.3333333333333333703, 0.3299404806269776169, 0.3333333333333333703, 0.3299404806269776169, 0.3333333333333333703, 0.3299404806269776169, 0.3333333333333333703, 0.3299404806269776169, 0.3333333333333333703, 0.3299404806269776169, 0.3333333333333333703, 0.3299404806269776169, 0.3333333333333333703, 0.3299404806269776169, 0.3333333333333333703, 0.3299404806269776169, 0.3333333333333333703, 0.3299404806269776169, 0.3333333333333333703, 0.3299404806269776169, 0.3333333333333333703, 0.3299404806269776169, 0.3333333333333333703, 0.3299404806269776169, 0.3333333333333333703, 0.3299404806269776169, 0.3333333333333333703, 0.3299404806269776169, 0.3333333333333333703, 0.3299404806269776169, 0.3333333333333333703, 0.3299404806269776169, 0.3333333333333333703, 0.3299404806269776169, 0.3333333333333333703, 0.3299404806269776169, 0.3333333333333333703, 0.3299404806269776169, 0.3333333333333333703, 0.3299404806269776169, 0.3333333333333333703, 0.3299404806269776169, 0.3333333333333333703, 0.3299404806269776169, 0.3333333333333333703, 0.3299404806269776169, 0.3333333333333333703, 0.3299404806269776169, 0.3333333333333333703, 0.3299404806269776169, 0.3333333333333333703, 0.3299404806269776169, 0.3333333333333333703, 0.3299404806269776169, 0.3333333333333333703, 0.3299404806269776169, 0.3333333333333333703, 0.3299404806269776169, 0.3333333333333333703, 0.3299404806269776169, 0.3333333333333333703, 0.3299404806269776169, 0.3333333333333333703, 0.3299404806269776169, 0.3333333333333333703, 0.3299404806269776169, 0.3333333333333333703, 0.3299404806269776169, 0.3333333333333333703, 0.3299404806269776169, 0.3333333333333333703, 0.3299404806269776169, 0.3333333333333333703, 0.3299404806269776169, 0.3333333333333333703, 0.3299404806269776169, 0.3333333333333333703, 0.3299404806269776169, 0.3333333333333333703, 0.3299404806269776169, 0.3333333333333333703, 0.3299404806269776169, 0.3333333333333333703, 0.3299404806269776169, 0.3333333333333333703, 0.3299404806269776169, 0.3333333333333333703, 0.3299404806269776169, 0.3333333333333333703, 0.3299404806269776169, 0.3333333333333333703, 0.3299404806269776169, 0.3333333333333333703, 0.3299404806269776169, 0.3333333333333333703, 0.3299404806269776169, 0.3333333333333333703, 0.3299404806269776169, 0.3333333333333333703, 0.3299404806269776169, 0.3333333333333333703, 0.3299404806269776169, 0.3333333333333333703, 0.3299404806269776169, 0.3333333333333333703, 0.3299404806269776169, 0.3333333333333333703, 0.3299404806269776169, 0.3333333333333333703, 0.3299404806269776169, 0.3333333333333333703, 0.3299404806269776169, 0.3333333333333333703, 0.3299404806269776169, 0.3333333333333333703, 0.3299404806269776169, 0.3333333333333333703, 0.3299404806269776169, 0.3333333333333333703, 0.3299404806269776169, 0.3333333333333333703, 0.3299404806269776169, 0.3333333333333333703, 0.3299404806269776169, 0.3333333333333333703, 0.3299404806269776169, 0.3333333333333333703, 0.3299404806269776169, 0.3333333333333333703, 0.3299404806269776169, 0.3333333333333333703, 0.3299404806269776169, 0.3333333333333333703, 0.3299404806269776169, 0.3333333333333333703, 0.3299404806269776169, 0.3333333333333333703, 0.3299404806269776169, 0.3333333333333333703, 0.3299404806269776169, 0.3333333333333333703, 0.3299404806269776169, 0.3333333333333333703, 0.3299404806269776169, 0.3333333333333333703, 0.3299404806269776169, 0.3333333333333333703, 0.3299404806269776169, 0.3333333333333333703, 0.3299404806269776169, 0.3333333333333333703, 0.3299404806269776169, 0.3333333333333333703, 0.3299404806269776169, 0.3333333333333333703, 0.3299404806269776169, 0.3333333333333333703, 0.3299404806269776169, 0.3333333333333333703, 0.3299404806269776169, 0.3333333333333333703, 0.3299404806269776169, 0.3333333333333333703, 0.3299404806269776169, 0.3333333333333333703, 0.3299404806269776169, 0.3333333333333333703, 0.3299404806269776169, 0.3333333333333333703, 0.3299404806269776169, 0.3333333333333333703, 0.3299404806269776169, 0.3333333333333333703, 0.3299404806269776169, 0.3333333333333333703, 0.3299404806269776169, 0.3333333333333333703, 0.3299404806269776169, 0.3333333333333333703, 0.3299404806269776169, 0.3333333333333333703, 0.3299404806269776169, 0.3333333333333333703, 0.3299404806269776169, 0.3333333333333333703, 0.3299404806269776169, 0.3333333333333333703, 0.3299404806269776169, 0.3333333333333333703, 0.3299404806269776169, 0.3333333333333333703, 0.3299404806269776169, 0.3333333333333333703, 0.3299404806269776169, 0.3333333333333333703, 0.3299404806269776169, 0.3333333333333333703, 0.3299404806269776169, 0.3333333333333333703, 0.3299404806269776169, 0.3333333333333333703, 0.3299404806269776169, 0.3333333333333333703, 0.3299404806269776169, 0.3333333333333333703, 0.3299404806269776169, 0.3333333333333333703, 0.3299404806269776169, 0.3333333333333333703, 0.3299404806269776169, 0.3333333333333333703, 0.3299404806269776169, 0.3333333333333333703, 0.3299404806269776169, 0.3333333333333333703, 0.3299404806269776169, 0.3333333333333333703, 0.3299404806269776169, 0.3333333333333333703, 0.3299404806269776169, 0.3333333333333333703, 0.3299404806269776169, 0.3333333333333333703, 0.3299404806269776169, 0.3333333333333333703, 0.3299404806269776169, 0.3333333333333333703, 0.3299404806269776169, 0.3333333333333333703, 0.3299404806269776169, 0.3333333333333333703, 0.3299404806269776169, 0.3333333333333333703, 0.3299404806269776169, 0.3333333333333333703, 0.3299404806269776169, 0.3333333333333333703, 0.3299404806269776169, 0.3333333333333333703, 0.3299404806269776169, 0.3333333333333333703, 0.3299404806269776169, 0.3333333333333333703, 0.3299404806269776169, 0.3333333333333333703, 0.3299404806269776169, 0.3333333333333333703, 0.3299404806269776169, 0.3333333333333333703, 0.3299404806269776169, 0.3333333333333333703, 0.3299404806269776169, 0.3333333333333333703, 0.3299404806269776169, 0.3333333333333333703, 0.3299404806269776169, 0.3333333333333333703, 0.3299404806269776169, 0.3333333333333333703, 0.3299404806269776169, 0.3333333333333333703, 0.3299404806269776169, 0.3333333333333333703, 0.3299404806269776169, 0.3333333333333333703, 0.3299404806269776169, 0.3333333333333333703, 0.3299404806269776169, 0.3333333333333333703, 0.3299404806269776169, 0.3333333333333333703, 0.3299404806269776169, 0.3333333333333333703, 0.3299404806269776169, 0.3333333333333333703, 0.3299404806269776169, 0.3333333333333333703, 0.3299404806269776169, 0.3333333333333333703, 0.3299404806269776169, 0.3333333333333333703, 0.3299404806269776169, 0.3333333333333333703, 0.3299404806269776169, 0.3333333333333333703, 0.3299404806269776169, 0.3333333333333333703, 0.3299404806269776169, 0.3333333333333333703, 0.3299404806269776169, 0.3333333333333333703, 0.3299404806269776169, 0.3333333333333333703, 0.3299404806269776169, 0.3333333333333333703, 0.3299404806269776169, 0.3333333333333333703, 0.3299404806269776169, 0.3333333333333333703, 0.3299404806269776169, 0.3333333333333333703, 0.3299404806269776169, 0.3333333333333333703, 0.3299404806269776169, 0.3333333333333333703, 0.3299404806269776169, 0.3333333333333333703, 0.3299404806269776169, 0.3333333333333333703, 0.3299404806269776169, 0.3333333333333333703, 0.3299404806269776169, 0.3333333333333333703, 0.3299404806269776169, 0.3333333333333333703, 0.3299404806269776169, 0.3333333333333333703, 0.3299404806269776169, 0.3333333333333333703, 0.3299404806269776169, 0.3333333333333333703, 0.3299404806269776169, 0.3333333333333333703, 0.3299404806269776169, 0.3333333333333333703, 0.3299404806269776169, 0.3333333333333333703, 0.3299404806269776169, 0.3333333333333333703, 0.3299404806269776169, 0.3333333333333333703, 0.3299404806269776169, 0.3333333333333333703, 0.3299404806269776169, 0.3333333333333333703, 0.3299404806269776169, 0.3333333333333333703, 0.3299404806269776169, 0.3333333333333333703, 0.3299404806269776169, 0.3333333333333333703, 0.3299404806269776169, 0.3333333333333333703, 0.3299404806269776169, 0.3333333333333333703, 0.3299404806269776169, 0.3333333333333333703, 0.3299404806269776169, 0.3333333333333333703, 0.3299404806269776169, 0.3333333333333333703, 0.3299404806269776169, 0.3333333333333333703, 0.3299404806269776169, 0.3333333333333333703, 0.3299404806269776169, 0.3333333333333333703, 0.3320603117974822438, 0.3317425830320511193),
 ( 0.3333333333333333703, 0.3299404806269776169, 0.3333333333333333703, 0.3299404806269776169, 0.3333333333333333703, 0.3299404806269776169, 0.3333333333333333703, 0.3299404806269776169, 0.3333333333333333703, 0.3299404806269776169, 0.3333333333333333703, 0.3299404806269776169, 0.3333333333333333703, 0.3299404806269776169, 0.3333333333333333703, 0.3299404806269776169, 0.3333333333333333703, 0.3299404806269776169, 0.3333333333333333703, 0.3299404806269776169, 0.3333333333333333703, 0.3299404806269776169, 0.3333333333333333703, 0.3299404806269776169, 0.3333333333333333703, 0.3299404806269776169, 0.3333333333333333703, 0.3299404806269776169, 0.3333333333333333703, 0.3299404806269776169, 0.3333333333333333703, 0.3299404806269776169, 0.3333333333333333703, 0.3299404806269776169, 0.3333333333333333703, 0.3299404806269776169, 0.3333333333333333703, 0.3299404806269776169, 0.3333333333333333703, 0.3299404806269776169, 0.3333333333333333703, 0.3299404806269776169, 0.3333333333333333703, 0.3299404806269776169, 0.3333333333333333703, 0.3299404806269776169, 0.3333333333333333703, 0.3299404806269776169, 0.3333333333333333703, 0.3299404806269776169, 0.3333333333333333703, 0.3299404806269776169, 0.3333333333333333703, 0.3299404806269776169, 0.3333333333333333703, 0.3299404806269776169, 0.3333333333333333703, 0.3299404806269776169, 0.3333333333333333703, 0.3299404806269776169, 0.3333333333333333703, 0.3299404806269776169, 0.3333333333333333703, 0.3299404806269776169, 0.3333333333333333703, 0.3299404806269776169, 0.3333333333333333703, 0.3299404806269776169, 0.3333333333333333703, 0.3299404806269776169, 0.3333333333333333703, 0.3299404806269776169, 0.3333333333333333703, 0.3299404806269776169, 0.3333333333333333703, 0.3299404806269776169, 0.3333333333333333703, 0.3299404806269776169, 0.3333333333333333703, 0.3299404806269776169, 0.3333333333333333703, 0.3299404806269776169, 0.3333333333333333703, 0.3299404806269776169, 0.3333333333333333703, 0.3299404806269776169, 0.3333333333333333703, 0.3299404806269776169, 0.3333333333333333703, 0.3299404806269776169, 0.3333333333333333703, 0.3299404806269776169, 0.3333333333333333703, 0.3299404806269776169, 0.3333333333333333703, 0.3299404806269776169, 0.3333333333333333703, 0.3299404806269776169, 0.3333333333333333703, 0.3299404806269776169, 0.3333333333333333703, 0.3299404806269776169, 0.3333333333333333703, 0.3299404806269776169, 0.3333333333333333703, 0.3299404806269776169, 0.3333333333333333703, 0.3299404806269776169, 0.3333333333333333703, 0.3299404806269776169, 0.3333333333333333703, 0.3299404806269776169, 0.3333333333333333703, 0.3299404806269776169, 0.3333333333333333703, 0.3299404806269776169, 0.3333333333333333703, 0.3299404806269776169, 0.3333333333333333703, 0.3299404806269776169, 0.3333333333333333703, 0.3299404806269776169, 0.3333333333333333703, 0.3299404806269776169, 0.3333333333333333703, 0.3299404806269776169, 0.3333333333333333703, 0.3299404806269776169, 0.3333333333333333703, 0.3299404806269776169, 0.3333333333333333703, 0.3299404806269776169, 0.3333333333333333703, 0.3299404806269776169, 0.3333333333333333703, 0.3299404806269776169, 0.3333333333333333703, 0.3299404806269776169, 0.3333333333333333703, 0.3299404806269776169, 0.3333333333333333703, 0.3299404806269776169, 0.3333333333333333703, 0.3299404806269776169, 0.3333333333333333703, 0.3299404806269776169, 0.3333333333333333703, 0.3299404806269776169, 0.3333333333333333703, 0.3299404806269776169, 0.3333333333333333703, 0.3299404806269776169, 0.3333333333333333703, 0.3299404806269776169, 0.3333333333333333703, 0.3299404806269776169, 0.3333333333333333703, 0.3299404806269776169, 0.3333333333333333703, 0.3299404806269776169, 0.3333333333333333703, 0.3299404806269776169, 0.3333333333333333703, 0.3299404806269776169, 0.3333333333333333703, 0.3299404806269776169, 0.3333333333333333703, 0.3299404806269776169, 0.3333333333333333703, 0.3299404806269776169, 0.3333333333333333703, 0.3299404806269776169, 0.3333333333333333703, 0.3299404806269776169, 0.3333333333333333703, 0.3299404806269776169, 0.3333333333333333703, 0.3299404806269776169, 0.3333333333333333703, 0.3299404806269776169, 0.3333333333333333703, 0.3299404806269776169, 0.3333333333333333703, 0.3299404806269776169, 0.3333333333333333703, 0.3299404806269776169, 0.3333333333333333703, 0.3299404806269776169, 0.3333333333333333703, 0.3299404806269776169, 0.3333333333333333703, 0.3299404806269776169, 0.3333333333333333703, 0.3299404806269776169, 0.3333333333333333703, 0.3299404806269776169, 0.3333333333333333703, 0.3299404806269776169, 0.3333333333333333703, 0.3299404806269776169, 0.3333333333333333703, 0.3299404806269776169, 0.3333333333333333703, 0.3299404806269776169, 0.3333333333333333703, 0.3299404806269776169, 0.3333333333333333703, 0.3299404806269776169, 0.3333333333333333703, 0.3299404806269776169, 0.3333333333333333703, 0.3299404806269776169, 0.3333333333333333703, 0.3299404806269776169, 0.3333333333333333703, 0.3299404806269776169, 0.3333333333333333703, 0.3299404806269776169, 0.3333333333333333703, 0.3299404806269776169, 0.3333333333333333703, 0.3299404806269776169, 0.3333333333333333703, 0.3299404806269776169, 0.3333333333333333703, 0.3299404806269776169, 0.3333333333333333703, 0.3299404806269776169, 0.3333333333333333703, 0.3299404806269776169, 0.3333333333333333703, 0.3299404806269776169, 0.3333333333333333703, 0.3299404806269776169, 0.3333333333333333703, 0.3299404806269776169, 0.3333333333333333703, 0.3299404806269776169, 0.3333333333333333703, 0.3299404806269776169, 0.3333333333333333703, 0.3299404806269776169, 0.3333333333333333703, 0.3299404806269776169, 0.3333333333333333703, 0.3299404806269776169, 0.3333333333333333703, 0.3299404806269776169, 0.3333333333333333703, 0.3299404806269776169, 0.3333333333333333703, 0.3299404806269776169, 0.3333333333333333703, 0.3299404806269776169, 0.3333333333333333703, 0.3299404806269776169, 0.3333333333333333703, 0.3299404806269776169, 0.3333333333333333703, 0.3299404806269776169, 0.3333333333333333703, 0.3299404806269776169, 0.3333333333333333703, 0.3299404806269776169, 0.3333333333333333703, 0.3299404806269776169, 0.3333333333333333703, 0.3299404806269776169, 0.3333333333333333703, 0.3299404806269776169, 0.3333333333333333703, 0.3299404806269776169, 0.3333333333333333703, 0.3299404806269776169, 0.3333333333333333703, 0.3299404806269776169, 0.3333333333333333703, 0.3299404806269776169, 0.3333333333333333703, 0.3299404806269776169, 0.3333333333333333703, 0.3299404806269776169, 0.3333333333333333703, 0.3299404806269776169, 0.3333333333333333703, 0.3299404806269776169, 0.3333333333333333703, 0.3299404806269776169, 0.3333333333333333703, 0.3299404806269776169, 0.3333333333333333703, 0.3299404806269776169, 0.3333333333333333703, 0.3299404806269776169, 0.3333333333333333703, 0.3299404806269776169, 0.3333333333333333703, 0.3299404806269776169, 0.3333333333333333703, 0.3299404806269776169, 0.3333333333333333703, 0.3299404806269776169, 0.3333333333333333703, 0.3299404806269776169, 0.3333333333333333703, 0.3299404806269776169, 0.3333333333333333703, 0.3299404806269776169, 0.3333333333333333703, 0.3299404806269776169, 0.3333333333333333703, 0.3299404806269776169, 0.3333333333333333703, 0.3299404806269776169, 0.3333333333333333703, 0.3299404806269776169, 0.3333333333333333703, 0.3299404806269776169, 0.3333333333333333703, 0.3299404806269776169, 0.3333333333333333703, 0.3299404806269776169, 0.3333333333333333703, 0.3299404806269776169, 0.3333333333333333703, 0.3299404806269776169, 0.3333333333333333703, 0.3299404806269776169, 0.3333333333333333703, 0.3299404806269776169, 0.3333333333333333703, 0.3299404806269776169, 0.3333333333333333703, 0.3299404806269776169, 0.3333333333333333703, 0.3299404806269776169, 0.3333333333333333703, 0.3299404806269776169, 0.3333333333333333703, 0.3299404806269776169, 0.3333333333333333703, 0.3299404806269776169, 0.3333333333333333703, 0.3299404806269776169, 0.3333333333333333703, 0.3299404806269776169, 0.3333333333333333703, 0.3299404806269776169, 0.3333333333333333703, 0.3299404806269776169, 0.3333333333333333703, 0.3299404806269776169, 0.3333333333333333703, 0.3299404806269776169, 0.3333333333333333703, 0.3299404806269776169, 0.3333333333333333703, 0.3299404806269776169, 0.3333333333333333703, 0.3299404806269776169, 0.3333333333333333703, 0.3299404806269776169, 0.3333333333333333703, 0.3299404806269776169, 0.3333333333333333703, 0.3299404806269776169, 0.3333333333333333703, 0.3299404806269776169, 0.3333333333333333703, 0.3299404806269776169, 0.3333333333333333703, 0.3299404806269776169, 0.3333333333333333703, 0.3299404806269776169, 0.3333333333333333703, 0.3299404806269776169, 0.3333333333333333703, 0.3299404806269776169, 0.3333333333333333703, 0.3299404806269776169, 0.3333333333333333703, 0.3299404806269776169, 0.3333333333333333703, 0.3299404806269776169, 0.3333333333333333703, 0.3299404806269776169, 0.3333333333333333703, 0.3299404806269776169, 0.3333333333333333703, 0.3299404806269776169, 0.3333333333333333703, 0.3299404806269776169, 0.3333333333333333703, 0.3299404806269776169, 0.3333333333333333703, 0.3299404806269776169, 0.3333333333333333703, 0.3299404806269776169, 0.3333333333333333703, 0.3299404806269776169, 0.3333333333333333703, 0.3299404806269776169, 0.3333333333333333703, 0.3299404806269776169, 0.3333333333333333703, 0.3299404806269776169, 0.3333333333333333703, 0.3299404806269776169, 0.3333333333333333703, 0.3299404806269776169, 0.3333333333333333703, 0.3299404806269776169, 0.3333333333333333703, 0.3299404806269776169, 0.3333333333333333703, 0.3299404806269776169, 0.3333333333333333703, 0.3299404806269776169, 0.3333333333333333703, 0.3299404806269776169, 0.3333333333333333703, 0.3299404806269776169, 0.3333333333333333703, 0.3299404806269776169, 0.3333333333333333703, 0.3299404806269776169, 0.3333333333333333703, 0.3299404806269776169, 0.3333333333333333703, 0.3299404806269776169, 0.3333333333333333703, 0.3299404806269776169, 0.3333333333333333703, 0.3299404806269776169, 0.3333333333333333703, 0.3299404806269776169, 0.3333333333333333703, 0.3299404806269776169, 0.3333333333333333703, 0.3299404806269776169, 0.3333333333333333703, 0.3299404806269776169, 0.3333333333333333703, 0.3299404806269776169, 0.3333333333333333703, 0.3299404806269776169, 0.3333333333333333703, 0.3299404806269776169, 0.3333333333333333703, 0.3299404806269776169, 0.3333333333333333703, 0.3299404806269776169, 0.3333333333333333703, 0.3299404806269776169, 0.3333333333333333703, 0.3299404806269776169, 0.3333333333333333703, 0.3299404806269776169, 0.3333333333333333703, 0.3299404806269776169, 0.3333333333333333703, 0.3299404806269776169, 0.3333333333333333703, 0.3299404806269776169, 0.3333333333333333703, 0.3299404806269776169, 0.3333333333333333703, 0.3299404806269776169, 0.3333333333333333703, 0.3299404806269776169, 0.3333333333333333703, 0.3299404806269776169, 0.3333333333333333703, 0.3299404806269776169, 0.3333333333333333703, 0.3299404806269776169, 0.3333333333333333703, 0.3299404806269776169, 0.3333333333333333703, 0.3299404806269776169, 0.3333333333333333703, 0.3299404806269776169, 0.3333333333333333703, 0.3299404806269776169, 0.3333333333333333703, 0.3299404806269776169, 0.3333333333333333703, 0.3299404806269776169, 0.3333333333333333703, 0.3299404806269776169, 0.3333333333333333703, 0.3299404806269776169, 0.3333333333333333703, 0.3299404806269776169, 0.3333333333333333703, 0.3299404806269776169, 0.3333333333333333703, 0.3299404806269776169, 0.3333333333333333703, 0.3299404806269776169, 0.3333333333333333703, 0.3299404806269776169, 0.3333333333333333703, 0.3299404806269776169, 0.3333333333333333703, 0.3299404806269776169, 0.3333333333333333703, 0.3299404806269776169, 0.3333333333333333703, 0.3299404806269776169, 0.3333333333333333703, 0.3299404806269776169, 0.3333333333333333703, 0.3299404806269776169, 0.3333333333333333703, 0.3299404806269776169, 0.3333333333333333703, 0.3299404806269776169, 0.3333333333333333703, 0.3299404806269776169, 0.3333333333333333703, 0.3299404806269776169, 0.3333333333333333703, 0.3299404806269776169, 0.3333333333333333703, 0.3299404806269776169, 0.3333333333333333703, 0.3299404806269776169, 0.3333333333333333703, 0.3299404806269776169, 0.3333333333333333703, 0.3299404806269776169, 0.3333333333333333703, 0.3299404806269776169, 0.3333333333333333703, 0.3299404806269776169, 0.3333333333333333703, 0.3299404806269776169, 0.3333333333333333703, 0.3299404806269776169, 0.3333333333333333703, 0.3299404806269776169, 0.3333333333333333703, 0.3299404806269776169, 0.3333333333333333703, 0.3299404806269776169, 0.3333333333333333703, 0.3299404806269776169, 0.3333333333333333703, 0.3299404806269776169, 0.3333333333333333703, 0.3299404806269776169, 0.3333333333333333703, 0.3299404806269776169, 0.3333333333333333703, 0.3299404806269776169, 0.3333333333333333703, 0.3299404806269776169, 0.3333333333333333703, 0.3299404806269776169, 0.3333333333333333703, 0.3299404806269776169, 0.3333333333333333703, 0.3299404806269776169, 0.3333333333333333703, 0.3299404806269776169, 0.3333333333333333703, 0.3299404806269776169, 0.3333333333333333703, 0.3299404806269776169, 0.3333333333333333703, 0.3299404806269776169, 0.3333333333333333703, 0.3299404806269776169, 0.3333333333333333703, 0.3299404806269776169, 0.3333333333333333703, 0.3299404806269776169, 0.3333333333333333703, 0.3299404806269776169, 0.3333333333333333703, 0.3299404806269776169, 0.3333333333333333703, 0.3299404806269776169, 0.3333333333333333703, 0.3299404806269776169, 0.3333333333333333703, 0.3299404806269776169, 0.3333333333333333703, 0.3299404806269776169, 0.3333333333333333703, 0.3299404806269776169, 0.3333333333333333703, 0.3299404806269776169, 0.3333333333333333703, 0.3299404806269776169, 0.3333333333333333703, 0.3299404806269776169, 0.3333333333333333703, 0.3299404806269776169, 0.3333333333333333703, 0.3299404806269776169, 0.3333333333333333703, 0.3299404806269776169, 0.3333333333333333703, 0.3299404806269776169, 0.3333333333333333703, 0.3299404806269776169, 0.3333333333333333703, 0.3299404806269776169, 0.3333333333333333703, 0.3299404806269776169, 0.3333333333333333703, 0.3299404806269776169, 0.3333333333333333703, 0.3299404806269776169, 0.3333333333333333703, 0.3299404806269776169, 0.3333333333333333703, 0.3299404806269776169, 0.3333333333333333703, 0.3299404806269776169, 0.3333333333333333703, 0.3299404806269776169, 0.3333333333333333703, 0.3299404806269776169, 0.3333333333333333703, 0.3299404806269776169, 0.3333333333333333703, 0.3299404806269776169, 0.3333333333333333703, 0.3299404806269776169, 0.3333333333333333703, 0.3299404806269776169, 0.3333333333333333703, 0.3299404806269776169, 0.3333333333333333703, 0.3299404806269776169, 0.3333333333333333703, 0.3299404806269776169, 0.3333333333333333703, 0.3299404806269776169, 0.3333333333333333703, 0.3299404806269776169, 0.3333333333333333703, 0.3299404806269776169, 0.3333333333333333703, 0.3299404806269776169, 0.3333333333333333703, 0.3299404806269776169, 0.3333333333333333703, 0.3299404806269776169, 0.3333333333333333703, 0.3299404806269776169, 0.3333333333333333703, 0.3299404806269776169, 0.3333333333333333703, 0.3299404806269776169, 0.3333333333333333703, 0.3299404806269776169, 0.3333333333333333703, 0.3299404806269776169, 0.3333333333333333703, 0.3299404806269776169, 0.3333333333333333703, 0.3299404806269776169, 0.3333333333333333703, 0.3299404806269776169, 0.3333333333333333703, 0.3299404806269776169, 0.3333333333333333703, 0.3299404806269776169, 0.3333333333333333703, 0.3299404806269776169, 0.3333333333333333703, 0.3299404806269776169, 0.3333333333333333703, 0.3299404806269776169, 0.3333333333333333703, 0.3299404806269776169, 0.3333333333333333703, 0.3299404806269776169, 0.3333333333333333703, 0.3299404806269776169, 0.3333333333333333703, 0.3299404806269776169, 0.3333333333333333703, 0.3299404806269776169, 0.3333333333333333703, 0.3299404806269776169, 0.3333333333333333703, 0.3299404806269776169, 0.3333333333333333703, 0.3299404806269776169, 0.3333333333333333703, 0.3299404806269776169, 0.3333333333333333703, 0.3299404806269776169, 0.3333333333333333703, 0.3299404806269776169, 0.3333333333333333703, 0.3299404806269776169, 0.3333333333333333703, 0.3299404806269776169, 0.3333333333333333703, 0.3299404806269776169, 0.3333333333333333703, 0.3299404806269776169, 0.3333333333333333703, 0.3299404806269776169, 0.3333333333333333703, 0.3299404806269776169, 0.3333333333333333703, 0.3299404806269776169, 0.3333333333333333703, 0.3299404806269776169, 0.3333333333333333703, 0.3299404806269776169, 0.3333333333333333703, 0.3299404806269776169, 0.3333333333333333703, 0.3299404806269776169, 0.3333333333333333703, 0.3299404806269776169, 0.3333333333333333703, 0.3299404806269776169, 0.3333333333333333703, 0.3299404806269776169, 0.3333333333333333703, 0.3299404806269776169, 0.3333333333333333703, 0.3299404806269776169, 0.3333333333333333703, 0.3299404806269776169, 0.3333333333333333703, 0.3299404806269776169, 0.3333333333333333703, 0.3299404806269776169, 0.3333333333333333703, 0.3299404806269776169, 0.3333333333333333703, 0.3299404806269776169, 0.3333333333333333703, 0.3299404806269776169, 0.3333333333333333703, 0.3299404806269776169, 0.3333333333333333703, 0.3299404806269776169, 0.3333333333333333703, 0.3299404806269776169, 0.3333333333333333703, 0.3299404806269776169, 0.3333333333333333703, 0.3299404806269776169, 0.3333333333333333703, 0.3299404806269776169, 0.3333333333333333703, 0.3299404806269776169, 0.3333333333333333703, 0.3299404806269776169, 0.3333333333333333703, 0.3299404806269776169, 0.3333333333333333703, 0.3299404806269776169, 0.3333333333333333703, 0.3299404806269776169, 0.3333333333333333703, 0.3299404806269776169, 0.3333333333333333703, 0.3299404806269776169, 0.3333333333333333703, 0.3299404806269776169, 0.3333333333333333703, 0.3299404806269776169, 0.3333333333333333703, 0.3299404806269776169, 0.3333333333333333703, 0.3299404806269776169, 0.3333333333333333703, 0.3299404806269776169, 0.3333333333333333703, 0.3299404806269776169, 0.3333333333333333703, 0.3299404806269776169, 0.3333333333333333703, 0.3299404806269776169, 0.3333333333333333703, 0.3299404806269776169, 0.3333333333333333703, 0.3299404806269776169, 0.3333333333333333703, 0.3299404806269776169, 0.3333333333333333703, 0.3299404806269776169, 0.3333333333333333703, 0.3299404806269776169, 0.3333333333333333703, 0.3299404806269776169, 0.3333333333333333703, 0.3299404806269776169, 0.3333333333333333703, 0.3299404806269776169, 0.3333333333333333703, 0.3299404806269776169, 0.3333333333333333703, 0.3299404806269776169, 0.3333333333333333703, 0.3299404806269776169, 0.3333333333333333703, 0.3299404806269776169, 0.3333333333333333703, 0.3299404806269776169, 0.3333333333333333703, 0.3299404806269776169, 0.3333333333333333703, 0.3299404806269776169, 0.3333333333333333703, 0.3299404806269776169, 0.3333333333333333703, 0.3299404806269776169, 0.3333333333333333703, 0.3299404806269776169, 0.3333333333333333703, 0.3299404806269776169, 0.3333333333333333703, 0.3299404806269776169, 0.3333333333333333703, 0.3299404806269776169, 0.3333333333333333703, 0.3299404806269776169, 0.3333333333333333703, 0.3299404806269776169, 0.3333333333333333703, 0.3299404806269776169, 0.3333333333333333703, 0.3299404806269776169, 0.3333333333333333703, 0.3299404806269776169, 0.3333333333333333703, 0.3299404806269776169, 0.3333333333333333703, 0.3299404806269776169, 0.3333333333333333703, 0.3299404806269776169, 0.3333333333333333703, 0.3299404806269776169, 0.3333333333333333703, 0.3299404806269776169, 0.3333333333333333703, 0.3299404806269776169, 0.3333333333333333703, 0.3299404806269776169, 0.3333333333333333703, 0.3299404806269776169, 0.3333333333333333703, 0.3299404806269776169, 0.3333333333333333703, 0.3299404806269776169, 0.3333333333333333703, 0.3299404806269776169, 0.3333333333333333703, 0.3320603117974822438, 0.3317425830320511193),
 ( 1.000000000000000000, 0.9898214418809326842, 1.000000000000000000, 0.9898214418809326842, 1.000000000000000000, 0.9898214418809326842, 1.000000000000000000, 0.9898214418809326842, 1.000000000000000000, 0.9898214418809326842, 1.000000000000000000, 0.9898214418809326842, 1.000000000000000000, 0.9898214418809326842, 1.000000000000000000, 0.9898214418809326842, 1.000000000000000000, 0.9898214418809326842, 1.000000000000000000, 0.9898214418809326842, 1.000000000000000000, 0.9898214418809326842, 1.000000000000000000, 0.9898214418809326842, 1.000000000000000000, 0.9898214418809326842, 1.000000000000000000, 0.9898214418809326842, 1.000000000000000000, 0.9898214418809326842, 1.000000000000000000, 0.9898214418809326842, 1.000000000000000000, 0.9898214418809326842, 1.000000000000000000, 0.9898214418809326842, 1.000000000000000000, 0.9898214418809326842, 1.000000000000000000, 0.9898214418809326842, 1.000000000000000000, 0.9898214418809326842, 1.000000000000000000, 0.9898214418809326842, 1.000000000000000000, 0.9898214418809326842, 1.000000000000000000, 0.9898214418809326842, 1.000000000000000000, 0.9898214418809326842, 1.000000000000000000, 0.9898214418809326842, 1.000000000000000000, 0.9898214418809326842, 1.000000000000000000, 0.9898214418809326842, 1.000000000000000000, 0.9898214418809326842, 1.000000000000000000, 0.9898214418809326842, 1.000000000000000000, 0.9898214418809326842, 1.000000000000000000, 0.9898214418809326842, 1.000000000000000000, 0.9898214418809326842, 1.000000000000000000, 0.9898214418809326842, 1.000000000000000000, 0.9898214418809326842, 1.000000000000000000, 0.9898214418809326842, 1.000000000000000000, 0.9898214418809326842, 1.000000000000000000, 0.9898214418809326842, 1.000000000000000000, 0.9898214418809326842, 1.000000000000000000, 0.9898214418809326842, 1.000000000000000000, 0.9898214418809326842, 1.000000000000000000, 0.9898214418809326842, 1.000000000000000000, 0.9898214418809326842, 1.000000000000000000, 0.9898214418809326842, 1.000000000000000000, 0.9898214418809326842, 1.000000000000000000, 0.9898214418809326842, 1.000000000000000000, 0.9898214418809326842, 1.000000000000000000, 0.9898214418809326842, 1.000000000000000000, 0.9898214418809326842, 1.000000000000000000, 0.9898214418809326842, 1.000000000000000000, 0.9898214418809326842, 1.000000000000000000, 0.9898214418809326842, 1.000000000000000000, 0.9898214418809326842, 1.000000000000000000, 0.9898214418809326842, 1.000000000000000000, 0.9898214418809326842, 1.000000000000000000, 0.9898214418809326842, 1.000000000000000000, 0.9898214418809326842, 1.000000000000000000, 0.9898214418809326842, 1.000000000000000000, 0.9898214418809326842, 1.000000000000000000, 0.9898214418809326842, 1.000000000000000000, 0.9898214418809326842, 1.000000000000000000, 0.9898214418809326842, 1.000000000000000000, 0.9898214418809326842, 1.000000000000000000, 0.9898214418809326842, 1.000000000000000000, 0.9898214418809326842, 1.000000000000000000, 0.9898214418809326842, 1.000000000000000000, 0.9898214418809326842, 1.000000000000000000, 0.9898214418809326842, 1.000000000000000000, 0.9898214418809326842, 1.000000000000000000, 0.9898214418809326842, 1.000000000000000000, 0.9898214418809326842, 1.000000000000000000, 0.9898214418809326842, 1.000000000000000000, 0.9898214418809326842, 1.000000000000000000, 0.9898214418809326842, 1.000000000000000000, 0.9898214418809326842, 1.000000000000000000, 0.9898214418809326842, 1.000000000000000000, 0.9898214418809326842, 1.000000000000000000, 0.9898214418809326842, 1.000000000000000000, 0.9898214418809326842, 1.000000000000000000, 0.9898214418809326842, 1.000000000000000000, 0.9898214418809326842, 1.000000000000000000, 0.9898214418809326842, 1.000000000000000000, 0.9898214418809326842, 1.000000000000000000, 0.9898214418809326842, 1.000000000000000000, 0.9898214418809326842, 1.000000000000000000, 0.9898214418809326842, 1.000000000000000000, 0.9898214418809326842, 1.000000000000000000, 0.9898214418809326842, 1.000000000000000000, 0.9898214418809326842, 1.000000000000000000, 0.9898214418809326842, 1.000000000000000000, 0.9898214418809326842, 1.000000000000000000, 0.9898214418809326842, 1.000000000000000000, 0.9898214418809326842, 1.000000000000000000, 0.9898214418809326842, 1.000000000000000000, 0.9898214418809326842, 1.000000000000000000, 0.9898214418809326842, 1.000000000000000000, 0.9898214418809326842, 1.000000000000000000, 0.9898214418809326842, 1.000000000000000000, 0.9898214418809326842, 1.000000000000000000, 0.9898214418809326842, 1.000000000000000000, 0.9898214418809326842, 1.000000000000000000, 0.9898214418809326842, 1.000000000000000000, 0.9898214418809326842, 1.000000000000000000, 0.9898214418809326842, 1.000000000000000000, 0.9898214418809326842, 1.000000000000000000, 0.9898214418809326842, 1.000000000000000000, 0.9898214418809326842, 1.000000000000000000, 0.9898214418809326842, 1.000000000000000000, 0.9898214418809326842, 1.000000000000000000, 0.9898214418809326842, 1.000000000000000000, 0.9898214418809326842, 1.000000000000000000, 0.9898214418809326842, 1.000000000000000000, 0.9898214418809326842, 1.000000000000000000, 0.9898214418809326842, 1.000000000000000000, 0.9898214418809326842, 1.000000000000000000, 0.9898214418809326842, 1.000000000000000000, 0.9898214418809326842, 1.000000000000000000, 0.9898214418809326842, 1.000000000000000000, 0.9898214418809326842, 1.000000000000000000, 0.9898214418809326842, 1.000000000000000000, 0.9898214418809326842, 1.000000000000000000, 0.9898214418809326842, 1.000000000000000000, 0.9898214418809326842, 1.000000000000000000, 0.9898214418809326842, 1.000000000000000000, 0.9898214418809326842, 1.000000000000000000, 0.9898214418809326842, 1.000000000000000000, 0.9898214418809326842, 1.000000000000000000, 0.9898214418809326842, 1.000000000000000000, 0.9898214418809326842, 1.000000000000000000, 0.9898214418809326842, 1.000000000000000000, 0.9898214418809326842, 1.000000000000000000, 0.9898214418809326842, 1.000000000000000000, 0.9898214418809326842, 1.000000000000000000, 0.9898214418809326842, 1.000000000000000000, 0.9898214418809326842, 1.000000000000000000, 0.9898214418809326842, 1.000000000000000000, 0.9898214418809326842, 1.000000000000000000, 0.9898214418809326842, 1.000000000000000000, 0.9898214418809326842, 1.000000000000000000, 0.9898214418809326842, 1.000000000000000000, 0.9898214418809326842, 1.000000000000000000, 0.9898214418809326842, 1.000000000000000000, 0.9898214418809326842, 1.000000000000000000, 0.9898214418809326842, 1.000000000000000000, 0.9898214418809326842, 1.000000000000000000, 0.9898214418809326842, 1.000000000000000000, 0.9898214418809326842, 1.000000000000000000, 0.9898214418809326842, 1.000000000000000000, 0.9898214418809326842, 1.000000000000000000, 0.9898214418809326842, 1.000000000000000000, 0.9898214418809326842, 1.000000000000000000, 0.9898214418809326842, 1.000000000000000000, 0.9898214418809326842, 1.000000000000000000, 0.9898214418809326842, 1.000000000000000000, 0.9898214418809326842, 1.000000000000000000, 0.9898214418809326842, 1.000000000000000000, 0.9898214418809326842, 1.000000000000000000, 0.9898214418809326842, 1.000000000000000000, 0.9898214418809326842, 1.000000000000000000, 0.9898214418809326842, 1.000000000000000000, 0.9898214418809326842, 1.000000000000000000, 0.9898214418809326842, 1.000000000000000000, 0.9898214418809326842, 1.000000000000000000, 0.9898214418809326842, 1.000000000000000000, 0.9898214418809326842, 1.000000000000000000, 0.9898214418809326842, 1.000000000000000000, 0.9898214418809326842, 1.000000000000000000, 0.9898214418809326842, 1.000000000000000000, 0.9898214418809326842, 1.000000000000000000, 0.9898214418809326842, 1.000000000000000000, 0.9898214418809326842, 1.000000000000000000, 0.9898214418809326842, 1.000000000000000000, 0.9898214418809326842, 1.000000000000000000, 0.9898214418809326842, 1.000000000000000000, 0.9898214418809326842, 1.000000000000000000, 0.9898214418809326842, 1.000000000000000000, 0.9898214418809326842, 1.000000000000000000, 0.9898214418809326842, 1.000000000000000000, 0.9898214418809326842, 1.000000000000000000, 0.9898214418809326842, 1.000000000000000000, 0.9898214418809326842, 1.000000000000000000, 0.9898214418809326842, 1.000000000000000000, 0.9898214418809326842, 1.000000000000000000, 0.9898214418809326842, 1.000000000000000000, 0.9898214418809326842, 1.000000000000000000, 0.9898214418809326842, 1.000000000000000000, 0.9898214418809326842, 1.000000000000000000, 0.9898214418809326842, 1.000000000000000000, 0.9898214418809326842, 1.000000000000000000, 0.9898214418809326842, 1.000000000000000000, 0.9898214418809326842, 1.000000000000000000, 0.9898214418809326842, 1.000000000000000000, 0.9898214418809326842, 1.000000000000000000, 0.9898214418809326842, 1.000000000000000000, 0.9898214418809326842, 1.000000000000000000, 0.9898214418809326842, 1.000000000000000000, 0.9898214418809326842, 1.000000000000000000, 0.9898214418809326842, 1.000000000000000000, 0.9898214418809326842, 1.000000000000000000, 0.9898214418809326842, 1.000000000000000000, 0.9898214418809326842, 1.000000000000000000, 0.9898214418809326842, 1.000000000000000000, 0.9898214418809326842, 1.000000000000000000, 0.9898214418809326842, 1.000000000000000000, 0.9898214418809326842, 1.000000000000000000, 0.9898214418809326842, 1.000000000000000000, 0.9898214418809326842, 1.000000000000000000, 0.9898214418809326842, 1.000000000000000000, 0.9898214418809326842, 1.000000000000000000, 0.9898214418809326842, 1.000000000000000000, 0.9898214418809326842, 1.000000000000000000, 0.9898214418809326842, 1.000000000000000000, 0.9898214418809326842, 1.000000000000000000, 0.9898214418809326842, 1.000000000000000000, 0.9898214418809326842, 1.000000000000000000, 0.9898214418809326842, 1.000000000000000000, 0.9898214418809326842, 1.000000000000000000, 0.9898214418809326842, 1.000000000000000000, 0.9898214418809326842, 1.000000000000000000, 0.9898214418809326842, 1.000000000000000000, 0.9898214418809326842, 1.000000000000000000, 0.9898214418809326842, 1.000000000000000000, 0.9898214418809326842, 1.000000000000000000, 0.9898214418809326842, 1.000000000000000000, 0.9898214418809326842, 1.000000000000000000, 0.9898214418809326842, 1.000000000000000000, 0.9898214418809326842, 1.000000000000000000, 0.9898214418809326842, 1.000000000000000000, 0.9898214418809326842, 1.000000000000000000, 0.9898214418809326842, 1.000000000000000000, 0.9898214418809326842, 1.000000000000000000, 0.9898214418809326842, 1.000000000000000000, 0.9898214418809326842, 1.000000000000000000, 0.9898214418809326842, 1.000000000000000000, 0.9898214418809326842, 1.000000000000000000, 0.9898214418809326842, 1.000000000000000000, 0.9898214418809326842, 1.000000000000000000, 0.9898214418809326842, 1.000000000000000000, 0.9898214418809326842, 1.000000000000000000, 0.9898214418809326842, 1.000000000000000000, 0.9898214418809326842, 1.000000000000000000, 0.9898214418809326842, 1.000000000000000000, 0.9898214418809326842, 1.000000000000000000, 0.9898214418809326842, 1.000000000000000000, 0.9898214418809326842, 1.000000000000000000, 0.9898214418809326842, 1.000000000000000000, 0.9898214418809326842, 1.000000000000000000, 0.9898214418809326842, 1.000000000000000000, 0.9898214418809326842, 1.000000000000000000, 0.9898214418809326842, 1.000000000000000000, 0.9898214418809326842, 1.000000000000000000, 0.9898214418809326842, 1.000000000000000000, 0.9898214418809326842, 1.000000000000000000, 0.9898214418809326842, 1.000000000000000000, 0.9898214418809326842, 1.000000000000000000, 0.9898214418809326842, 1.000000000000000000, 0.9898214418809326842, 1.000000000000000000, 0.9898214418809326842, 1.000000000000000000, 0.9898214418809326842, 1.000000000000000000, 0.9898214418809326842, 1.000000000000000000, 0.9898214418809326842, 1.000000000000000000, 0.9898214418809326842, 1.000000000000000000, 0.9898214418809326842, 1.000000000000000000, 0.9898214418809326842, 1.000000000000000000, 0.9898214418809326842, 1.000000000000000000, 0.9898214418809326842, 1.000000000000000000, 0.9898214418809326842, 1.000000000000000000, 0.9898214418809326842, 1.000000000000000000, 0.9898214418809326842, 1.000000000000000000, 0.9898214418809326842, 1.000000000000000000, 0.9898214418809326842, 1.000000000000000000, 0.9898214418809326842, 1.000000000000000000, 0.9898214418809326842, 1.000000000000000000, 0.9898214418809326842, 1.000000000000000000, 0.9898214418809326842, 1.000000000000000000, 0.9898214418809326842, 1.000000000000000000, 0.9898214418809326842, 1.000000000000000000, 0.9898214418809326842, 1.000000000000000000, 0.9898214418809326842, 1.000000000000000000, 0.9898214418809326842, 1.000000000000000000, 0.9898214418809326842, 1.000000000000000000, 0.9898214418809326842, 1.000000000000000000, 0.9898214418809326842, 1.000000000000000000, 0.9898214418809326842, 1.000000000000000000, 0.9898214418809326842, 1.000000000000000000, 0.9898214418809326842, 1.000000000000000000, 0.9898214418809326842, 1.000000000000000000, 0.9898214418809326842, 1.000000000000000000, 0.9898214418809326842, 1.000000000000000000, 0.9898214418809326842, 1.000000000000000000, 0.9898214418809326842, 1.000000000000000000, 0.9898214418809326842, 1.000000000000000000, 0.9898214418809326842, 1.000000000000000000, 0.9898214418809326842, 1.000000000000000000, 0.9898214418809326842, 1.000000000000000000, 0.9898214418809326842, 1.000000000000000000, 0.9898214418809326842, 1.000000000000000000, 0.9898214418809326842, 1.000000000000000000, 0.9898214418809326842, 1.000000000000000000, 0.9898214418809326842, 1.000000000000000000, 0.9898214418809326842, 1.000000000000000000, 0.9898214418809326842, 1.000000000000000000, 0.9898214418809326842, 1.000000000000000000, 0.9898214418809326842, 1.000000000000000000, 0.9898214418809326842, 1.000000000000000000, 0.9898214418809326842, 1.000000000000000000, 0.9898214418809326842, 1.000000000000000000, 0.9898214418809326842, 1.000000000000000000, 0.9898214418809326842, 1.000000000000000000, 0.9898214418809326842, 1.000000000000000000, 0.9898214418809326842, 1.000000000000000000, 0.9898214418809326842, 1.000000000000000000, 0.9898214418809326842, 1.000000000000000000, 0.9898214418809326842, 1.000000000000000000, 0.9898214418809326842, 1.000000000000000000, 0.9898214418809326842, 1.000000000000000000, 0.9898214418809326842, 1.000000000000000000, 0.9898214418809326842, 1.000000000000000000, 0.9898214418809326842, 1.000000000000000000, 0.9898214418809326842, 1.000000000000000000, 0.9898214418809326842, 1.000000000000000000, 0.9898214418809326842, 1.000000000000000000, 0.9898214418809326842, 1.000000000000000000, 0.9898214418809326842, 1.000000000000000000, 0.9898214418809326842, 1.000000000000000000, 0.9898214418809326842, 1.000000000000000000, 0.9898214418809326842, 1.000000000000000000, 0.9898214418809326842, 1.000000000000000000, 0.9898214418809326842, 1.000000000000000000, 0.9898214418809326842, 1.000000000000000000, 0.9898214418809326842, 1.000000000000000000, 0.9898214418809326842, 1.000000000000000000, 0.9898214418809326842, 1.000000000000000000, 0.9898214418809326842, 1.000000000000000000, 0.9898214418809326842, 1.000000000000000000, 0.9898214418809326842, 1.000000000000000000, 0.9898214418809326842, 1.000000000000000000, 0.9898214418809326842, 1.000000000000000000, 0.9898214418809326842, 1.000000000000000000, 0.9898214418809326842, 1.000000000000000000, 0.9898214418809326842, 1.000000000000000000, 0.9898214418809326842, 1.000000000000000000, 0.9898214418809326842, 1.000000000000000000, 0.9898214418809326842, 1.000000000000000000, 0.9898214418809326842, 1.000000000000000000, 0.9898214418809326842, 1.000000000000000000, 0.9898214418809326842, 1.000000000000000000, 0.9898214418809326842, 1.000000000000000000, 0.9898214418809326842, 1.000000000000000000, 0.9898214418809326842, 1.000000000000000000, 0.9898214418809326842, 1.000000000000000000, 0.9898214418809326842, 1.000000000000000000, 0.9898214418809326842, 1.000000000000000000, 0.9898214418809326842, 1.000000000000000000, 0.9898214418809326842, 1.000000000000000000, 0.9898214418809326842, 1.000000000000000000, 0.9898214418809326842, 1.000000000000000000, 0.9898214418809326842, 1.000000000000000000, 0.9898214418809326842, 1.000000000000000000, 0.9898214418809326842, 1.000000000000000000, 0.9898214418809326842, 1.000000000000000000, 0.9898214418809326842, 1.000000000000000000, 0.9898214418809326842, 1.000000000000000000, 0.9898214418809326842, 1.000000000000000000, 0.9898214418809326842, 1.000000000000000000, 0.9898214418809326842, 1.000000000000000000, 0.9898214418809326842, 1.000000000000000000, 0.9898214418809326842, 1.000000000000000000, 0.9898214418809326842, 1.000000000000000000, 0.9898214418809326842, 1.000000000000000000, 0.9898214418809326842, 1.000000000000000000, 0.9898214418809326842, 1.000000000000000000, 0.9898214418809326842, 1.000000000000000000, 0.9898214418809326842, 1.000000000000000000, 0.9898214418809326842, 1.000000000000000000, 0.9898214418809326842, 1.000000000000000000, 0.9898214418809326842, 1.000000000000000000, 0.9898214418809326842, 1.000000000000000000, 0.9898214418809326842, 1.000000000000000000, 0.9898214418809326842, 1.000000000000000000, 0.9898214418809326842, 1.000000000000000000, 0.9898214418809326842, 1.000000000000000000, 0.9898214418809326842, 1.000000000000000000, 0.9898214418809326842, 1.000000000000000000, 0.9898214418809326842, 1.000000000000000000, 0.9898214418809326842, 1.000000000000000000, 0.9898214418809326842, 1.000000000000000000, 0.9898214418809326842, 1.000000000000000000, 0.9898214418809326842, 1.000000000000000000, 0.9898214418809326842, 1.000000000000000000, 0.9898214418809326842, 1.000000000000000000, 0.9898214418809326842, 1.000000000000000000, 0.9898214418809326842, 1.000000000000000000, 0.9898214418809326842, 1.000000000000000000, 0.9898214418809326842, 1.000000000000000000, 0.9898214418809326842, 1.000000000000000000, 0.9898214418809326842, 1.000000000000000000, 0.9898214418809326842, 1.000000000000000000, 0.9898214418809326842, 1.000000000000000000, 0.9898214418809326842, 1.000000000000000000, 0.9898214418809326842, 1.000000000000000000, 0.9898214418809326842, 1.000000000000000000, 0.9898214418809326842, 1.000000000000000000, 0.9898214418809326842, 1.000000000000000000, 0.9898214418809326842, 1.000000000000000000, 0.9898214418809326842, 1.000000000000000000, 0.9898214418809326842, 1.000000000000000000, 0.9898214418809326842, 1.000000000000000000, 0.9898214418809326842, 1.000000000000000000, 0.9898214418809326842, 1.000000000000000000, 0.9898214418809326842, 1.000000000000000000, 0.9898214418809326842, 1.000000000000000000, 0.9898214418809326842, 1.000000000000000000, 0.9898214418809326842, 1.000000000000000000, 0.9898214418809326842, 1.000000000000000000, 0.9898214418809326842, 1.000000000000000000, 0.9898214418809326842, 1.000000000000000000, 0.9898214418809326842, 1.000000000000000000, 0.9898214418809326842, 1.000000000000000000, 0.9898214418809326842, 1.000000000000000000, 0.9898214418809326842, 1.000000000000000000, 0.9898214418809326842, 1.000000000000000000, 0.9898214418809326842, 1.000000000000000000, 0.9898214418809326842, 1.000000000000000000, 0.9898214418809326842, 1.000000000000000000, 0.9898214418809326842, 1.000000000000000000, 0.9898214418809326842, 1.000000000000000000, 0.9898214418809326842, 1.000000000000000000, 0.9898214418809326842, 1.000000000000000000, 0.9898214418809326842, 1.000000000000000000, 0.9961809353924466759, 0.9952277490961531914),
 ( 0.3333333333333333703, 0.3299404806269776169, 0.3333333333333333703, 0.3299404806269776169, 0.3333333333333333703, 0.3299404806269776169, 0.3333333333333333703, 0.3299404806269776169, 0.3333333333333333703, 0.3299404806269776169, 0.3333333333333333703, 0.3299404806269776169, 0.3333333333333333703, 0.3299404806269776169, 0.3333333333333333703, 0.3299404806269776169, 0.3333333333333333703, 0.3299404806269776169, 0.3333333333333333703, 0.3299404806269776169, 0.3333333333333333703, 0.3299404806269776169, 0.3333333333333333703, 0.3299404806269776169, 0.3333333333333333703, 0.3299404806269776169, 0.3333333333333333703, 0.3299404806269776169, 0.3333333333333333703, 0.3299404806269776169, 0.3333333333333333703, 0.3299404806269776169, 0.3333333333333333703, 0.3299404806269776169, 0.3333333333333333703, 0.3299404806269776169, 0.3333333333333333703, 0.3299404806269776169, 0.3333333333333333703, 0.3299404806269776169, 0.3333333333333333703, 0.3299404806269776169, 0.3333333333333333703, 0.3299404806269776169, 0.3333333333333333703, 0.3299404806269776169, 0.3333333333333333703, 0.3299404806269776169, 0.3333333333333333703, 0.3299404806269776169, 0.3333333333333333703, 0.3299404806269776169, 0.3333333333333333703, 0.3299404806269776169, 0.3333333333333333703, 0.3299404806269776169, 0.3333333333333333703, 0.3299404806269776169, 0.3333333333333333703, 0.3299404806269776169, 0.3333333333333333703, 0.3299404806269776169, 0.3333333333333333703, 0.3299404806269776169, 0.3333333333333333703, 0.3299404806269776169, 0.3333333333333333703, 0.3299404806269776169, 0.3333333333333333703, 0.3299404806269776169, 0.3333333333333333703, 0.3299404806269776169, 0.3333333333333333703, 0.3299404806269776169, 0.3333333333333333703, 0.3299404806269776169, 0.3333333333333333703, 0.3299404806269776169, 0.3333333333333333703, 0.3299404806269776169, 0.3333333333333333703, 0.3299404806269776169, 0.3333333333333333703, 0.3299404806269776169, 0.3333333333333333703, 0.3299404806269776169, 0.3333333333333333703, 0.3299404806269776169, 0.3333333333333333703, 0.3299404806269776169, 0.3333333333333333703, 0.3299404806269776169, 0.3333333333333333703, 0.3299404806269776169, 0.3333333333333333703, 0.3299404806269776169, 0.3333333333333333703, 0.3299404806269776169, 0.3333333333333333703, 0.3299404806269776169, 0.3333333333333333703, 0.3299404806269776169, 0.3333333333333333703, 0.3299404806269776169, 0.3333333333333333703, 0.3299404806269776169, 0.3333333333333333703, 0.3299404806269776169, 0.3333333333333333703, 0.3299404806269776169, 0.3333333333333333703, 0.3299404806269776169, 0.3333333333333333703, 0.3299404806269776169, 0.3333333333333333703, 0.3299404806269776169, 0.3333333333333333703, 0.3299404806269776169, 0.3333333333333333703, 0.3299404806269776169, 0.3333333333333333703, 0.3299404806269776169, 0.3333333333333333703, 0.3299404806269776169, 0.3333333333333333703, 0.3299404806269776169, 0.3333333333333333703, 0.3299404806269776169, 0.3333333333333333703, 0.3299404806269776169, 0.3333333333333333703, 0.3299404806269776169, 0.3333333333333333703, 0.3299404806269776169, 0.3333333333333333703, 0.3299404806269776169, 0.3333333333333333703, 0.3299404806269776169, 0.3333333333333333703, 0.3299404806269776169, 0.3333333333333333703, 0.3299404806269776169, 0.3333333333333333703, 0.3299404806269776169, 0.3333333333333333703, 0.3299404806269776169, 0.3333333333333333703, 0.3299404806269776169, 0.3333333333333333703, 0.3299404806269776169, 0.3333333333333333703, 0.3299404806269776169, 0.3333333333333333703, 0.3299404806269776169, 0.3333333333333333703, 0.3299404806269776169, 0.3333333333333333703, 0.3299404806269776169, 0.3333333333333333703, 0.3299404806269776169, 0.3333333333333333703, 0.3299404806269776169, 0.3333333333333333703, 0.3299404806269776169, 0.3333333333333333703, 0.3299404806269776169, 0.3333333333333333703, 0.3299404806269776169, 0.3333333333333333703, 0.3299404806269776169, 0.3333333333333333703, 0.3299404806269776169, 0.3333333333333333703, 0.3299404806269776169, 0.3333333333333333703, 0.3299404806269776169, 0.3333333333333333703, 0.3299404806269776169, 0.3333333333333333703, 0.3299404806269776169, 0.3333333333333333703, 0.3299404806269776169, 0.3333333333333333703, 0.3299404806269776169, 0.3333333333333333703, 0.3299404806269776169, 0.3333333333333333703, 0.3299404806269776169, 0.3333333333333333703, 0.3299404806269776169, 0.3333333333333333703, 0.3299404806269776169, 0.3333333333333333703, 0.3299404806269776169, 0.3333333333333333703, 0.3299404806269776169, 0.3333333333333333703, 0.3299404806269776169, 0.3333333333333333703, 0.3299404806269776169, 0.3333333333333333703, 0.3299404806269776169, 0.3333333333333333703, 0.3299404806269776169, 0.3333333333333333703, 0.3299404806269776169, 0.3333333333333333703, 0.3299404806269776169, 0.3333333333333333703, 0.3299404806269776169, 0.3333333333333333703, 0.3299404806269776169, 0.3333333333333333703, 0.3299404806269776169, 0.3333333333333333703, 0.3299404806269776169, 0.3333333333333333703, 0.3299404806269776169, 0.3333333333333333703, 0.3299404806269776169, 0.3333333333333333703, 0.3299404806269776169, 0.3333333333333333703, 0.3299404806269776169, 0.3333333333333333703, 0.3299404806269776169, 0.3333333333333333703, 0.3299404806269776169, 0.3333333333333333703, 0.3299404806269776169, 0.3333333333333333703, 0.3299404806269776169, 0.3333333333333333703, 0.3299404806269776169, 0.3333333333333333703, 0.3299404806269776169, 0.3333333333333333703, 0.3299404806269776169, 0.3333333333333333703, 0.3299404806269776169, 0.3333333333333333703, 0.3299404806269776169, 0.3333333333333333703, 0.3299404806269776169, 0.3333333333333333703, 0.3299404806269776169, 0.3333333333333333703, 0.3299404806269776169, 0.3333333333333333703, 0.3299404806269776169, 0.3333333333333333703, 0.3299404806269776169, 0.3333333333333333703, 0.3299404806269776169, 0.3333333333333333703, 0.3299404806269776169, 0.3333333333333333703, 0.3299404806269776169, 0.3333333333333333703, 0.3299404806269776169, 0.3333333333333333703, 0.3299404806269776169, 0.3333333333333333703, 0.3299404806269776169, 0.3333333333333333703, 0.3299404806269776169, 0.3333333333333333703, 0.3299404806269776169, 0.3333333333333333703, 0.3299404806269776169, 0.3333333333333333703, 0.3299404806269776169, 0.3333333333333333703, 0.3299404806269776169, 0.3333333333333333703, 0.3299404806269776169, 0.3333333333333333703, 0.3299404806269776169, 0.3333333333333333703, 0.3299404806269776169, 0.3333333333333333703, 0.3299404806269776169, 0.3333333333333333703, 0.3299404806269776169, 0.3333333333333333703, 0.3299404806269776169, 0.3333333333333333703, 0.3299404806269776169, 0.3333333333333333703, 0.3299404806269776169, 0.3333333333333333703, 0.3299404806269776169, 0.3333333333333333703, 0.3299404806269776169, 0.3333333333333333703, 0.3299404806269776169, 0.3333333333333333703, 0.3299404806269776169, 0.3333333333333333703, 0.3299404806269776169, 0.3333333333333333703, 0.3299404806269776169, 0.3333333333333333703, 0.3299404806269776169, 0.3333333333333333703, 0.3299404806269776169, 0.3333333333333333703, 0.3299404806269776169, 0.3333333333333333703, 0.3299404806269776169, 0.3333333333333333703, 0.3299404806269776169, 0.3333333333333333703, 0.3299404806269776169, 0.3333333333333333703, 0.3299404806269776169, 0.3333333333333333703, 0.3299404806269776169, 0.3333333333333333703, 0.3299404806269776169, 0.3333333333333333703, 0.3299404806269776169, 0.3333333333333333703, 0.3299404806269776169, 0.3333333333333333703, 0.3299404806269776169, 0.3333333333333333703, 0.3299404806269776169, 0.3333333333333333703, 0.3299404806269776169, 0.3333333333333333703, 0.3299404806269776169, 0.3333333333333333703, 0.3299404806269776169, 0.3333333333333333703, 0.3299404806269776169, 0.3333333333333333703, 0.3299404806269776169, 0.3333333333333333703, 0.3299404806269776169, 0.3333333333333333703, 0.3299404806269776169, 0.3333333333333333703, 0.3299404806269776169, 0.3333333333333333703, 0.3299404806269776169, 0.3333333333333333703, 0.3299404806269776169, 0.3333333333333333703, 0.3299404806269776169, 0.3333333333333333703, 0.3299404806269776169, 0.3333333333333333703, 0.3299404806269776169, 0.3333333333333333703, 0.3299404806269776169, 0.3333333333333333703, 0.3299404806269776169, 0.3333333333333333703, 0.3299404806269776169, 0.3333333333333333703, 0.3299404806269776169, 0.3333333333333333703, 0.3299404806269776169, 0.3333333333333333703, 0.3299404806269776169, 0.3333333333333333703, 0.3299404806269776169, 0.3333333333333333703, 0.3299404806269776169, 0.3333333333333333703, 0.3299404806269776169, 0.3333333333333333703, 0.3299404806269776169, 0.3333333333333333703, 0.3299404806269776169, 0.3333333333333333703, 0.3299404806269776169, 0.3333333333333333703, 0.3299404806269776169, 0.3333333333333333703, 0.3299404806269776169, 0.3333333333333333703, 0.3299404806269776169, 0.3333333333333333703, 0.3299404806269776169, 0.3333333333333333703, 0.3299404806269776169, 0.3333333333333333703, 0.3299404806269776169, 0.3333333333333333703, 0.3299404806269776169, 0.3333333333333333703, 0.3299404806269776169, 0.3333333333333333703, 0.3299404806269776169, 0.3333333333333333703, 0.3299404806269776169, 0.3333333333333333703, 0.3299404806269776169, 0.3333333333333333703, 0.3299404806269776169, 0.3333333333333333703, 0.3299404806269776169, 0.3333333333333333703, 0.3299404806269776169, 0.3333333333333333703, 0.3299404806269776169, 0.3333333333333333703, 0.3299404806269776169, 0.3333333333333333703, 0.3299404806269776169, 0.3333333333333333703, 0.3299404806269776169, 0.3333333333333333703, 0.3299404806269776169, 0.3333333333333333703, 0.3299404806269776169, 0.3333333333333333703, 0.3299404806269776169, 0.3333333333333333703, 0.3299404806269776169, 0.3333333333333333703, 0.3299404806269776169, 0.3333333333333333703, 0.3299404806269776169, 0.3333333333333333703, 0.3299404806269776169, 0.3333333333333333703, 0.3299404806269776169, 0.3333333333333333703, 0.3299404806269776169, 0.3333333333333333703, 0.3299404806269776169, 0.3333333333333333703, 0.3299404806269776169, 0.3333333333333333703, 0.3299404806269776169, 0.3333333333333333703, 0.3299404806269776169, 0.3333333333333333703, 0.3299404806269776169, 0.3333333333333333703, 0.3299404806269776169, 0.3333333333333333703, 0.3299404806269776169, 0.3333333333333333703, 0.3299404806269776169, 0.3333333333333333703, 0.3299404806269776169, 0.3333333333333333703, 0.3299404806269776169, 0.3333333333333333703, 0.3299404806269776169, 0.3333333333333333703, 0.3299404806269776169, 0.3333333333333333703, 0.3299404806269776169, 0.3333333333333333703, 0.3299404806269776169, 0.3333333333333333703, 0.3299404806269776169, 0.3333333333333333703, 0.3299404806269776169, 0.3333333333333333703, 0.3299404806269776169, 0.3333333333333333703, 0.3299404806269776169, 0.3333333333333333703, 0.3299404806269776169, 0.3333333333333333703, 0.3299404806269776169, 0.3333333333333333703, 0.3299404806269776169, 0.3333333333333333703, 0.3299404806269776169, 0.3333333333333333703, 0.3299404806269776169, 0.3333333333333333703, 0.3299404806269776169, 0.3333333333333333703, 0.3299404806269776169, 0.3333333333333333703, 0.3299404806269776169, 0.3333333333333333703, 0.3299404806269776169, 0.3333333333333333703, 0.3299404806269776169, 0.3333333333333333703, 0.3299404806269776169, 0.3333333333333333703, 0.3299404806269776169, 0.3333333333333333703, 0.3299404806269776169, 0.3333333333333333703, 0.3299404806269776169, 0.3333333333333333703, 0.3299404806269776169, 0.3333333333333333703, 0.3299404806269776169, 0.3333333333333333703, 0.3299404806269776169, 0.3333333333333333703, 0.3299404806269776169, 0.3333333333333333703, 0.3299404806269776169, 0.3333333333333333703, 0.3299404806269776169, 0.3333333333333333703, 0.3299404806269776169, 0.3333333333333333703, 0.3299404806269776169, 0.3333333333333333703, 0.3299404806269776169, 0.3333333333333333703, 0.3299404806269776169, 0.3333333333333333703, 0.3299404806269776169, 0.3333333333333333703, 0.3299404806269776169, 0.3333333333333333703, 0.3299404806269776169, 0.3333333333333333703, 0.3299404806269776169, 0.3333333333333333703, 0.3299404806269776169, 0.3333333333333333703, 0.3299404806269776169, 0.3333333333333333703, 0.3299404806269776169, 0.3333333333333333703, 0.3299404806269776169, 0.3333333333333333703, 0.3299404806269776169, 0.3333333333333333703, 0.3299404806269776169, 0.3333333333333333703, 0.3299404806269776169, 0.3333333333333333703, 0.3299404806269776169, 0.3333333333333333703, 0.3299404806269776169, 0.3333333333333333703, 0.3299404806269776169, 0.3333333333333333703, 0.3299404806269776169, 0.3333333333333333703, 0.3299404806269776169, 0.3333333333333333703, 0.3299404806269776169, 0.3333333333333333703, 0.3299404806269776169, 0.3333333333333333703, 0.3299404806269776169, 0.3333333333333333703, 0.3299404806269776169, 0.3333333333333333703, 0.3299404806269776169, 0.3333333333333333703, 0.3299404806269776169, 0.3333333333333333703, 0.3299404806269776169, 0.3333333333333333703, 0.3299404806269776169, 0.3333333333333333703, 0.3299404806269776169, 0.3333333333333333703, 0.3299404806269776169, 0.3333333333333333703, 0.3299404806269776169, 0.3333333333333333703, 0.3299404806269776169, 0.3333333333333333703, 0.3299404806269776169, 0.3333333333333333703, 0.3299404806269776169, 0.3333333333333333703, 0.3299404806269776169, 0.3333333333333333703, 0.3299404806269776169, 0.3333333333333333703, 0.3299404806269776169, 0.3333333333333333703, 0.3299404806269776169, 0.3333333333333333703, 0.3299404806269776169, 0.3333333333333333703, 0.3299404806269776169, 0.3333333333333333703, 0.3299404806269776169, 0.3333333333333333703, 0.3299404806269776169, 0.3333333333333333703, 0.3299404806269776169, 0.3333333333333333703, 0.3299404806269776169, 0.3333333333333333703, 0.3299404806269776169, 0.3333333333333333703, 0.3299404806269776169, 0.3333333333333333703, 0.3299404806269776169, 0.3333333333333333703, 0.3299404806269776169, 0.3333333333333333703, 0.3299404806269776169, 0.3333333333333333703, 0.3299404806269776169, 0.3333333333333333703, 0.3299404806269776169, 0.3333333333333333703, 0.3299404806269776169, 0.3333333333333333703, 0.3299404806269776169, 0.3333333333333333703, 0.3299404806269776169, 0.3333333333333333703, 0.3299404806269776169, 0.3333333333333333703, 0.3299404806269776169, 0.3333333333333333703, 0.3299404806269776169, 0.3333333333333333703, 0.3299404806269776169, 0.3333333333333333703, 0.3299404806269776169, 0.3333333333333333703, 0.3299404806269776169, 0.3333333333333333703, 0.3299404806269776169, 0.3333333333333333703, 0.3299404806269776169, 0.3333333333333333703, 0.3299404806269776169, 0.3333333333333333703, 0.3299404806269776169, 0.3333333333333333703, 0.3299404806269776169, 0.3333333333333333703, 0.3299404806269776169, 0.3333333333333333703, 0.3299404806269776169, 0.3333333333333333703, 0.3299404806269776169, 0.3333333333333333703, 0.3299404806269776169, 0.3333333333333333703, 0.3299404806269776169, 0.3333333333333333703, 0.3299404806269776169, 0.3333333333333333703, 0.3299404806269776169, 0.3333333333333333703, 0.3299404806269776169, 0.3333333333333333703, 0.3299404806269776169, 0.3333333333333333703, 0.3299404806269776169, 0.3333333333333333703, 0.3299404806269776169, 0.3333333333333333703, 0.3299404806269776169, 0.3333333333333333703, 0.3299404806269776169, 0.3333333333333333703, 0.3299404806269776169, 0.3333333333333333703, 0.3299404806269776169, 0.3333333333333333703, 0.3299404806269776169, 0.3333333333333333703, 0.3299404806269776169, 0.3333333333333333703, 0.3299404806269776169, 0.3333333333333333703, 0.3299404806269776169, 0.3333333333333333703, 0.3299404806269776169, 0.3333333333333333703, 0.3299404806269776169, 0.3333333333333333703, 0.3299404806269776169, 0.3333333333333333703, 0.3299404806269776169, 0.3333333333333333703, 0.3299404806269776169, 0.3333333333333333703, 0.3299404806269776169, 0.3333333333333333703, 0.3299404806269776169, 0.3333333333333333703, 0.3299404806269776169, 0.3333333333333333703, 0.3299404806269776169, 0.3333333333333333703, 0.3299404806269776169, 0.3333333333333333703, 0.3299404806269776169, 0.3333333333333333703, 0.3299404806269776169, 0.3333333333333333703, 0.3299404806269776169, 0.3333333333333333703, 0.3299404806269776169, 0.3333333333333333703, 0.3299404806269776169, 0.3333333333333333703, 0.3299404806269776169, 0.3333333333333333703, 0.3299404806269776169, 0.3333333333333333703, 0.3299404806269776169, 0.3333333333333333703, 0.3299404806269776169, 0.3333333333333333703, 0.3299404806269776169, 0.3333333333333333703, 0.3299404806269776169, 0.3333333333333333703, 0.3299404806269776169, 0.3333333333333333703, 0.3299404806269776169, 0.3333333333333333703, 0.3299404806269776169, 0.3333333333333333703, 0.3299404806269776169, 0.3333333333333333703, 0.3299404806269776169, 0.3333333333333333703, 0.3299404806269776169, 0.3333333333333333703, 0.3299404806269776169, 0.3333333333333333703, 0.3299404806269776169, 0.3333333333333333703, 0.3299404806269776169, 0.3333333333333333703, 0.3299404806269776169, 0.3333333333333333703, 0.3299404806269776169, 0.3333333333333333703, 0.3299404806269776169, 0.3333333333333333703, 0.3299404806269776169, 0.3333333333333333703, 0.3299404806269776169, 0.3333333333333333703, 0.3299404806269776169, 0.3333333333333333703, 0.3299404806269776169, 0.3333333333333333703, 0.3299404806269776169, 0.3333333333333333703, 0.3299404806269776169, 0.3333333333333333703, 0.3299404806269776169, 0.3333333333333333703, 0.3299404806269776169, 0.3333333333333333703, 0.3299404806269776169, 0.3333333333333333703, 0.3299404806269776169, 0.3333333333333333703, 0.3299404806269776169, 0.3333333333333333703, 0.3299404806269776169, 0.3333333333333333703, 0.3299404806269776169, 0.3333333333333333703, 0.3299404806269776169, 0.3333333333333333703, 0.3299404806269776169, 0.3333333333333333703, 0.3299404806269776169, 0.3333333333333333703, 0.3299404806269776169, 0.3333333333333333703, 0.3299404806269776169, 0.3333333333333333703, 0.3299404806269776169, 0.3333333333333333703, 0.3299404806269776169, 0.3333333333333333703, 0.3299404806269776169, 0.3333333333333333703, 0.3299404806269776169, 0.3333333333333333703, 0.3299404806269776169, 0.3333333333333333703, 0.3299404806269776169, 0.3333333333333333703, 0.3299404806269776169, 0.3333333333333333703, 0.3299404806269776169, 0.3333333333333333703, 0.3299404806269776169, 0.3333333333333333703, 0.3299404806269776169, 0.3333333333333333703, 0.3299404806269776169, 0.3333333333333333703, 0.3299404806269776169, 0.3333333333333333703, 0.3299404806269776169, 0.3333333333333333703, 0.3299404806269776169, 0.3333333333333333703, 0.3299404806269776169, 0.3333333333333333703, 0.3299404806269776169, 0.3333333333333333703, 0.3299404806269776169, 0.3333333333333333703, 0.3299404806269776169, 0.3333333333333333703, 0.3299404806269776169, 0.3333333333333333703, 0.3299404806269776169, 0.3333333333333333703, 0.3299404806269776169, 0.3333333333333333703, 0.3299404806269776169, 0.3333333333333333703, 0.3299404806269776169, 0.3333333333333333703, 0.3299404806269776169, 0.3333333333333333703, 0.3299404806269776169, 0.3333333333333333703, 0.3299404806269776169, 0.3333333333333333703, 0.3299404806269776169, 0.3333333333333333703, 0.3299404806269776169, 0.3333333333333333703, 0.3299404806269776169, 0.3333333333333333703, 0.3299404806269776169, 0.3333333333333333703, 0.3299404806269776169, 0.3333333333333333703, 0.3299404806269776169, 0.3333333333333333703, 0.3299404806269776169, 0.3333333333333333703, 0.3299404806269776169, 0.3333333333333333703, 0.3299404806269776169, 0.3333333333333333703, 0.3299404806269776169, 0.3333333333333333703, 0.3299404806269776169, 0.3333333333333333703, 0.3299404806269776169, 0.3333333333333333703, 0.3299404806269776169, 0.3333333333333333703, 0.3299404806269776169, 0.3333333333333333703, 0.3299404806269776169, 0.3333333333333333703, 0.3320603117974822438, 0.3317425830320511193),
 ( 0.3333333333333333703, 0.3299404806269776169, 0.3333333333333333703, 0.3299404806269776169, 0.3333333333333333703, 0.3299404806269776169, 0.3333333333333333703, 0.3299404806269776169, 0.3333333333333333703, 0.3299404806269776169, 0.3333333333333333703, 0.3299404806269776169, 0.3333333333333333703, 0.3299404806269776169, 0.3333333333333333703, 0.3299404806269776169, 0.3333333333333333703, 0.3299404806269776169, 0.3333333333333333703, 0.3299404806269776169, 0.3333333333333333703, 0.3299404806269776169, 0.3333333333333333703, 0.3299404806269776169, 0.3333333333333333703, 0.3299404806269776169, 0.3333333333333333703, 0.3299404806269776169, 0.3333333333333333703, 0.3299404806269776169, 0.3333333333333333703, 0.3299404806269776169, 0.3333333333333333703, 0.3299404806269776169, 0.3333333333333333703, 0.3299404806269776169, 0.3333333333333333703, 0.3299404806269776169, 0.3333333333333333703, 0.3299404806269776169, 0.3333333333333333703, 0.3299404806269776169, 0.3333333333333333703, 0.3299404806269776169, 0.3333333333333333703, 0.3299404806269776169, 0.3333333333333333703, 0.3299404806269776169, 0.3333333333333333703, 0.3299404806269776169, 0.3333333333333333703, 0.3299404806269776169, 0.3333333333333333703, 0.3299404806269776169, 0.3333333333333333703, 0.3299404806269776169, 0.3333333333333333703, 0.3299404806269776169, 0.3333333333333333703, 0.3299404806269776169, 0.3333333333333333703, 0.3299404806269776169, 0.3333333333333333703, 0.3299404806269776169, 0.3333333333333333703, 0.3299404806269776169, 0.3333333333333333703, 0.3299404806269776169, 0.3333333333333333703, 0.3299404806269776169, 0.3333333333333333703, 0.3299404806269776169, 0.3333333333333333703, 0.3299404806269776169, 0.3333333333333333703, 0.3299404806269776169, 0.3333333333333333703, 0.3299404806269776169, 0.3333333333333333703, 0.3299404806269776169, 0.3333333333333333703, 0.3299404806269776169, 0.3333333333333333703, 0.3299404806269776169, 0.3333333333333333703, 0.3299404806269776169, 0.3333333333333333703, 0.3299404806269776169, 0.3333333333333333703, 0.3299404806269776169, 0.3333333333333333703, 0.3299404806269776169, 0.3333333333333333703, 0.3299404806269776169, 0.3333333333333333703, 0.3299404806269776169, 0.3333333333333333703, 0.3299404806269776169, 0.3333333333333333703, 0.3299404806269776169, 0.3333333333333333703, 0.3299404806269776169, 0.3333333333333333703, 0.3299404806269776169, 0.3333333333333333703, 0.3299404806269776169, 0.3333333333333333703, 0.3299404806269776169, 0.3333333333333333703, 0.3299404806269776169, 0.3333333333333333703, 0.3299404806269776169, 0.3333333333333333703, 0.3299404806269776169, 0.3333333333333333703, 0.3299404806269776169, 0.3333333333333333703, 0.3299404806269776169, 0.3333333333333333703, 0.3299404806269776169, 0.3333333333333333703, 0.3299404806269776169, 0.3333333333333333703, 0.3299404806269776169, 0.3333333333333333703, 0.3299404806269776169, 0.3333333333333333703, 0.3299404806269776169, 0.3333333333333333703, 0.3299404806269776169, 0.3333333333333333703, 0.3299404806269776169, 0.3333333333333333703, 0.3299404806269776169, 0.3333333333333333703, 0.3299404806269776169, 0.3333333333333333703, 0.3299404806269776169, 0.3333333333333333703, 0.3299404806269776169, 0.3333333333333333703, 0.3299404806269776169, 0.3333333333333333703, 0.3299404806269776169, 0.3333333333333333703, 0.3299404806269776169, 0.3333333333333333703, 0.3299404806269776169, 0.3333333333333333703, 0.3299404806269776169, 0.3333333333333333703, 0.3299404806269776169, 0.3333333333333333703, 0.3299404806269776169, 0.3333333333333333703, 0.3299404806269776169, 0.3333333333333333703, 0.3299404806269776169, 0.3333333333333333703, 0.3299404806269776169, 0.3333333333333333703, 0.3299404806269776169, 0.3333333333333333703, 0.3299404806269776169, 0.3333333333333333703, 0.3299404806269776169, 0.3333333333333333703, 0.3299404806269776169, 0.3333333333333333703, 0.3299404806269776169, 0.3333333333333333703, 0.3299404806269776169, 0.3333333333333333703, 0.3299404806269776169, 0.3333333333333333703, 0.3299404806269776169, 0.3333333333333333703, 0.3299404806269776169, 0.3333333333333333703, 0.3299404806269776169, 0.3333333333333333703, 0.3299404806269776169, 0.3333333333333333703, 0.3299404806269776169, 0.3333333333333333703, 0.3299404806269776169, 0.3333333333333333703, 0.3299404806269776169, 0.3333333333333333703, 0.3299404806269776169, 0.3333333333333333703, 0.3299404806269776169, 0.3333333333333333703, 0.3299404806269776169, 0.3333333333333333703, 0.3299404806269776169, 0.3333333333333333703, 0.3299404806269776169, 0.3333333333333333703, 0.3299404806269776169, 0.3333333333333333703, 0.3299404806269776169, 0.3333333333333333703, 0.3299404806269776169, 0.3333333333333333703, 0.3299404806269776169, 0.3333333333333333703, 0.3299404806269776169, 0.3333333333333333703, 0.3299404806269776169, 0.3333333333333333703, 0.3299404806269776169, 0.3333333333333333703, 0.3299404806269776169, 0.3333333333333333703, 0.3299404806269776169, 0.3333333333333333703, 0.3299404806269776169, 0.3333333333333333703, 0.3299404806269776169, 0.3333333333333333703, 0.3299404806269776169, 0.3333333333333333703, 0.3299404806269776169, 0.3333333333333333703, 0.3299404806269776169, 0.3333333333333333703, 0.3299404806269776169, 0.3333333333333333703, 0.3299404806269776169, 0.3333333333333333703, 0.3299404806269776169, 0.3333333333333333703, 0.3299404806269776169, 0.3333333333333333703, 0.3299404806269776169, 0.3333333333333333703, 0.3299404806269776169, 0.3333333333333333703, 0.3299404806269776169, 0.3333333333333333703, 0.3299404806269776169, 0.3333333333333333703, 0.3299404806269776169, 0.3333333333333333703, 0.3299404806269776169, 0.3333333333333333703, 0.3299404806269776169, 0.3333333333333333703, 0.3299404806269776169, 0.3333333333333333703, 0.3299404806269776169, 0.3333333333333333703, 0.3299404806269776169, 0.3333333333333333703, 0.3299404806269776169, 0.3333333333333333703, 0.3299404806269776169, 0.3333333333333333703, 0.3299404806269776169, 0.3333333333333333703, 0.3299404806269776169, 0.3333333333333333703, 0.3299404806269776169, 0.3333333333333333703, 0.3299404806269776169, 0.3333333333333333703, 0.3299404806269776169, 0.3333333333333333703, 0.3299404806269776169, 0.3333333333333333703, 0.3299404806269776169, 0.3333333333333333703, 0.3299404806269776169, 0.3333333333333333703, 0.3299404806269776169, 0.3333333333333333703, 0.3299404806269776169, 0.3333333333333333703, 0.3299404806269776169, 0.3333333333333333703, 0.3299404806269776169, 0.3333333333333333703, 0.3299404806269776169, 0.3333333333333333703, 0.3299404806269776169, 0.3333333333333333703, 0.3299404806269776169, 0.3333333333333333703, 0.3299404806269776169, 0.3333333333333333703, 0.3299404806269776169, 0.3333333333333333703, 0.3299404806269776169, 0.3333333333333333703, 0.3299404806269776169, 0.3333333333333333703, 0.3299404806269776169, 0.3333333333333333703, 0.3299404806269776169, 0.3333333333333333703, 0.3299404806269776169, 0.3333333333333333703, 0.3299404806269776169, 0.3333333333333333703, 0.3299404806269776169, 0.3333333333333333703, 0.3299404806269776169, 0.3333333333333333703, 0.3299404806269776169, 0.3333333333333333703, 0.3299404806269776169, 0.3333333333333333703, 0.3299404806269776169, 0.3333333333333333703, 0.3299404806269776169, 0.3333333333333333703, 0.3299404806269776169, 0.3333333333333333703, 0.3299404806269776169, 0.3333333333333333703, 0.3299404806269776169, 0.3333333333333333703, 0.3299404806269776169, 0.3333333333333333703, 0.3299404806269776169, 0.3333333333333333703, 0.3299404806269776169, 0.3333333333333333703, 0.3299404806269776169, 0.3333333333333333703, 0.3299404806269776169, 0.3333333333333333703, 0.3299404806269776169, 0.3333333333333333703, 0.3299404806269776169, 0.3333333333333333703, 0.3299404806269776169, 0.3333333333333333703, 0.3299404806269776169, 0.3333333333333333703, 0.3299404806269776169, 0.3333333333333333703, 0.3299404806269776169, 0.3333333333333333703, 0.3299404806269776169, 0.3333333333333333703, 0.3299404806269776169, 0.3333333333333333703, 0.3299404806269776169, 0.3333333333333333703, 0.3299404806269776169, 0.3333333333333333703, 0.3299404806269776169, 0.3333333333333333703, 0.3299404806269776169, 0.3333333333333333703, 0.3299404806269776169, 0.3333333333333333703, 0.3299404806269776169, 0.3333333333333333703, 0.3299404806269776169, 0.3333333333333333703, 0.3299404806269776169, 0.3333333333333333703, 0.3299404806269776169, 0.3333333333333333703, 0.3299404806269776169, 0.3333333333333333703, 0.3299404806269776169, 0.3333333333333333703, 0.3299404806269776169, 0.3333333333333333703, 0.3299404806269776169, 0.3333333333333333703, 0.3299404806269776169, 0.3333333333333333703, 0.3299404806269776169, 0.3333333333333333703, 0.3299404806269776169, 0.3333333333333333703, 0.3299404806269776169, 0.3333333333333333703, 0.3299404806269776169, 0.3333333333333333703, 0.3299404806269776169, 0.3333333333333333703, 0.3299404806269776169, 0.3333333333333333703, 0.3299404806269776169, 0.3333333333333333703, 0.3299404806269776169, 0.3333333333333333703, 0.3299404806269776169, 0.3333333333333333703, 0.3299404806269776169, 0.3333333333333333703, 0.3299404806269776169, 0.3333333333333333703, 0.3299404806269776169, 0.3333333333333333703, 0.3299404806269776169, 0.3333333333333333703, 0.3299404806269776169, 0.3333333333333333703, 0.3299404806269776169, 0.3333333333333333703, 0.3299404806269776169, 0.3333333333333333703, 0.3299404806269776169, 0.3333333333333333703, 0.3299404806269776169, 0.3333333333333333703, 0.3299404806269776169, 0.3333333333333333703, 0.3299404806269776169, 0.3333333333333333703, 0.3299404806269776169, 0.3333333333333333703, 0.3299404806269776169, 0.3333333333333333703, 0.3299404806269776169, 0.3333333333333333703, 0.3299404806269776169, 0.3333333333333333703, 0.3299404806269776169, 0.3333333333333333703, 0.3299404806269776169, 0.3333333333333333703, 0.3299404806269776169, 0.3333333333333333703, 0.3299404806269776169, 0.3333333333333333703, 0.3299404806269776169, 0.3333333333333333703, 0.3299404806269776169, 0.3333333333333333703, 0.3299404806269776169, 0.3333333333333333703, 0.3299404806269776169, 0.3333333333333333703, 0.3299404806269776169, 0.3333333333333333703, 0.3299404806269776169, 0.3333333333333333703, 0.3299404806269776169, 0.3333333333333333703, 0.3299404806269776169, 0.3333333333333333703, 0.3299404806269776169, 0.3333333333333333703, 0.3299404806269776169, 0.3333333333333333703, 0.3299404806269776169, 0.3333333333333333703, 0.3299404806269776169, 0.3333333333333333703, 0.3299404806269776169, 0.3333333333333333703, 0.3299404806269776169, 0.3333333333333333703, 0.3299404806269776169, 0.3333333333333333703, 0.3299404806269776169, 0.3333333333333333703, 0.3299404806269776169, 0.3333333333333333703, 0.3299404806269776169, 0.3333333333333333703, 0.3299404806269776169, 0.3333333333333333703, 0.3299404806269776169, 0.3333333333333333703, 0.3299404806269776169, 0.3333333333333333703, 0.3299404806269776169, 0.3333333333333333703, 0.3299404806269776169, 0.3333333333333333703, 0.3299404806269776169, 0.3333333333333333703, 0.3299404806269776169, 0.3333333333333333703, 0.3299404806269776169, 0.3333333333333333703, 0.3299404806269776169, 0.3333333333333333703, 0.3299404806269776169, 0.3333333333333333703, 0.3299404806269776169, 0.3333333333333333703, 0.3299404806269776169, 0.3333333333333333703, 0.3299404806269776169, 0.3333333333333333703, 0.3299404806269776169, 0.3333333333333333703, 0.3299404806269776169, 0.3333333333333333703, 0.3299404806269776169, 0.3333333333333333703, 0.3299404806269776169, 0.3333333333333333703, 0.3299404806269776169, 0.3333333333333333703, 0.3299404806269776169, 0.3333333333333333703, 0.3299404806269776169, 0.3333333333333333703, 0.3299404806269776169, 0.3333333333333333703, 0.3299404806269776169, 0.3333333333333333703, 0.3299404806269776169, 0.3333333333333333703, 0.3299404806269776169, 0.3333333333333333703, 0.3299404806269776169, 0.3333333333333333703, 0.3299404806269776169, 0.3333333333333333703, 0.3299404806269776169, 0.3333333333333333703, 0.3299404806269776169, 0.3333333333333333703, 0.3299404806269776169, 0.3333333333333333703, 0.3299404806269776169, 0.3333333333333333703, 0.3299404806269776169, 0.3333333333333333703, 0.3299404806269776169, 0.3333333333333333703, 0.3299404806269776169, 0.3333333333333333703, 0.3299404806269776169, 0.3333333333333333703, 0.3299404806269776169, 0.3333333333333333703, 0.3299404806269776169, 0.3333333333333333703, 0.3299404806269776169, 0.3333333333333333703, 0.3299404806269776169, 0.3333333333333333703, 0.3299404806269776169, 0.3333333333333333703, 0.3299404806269776169, 0.3333333333333333703, 0.3299404806269776169, 0.3333333333333333703, 0.3299404806269776169, 0.3333333333333333703, 0.3299404806269776169, 0.3333333333333333703, 0.3299404806269776169, 0.3333333333333333703, 0.3299404806269776169, 0.3333333333333333703, 0.3299404806269776169, 0.3333333333333333703, 0.3299404806269776169, 0.3333333333333333703, 0.3299404806269776169, 0.3333333333333333703, 0.3299404806269776169, 0.3333333333333333703, 0.3299404806269776169, 0.3333333333333333703, 0.3299404806269776169, 0.3333333333333333703, 0.3299404806269776169, 0.3333333333333333703, 0.3299404806269776169, 0.3333333333333333703, 0.3299404806269776169, 0.3333333333333333703, 0.3299404806269776169, 0.3333333333333333703, 0.3299404806269776169, 0.3333333333333333703, 0.3299404806269776169, 0.3333333333333333703, 0.3299404806269776169, 0.3333333333333333703, 0.3299404806269776169, 0.3333333333333333703, 0.3299404806269776169, 0.3333333333333333703, 0.3299404806269776169, 0.3333333333333333703, 0.3299404806269776169, 0.3333333333333333703, 0.3299404806269776169, 0.3333333333333333703, 0.3299404806269776169, 0.3333333333333333703, 0.3299404806269776169, 0.3333333333333333703, 0.3299404806269776169, 0.3333333333333333703, 0.3299404806269776169, 0.3333333333333333703, 0.3299404806269776169, 0.3333333333333333703, 0.3299404806269776169, 0.3333333333333333703, 0.3299404806269776169, 0.3333333333333333703, 0.3299404806269776169, 0.3333333333333333703, 0.3299404806269776169, 0.3333333333333333703, 0.3299404806269776169, 0.3333333333333333703, 0.3299404806269776169, 0.3333333333333333703, 0.3299404806269776169, 0.3333333333333333703, 0.3299404806269776169, 0.3333333333333333703, 0.3299404806269776169, 0.3333333333333333703, 0.3299404806269776169, 0.3333333333333333703, 0.3299404806269776169, 0.3333333333333333703, 0.3299404806269776169, 0.3333333333333333703, 0.3299404806269776169, 0.3333333333333333703, 0.3299404806269776169, 0.3333333333333333703, 0.3299404806269776169, 0.3333333333333333703, 0.3299404806269776169, 0.3333333333333333703, 0.3299404806269776169, 0.3333333333333333703, 0.3299404806269776169, 0.3333333333333333703, 0.3299404806269776169, 0.3333333333333333703, 0.3299404806269776169, 0.3333333333333333703, 0.3299404806269776169, 0.3333333333333333703, 0.3299404806269776169, 0.3333333333333333703, 0.3299404806269776169, 0.3333333333333333703, 0.3299404806269776169, 0.3333333333333333703, 0.3299404806269776169, 0.3333333333333333703, 0.3299404806269776169, 0.3333333333333333703, 0.3299404806269776169, 0.3333333333333333703, 0.3299404806269776169, 0.3333333333333333703, 0.3299404806269776169, 0.3333333333333333703, 0.3299404806269776169, 0.3333333333333333703, 0.3299404806269776169, 0.3333333333333333703, 0.3299404806269776169, 0.3333333333333333703, 0.3299404806269776169, 0.3333333333333333703, 0.3299404806269776169, 0.3333333333333333703, 0.3299404806269776169, 0.3333333333333333703, 0.3299404806269776169, 0.3333333333333333703, 0.3299404806269776169, 0.3333333333333333703, 0.3299404806269776169, 0.3333333333333333703, 0.3299404806269776169, 0.3333333333333333703, 0.3299404806269776169, 0.3333333333333333703, 0.3299404806269776169, 0.3333333333333333703, 0.3299404806269776169, 0.3333333333333333703, 0.3299404806269776169, 0.3333333333333333703, 0.3299404806269776169, 0.3333333333333333703, 0.3299404806269776169, 0.3333333333333333703, 0.3299404806269776169, 0.3333333333333333703, 0.3299404806269776169, 0.3333333333333333703, 0.3299404806269776169, 0.3333333333333333703, 0.3299404806269776169, 0.3333333333333333703, 0.3299404806269776169, 0.3333333333333333703, 0.3299404806269776169, 0.3333333333333333703, 0.3299404806269776169, 0.3333333333333333703, 0.3299404806269776169, 0.3333333333333333703, 0.3299404806269776169, 0.3333333333333333703, 0.3299404806269776169, 0.3333333333333333703, 0.3299404806269776169, 0.3333333333333333703, 0.3299404806269776169, 0.3333333333333333703, 0.3299404806269776169, 0.3333333333333333703, 0.3299404806269776169, 0.3333333333333333703, 0.3299404806269776169, 0.3333333333333333703, 0.3299404806269776169, 0.3333333333333333703, 0.3299404806269776169, 0.3333333333333333703, 0.3299404806269776169, 0.3333333333333333703, 0.3299404806269776169, 0.3333333333333333703, 0.3299404806269776169, 0.3333333333333333703, 0.3299404806269776169, 0.3333333333333333703, 0.3299404806269776169, 0.3333333333333333703, 0.3299404806269776169, 0.3333333333333333703, 0.3299404806269776169, 0.3333333333333333703, 0.3299404806269776169, 0.3333333333333333703, 0.3299404806269776169, 0.3333333333333333703, 0.3299404806269776169, 0.3333333333333333703, 0.3299404806269776169, 0.3333333333333333703, 0.3299404806269776169, 0.3333333333333333703, 0.3299404806269776169, 0.3333333333333333703, 0.3299404806269776169, 0.3333333333333333703, 0.3299404806269776169, 0.3333333333333333703, 0.3299404806269776169, 0.3333333333333333703, 0.3299404806269776169, 0.3333333333333333703, 0.3299404806269776169, 0.3333333333333333703, 0.3299404806269776169, 0.3333333333333333703, 0.3299404806269776169, 0.3333333333333333703, 0.3299404806269776169, 0.3333333333333333703, 0.3299404806269776169, 0.3333333333333333703, 0.3299404806269776169, 0.3333333333333333703, 0.3299404806269776169, 0.3333333333333333703, 0.3299404806269776169, 0.3333333333333333703, 0.3299404806269776169, 0.3333333333333333703, 0.3299404806269776169, 0.3333333333333333703, 0.3299404806269776169, 0.3333333333333333703, 0.3299404806269776169, 0.3333333333333333703, 0.3299404806269776169, 0.3333333333333333703, 0.3299404806269776169, 0.3333333333333333703, 0.3299404806269776169, 0.3333333333333333703, 0.3299404806269776169, 0.3333333333333333703, 0.3299404806269776169, 0.3333333333333333703, 0.3299404806269776169, 0.3333333333333333703, 0.3299404806269776169, 0.3333333333333333703, 0.3299404806269776169, 0.3333333333333333703, 0.3299404806269776169, 0.3333333333333333703, 0.3299404806269776169, 0.3333333333333333703, 0.3299404806269776169, 0.3333333333333333703, 0.3299404806269776169, 0.3333333333333333703, 0.3299404806269776169, 0.3333333333333333703, 0.3299404806269776169, 0.3333333333333333703, 0.3299404806269776169, 0.3333333333333333703, 0.3299404806269776169, 0.3333333333333333703, 0.3299404806269776169, 0.3333333333333333703, 0.3299404806269776169, 0.3333333333333333703, 0.3299404806269776169, 0.3333333333333333703, 0.3299404806269776169, 0.3333333333333333703, 0.3299404806269776169, 0.3333333333333333703, 0.3299404806269776169, 0.3333333333333333703, 0.3299404806269776169, 0.3333333333333333703, 0.3299404806269776169, 0.3333333333333333703, 0.3299404806269776169, 0.3333333333333333703, 0.3299404806269776169, 0.3333333333333333703, 0.3299404806269776169, 0.3333333333333333703, 0.3299404806269776169, 0.3333333333333333703, 0.3299404806269776169, 0.3333333333333333703, 0.3299404806269776169, 0.3333333333333333703, 0.3299404806269776169, 0.3333333333333333703, 0.3299404806269776169, 0.3333333333333333703, 0.3299404806269776169, 0.3333333333333333703, 0.3299404806269776169, 0.3333333333333333703, 0.3299404806269776169, 0.3333333333333333703, 0.3299404806269776169, 0.3333333333333333703, 0.3299404806269776169, 0.3333333333333333703, 0.3320603117974822438, 0.3317425830320511193),
 ( 1.000000000000000000, 0.9898214418809326842, 1.000000000000000000, 0.9898214418809326842, 1.000000000000000000, 0.9898214418809326842, 1.000000000000000000, 0.9898214418809326842, 1.000000000000000000, 0.9898214418809326842, 1.000000000000000000, 0.9898214418809326842, 1.000000000000000000, 0.9898214418809326842, 1.000000000000000000, 0.9898214418809326842, 1.000000000000000000, 0.9898214418809326842, 1.000000000000000000, 0.9898214418809326842, 1.000000000000000000, 0.9898214418809326842, 1.000000000000000000, 0.9898214418809326842, 1.000000000000000000, 0.9898214418809326842, 1.000000000000000000, 0.9898214418809326842, 1.000000000000000000, 0.9898214418809326842, 1.000000000000000000, 0.9898214418809326842, 1.000000000000000000, 0.9898214418809326842, 1.000000000000000000, 0.9898214418809326842, 1.000000000000000000, 0.9898214418809326842, 1.000000000000000000, 0.9898214418809326842, 1.000000000000000000, 0.9898214418809326842, 1.000000000000000000, 0.9898214418809326842, 1.000000000000000000, 0.9898214418809326842, 1.000000000000000000, 0.9898214418809326842, 1.000000000000000000, 0.9898214418809326842, 1.000000000000000000, 0.9898214418809326842, 1.000000000000000000, 0.9898214418809326842, 1.000000000000000000, 0.9898214418809326842, 1.000000000000000000, 0.9898214418809326842, 1.000000000000000000, 0.9898214418809326842, 1.000000000000000000, 0.9898214418809326842, 1.000000000000000000, 0.9898214418809326842, 1.000000000000000000, 0.9898214418809326842, 1.000000000000000000, 0.9898214418809326842, 1.000000000000000000, 0.9898214418809326842, 1.000000000000000000, 0.9898214418809326842, 1.000000000000000000, 0.9898214418809326842, 1.000000000000000000, 0.9898214418809326842, 1.000000000000000000, 0.9898214418809326842, 1.000000000000000000, 0.9898214418809326842, 1.000000000000000000, 0.9898214418809326842, 1.000000000000000000, 0.9898214418809326842, 1.000000000000000000, 0.9898214418809326842, 1.000000000000000000, 0.9898214418809326842, 1.000000000000000000, 0.9898214418809326842, 1.000000000000000000, 0.9898214418809326842, 1.000000000000000000, 0.9898214418809326842, 1.000000000000000000, 0.9898214418809326842, 1.000000000000000000, 0.9898214418809326842, 1.000000000000000000, 0.9898214418809326842, 1.000000000000000000, 0.9898214418809326842, 1.000000000000000000, 0.9898214418809326842, 1.000000000000000000, 0.9898214418809326842, 1.000000000000000000, 0.9898214418809326842, 1.000000000000000000, 0.9898214418809326842, 1.000000000000000000, 0.9898214418809326842, 1.000000000000000000, 0.9898214418809326842, 1.000000000000000000, 0.9898214418809326842, 1.000000000000000000, 0.9898214418809326842, 1.000000000000000000, 0.9898214418809326842, 1.000000000000000000, 0.9898214418809326842, 1.000000000000000000, 0.9898214418809326842, 1.000000000000000000, 0.9898214418809326842, 1.000000000000000000, 0.9898214418809326842, 1.000000000000000000, 0.9898214418809326842, 1.000000000000000000, 0.9898214418809326842, 1.000000000000000000, 0.9898214418809326842, 1.000000000000000000, 0.9898214418809326842, 1.000000000000000000, 0.9898214418809326842, 1.000000000000000000, 0.9898214418809326842, 1.000000000000000000, 0.9898214418809326842, 1.000000000000000000, 0.9898214418809326842, 1.000000000000000000, 0.9898214418809326842, 1.000000000000000000, 0.9898214418809326842, 1.000000000000000000, 0.9898214418809326842, 1.000000000000000000, 0.9898214418809326842, 1.000000000000000000, 0.9898214418809326842, 1.000000000000000000, 0.9898214418809326842, 1.000000000000000000, 0.9898214418809326842, 1.000000000000000000, 0.9898214418809326842, 1.000000000000000000, 0.9898214418809326842, 1.000000000000000000, 0.9898214418809326842, 1.000000000000000000, 0.9898214418809326842, 1.000000000000000000, 0.9898214418809326842, 1.000000000000000000, 0.9898214418809326842, 1.000000000000000000, 0.9898214418809326842, 1.000000000000000000, 0.9898214418809326842, 1.000000000000000000, 0.9898214418809326842, 1.000000000000000000, 0.9898214418809326842, 1.000000000000000000, 0.9898214418809326842, 1.000000000000000000, 0.9898214418809326842, 1.000000000000000000, 0.9898214418809326842, 1.000000000000000000, 0.9898214418809326842, 1.000000000000000000, 0.9898214418809326842, 1.000000000000000000, 0.9898214418809326842, 1.000000000000000000, 0.9898214418809326842, 1.000000000000000000, 0.9898214418809326842, 1.000000000000000000, 0.9898214418809326842, 1.000000000000000000, 0.9898214418809326842, 1.000000000000000000, 0.9898214418809326842, 1.000000000000000000, 0.9898214418809326842, 1.000000000000000000, 0.9898214418809326842, 1.000000000000000000, 0.9898214418809326842, 1.000000000000000000, 0.9898214418809326842, 1.000000000000000000, 0.9898214418809326842, 1.000000000000000000, 0.9898214418809326842, 1.000000000000000000, 0.9898214418809326842, 1.000000000000000000, 0.9898214418809326842, 1.000000000000000000, 0.9898214418809326842, 1.000000000000000000, 0.9898214418809326842, 1.000000000000000000, 0.9898214418809326842, 1.000000000000000000, 0.9898214418809326842, 1.000000000000000000, 0.9898214418809326842, 1.000000000000000000, 0.9898214418809326842, 1.000000000000000000, 0.9898214418809326842, 1.000000000000000000, 0.9898214418809326842, 1.000000000000000000, 0.9898214418809326842, 1.000000000000000000, 0.9898214418809326842, 1.000000000000000000, 0.9898214418809326842, 1.000000000000000000, 0.9898214418809326842, 1.000000000000000000, 0.9898214418809326842, 1.000000000000000000, 0.9898214418809326842, 1.000000000000000000, 0.9898214418809326842, 1.000000000000000000, 0.9898214418809326842, 1.000000000000000000, 0.9898214418809326842, 1.000000000000000000, 0.9898214418809326842, 1.000000000000000000, 0.9898214418809326842, 1.000000000000000000, 0.9898214418809326842, 1.000000000000000000, 0.9898214418809326842, 1.000000000000000000, 0.9898214418809326842, 1.000000000000000000, 0.9898214418809326842, 1.000000000000000000, 0.9898214418809326842, 1.000000000000000000, 0.9898214418809326842, 1.000000000000000000, 0.9898214418809326842, 1.000000000000000000, 0.9898214418809326842, 1.000000000000000000, 0.9898214418809326842, 1.000000000000000000, 0.9898214418809326842, 1.000000000000000000, 0.9898214418809326842, 1.000000000000000000, 0.9898214418809326842, 1.000000000000000000, 0.9898214418809326842, 1.000000000000000000, 0.9898214418809326842, 1.000000000000000000, 0.9898214418809326842, 1.000000000000000000, 0.9898214418809326842, 1.000000000000000000, 0.9898214418809326842, 1.000000000000000000, 0.9898214418809326842, 1.000000000000000000, 0.9898214418809326842, 1.000000000000000000, 0.9898214418809326842, 1.000000000000000000, 0.9898214418809326842, 1.000000000000000000, 0.9898214418809326842, 1.000000000000000000, 0.9898214418809326842, 1.000000000000000000, 0.9898214418809326842, 1.000000000000000000, 0.9898214418809326842, 1.000000000000000000, 0.9898214418809326842, 1.000000000000000000, 0.9898214418809326842, 1.000000000000000000, 0.9898214418809326842, 1.000000000000000000, 0.9898214418809326842, 1.000000000000000000, 0.9898214418809326842, 1.000000000000000000, 0.9898214418809326842, 1.000000000000000000, 0.9898214418809326842, 1.000000000000000000, 0.9898214418809326842, 1.000000000000000000, 0.9898214418809326842, 1.000000000000000000, 0.9898214418809326842, 1.000000000000000000, 0.9898214418809326842, 1.000000000000000000, 0.9898214418809326842, 1.000000000000000000, 0.9898214418809326842, 1.000000000000000000, 0.9898214418809326842, 1.000000000000000000, 0.9898214418809326842, 1.000000000000000000, 0.9898214418809326842, 1.000000000000000000, 0.9898214418809326842, 1.000000000000000000, 0.9898214418809326842, 1.000000000000000000, 0.9898214418809326842, 1.000000000000000000, 0.9898214418809326842, 1.000000000000000000, 0.9898214418809326842, 1.000000000000000000, 0.9898214418809326842, 1.000000000000000000, 0.9898214418809326842, 1.000000000000000000, 0.9898214418809326842, 1.000000000000000000, 0.9898214418809326842, 1.000000000000000000, 0.9898214418809326842, 1.000000000000000000, 0.9898214418809326842, 1.000000000000000000, 0.9898214418809326842, 1.000000000000000000, 0.9898214418809326842, 1.000000000000000000, 0.9898214418809326842, 1.000000000000000000, 0.9898214418809326842, 1.000000000000000000, 0.9898214418809326842, 1.000000000000000000, 0.9898214418809326842, 1.000000000000000000, 0.9898214418809326842, 1.000000000000000000, 0.9898214418809326842, 1.000000000000000000, 0.9898214418809326842, 1.000000000000000000, 0.9898214418809326842, 1.000000000000000000, 0.9898214418809326842, 1.000000000000000000, 0.9898214418809326842, 1.000000000000000000, 0.9898214418809326842, 1.000000000000000000, 0.9898214418809326842, 1.000000000000000000, 0.9898214418809326842, 1.000000000000000000, 0.9898214418809326842, 1.000000000000000000, 0.9898214418809326842, 1.000000000000000000, 0.9898214418809326842, 1.000000000000000000, 0.9898214418809326842, 1.000000000000000000, 0.9898214418809326842, 1.000000000000000000, 0.9898214418809326842, 1.000000000000000000, 0.9898214418809326842, 1.000000000000000000, 0.9898214418809326842, 1.000000000000000000, 0.9898214418809326842, 1.000000000000000000, 0.9898214418809326842, 1.000000000000000000, 0.9898214418809326842, 1.000000000000000000, 0.9898214418809326842, 1.000000000000000000, 0.9898214418809326842, 1.000000000000000000, 0.9898214418809326842, 1.000000000000000000, 0.9898214418809326842, 1.000000000000000000, 0.9898214418809326842, 1.000000000000000000, 0.9898214418809326842, 1.000000000000000000, 0.9898214418809326842, 1.000000000000000000, 0.9898214418809326842, 1.000000000000000000, 0.9898214418809326842, 1.000000000000000000, 0.9898214418809326842, 1.000000000000000000, 0.9898214418809326842, 1.000000000000000000, 0.9898214418809326842, 1.000000000000000000, 0.9898214418809326842, 1.000000000000000000, 0.9898214418809326842, 1.000000000000000000, 0.9898214418809326842, 1.000000000000000000, 0.9898214418809326842, 1.000000000000000000, 0.9898214418809326842, 1.000000000000000000, 0.9898214418809326842, 1.000000000000000000, 0.9898214418809326842, 1.000000000000000000, 0.9898214418809326842, 1.000000000000000000, 0.9898214418809326842, 1.000000000000000000, 0.9898214418809326842, 1.000000000000000000, 0.9898214418809326842, 1.000000000000000000, 0.9898214418809326842, 1.000000000000000000, 0.9898214418809326842, 1.000000000000000000, 0.9898214418809326842, 1.000000000000000000, 0.9898214418809326842, 1.000000000000000000, 0.9898214418809326842, 1.000000000000000000, 0.9898214418809326842, 1.000000000000000000, 0.9898214418809326842, 1.000000000000000000, 0.9898214418809326842, 1.000000000000000000, 0.9898214418809326842, 1.000000000000000000, 0.9898214418809326842, 1.000000000000000000, 0.9898214418809326842, 1.000000000000000000, 0.9898214418809326842, 1.000000000000000000, 0.9898214418809326842, 1.000000000000000000, 0.9898214418809326842, 1.000000000000000000, 0.9898214418809326842, 1.000000000000000000, 0.9898214418809326842, 1.000000000000000000, 0.9898214418809326842, 1.000000000000000000, 0.9898214418809326842, 1.000000000000000000, 0.9898214418809326842, 1.000000000000000000, 0.9898214418809326842, 1.000000000000000000, 0.9898214418809326842, 1.000000000000000000, 0.9898214418809326842, 1.000000000000000000, 0.9898214418809326842, 1.000000000000000000, 0.9898214418809326842, 1.000000000000000000, 0.9898214418809326842, 1.000000000000000000, 0.9898214418809326842, 1.000000000000000000, 0.9898214418809326842, 1.000000000000000000, 0.9898214418809326842, 1.000000000000000000, 0.9898214418809326842, 1.000000000000000000, 0.9898214418809326842, 1.000000000000000000, 0.9898214418809326842, 1.000000000000000000, 0.9898214418809326842, 1.000000000000000000, 0.9898214418809326842, 1.000000000000000000, 0.9898214418809326842, 1.000000000000000000, 0.9898214418809326842, 1.000000000000000000, 0.9898214418809326842, 1.000000000000000000, 0.9898214418809326842, 1.000000000000000000, 0.9898214418809326842, 1.000000000000000000, 0.9898214418809326842, 1.000000000000000000, 0.9898214418809326842, 1.000000000000000000, 0.9898214418809326842, 1.000000000000000000, 0.9898214418809326842, 1.000000000000000000, 0.9898214418809326842, 1.000000000000000000, 0.9898214418809326842, 1.000000000000000000, 0.9898214418809326842, 1.000000000000000000, 0.9898214418809326842, 1.000000000000000000, 0.9898214418809326842, 1.000000000000000000, 0.9898214418809326842, 1.000000000000000000, 0.9898214418809326842, 1.000000000000000000, 0.9898214418809326842, 1.000000000000000000, 0.9898214418809326842, 1.000000000000000000, 0.9898214418809326842, 1.000000000000000000, 0.9898214418809326842, 1.000000000000000000, 0.9898214418809326842, 1.000000000000000000, 0.9898214418809326842, 1.000000000000000000, 0.9898214418809326842, 1.000000000000000000, 0.9898214418809326842, 1.000000000000000000, 0.9898214418809326842, 1.000000000000000000, 0.9898214418809326842, 1.000000000000000000, 0.9898214418809326842, 1.000000000000000000, 0.9898214418809326842, 1.000000000000000000, 0.9898214418809326842, 1.000000000000000000, 0.9898214418809326842, 1.000000000000000000, 0.9898214418809326842, 1.000000000000000000, 0.9898214418809326842, 1.000000000000000000, 0.9898214418809326842, 1.000000000000000000, 0.9898214418809326842, 1.000000000000000000, 0.9898214418809326842, 1.000000000000000000, 0.9898214418809326842, 1.000000000000000000, 0.9898214418809326842, 1.000000000000000000, 0.9898214418809326842, 1.000000000000000000, 0.9898214418809326842, 1.000000000000000000, 0.9898214418809326842, 1.000000000000000000, 0.9898214418809326842, 1.000000000000000000, 0.9898214418809326842, 1.000000000000000000, 0.9898214418809326842, 1.000000000000000000, 0.9898214418809326842, 1.000000000000000000, 0.9898214418809326842, 1.000000000000000000, 0.9898214418809326842, 1.000000000000000000, 0.9898214418809326842, 1.000000000000000000, 0.9898214418809326842, 1.000000000000000000, 0.9898214418809326842, 1.000000000000000000, 0.9898214418809326842, 1.000000000000000000, 0.9898214418809326842, 1.000000000000000000, 0.9898214418809326842, 1.000000000000000000, 0.9898214418809326842, 1.000000000000000000, 0.9898214418809326842, 1.000000000000000000, 0.9898214418809326842, 1.000000000000000000, 0.9898214418809326842, 1.000000000000000000, 0.9898214418809326842, 1.000000000000000000, 0.9898214418809326842, 1.000000000000000000, 0.9898214418809326842, 1.000000000000000000, 0.9898214418809326842, 1.000000000000000000, 0.9898214418809326842, 1.000000000000000000, 0.9898214418809326842, 1.000000000000000000, 0.9898214418809326842, 1.000000000000000000, 0.9898214418809326842, 1.000000000000000000, 0.9898214418809326842, 1.000000000000000000, 0.9898214418809326842, 1.000000000000000000, 0.9898214418809326842, 1.000000000000000000, 0.9898214418809326842, 1.000000000000000000, 0.9898214418809326842, 1.000000000000000000, 0.9898214418809326842, 1.000000000000000000, 0.9898214418809326842, 1.000000000000000000, 0.9898214418809326842, 1.000000000000000000, 0.9898214418809326842, 1.000000000000000000, 0.9898214418809326842, 1.000000000000000000, 0.9898214418809326842, 1.000000000000000000, 0.9898214418809326842, 1.000000000000000000, 0.9898214418809326842, 1.000000000000000000, 0.9898214418809326842, 1.000000000000000000, 0.9898214418809326842, 1.000000000000000000, 0.9898214418809326842, 1.000000000000000000, 0.9898214418809326842, 1.000000000000000000, 0.9898214418809326842, 1.000000000000000000, 0.9898214418809326842, 1.000000000000000000, 0.9898214418809326842, 1.000000000000000000, 0.9898214418809326842, 1.000000000000000000, 0.9898214418809326842, 1.000000000000000000, 0.9898214418809326842, 1.000000000000000000, 0.9898214418809326842, 1.000000000000000000, 0.9898214418809326842, 1.000000000000000000, 0.9898214418809326842, 1.000000000000000000, 0.9898214418809326842, 1.000000000000000000, 0.9898214418809326842, 1.000000000000000000, 0.9898214418809326842, 1.000000000000000000, 0.9898214418809326842, 1.000000000000000000, 0.9898214418809326842, 1.000000000000000000, 0.9898214418809326842, 1.000000000000000000, 0.9898214418809326842, 1.000000000000000000, 0.9898214418809326842, 1.000000000000000000, 0.9898214418809326842, 1.000000000000000000, 0.9898214418809326842, 1.000000000000000000, 0.9898214418809326842, 1.000000000000000000, 0.9898214418809326842, 1.000000000000000000, 0.9898214418809326842, 1.000000000000000000, 0.9898214418809326842, 1.000000000000000000, 0.9898214418809326842, 1.000000000000000000, 0.9898214418809326842, 1.000000000000000000, 0.9898214418809326842, 1.000000000000000000, 0.9898214418809326842, 1.000000000000000000, 0.9898214418809326842, 1.000000000000000000, 0.9898214418809326842, 1.000000000000000000, 0.9898214418809326842, 1.000000000000000000, 0.9898214418809326842, 1.000000000000000000, 0.9898214418809326842, 1.000000000000000000, 0.9898214418809326842, 1.000000000000000000, 0.9898214418809326842, 1.000000000000000000, 0.9898214418809326842, 1.000000000000000000, 0.9898214418809326842, 1.000000000000000000, 0.9898214418809326842, 1.000000000000000000, 0.9898214418809326842, 1.000000000000000000, 0.9898214418809326842, 1.000000000000000000, 0.9898214418809326842, 1.000000000000000000, 0.9898214418809326842, 1.000000000000000000, 0.9898214418809326842, 1.000000000000000000, 0.9898214418809326842, 1.000000000000000000, 0.9898214418809326842, 1.000000000000000000, 0.9898214418809326842, 1.000000000000000000, 0.9898214418809326842, 1.000000000000000000, 0.9898214418809326842, 1.000000000000000000, 0.9898214418809326842, 1.000000000000000000, 0.9898214418809326842, 1.000000000000000000, 0.9898214418809326842, 1.000000000000000000, 0.9898214418809326842, 1.000000000000000000, 0.9898214418809326842, 1.000000000000000000, 0.9898214418809326842, 1.000000000000000000, 0.9898214418809326842, 1.000000000000000000, 0.9898214418809326842, 1.000000000000000000, 0.9898214418809326842, 1.000000000000000000, 0.9898214418809326842, 1.000000000000000000, 0.9898214418809326842, 1.000000000000000000, 0.9898214418809326842, 1.000000000000000000, 0.9898214418809326842, 1.000000000000000000, 0.9898214418809326842, 1.000000000000000000, 0.9898214418809326842, 1.000000000000000000, 0.9898214418809326842, 1.000000000000000000, 0.9898214418809326842, 1.000000000000000000, 0.9898214418809326842, 1.000000000000000000, 0.9898214418809326842, 1.000000000000000000, 0.9898214418809326842, 1.000000000000000000, 0.9898214418809326842, 1.000000000000000000, 0.9898214418809326842, 1.000000000000000000, 0.9898214418809326842, 1.000000000000000000, 0.9898214418809326842, 1.000000000000000000, 0.9898214418809326842, 1.000000000000000000, 0.9898214418809326842, 1.000000000000000000, 0.9898214418809326842, 1.000000000000000000, 0.9898214418809326842, 1.000000000000000000, 0.9898214418809326842, 1.000000000000000000, 0.9898214418809326842, 1.000000000000000000, 0.9898214418809326842, 1.000000000000000000, 0.9898214418809326842, 1.000000000000000000, 0.9898214418809326842, 1.000000000000000000, 0.9898214418809326842, 1.000000000000000000, 0.9898214418809326842, 1.000000000000000000, 0.9898214418809326842, 1.000000000000000000, 0.9898214418809326842, 1.000000000000000000, 0.9898214418809326842, 1.000000000000000000, 0.9898214418809326842, 1.000000000000000000, 0.9898214418809326842, 1.000000000000000000, 0.9898214418809326842, 1.000000000000000000, 0.9961809353924466759, 0.9952277490961531914) ) ) 
 REPRESENTATION_ITEM ( '' )  SURFACE ( )  );
#43036=CARTESIAN_POINT ( 'NONE',  ( 784.1219089521767955, -141.2817908451530400, -315.0488828828318333 ) ) ;
#43040=CARTESIAN_POINT ( 'NONE',  ( 803.8556311672234642, -9.623778108051251223, -365.6418435158340117 ) ) ;
#43041=CARTESIAN_POINT ( 'NONE',  ( 767.6429770376291799, -345.1800572038739574, -306.8695393053162093 ) ) ;
#43042=CARTESIAN_POINT ( 'NONE',  ( 787.4999999999992042, -512.9681489794448908, -339.9999999999999432 ) ) ;
#43047=CARTESIAN_POINT ( 'NONE',  ( 764.3348316497523456, -190.7146871989597798, -308.6759233522265617 ) ) ;
#43049=CARTESIAN_POINT ( 'NONE',  ( 810.1134526219336749, -440.5328690171407970, -357.8822607201570349 ) ) ;
#43055=CARTESIAN_POINT ( 'NONE',  ( 789.9200121543843807, 22.01258552831228599, -317.0176451133914384 ) ) ;
#43062=CARTESIAN_POINT ( 'NONE',  ( 790.8726784830453198, -298.7146871989593251, -362.5472867521010585 ) ) ;
#43064=CARTESIAN_POINT ( 'NONE',  ( 783.7566961878529810, -288.8965053807775121, -305.1792804349288417 ) ) ;
#43065=CARTESIAN_POINT ( 'NONE',  ( 779.9999999999992042, 166.4563064324884465, -339.9999999999999432 ) ) ;
#43069=CARTESIAN_POINT ( 'NONE',  ( 773.3843516231979720, -85.44195992623282621, -364.4086373105754433 ) ) ;
#43071=CARTESIAN_POINT ( 'NONE',  ( 805.0032342141412300, -133.5436935675110135, -314.9967657858571783 ) ) ;
#43074=CARTESIAN_POINT ( 'NONE',  ( 797.8594530101009923, -157.5436935675109282, -322.1405469898982119 ) ) ;
#43077=CARTESIAN_POINT ( 'NONE',  ( 799.2566176426618085, -408.0090635724249069, -324.0069404352559559 ) ) ;
#43085=ORIENTED_EDGE ( 'NONE', *, *, #21300, .F. ) ;
#43086=CARTESIAN_POINT ( 'NONE',  ( 763.8424801807145741, -402.0090635724250205, -320.5453621957614700 ) ) ;
#43088=CARTESIAN_POINT ( 'NONE',  ( 764.1737431748507561, -202.3726999360618777, -371.6461892240376415 ) ) ;
#43093=CARTESIAN_POINT ( 'NONE',  ( 757.2208543904082489, -328.7146871989592682, -350.9844846989624330 ) ) ;
#43095=CARTESIAN_POINT ( 'NONE',  ( 746.4236121716829757, -183.8272453906074020, -328.8385539511384650 ) ) ;
#43099=CARTESIAN_POINT ( 'NONE',  ( 811.0346526505617248, -254.6346026584197091, -323.0537975583478101 ) ) ;
#43101=CARTESIAN_POINT ( 'NONE',  ( 802.1676090361156639, -14.63460265842049424, -327.8955696845344505 ) ) ;
#43102=EDGE_CURVE ( 'NONE', #24267, #25862, #37752, .T. ) ;
#43105=CARTESIAN_POINT ( 'NONE',  ( 776.2433038121456548, -84.89650538077830788, -374.8207195650711014 ) ) ;
#43107=CARTESIAN_POINT ( 'NONE',  ( 782.4968714119720516, -346.8164208402376971, -305.0891759886411023 ) ) ;
#43115=CARTESIAN_POINT ( 'NONE',  ( 771.2368401574024119, -421.4419599262317888, -374.2805881961240857 ) ) ;
#43116=CARTESIAN_POINT ( 'NONE',  ( 814.8207195650702488, -2.190881754244347945, -336.2433038121456548 ) ) ;
#43120=CARTESIAN_POINT ( 'NONE',  ( 784.0799538623451781, -179.8055962898688733, -364.6971507214555572 ) ) ;
#43122=CARTESIAN_POINT ( 'NONE',  ( 814.8230680027162407, -197.8055962898688733, -333.7305795820267917 ) ) ;
#43128=CARTESIAN_POINT ( 'NONE',  ( 803.6646147819161570, -137.9073299311473875, -348.8264449731210561 ) ) ;
#43131=CARTESIAN_POINT ( 'NONE',  ( 746.8695393053150156, -53.90732993114765037, -327.6429770376306010 ) ) ;
#43133=CARTESIAN_POINT ( 'NONE',  ( 747.6481478633932056, -445.0999726633338582, -353.4146539503763620 ) ) ;
#43135=CARTESIAN_POINT ( 'NONE',  ( 784.1219089521767955, -333.2817908451523863, -315.0488828828318333 ) ) ;
#43139=CARTESIAN_POINT ( 'NONE',  ( 800.0135310231082713, -302.0891481129650629, -325.0180583372163028 ) ) ;
#43143=CARTESIAN_POINT ( 'NONE',  ( 757.4527132478984868, -280.3726999360616787, -329.1273215169538844 ) ) ;
#43144=CARTESIAN_POINT ( 'NONE',  ( 805.1927285166397041, -280.8164208402378677, -341.8018195045277707 ) ) ;
#43146=CARTESIAN_POINT ( 'NONE',  ( 759.9864689768902508, -122.0891481129656171, -354.9819416627836404 ) ) ;
#43154=CARTESIAN_POINT ( 'NONE',  ( 804.1009440267234822, -71.46360902697141171, -314.0944755984392600 ) ) ;
#43160=CARTESIAN_POINT ( 'NONE',  ( 749.2812353651451076, -102.4527844766020337, -323.2262854647983090 ) ) ;
#43165=CARTESIAN_POINT ( 'NONE',  ( 749.2812353651451076, -222.4527844766016642, -323.2262854647983090 ) ) ;
#43169=CARTESIAN_POINT ( 'NONE',  ( 781.2497674668890113, -324.3510508353229511, -375.3608509340180603 ) ) ;
#43171=CARTESIAN_POINT ( 'NONE',  ( 787.4397851343537695, -309.7255117493287457, -374.2001403089903988 ) ) ;
#43175=CARTESIAN_POINT ( 'NONE',  ( 804.9363028652555840, -424.2709662947829088, -338.2165204200192079 ) ) ;
#43176=CARTESIAN_POINT ( 'NONE',  ( 759.8311093483677041, -94.16923265350555994, -310.9282345327691814 ) ) ;
#43182=CARTESIAN_POINT ( 'NONE',  ( 803.8651313633788504, -245.2601417444141987, -332.4468031744301015 ) ) ;
#43184=CARTESIAN_POINT ( 'NONE',  ( 803.8556311672234642, -57.62377810805111267, -365.6418435158340117 ) ) ;
#43185=CARTESIAN_POINT ( 'NONE',  ( 799.5976253717891495, -452.9681489794447771, -356.1016198435977458 ) ) ;
#43187=CARTESIAN_POINT ( 'NONE',  ( 776.2046728542105711, -356.1908817542432075, -304.8212110874238761 ) ) ;
#43191=CARTESIAN_POINT ( 'NONE',  ( 775.8780910478218402, -177.2817908451528695, -364.9511171171680530 ) ) ;
#43192=CARTESIAN_POINT ( 'NONE',  ( 804.4286716492782716, -185.3618753856926844, -345.3141322388244703 ) ) ;
#43193=CARTESIAN_POINT ( 'NONE',  ( 771.1735550268780344, -369.1800572038739006, -316.3353852180828198 ) ) ;
#43195=CARTESIAN_POINT ( 'NONE',  ( 805.0264073115434940, 17.64894916467593688, -339.4763451958999099 ) ) ;
#43203=ORIENTED_EDGE ( 'NONE', *, *, #11778, .T. ) ;
#43204=CARTESIAN_POINT ( 'NONE',  ( 762.1177392798416577, -402.5545181178795247, -309.8865473780659272 ) ) ;
#43206=CARTESIAN_POINT ( 'NONE',  ( 808.0189434323515343, -14.08914811296595460, -319.0252816721025511 ) ) ;
#43209=CARTESIAN_POINT ( 'NONE',  ( 774.6858677611749044, -345.7255117493285184, -315.5713283507209894 ) ) ;
#43210=CARTESIAN_POINT ( 'NONE',  ( 781.7834795799800531, 13.18357915976123174, -315.0636971347436202 ) ) ;
#43212=CARTESIAN_POINT ( 'NONE',  ( 805.2837595273609850, -242.7363362996980811, -340.5290396650784714 ) ) ;
#43221=CARTESIAN_POINT ( 'NONE',  ( 762.3223304703356007, -319.5436935675104451, -322.3223304703362828 ) ) ;
#43227=CARTESIAN_POINT ( 'NONE',  ( 811.3240766477731540, -76.37269993606228979, -355.6651683502462902 ) ) ;
#43228=CARTESIAN_POINT ( 'NONE',  ( 802.7791456095903868, -124.7146871989599930, -329.0155153010375102 ) ) ;
#43232=CARTESIAN_POINT ( 'NONE',  ( 758.0580252608178853, -30.45278447660226817, -328.0187753319985404 ) ) ;
#43233=CARTESIAN_POINT ( 'NONE',  ( 775.9200461376533440, -119.8055962898690865, -315.3028492785443291 ) ) ;
#43234=CARTESIAN_POINT ( 'NONE',  ( 778.2165204200184689, -94.81642084023843609, -364.9363028652563230 ) ) ;
#43235=CARTESIAN_POINT ( 'NONE',  ( 788.7631598425961101, 22.55804007376682918, -305.7194118038759143 ) ) ;
#43248=CARTESIAN_POINT ( 'NONE',  ( 761.4292242960306112, -65.46360902697142592, -323.2154366446414429 ) ) ;
#43250=CARTESIAN_POINT ( 'NONE',  ( 795.1360043628808398, -284.0891481129651197, -360.2193346964456282 ) ) ;
#43252=CARTESIAN_POINT ( 'NONE',  ( 800.2193346964447755, -402.9982390220555430, -355.1360043628815788 ) ) ;
#43253=CARTESIAN_POINT ( 'NONE',  ( 792.1044303154645831, -36.45278447660223975, -317.8323909638837677 ) ) ;
#43256=LINE ( 'NONE', #31934, #35355 ) ;
#43258=CARTESIAN_POINT ( 'NONE',  ( 762.1177392798416577, -18.55451811788065797, -309.8865473780659272 ) ) ;
#43261=CARTESIAN_POINT ( 'NONE',  ( 814.8207195650702488, -314.1908817542433781, -336.2433038121456548 ) ) ;
#43264=CARTESIAN_POINT ( 'NONE',  ( 802.1676090361156639, -254.6346026584196238, -327.8955696845344505 ) ) ;
#43266=CARTESIAN_POINT ( 'NONE',  ( 763.8424801807145741, -138.0090635724257311, -320.5453621957614700 ) ) ;
#43269=CARTESIAN_POINT ( 'NONE',  ( 768.8385539511368734, -23.26014174441484883, -306.4236121716840557 ) ) ;
#43270=CARTESIAN_POINT ( 'NONE',  ( 813.1304606946831655, -353.9073299311467053, -352.3570229623691716 ) ) ;
#43275=CARTESIAN_POINT ( 'NONE',  ( 815.0009284576459549, -222.3510508353233206, -338.7629533639073429 ) ) ;
#43277=CARTESIAN_POINT ( 'NONE',  ( 796.9462024416508257, 11.54721552339760038, -308.9653473494370246 ) ) ;
#43284=CARTESIAN_POINT ( 'NONE',  ( 795.9930595647434757, -27.07832356259665474, -320.7433823573372820 ) ) ;
#43292=CARTESIAN_POINT ( 'NONE',  ( 802.7791456095903868, -292.7146871989594956, -329.0155153010375102 ) ) ;
#43295=CARTESIAN_POINT ( 'NONE',  ( 801.9858362298568863, -315.0783235625957559, -312.7379699480935642 ) ) ;
#43296=CARTESIAN_POINT ( 'NONE',  ( 779.9999999999992042, -452.9681489794448339, -339.9999999999999432 ) ) ;
#43300=CARTESIAN_POINT ( 'NONE',  ( 770.0799878456142551, -85.98741447168738716, -362.9823548866085616 ) ) ;
#43302=CARTESIAN_POINT ( 'NONE',  ( 799.9999999999993179, 205.0000000000000568, -360.0000000000000000 ) ) ;
#43303=CARTESIAN_POINT ( 'NONE',  ( 772.5602148656447525, -177.7255117493290868, -305.7998596910095443 ) ) ;
#43305=CARTESIAN_POINT ( 'NONE',  ( 791.9812246680005501, -140.6346026584201070, -361.9419747391813189 ) ) ;
#43307=CARTESIAN_POINT ( 'NONE',  ( 755.8894580844503253, -423.8272453906067199, -332.3691319403863531 ) ) ;
#43317=CARTESIAN_POINT ( 'NONE',  ( 802.9823548866075953, -409.0999726633340288, -330.0799878456151077 ) ) ;
#43319=CARTESIAN_POINT ( 'NONE',  ( 793.5525998758768083, -199.0999726633346825, -372.6845335610516941 ) ) ;
#43324=CARTESIAN_POINT ( 'NONE',  ( 786.6156483768007774, -337.4419599262319593, -315.5913626894246136 ) ) ;
#43326=CARTESIAN_POINT ( 'NONE',  ( 757.7880784355613741, -186.0090635724255890, -312.4576283171834916 ) ) ;
#43327=FACE_BOUND ( 'NONE', #32625, .T. ) ;
#43329=AXIS2_PLACEMENT_3D ( 'NONE', #5188, #33362, #1493 ) ;
#43332=CARTESIAN_POINT ( 'NONE',  ( 767.6429770376291799, -249.1800572038742700, -306.8695393053162093 ) ) ;
#43334=CARTESIAN_POINT ( 'NONE',  ( 778.2165204200184689, 1.183579159761269040, -364.9363028652563230 ) ) ;
#43336=CARTESIAN_POINT ( 'NONE',  ( 746.7653713866222915, -137.2601417444144829, -351.0478386215610271 ) ) ;
#43338=CARTESIAN_POINT ( 'NONE',  ( 772.5602148656447525, -369.7255117493284615, -305.7998596910095443 ) ) ;
#43344=CARTESIAN_POINT ( 'NONE',  ( 776.2433038121456548, -420.8965053807772279, -374.8207195650711014 ) ) ;
#43345=CARTESIAN_POINT ( 'NONE',  ( 795.8262568251477660, 1.627300063937458408, -308.3538107759623585 ) ) ;
#43350=CARTESIAN_POINT ( 'NONE',  ( 790.8726784830453198, -202.7146871989597514, -362.5472867521010585 ) ) ;
#43352=CARTESIAN_POINT ( 'NONE',  ( 805.9055244015594326, -219.6237781080506295, -315.8990559732753240 ) ) ;
#43355=CARTESIAN_POINT ( 'NONE',  ( 792.1044303154645831, -84.45278447660206211, -317.8323909638837677 ) ) ;
#43359=CARTESIAN_POINT ( 'NONE',  ( 754.8072714833581358, -148.8164208402382656, -338.1981804954720587 ) ) ;
#43361=CARTESIAN_POINT ( 'NONE',  ( 787.4397851343537695, -45.72551174932949181, -374.2001403089903988 ) ) ;
#43362=EDGE_CURVE ( 'NONE', #16032, #17925, #19744, .T. ) ;
#43364=CARTESIAN_POINT ( 'NONE',  ( 754.3581564841646241, -449.4636090269702322, -316.1443688327762516 ) ) ;
#43366=CARTESIAN_POINT ( 'NONE',  ( 763.0428371773158460, -323.4636090269706301, -358.7617431975195359 ) ) ;
#43370=CARTESIAN_POINT ( 'NONE',  ( 757.8323909638827445, -290.6346026584195101, -352.1044303154654358 ) ) ;
#43374=CARTESIAN_POINT ( 'NONE',  ( 769.9779781133707957, -283.0999726633344267, -316.7813123517150871 ) ) ;
#43375=CARTESIAN_POINT ( 'NONE',  ( 755.5713283507202505, -293.3618753856923718, -334.6858677611754729 ) ) ;
#43376=CARTESIAN_POINT ( 'NONE',  ( 756.5762568750052424, -147.1800572038746395, -348.7366044899774238 ) ) ;
#43381=CARTESIAN_POINT ( 'NONE',  ( 813.5763878283155464, -99.82724539060768620, -351.1614460488615350 ) ) ;
#43384=EDGE_CURVE ( 'NONE', #11148, #39743, #26885, .T. ) ;
#43388=CARTESIAN_POINT ( 'NONE',  ( 751.9810565676468741, -146.0891481129655176, -360.9747183278973921 ) ) ;
#43394=CARTESIAN_POINT ( 'NONE',  ( 787.4397851343537695, -261.7255117493288026, -374.2001403089903988 ) ) ;
#43398=CARTESIAN_POINT ( 'NONE',  ( 798.0661480581538854, -290.5328690171412518, -309.5768839229118043 ) ) ;
#43400=CARTESIAN_POINT ( 'NONE',  ( 751.9810565676468741, -338.0891481129649492, -360.9747183278973921 ) ) ;
#43404=CARTESIAN_POINT ( 'NONE',  ( 774.6312213355099630, -407.3618753856920307, -364.6798772138717482 ) ) ;
#43405=CARTESIAN_POINT ( 'NONE',  ( 811.6461892240364477, -100.7146871989600356, -324.1737431748509835 ) ) ;
#43409=CARTESIAN_POINT ( 'NONE',  ( 801.3366627262608972, -224.5328690171415076, -353.0897708529566899 ) ) ;
#43411=CARTESIAN_POINT ( 'NONE',  ( 768.8385539511368734, -71.26014174441469606, -306.4236121716840557 ) ) ;
#43412=CARTESIAN_POINT ( 'NONE',  ( 804.5667330414263461, -452.9681489794450044, -348.7981942340067576 ) ) ;
#43415=CARTESIAN_POINT ( 'NONE',  ( 773.7305795820266212, -345.2817908451523863, -374.8230680027170365 ) ) ;
#43419=CARTESIAN_POINT ( 'NONE',  ( 802.9823548866075953, -169.0999726633347393, -330.0799878456151077 ) ) ;
#43420=CARTESIAN_POINT ( 'NONE',  ( 781.8018195045266339, -190.2709662947835909, -365.1927285166406705 ) ) ;
#43421=CARTESIAN_POINT ( 'NONE',  ( 756.5762568750052424, -387.1800572038738437, -348.7366044899774238 ) ) ;
#43423=CARTESIAN_POINT ( 'NONE',  ( 794.1144889064781864, 13.83076734649413098, -360.9840315886528401 ) ) ;
#43431=CARTESIAN_POINT ( 'NONE',  ( 744.6391490659812007, -422.7363362996975980, -338.7502325331110455 ) ) ;
#43432=CARTESIAN_POINT ( 'NONE',  ( 746.8695393053151292, -29.90732993114772142, -327.6429770376306578 ) ) ;
#43434=CARTESIAN_POINT ( 'NONE',  ( 756.5762568750052424, -387.1800572038738437, -348.7366044899774238 ) ) ;
#43435=CARTESIAN_POINT ( 'NONE',  ( 804.4286716492782716, 6.638124614306706306, -345.3141322388244703 ) ) ;
#43438=CARTESIAN_POINT ( 'NONE',  ( 754.7162404726377645, -254.7363362996981095, -339.4709603349214717 ) ) ;
#43439=CARTESIAN_POINT ( 'NONE',  ( 777.5031285880264704, -166.8164208402382087, -374.9108240113588408 ) ) ;
#43442=CARTESIAN_POINT ( 'NONE',  ( 772.8365271371600329, 16.45630643248849267, -315.6518837687410723 ) ) ;
#43448=CARTESIAN_POINT ( 'NONE',  ( 785.3141322388236176, -309.7255117493287457, -364.4286716492789537 ) ) ;
#43451=CARTESIAN_POINT ( 'NONE',  ( 814.2805881961230625, -49.64542720878965554, -331.2368401574024119 ) ) ;
#43452=CARTESIAN_POINT ( 'NONE',  ( 765.8855110935204493, -118.1692326535054463, -319.0159684113471599 ) ) ;
#43455=CARTESIAN_POINT ( 'NONE',  ( 803.6646147819161570, -17.90732993114776406, -348.8264449731210561 ) ) ;
#43456=CARTESIAN_POINT ( 'NONE',  ( 794.1144889064781864, -130.1692326535054463, -360.9840315886528401 ) ) ;
#43457=CARTESIAN_POINT ( 'NONE',  ( 797.6776695296629214, -139.5436935675110135, -357.6776695296636603 ) ) ;
#43458=CARTESIAN_POINT ( 'NONE',  ( 783.0433043558608688, -432.8965053807771142, -315.1538015810313027 ) ) ;
#43469=CARTESIAN_POINT ( 'NONE',  ( 793.9708237608222134, -94.91815448151677970, -319.2295555964448681 ) ) ;
#43471=CARTESIAN_POINT ( 'NONE',  ( 759.9864689768902508, -290.0891481129650629, -354.9819416627836404 ) ) ;
#43473=CARTESIAN_POINT ( 'NONE',  ( 774.6312213355099630, -407.3618753856920307, -364.6798772138717482 ) ) ;
#43474=CARTESIAN_POINT ( 'NONE',  ( 804.4286716492782716, -65.36187538569306810, -345.3141322388244703 ) ) ;
#43478=CARTESIAN_POINT ( 'NONE',  ( 809.0717654672305343, -28.91815448151699286, -360.1688906516309885 ) ) ;
#43481=CARTESIAN_POINT ( 'NONE',  ( 783.7953271457878373, -320.1908817542434349, -375.1787889125761239 ) ) ;
#43484=CARTESIAN_POINT ( 'NONE',  ( 755.0636971347428243, -292.2709662947831930, -341.7834795799807353 ) ) ;
#43486=CARTESIAN_POINT ( 'NONE',  ( 763.0428371773158460, -155.4636090269711417, -358.7617431975195359 ) ) ;
#43490=CARTESIAN_POINT ( 'NONE',  ( 745.0891759886404770, -364.2709662947830793, -342.4968714119734159 ) ) ;
#43494=CARTESIAN_POINT ( 'NONE',  ( 813.9316612368132837, -223.4419599262323857, -348.6739635108323228 ) ) ;
#43496=CARTESIAN_POINT ( 'NONE',  ( 814.9108240113580450, 7.729033705215793582, -337.5031285880265273 ) ) ;
#43501=CARTESIAN_POINT ( 'NONE',  ( 803.8651313633788504, -29.26014174441482751, -332.4468031744301015 ) ) ;
#43507=CARTESIAN_POINT ( 'NONE',  ( 755.0488828828309806, -329.8055962898683902, -344.1219089521771934 ) ) ;
#43510=CARTESIAN_POINT ( 'NONE',  ( 759.8311093483677041, -334.1692326535047073, -310.9282345327691814 ) ) ;
#43517=LINE ( 'NONE', #43302, #6196 ) ;
#43519=CARTESIAN_POINT ( 'NONE',  ( 746.8695393053150156, -173.9073299311472169, -327.6429770376306010 ) ) ;
#43521=CARTESIAN_POINT ( 'NONE',  ( 757.8323909638828582, -170.6346026584199933, -352.1044303154654358 ) ) ;
#43523=CARTESIAN_POINT ( 'NONE',  ( 802.9823548866075953, -433.0999726633339151, -330.0799878456151077 ) ) ;
#43527=DIRECTION ( 'NONE',  ( -0.000000000000000000, 1.000000000000000000, -0.000000000000000000 ) ) ;
#43530=CARTESIAN_POINT ( 'NONE',  ( 761.4292242960306112, -425.4636090269703459, -323.2154366446414429 ) ) ;
#43531=CARTESIAN_POINT ( 'NONE',  ( 772.4999999999993179, -462.9681489794447202, -270.0000000000000568 ) ) ;
#43532=CARTESIAN_POINT ( 'NONE',  ( 811.3240766477731540, -220.3726999360618208, -355.6651683502462902 ) ) ;
#43535=PLANE ( 'NONE',  #43958 ) ;
#43536=CARTESIAN_POINT ( 'NONE',  ( 805.0264073115434940, -318.3510508353230080, -339.4763451958999099 ) ) ;
#43538=CARTESIAN_POINT ( 'NONE',  ( 791.0478386215596629, -213.8272453906073167, -306.7653713866226326 ) ) ;
#43543=CARTESIAN_POINT ( 'NONE',  ( 745.7998596910086917, -245.3618753856925139, -332.5602148656461168 ) ) ;
#43546=CARTESIAN_POINT ( 'NONE',  ( 785.3687786644884454, -11.36187538569323863, -315.3201227861279676 ) ) ;
#43548=CARTESIAN_POINT ( 'NONE',  ( 800.1688906516307043, -130.1692326535054463, -369.0717654672308186 ) ) ;
#43550=CARTESIAN_POINT ( 'NONE',  ( 749.2812353651451076, -366.4527844766012095, -323.2262854647983090 ) ) ;
#43555=CARTESIAN_POINT ( 'NONE',  ( 785.3141322388236176, -381.7255117493284615, -364.4286716492789537 ) ) ;
#43556=CARTESIAN_POINT ( 'NONE',  ( 766.4474001241216001, 4.900027336664720679, -307.3154664389482491 ) ) ;
#43557=DIRECTION ( 'NONE',  ( -0.000000000000000000, -0.000000000000000000, 1.000000000000000000 ) ) ;
#43561=CARTESIAN_POINT ( 'NONE',  ( 754.8983024940795303, -210.8965053807778816, -336.9254006560228163 ) ) ;
#43563=CARTESIAN_POINT ( 'NONE',  ( 764.3348316497523456, -238.7146871989596661, -308.6759233522265617 ) ) ;
#43571=CARTESIAN_POINT ( 'NONE',  ( 759.0252816721024374, -72.99823902205667991, -368.0189434323527280 ) ) ;
#43572=CARTESIAN_POINT ( 'NONE',  ( 797.6776695296629214, -67.54369356751125508, -357.6776695296636603 ) ) ;
#43574=CARTESIAN_POINT ( 'NONE',  ( 784.1219089521767955, 2.718209154846545683, -315.0488828828318333 ) ) ;
#43576=CARTESIAN_POINT ( 'NONE',  ( 755.3028492785439312, -327.2817908451525000, -335.9200461376539693 ) ) ;
#43580=CARTESIAN_POINT ( 'NONE',  ( 759.9864689768902508, -338.0891481129649492, -354.9819416627836404 ) ) ;
#43584=CARTESIAN_POINT ( 'NONE',  ( 755.1538015810308480, -326.1908817542433781, -343.0433043558613804 ) ) ;
#43585=CARTESIAN_POINT ( 'NONE',  ( 804.9363028652555840, -280.2709662947833067, -338.2165204200192079 ) ) ;
#43587=CARTESIAN_POINT ( 'NONE',  ( 803.6646147819161570, -161.9073299311472454, -348.8264449731210561 ) ) ;
#43594=CARTESIAN_POINT ( 'NONE',  ( 745.5313806188320314, -87.28179084515316788, -333.7943932421247268 ) ) ;
#43601=CARTESIAN_POINT ( 'NONE',  ( 772.5602148656447525, -129.7255117493292289, -305.7998596910095443 ) ) ;
#43605=CARTESIAN_POINT ( 'NONE',  ( 751.9810565676468741, -266.0891481129651197, -360.9747183278973921 ) ) ;
#43609=CARTESIAN_POINT ( 'NONE',  ( 746.7653713866222915, -329.2601417444138860, -351.0478386215610271 ) ) ;
#43610=CARTESIAN_POINT ( 'NONE',  ( 758.8095938919642549, -80.08914811296574499, -311.6929314249763365 ) ) ;
#43613=CARTESIAN_POINT ( 'NONE',  ( 767.6429770376289525, -345.1800572038739006, -306.8695393053162093 ) ) ;
#43618=CARTESIAN_POINT ( 'NONE',  ( 781.8018195045266339, -430.2709662947827383, -365.1927285166406705 ) ) ;
#43620=CARTESIAN_POINT ( 'NONE',  ( 795.1360043628807261, -212.0891481129652902, -360.2193346964456282 ) ) ;
#43621=CARTESIAN_POINT ( 'NONE',  ( 751.2241431872005251, -112.1692326535054889, -359.9636004259367610 ) ) ;
#43625=CARTESIAN_POINT ( 'NONE',  ( 802.7791456095903868, -244.7146871989596093, -329.0155153010375102 ) ) ;
#43628=CARTESIAN_POINT ( 'NONE',  ( 772.5602148656447525, 14.27448825067031812, -305.7998596910095443 ) ) ;
#43629=CARTESIAN_POINT ( 'NONE',  ( 776.2433038121456548, -60.89650538077837894, -374.8207195650711014 ) ) ;
#43633=CARTESIAN_POINT ( 'NONE',  ( 771.3260364891663130, -379.6454272087886466, -306.0683387631859773 ) ) ;
#43636=CARTESIAN_POINT ( 'NONE',  ( 804.8461984189677878, -194.1908817542437475, -336.9566956441385628 ) ) ;
#43637=CARTESIAN_POINT ( 'NONE',  ( 755.3201227861273992, -171.7255117493291152, -345.3687786644892981 ) ) ;
#43639=CARTESIAN_POINT ( 'NONE',  ( 785.3687786644885591, -371.3618753856920307, -315.3201227861280813 ) ) ;
#43642=CARTESIAN_POINT ( 'NONE',  ( 784.0799538623451781, 12.19440371013049784, -364.6971507214555572 ) ) ;
#43646=CARTESIAN_POINT ( 'NONE',  ( 792.0613484971601110, -458.0032201311295807, -367.4685979341032294 ) ) ;
#43650=ORIENTED_EDGE ( 'NONE', *, *, #18208, .T. ) ;
#43651=CARTESIAN_POINT ( 'NONE',  ( 754.3581564841646241, -401.4636090269704027, -316.1443688327762516 ) ) ;
#43652=CARTESIAN_POINT ( 'NONE',  ( 792.3570229623691148, -21.18005720387502322, -373.1304606946836770 ) ) ;
#43654=CARTESIAN_POINT ( 'NONE',  ( 762.1405469898971887, -409.5436935675101040, -357.8594530101015607 ) ) ;
#43655=CARTESIAN_POINT ( 'NONE',  ( 756.5762568750052424, -3.180057203875080063, -348.7366044899774238 ) ) ;
#43658=CARTESIAN_POINT ( 'NONE',  ( 783.0745993439762742, -248.1908817542435202, -365.1016975059196739 ) ) ;
#43659=CARTESIAN_POINT ( 'NONE',  ( 772.5602148656447525, -153.7255117493291721, -305.7998596910095443 ) ) ;
#43662=CARTESIAN_POINT ( 'NONE',  ( 795.2260422076361692, 16.45630643248849978, -314.2591110605560516 ) ) ;
#43665=EDGE_CURVE ( 'NONE', #23858, #19525, #5, .T. ) ;
#43668=CARTESIAN_POINT ( 'NONE',  ( 759.7806653035534055, -318.9982390220557704, -324.8639956371180801 ) ) ;
#43671=CARTESIAN_POINT ( 'NONE',  ( 747.6481478633932056, -109.0999726633349241, -353.4146539503763620 ) ) ;
#43672=CARTESIAN_POINT ( 'NONE',  ( 804.1601925771018387, -127.4419599262326983, -346.5483106153029098 ) ) ;
#43675=CARTESIAN_POINT ( 'NONE',  ( 804.9363028652555840, -16.27096629478413092, -338.2165204200192079 ) ) ;
#43676=CARTESIAN_POINT ( 'NONE',  ( 776.9566956441375396, -132.8965053807781374, -364.8461984189686405 ) ) ;
#43677=CARTESIAN_POINT ( 'NONE',  ( 756.3353852180819104, -125.9073299311474159, -331.1735550268788302 ) ) ;
#43679=CARTESIAN_POINT ( 'NONE',  ( 801.3366627262608972, -440.5328690171407970, -353.0897708529566899 ) ) ;
#43683=VERTEX_POINT ( 'NONE', #6664 ) ;
#43690=CARTESIAN_POINT ( 'NONE',  ( 802.9823548866075953, -73.09997266333502353, -330.0799878456151077 ) ) ;
#43692=CARTESIAN_POINT ( 'NONE',  ( 754.8072714833583632, -292.8164208402378108, -338.1981804954721156 ) ) ;
#43694=CARTESIAN_POINT ( 'NONE',  ( 778.1981804954714335, -394.2709662947827951, -314.8072714833589885 ) ) ;
#43695=CARTESIAN_POINT ( 'NONE',  ( 774.6312213355099630, -47.36187538569312494, -364.6798772138717482 ) ) ;
#43699=CARTESIAN_POINT ( 'NONE',  ( 749.5768839229115201, -12.55451811788067751, -358.0661480581553064 ) ) ;
#43702=CARTESIAN_POINT ( 'NONE',  ( 749.5768839229115201, -300.5545181178797520, -358.0661480581553064 ) ) ;
#43705=CARTESIAN_POINT ( 'NONE',  ( 754.8072714833581358, -292.8164208402376971, -338.1981804954720587 ) ) ;
#43707=CARTESIAN_POINT ( 'NONE',  ( 801.5560724626406000, -144.5545181178802636, -326.7756240680316182 ) ) ;
#43709=CARTESIAN_POINT ( 'NONE',  ( 754.0944755984390895, -15.62377810805123524, -364.1009440267246760 ) ) ;
#43710=CARTESIAN_POINT ( 'NONE',  ( 810.7187646348534145, -330.4527844766013231, -356.7737145352016341 ) ) ;
#43715=CARTESIAN_POINT ( 'NONE',  ( 811.0346526505616112, 9.365397341579420498, -323.0537975583477532 ) ) ;
#43721=CARTESIAN_POINT ( 'NONE',  ( 790.8726784830453198, -10.71468719896033761, -362.5472867521010585 ) ) ;
#43726=CARTESIAN_POINT ( 'NONE',  ( 783.0433043558608688, -312.8965053807775689, -315.1538015810313027 ) ) ;
#43728=CARTESIAN_POINT ( 'NONE',  ( 803.8556311672234642, -345.6237781080501463, -365.6418435158340117 ) ) ;
#43734=CARTESIAN_POINT ( 'NONE',  ( 744.7301800767019131, -172.8164208402381234, -337.4774526936615757 ) ) ;
#43737=CARTESIAN_POINT ( 'NONE',  ( 778.2165204200184689, -166.8164208402382087, -364.9363028652563230 ) ) ;
#43739=CARTESIAN_POINT ( 'NONE',  ( 805.2837595273609850, -410.7363362996976548, -340.5290396650784714 ) ) ;
#43745=CARTESIAN_POINT ( 'NONE',  ( 804.8461984189677878, -434.1908817542430370, -336.9566956441385628 ) ) ;
#43748=CARTESIAN_POINT ( 'NONE',  ( 786.2694204179717872, -189.2817908451528979, -305.1769319972829067 ) ) ;
#43751=DIRECTION ( 'NONE',  ( -1.000000000000000000, -0.000000000000000000, -0.000000000000000000 ) ) ;
#43752=CARTESIAN_POINT ( 'NONE',  ( 756.5762568750052424, -171.1800572038745543, -348.7366044899774238 ) ) ;
#43753=CARTESIAN_POINT ( 'NONE',  ( 804.9511171171677688, -341.8055962898683333, -335.8780910478229202 ) ) ;
#43755=CARTESIAN_POINT ( 'NONE',  ( 788.6739635108323228, -223.6454272087891013, -373.9316612368139090 ) ) ;
#43758=CARTESIAN_POINT ( 'NONE',  ( 790.0220218866281812, -31.09997266333516919, -363.2186876482849129 ) ) ;
#43760=CARTESIAN_POINT ( 'NONE',  ( 755.2512626584698410, -247.5436935675106724, -315.2512626584710915 ) ) ;
#43762=CARTESIAN_POINT ( 'NONE',  ( 755.3201227861273992, -3.725511749329622813, -345.3687786644892981 ) ) ;
#43764=CARTESIAN_POINT ( 'NONE',  ( 752.4576283171824116, -117.0783235625963528, -317.7880784355627952 ) ) ;
#43766=CARTESIAN_POINT ( 'NONE',  ( 747.2067596250078623, -387.1800572038738437, -352.2312462859687230 ) ) ;
#43771=CARTESIAN_POINT ( 'NONE',  ( 795.1360043628807261, -380.0891481129646650, -360.2193346964456282 ) ) ;
#43772=CARTESIAN_POINT ( 'NONE',  ( 755.2512626584698410, 16.45630643248848912, -315.2512626584710915 ) ) ;
#43773=CARTESIAN_POINT ( 'NONE',  ( 814.9108240113580450, -448.2709662947827951, -337.5031285880265273 ) ) ;
#43776=ORIENTED_EDGE ( 'NONE', *, *, #42420, .F. ) ;
#43777=CARTESIAN_POINT ( 'NONE',  ( 779.4709603349208464, -216.3510508353233490, -314.7162404726379918 ) ) ;
#43781=CARTESIAN_POINT ( 'NONE',  ( 761.9338519418445230, -230.5328690171415076, -370.4231160770881957 ) ) ;
#43785=CARTESIAN_POINT ( 'NONE',  ( 762.3223304703356007, -151.5436935675109851, -322.3223304703362828 ) ) ;
#43787=CARTESIAN_POINT ( 'NONE',  ( 767.6429770376289525, -81.18005720387481006, -306.8695393053162093 ) ) ;
#43789=CARTESIAN_POINT ( 'NONE',  ( 774.6312213355098493, -71.36187538569303968, -364.6798772138717482 ) ) ;
#43791=CARTESIAN_POINT ( 'NONE',  ( 760.7433823573367135, -12.00906357242613609, -355.9930595647440441 ) ) ;
#43792=ORIENTED_EDGE ( 'NONE', *, *, #14813, .F. ) ;
#43793=CARTESIAN_POINT ( 'NONE',  ( 766.9102291470427417, -330.5545181178796952, -318.6633372737382501 ) ) ;
#43801=CARTESIAN_POINT ( 'NONE',  ( 769.9779781133707957, -331.0999726633342561, -316.7813123517150871 ) ) ;
#43802=CARTESIAN_POINT ( 'NONE',  ( 788.8264449731200330, -309.1800572038740711, -363.6646147819171233 ) ) ;
#43803=CARTESIAN_POINT ( 'NONE',  ( 771.2633955100217236, -143.9073299311473590, -363.4237431249939618 ) ) ;
#43807=CARTESIAN_POINT ( 'NONE',  ( 768.9521613784389729, -105.8272453906076578, -373.2346286133773106 ) ) ;
#43813=CIRCLE ( 'NONE', #29811, 30.00000000000002842 ) ;
#43814=CARTESIAN_POINT ( 'NONE',  ( 777.5031285880264704, -142.8164208402382656, -374.9108240113588408 ) ) ;
#43816=CARTESIAN_POINT ( 'NONE',  ( 801.1904061080336987, -284.0891481129650629, -368.3070685750235498 ) ) ;
#43818=CARTESIAN_POINT ( 'NONE',  ( 755.2512626584698410, -439.5436935675101040, -315.2512626584710915 ) ) ;
#43821=CARTESIAN_POINT ( 'NONE',  ( 756.1443688327750579, -333.6237781080502600, -314.3581564841659315 ) ) ;
#43822=CARTESIAN_POINT ( 'NONE',  ( 747.2067596250078623, -75.18005720387485269, -352.2312462859687230 ) ) ;
#43825=CARTESIAN_POINT ( 'NONE',  ( 755.2512626584698410, -343.5436935675103314, -315.2512626584710915 ) ) ;
#43830=CARTESIAN_POINT ( 'NONE',  ( 756.3353852180819104, -221.9073299311470464, -331.1735550268788302 ) ) ;
#43831=CARTESIAN_POINT ( 'NONE',  ( 814.8230680027162407, -125.8055962898690581, -333.7305795820267917 ) ) ;
#43837=CARTESIAN_POINT ( 'NONE',  ( 770.0799878456142551, -229.9874144716869466, -362.9823548866085616 ) ) ;
#43839=CARTESIAN_POINT ( 'NONE',  ( 744.8212110874229666, -426.8965053807771142, -336.2046728542121627 ) ) ;
#43840=CARTESIAN_POINT ( 'NONE',  ( 811.6461892240364477, -76.71468719896012090, -324.1737431748509835 ) ) ;
#43845=VERTEX_POINT ( 'NONE', #17533 ) ;
#43846=CARTESIAN_POINT ( 'NONE',  ( 749.5768839229115201, -372.5545181178796383, -358.0661480581553064 ) ) ;
#43848=CARTESIAN_POINT ( 'NONE',  ( 791.9812246680005501, -236.6346026584198228, -361.9419747391813189 ) ) ;
#43851=CARTESIAN_POINT ( 'NONE',  ( 793.0897708529556667, -222.5545181178800362, -361.3366627262616362 ) ) ;
#43852=CARTESIAN_POINT ( 'NONE',  ( 803.6646147819161570, -185.9073299311472454, -348.8264449731210561 ) ) ;
#43853=CARTESIAN_POINT ( 'NONE',  ( 754.8072714833583632, -388.8164208402374129, -338.1981804954721156 ) ) ;
#43856=CARTESIAN_POINT ( 'NONE',  ( 791.9812246680005501, -116.6346026584201780, -361.9419747391813189 ) ) ;
#43864=AXIS2_PLACEMENT_3D ( 'NONE', #3349, #42140, #33121 ) ;
#43870=CARTESIAN_POINT ( 'NONE',  ( 809.0717654672305343, -436.9181544815157281, -360.1688906516309885 ) ) ;
#43871=CARTESIAN_POINT ( 'NONE',  ( 759.0252816721024374, -48.99823902205675807, -368.0189434323527280 ) ) ;
#43873=CARTESIAN_POINT ( 'NONE',  ( 755.3201227861273992, -411.7255117493282910, -345.3687786644892981 ) ) ;
#43874=CARTESIAN_POINT ( 'NONE',  ( 771.2633955100217236, -23.90732993114773919, -363.4237431249939618 ) ) ;
#43877=CARTESIAN_POINT ( 'NONE',  ( 798.5707757039680246, -245.4636090269709143, -356.7845633553585003 ) ) ;
#43878=CARTESIAN_POINT ( 'NONE',  ( 777.4774526936600978, -178.2709662947835625, -304.7301800767027657 ) ) ;
#43883=CARTESIAN_POINT ( 'NONE',  ( 791.7419236033215384, 16.45630643248850689, -314.5156751397937001 ) ) ;
#43885=AXIS2_PLACEMENT_3D ( 'NONE', #33492, #1840, #2296 ) ;
#43888=CARTESIAN_POINT ( 'NONE',  ( 804.6798772138708955, -327.7255117493285184, -334.6312213355107019 ) ) ;
#43891=CARTESIAN_POINT ( 'NONE',  ( 760.0363995740630116, -82.91815448151682233, -368.7758568127991907 ) ) ;
#43892=CARTESIAN_POINT ( 'NONE',  ( 790.8726784830453198, -130.7146871989599504, -362.5472867521010585 ) ) ;
#43898=CARTESIAN_POINT ( 'NONE',  ( 795.1360043628807261, -20.08914811296592973, -360.2193346964456282 ) ) ;
#43899=CARTESIAN_POINT ( 'NONE',  ( 756.7813123517142913, -115.9874144716872877, -329.9779781133712504 ) ) ;
#43900=CARTESIAN_POINT ( 'NONE',  ( 804.6798772138708955, -135.7255117493291152, -334.6312213355107019 ) ) ;
#43903=CARTESIAN_POINT ( 'NONE',  ( 775.9200461376533440, -431.8055962898681059, -315.3028492785443291 ) ) ;
#43909=CARTESIAN_POINT ( 'NONE',  ( 799.9636004259356241, -286.9181544815161828, -311.2241431872006956 ) ) ;
#43916=CARTESIAN_POINT ( 'NONE',  ( 804.8461984189677878, -98.19088175424404596, -336.9566956441385628 ) ) ;
#43917=CARTESIAN_POINT ( 'NONE',  ( 755.3201227861273992, -291.7255117493286320, -345.3687786644892981 ) ) ;
#43920=CARTESIAN_POINT ( 'NONE',  ( 759.9864689768902508, -410.0891481129647218, -354.9819416627836404 ) ) ;
#43921=CARTESIAN_POINT ( 'NONE',  ( 755.3201227861273992, -99.72551174932928575, -345.3687786644892981 ) ) ;
#43922=CIRCLE ( 'NONE', #37299, 30.00000000000008171 ) ;
#43927=EDGE_CURVE ( 'NONE', #38426, #30631, #4999, .T. ) ;
#43928=CARTESIAN_POINT ( 'NONE',  ( 814.4686193811664907, -3.281790845153435221, -346.2056067578752732 ) ) ;
#43931=CARTESIAN_POINT ( 'NONE',  ( 791.0478386215596629, -309.8272453906070041, -306.7653713866226326 ) ) ;
#43934=CARTESIAN_POINT ( 'NONE',  ( 756.5762568750052424, -291.1800572038741848, -348.7366044899774238 ) ) ;
#43936=CARTESIAN_POINT ( 'NONE',  ( 802.9823548866075953, -169.0999726633347393, -330.0799878456151077 ) ) ;
#43941=CARTESIAN_POINT ( 'NONE',  ( 745.0891759886404770, -340.2709662947831362, -342.4968714119734159 ) ) ;
#43946=CARTESIAN_POINT ( 'NONE',  ( 768.8385539511368734, -431.2601417444136018, -306.4236121716840557 ) ) ;
#43948=DIRECTION ( 'NONE',  ( 0.000000000000000000, 0.000000000000000000, -1.000000000000000000 ) ) ;
#43951=CARTESIAN_POINT ( 'NONE',  ( 798.7617431975189675, -27.62377810805120149, -323.0428371773161871 ) ) ;
#43958=AXIS2_PLACEMENT_3D ( 'NONE', #43531, #21839, #15151 ) ;
#43959=CARTESIAN_POINT ( 'NONE',  ( 779.4709603349208464, -336.3510508353228943, -314.7162404726379918 ) ) ;
#43962=CARTESIAN_POINT ( 'NONE',  ( 758.0141637701419768, -327.0783235625956991, -367.2620300519063790 ) ) ;
#43964=ORIENTED_EDGE ( 'NONE', *, *, #30634, .T. ) ;
#43967=ORIENTED_EDGE ( 'NONE', *, *, #24972, .F. ) ;
#43970=CARTESIAN_POINT ( 'NONE',  ( 749.2812353651451076, -174.4527844766018063, -323.2262854647983090 ) ) ;
#43973=CARTESIAN_POINT ( 'NONE',  ( 764.8639956371174549, -176.0891481129654039, -319.7806653035542581 ) ) ;
#43975=CARTESIAN_POINT ( 'NONE',  ( 804.1105419155481968, -411.8272453906067199, -347.6308680596136469 ) ) ;
#43981=CARTESIAN_POINT ( 'NONE',  ( 799.2566176426618085, -432.0090635724247932, -324.0069404352559559 ) ) ;
#43983=CARTESIAN_POINT ( 'NONE',  ( 781.2370466360911223, -188.7363362996983085, -304.9990715423533629 ) ) ;
#43987=CARTESIAN_POINT ( 'NONE',  ( 802.1676090361156639, -182.6346026584199649, -327.8955696845344505 ) ) ;
#43988=CARTESIAN_POINT ( 'NONE',  ( 800.7704444035546203, -364.1692326535046504, -326.0291762391768771 ) ) ;
#43990=CARTESIAN_POINT ( 'NONE',  ( 766.4474001241216001, -211.0999726633346540, -307.3154664389482491 ) ) ;
#43993=CARTESIAN_POINT ( 'NONE',  ( 790.0220218866281812, -55.09997266333508747, -363.2186876482849129 ) ) ;
#43997=CARTESIAN_POINT ( 'NONE',  ( 804.7487373415286811, -259.5436935675106156, -364.7487373415288516 ) ) ;
#44001=CARTESIAN_POINT ( 'NONE',  ( 788.8264449731200330, -45.18005720387493085, -363.6646147819171233 ) ) ;
#44003=CARTESIAN_POINT ( 'NONE',  ( 759.8311093483677041, -118.1692326535054463, -310.9282345327691814 ) ) ;
#44005=CARTESIAN_POINT ( 'NONE',  ( 787.5162901302840055, -371.3618753856919739, -305.4481719005792684 ) ) ;
#44010=CARTESIAN_POINT ( 'NONE',  ( 802.1676090361156639, -398.6346026584193396, -327.8955696845344505 ) ) ;
#44012=CARTESIAN_POINT ( 'NONE',  ( 749.5768839229115201, -12.55451811788067751, -358.0661480581553064 ) ) ;
#44016=CARTESIAN_POINT ( 'NONE',  ( 756.7813123517142913, -211.9874144716869750, -329.9779781133712504 ) ) ;
#44018=CARTESIAN_POINT ( 'NONE',  ( 786.2056067578752163, -227.8055962898687596, -374.4686193811670023 ) ) ;
#44024=CIRCLE ( 'NONE', #13817, 30.00000000000008171 ) ;
#44025=CARTESIAN_POINT ( 'NONE',  ( 815.2698199232961542, -88.81642084023842187, -342.5225473063383106 ) ) ;
#44026=CARTESIAN_POINT ( 'NONE',  ( 781.7834795799800531, -58.81642084023854267, -315.0636971347436202 ) ) ;
#44028=CARTESIAN_POINT ( 'NONE',  ( 776.9254006560222479, -20.19088175424429110, -314.8983024940802125 ) ) ;
#44030=ORIENTED_EDGE ( 'NONE', *, *, #43362, .T. ) ;
#44031=CARTESIAN_POINT ( 'NONE',  ( 763.8424801807145741, -330.0090635724251342, -320.5453621957614700 ) ) ;
#44039=CARTESIAN_POINT ( 'NONE',  ( 804.1105419155481968, -315.8272453906070609, -347.6308680596136469 ) ) ;
#44040=CARTESIAN_POINT ( 'NONE',  ( 756.5762568750052424, -339.1800572038740142, -348.7366044899774238 ) ) ;
#44041=CARTESIAN_POINT ( 'NONE',  ( 781.8018195045266339, -142.2709662947837330, -365.1927285166406705 ) ) ;
#44046=CARTESIAN_POINT ( 'NONE',  ( 794.1144889064781864, -274.1692326535049915, -360.9840315886528401 ) ) ;
#44047=CARTESIAN_POINT ( 'NONE',  ( 755.8990559732751535, -131.4636090269711985, -365.9055244015606831 ) ) ;
#44054=CARTESIAN_POINT ( 'NONE',  ( 745.0891759886404770, -148.2709662947837330, -342.4968714119734159 ) ) ;
#44055=CARTESIAN_POINT ( 'NONE',  ( 758.7867965644026071, 16.45630643248849267, -318.7867965644036303 ) ) ;
#44057=CARTESIAN_POINT ( 'NONE',  ( 812.7932403749906598, -255.1800572038742700, -327.7687537140311633 ) ) ;
#44063=CARTESIAN_POINT ( 'NONE',  ( 814.8230680027162407, -341.8055962898683333, -333.7305795820267917 ) ) ;
#44065=CARTESIAN_POINT ( 'NONE',  ( 744.7301800767019131, -76.81642084023845030, -337.4774526936615757 ) ) ;
#44067=CARTESIAN_POINT ( 'NONE',  ( 759.0252816721024374, -360.9982390220557704, -368.0189434323527280 ) ) ;
#44071=CARTESIAN_POINT ( 'NONE',  ( 758.0141637701419768, -135.0783235625962959, -367.2620300519063790 ) ) ;
#44077=CARTESIAN_POINT ( 'NONE',  ( 784.0799538623451781, -11.80559628986942577, -364.6971507214555572 ) ) ;
#44079=CARTESIAN_POINT ( 'NONE',  ( 793.9861285913068514, -442.9180389616178672, -372.1637643035757606 ) ) ;
#44084=CARTESIAN_POINT ( 'NONE',  ( 799.9636004259356241, -382.9181544815159555, -311.2241431872006956 ) ) ;
#44085=EDGE_CURVE ( 'NONE', #21104, #27172, #23023, .T. ) ;
#44089=CARTESIAN_POINT ( 'NONE',  ( 754.7162404726377645, -230.7363362996981664, -339.4709603349214717 ) ) ;
#44090=CARTESIAN_POINT ( 'NONE',  ( 797.8594530101008786, -229.5436935675106440, -322.1405469898980982 ) ) ;
#44091=CARTESIAN_POINT ( 'NONE',  ( 794.9819416627830151, -396.9982390220556567, -319.9864689768909898 ) ) ;
#44094=CARTESIAN_POINT ( 'NONE',  ( 774.6858677611749044, -105.7255117493293000, -315.5713283507209894 ) ) ;
#44104=CARTESIAN_POINT ( 'NONE',  ( 814.2805881961230625, -433.6454272087884760, -331.2368401574024119 ) ) ;
#44105=CARTESIAN_POINT ( 'NONE',  ( 745.0891759886404770, -28.27096629478409540, -342.4968714119734159 ) ) ;
#44107=CARTESIAN_POINT ( 'NONE',  ( 795.1360043628807261, -380.0891481129646650, -360.2193346964456282 ) ) ;
#44108=CARTESIAN_POINT ( 'NONE',  ( 756.3353852180820240, -5.907329931147799584, -331.1735550268787733 ) ) ;
#44111=CARTESIAN_POINT ( 'NONE',  ( 760.7433823573367135, -276.0090635724253048, -355.9930595647440441 ) ) ;
#44112=CARTESIAN_POINT ( 'NONE',  ( 763.2262854647970016, -152.6346026584200786, -309.2812353651462445 ) ) ;
#44116=LINE ( 'NONE', #2297, #41659 ) ;
#44119=CARTESIAN_POINT ( 'NONE',  ( 803.6646147819161570, -353.9073299311467053, -348.8264449731210561 ) ) ;
#44121=CARTESIAN_POINT ( 'NONE',  ( 791.0478386215596629, -93.82724539060770041, -306.7653713866226326 ) ) ;
#44122=CARTESIAN_POINT ( 'NONE',  ( 805.1016975059191054, -102.8965053807782368, -343.0745993439771837 ) ) ;
#44126=CARTESIAN_POINT ( 'NONE',  ( 804.9363028652555840, -40.27096629478405987, -338.2165204200192079 ) ) ;
#44127=CARTESIAN_POINT ( 'NONE',  ( 799.4546378042377910, -129.0783235625963243, -356.1575198192848006 ) ) ;
#44128=CARTESIAN_POINT ( 'NONE',  ( 804.4286716492782716, -137.3618753856928265, -345.3141322388244703 ) ) ;
#44131=CARTESIAN_POINT ( 'NONE',  ( 808.7758568127978833, 19.83076734649410966, -320.0363995740631822 ) ) ;
#44137=CARTESIAN_POINT ( 'NONE',  ( 776.2046728542105711, -260.1908817542435486, -304.8212110874238761 ) ) ;
#44138=EDGE_LOOP ( 'NONE', ( #38952, #34383 ) ) ;
#44145=CARTESIAN_POINT ( 'NONE',  ( 801.5560724626406000, -120.5545181178803205, -326.7756240680316182 ) ) ;
#44146=CARTESIAN_POINT ( 'NONE',  ( 765.0180583372156207, -120.9982390220565378, -360.0135310231089534 ) ) ;
#44147=CARTESIAN_POINT ( 'NONE',  ( 774.6858677611749044, -297.7255117493286889, -315.5713283507209894 ) ) ;
#44149=CARTESIAN_POINT ( 'NONE',  ( 804.9363028652555840, -424.2709662947829088, -338.2165204200192079 ) ) ;
#44150=CARTESIAN_POINT ( 'NONE',  ( 768.0187753319979720, -80.63460265842029173, -318.0580252608186242 ) ) ;
#44156=CARTESIAN_POINT ( 'NONE',  ( 799.9636004259356241, -334.9181544815160692, -311.2241431872006956 ) ) ;
#44160=DIRECTION ( 'NONE',  ( 0.000000000000000000, 0.000000000000000000, -1.000000000000000000 ) ) ;
#44161=CARTESIAN_POINT ( 'NONE',  ( 788.7366044899766848, -299.9073299311468759, -316.5762568750059813 ) ) ;
#44163=DIRECTION ( 'NONE',  ( -1.000000000000000000, -0.000000000000000000, -0.000000000000000000 ) ) ;
#44164=CARTESIAN_POINT ( 'NONE',  ( 804.4086373105744769, -193.6454272087891582, -333.3843516231986541 ) ) ;
#44168=CARTESIAN_POINT ( 'NONE',  ( 772.5602148656447525, -369.7255117493284615, -305.7998596910095443 ) ) ;
#44173=CARTESIAN_POINT ( 'NONE',  ( 749.2812353651451076, -30.45278447660226817, -323.2262854647983090 ) ) ;
#44178=CARTESIAN_POINT ( 'NONE',  ( 776.9566956441375396, -12.89650538077851216, -364.8461984189686405 ) ) ;
#44185=CARTESIAN_POINT ( 'NONE',  ( 801.9419747391806368, -42.45278447660223264, -351.9812246680014027 ) ) ;
#44187=CARTESIAN_POINT ( 'NONE',  ( 760.5453621957607311, -333.0783235625956991, -323.8424801807151425 ) ) ;
#44190=CARTESIAN_POINT ( 'NONE',  ( 756.1443688327750579, -333.6237781080502600, -314.3581564841659315 ) ) ;
#44200=CARTESIAN_POINT ( 'NONE',  ( 811.0346526505616112, -182.6346026584199649, -323.0537975583477532 ) ) ;
#44203=CARTESIAN_POINT ( 'NONE',  ( 803.6646147819162707, -185.9073299311472169, -348.8264449731211130 ) ) ;
#44205=CARTESIAN_POINT ( 'NONE',  ( 805.2837595273609850, -458.7363362996973706, -340.5290396650784714 ) ) ;
#44212=CARTESIAN_POINT ( 'NONE',  ( 769.0155153010367712, -418.3726999360612808, -362.7791456095907279 ) ) ;
#44214=ORIENTED_EDGE ( 'NONE', *, *, #12264, .F. ) ;
#44215=CARTESIAN_POINT ( 'NONE',  ( 747.6481478633932056, -229.0999726633345404, -353.4146539503763620 ) ) ;
#44218=CARTESIAN_POINT ( 'NONE',  ( 804.9363028652555840, -184.2709662947835909, -338.2165204200192079 ) ) ;
#44219=CARTESIAN_POINT ( 'NONE',  ( 787.6308680596127942, -347.2601417444138860, -364.1105419155492768 ) ) ;
#44221=CARTESIAN_POINT ( 'NONE',  ( 745.5313806188320314, -231.2817908451527558, -333.7943932421247268 ) ) ;
#44224=CARTESIAN_POINT ( 'NONE',  ( 755.1538015810308480, -62.19088175424416676, -343.0433043558613804 ) ) ;
#44227=CARTESIAN_POINT ( 'NONE',  ( 763.2154366446407039, -429.6237781080499190, -321.4292242960311228 ) ) ;
#44228=CARTESIAN_POINT ( 'NONE',  ( 751.6929314249750860, -270.9982390220561115, -318.8095938919659034 ) ) ;
#44232=CARTESIAN_POINT ( 'NONE',  ( 762.1405469898971887, -49.54369356751129061, -357.8594530101015607 ) ) ;
#44235=CARTESIAN_POINT ( 'NONE',  ( 783.7566961878529810, -144.8965053807781089, -305.1792804349288417 ) ) ;
#44237=CARTESIAN_POINT ( 'NONE',  ( 805.0032342141412300, -397.5436935675100472, -314.9967657858571783 ) ) ;
#44241=CARTESIAN_POINT ( 'NONE',  ( 785.3141322388236176, -405.7255117493283478, -364.4286716492789537 ) ) ;
#44244=CARTESIAN_POINT ( 'NONE',  ( 757.7880784355613741, -18.00906357242611477, -312.4576283171834916 ) ) ;
#44248=CARTESIAN_POINT ( 'NONE',  ( 755.0488828828309806, -233.8055962898687028, -344.1219089521771934 ) ) ;
#44249=CARTESIAN_POINT ( 'NONE',  ( 764.8639956371174549, -128.0891481129655176, -319.7806653035542013 ) ) ;
#44251=CARTESIAN_POINT ( 'NONE',  ( 803.8556311672234642, -225.6237781080506011, -365.6418435158340117 ) ) ;
#44256=CARTESIAN_POINT ( 'NONE',  ( 804.4286716492782716, -185.3618753856926844, -345.3141322388244703 ) ) ;
#44259=CARTESIAN_POINT ( 'NONE',  ( 796.7737145352015204, -68.63460265842033436, -370.7187646348536987 ) ) ;
#44260=CARTESIAN_POINT ( 'NONE',  ( 756.3353852180820240, -77.90732993114757221, -331.1735550268787733 ) ) ;
#44262=CARTESIAN_POINT ( 'NONE',  ( 802.5472867521000353, -4.372699936062523385, -350.8726784830461156 ) ) ;
#44264=CARTESIAN_POINT ( 'NONE',  ( 769.0155153010367712, -370.3726999360613377, -362.7791456095907279 ) ) ;
#44271=CARTESIAN_POINT ( 'NONE',  ( 804.1105419155481968, -339.8272453906069472, -347.6308680596136469 ) ) ;
#44272=CARTESIAN_POINT ( 'NONE',  ( 754.8072714833581358, -316.8164208402377540, -338.1981804954720587 ) ) ;
#44273=CARTESIAN_POINT ( 'NONE',  ( 781.8018195045266339, -166.2709662947835909, -365.1927285166406705 ) ) ;
#44277=CARTESIAN_POINT ( 'NONE',  ( 764.0069404352550464, -255.0783235625958980, -359.2566176426627180 ) ) ;
#44278=CARTESIAN_POINT ( 'NONE',  ( 748.6759233522253680, -112.3726999360621761, -324.3348316497537098 ) ) ;
#44283=EDGE_LOOP ( 'NONE', ( #34481, #44787, #2807, #34075 ) ) ;
#44285=CARTESIAN_POINT ( 'NONE',  ( 787.5162901302840055, -155.3618753856927697, -305.4481719005793252 ) ) ;
#44288=CARTESIAN_POINT ( 'NONE',  ( 811.0346526505616112, -254.6346026584196238, -323.0537975583477532 ) ) ;
#44293=CARTESIAN_POINT ( 'NONE',  ( 744.8212110874229666, -354.8965053807774552, -336.2046728542121627 ) ) ;
#44294=CARTESIAN_POINT ( 'NONE',  ( 812.7932403749906598, -87.18005720387481006, -327.7687537140311633 ) ) ;
#44296=CARTESIAN_POINT ( 'NONE',  ( 777.4774526936600978, -346.2709662947830793, -304.7301800767027657 ) ) ;
#44301=CARTESIAN_POINT ( 'NONE',  ( 744.8212110874229666, -114.8965053807782226, -336.2046728542121627 ) ) ;
#44305=ORIENTED_EDGE ( 'NONE', *, *, #29910, .T. ) ;
#44307=CARTESIAN_POINT ( 'NONE',  ( 757.2208543904082489, -16.71468719896031985, -350.9844846989624330 ) ) ;
#44309=CARTESIAN_POINT ( 'NONE',  ( 746.7653713866222915, -425.2601417444136018, -351.0478386215610271 ) ) ;
#44313=CARTESIAN_POINT ( 'NONE',  ( 810.4231160770870019, -360.5545181178796383, -321.9338519418446936 ) ) ;
#44317=CARTESIAN_POINT ( 'NONE',  ( 757.4527132478984868, -208.3726999360619061, -329.1273215169538844 ) ) ;
#44318=CARTESIAN_POINT ( 'NONE',  ( 800.0135310231082713, -230.0891481129652618, -325.0180583372163028 ) ) ;
#44319=CARTESIAN_POINT ( 'NONE',  ( 805.1927285166399315, -424.8164208402373561, -341.8018195045277707 ) ) ;
#44322=CARTESIAN_POINT ( 'NONE',  ( 756.5762568750052424, -99.18005720387478164, -348.7366044899774238 ) ) ;
#44325=CARTESIAN_POINT ( 'NONE',  ( 793.2534793918160858, 16.75597696963228955, -312.9842977579731382 ) ) ;
#44331=CARTESIAN_POINT ( 'NONE',  ( 794.5607502887775127, -462.9631818684622999, -371.8524697363486666 ) ) ;
#44332=CARTESIAN_POINT ( 'NONE',  ( 747.2067596250078623, -27.18005720387500901, -352.2312462859687230 ) ) ;
#44334=CARTESIAN_POINT ( 'NONE',  ( 764.8639956371174549, -392.0891481129648355, -319.7806653035542013 ) ) ;
#44335=CARTESIAN_POINT ( 'NONE',  ( 778.1981804954715471, -10.27096629478415046, -314.8072714833591021 ) ) ;
#44338=CARTESIAN_POINT ( 'NONE',  ( 780.5236548040995785, -284.7363362996979390, -314.9735926884559944 ) ) ;
#44339=CARTESIAN_POINT ( 'NONE',  ( 772.4837098697144029, -167.3618753856927412, -374.5518280994205611 ) ) ;
#44344=CARTESIAN_POINT ( 'NONE',  ( 791.1614460488616487, -227.2601417444141987, -373.5763878283158874 ) ) ;
#44348=CARTESIAN_POINT ( 'NONE',  ( 804.4286716492782716, -353.3618753856922012, -345.3141322388244703 ) ) ;
#44350=CARTESIAN_POINT ( 'NONE',  ( 757.7880784355613741, -114.0090635724258163, -312.4576283171834916 ) ) ;
#44351=CARTESIAN_POINT ( 'NONE',  ( 804.9511171171677688, -149.8055962898689870, -335.8780910478229202 ) ) ;
#44354=CARTESIAN_POINT ( 'NONE',  ( 800.0135310231082713, -62.08914811296580183, -325.0180583372163028 ) ) ;
#44355=CARTESIAN_POINT ( 'NONE',  ( 780.5290396650775619, -156.3510508353235480, -365.2837595273619513 ) ) ;
#44356=CARTESIAN_POINT ( 'NONE',  ( 754.8072714833581358, -124.8164208402383508, -338.1981804954720587 ) ) ;
#44358=CARTESIAN_POINT ( 'NONE',  ( 812.6845335610512393, -7.987414471687621642, -353.5525998758768651 ) ) ;
#44365=CARTESIAN_POINT ( 'NONE',  ( 810.4231160770870019, -264.5545181178798657, -321.9338519418446936 ) ) ;
#44372=CARTESIAN_POINT ( 'NONE',  ( 798.5707757039680246, -101.4636090269713264, -356.7845633553585003 ) ) ;
#44373=CARTESIAN_POINT ( 'NONE',  ( 805.1927285166397041, -112.8164208402383508, -341.8018195045277707 ) ) ;
#44374=CARTESIAN_POINT ( 'NONE',  ( 762.3223304703356007, -319.5436935675104451, -322.3223304703362828 ) ) ;
#44376=CARTESIAN_POINT ( 'NONE',  ( 765.0180583372156207, -432.9982390220555999, -360.0135310231089534 ) ) ;
#44377=CARTESIAN_POINT ( 'NONE',  ( 804.4286716492782716, -89.36187538569299704, -345.3141322388244703 ) ) ;
#44379=DIRECTION ( 'NONE',  ( 0.000000000000000000, -0.000000000000000000, -1.000000000000000000 ) ) ;
#44383=CARTESIAN_POINT ( 'NONE',  ( 807.2620300519052989, -336.0090635724251911, -318.0141637701419768 ) ) ;
#44385=CARTESIAN_POINT ( 'NONE',  ( 788.8264449731200330, -285.1800572038740711, -363.6646147819171233 ) ) ;
#44387=CARTESIAN_POINT ( 'NONE',  ( 804.1105419155481968, -171.8272453906074304, -347.6308680596136469 ) ) ;
#44392=CARTESIAN_POINT ( 'NONE',  ( 810.7187646348534145, -378.4527844766011526, -356.7737145352016341 ) ) ;
#44397=CARTESIAN_POINT ( 'NONE',  ( 747.2067596250078623, -3.180057203875080063, -352.2312462859687230 ) ) ;
#44399=CARTESIAN_POINT ( 'NONE',  ( 800.0135310231082713, -254.0891481129652334, -325.0180583372163028 ) ) ;
#44403=CARTESIAN_POINT ( 'NONE',  ( 766.7756240680305382, -38.53286901714206891, -361.5560724626415663 ) ) ;
#44410=CARTESIAN_POINT ( 'NONE',  ( 798.7617431975189675, -315.6237781080503169, -323.0428371773161871 ) ) ;
#44414=CARTESIAN_POINT ( 'NONE',  ( 744.9990715423526808, -354.3510508353228943, -341.2370466360926002 ) ) ;
#44421=CARTESIAN_POINT ( 'NONE',  ( 751.6929314249748586, -222.9982390220561399, -318.8095938919659034 ) ) ;
#44423=ORIENTED_EDGE ( 'NONE', *, *, #24119, .F. ) ;
#44424=CARTESIAN_POINT ( 'NONE',  ( 795.1360043628808398, -164.0891481129654892, -360.2193346964456282 ) ) ;
#44426=CARTESIAN_POINT ( 'NONE',  ( 800.2193346964447755, -330.9982390220558273, -355.1360043628815788 ) ) ;
#44427=CARTESIAN_POINT ( 'NONE',  ( 787.5531968255692163, -453.8272453906066630, -316.1348686366205811 ) ) ;
#44434=CARTESIAN_POINT ( 'NONE',  ( 779.4763451958990572, -416.7363362996975980, -365.0264073115438919 ) ) ;
#44435=DIRECTION ( 'NONE',  ( -0.000000000000000000, 1.000000000000000000, -1.110223024625155554E-15 ) ) ;
#44438=CARTESIAN_POINT ( 'NONE',  ( 773.7305795820266212, -249.2817908451526421, -374.8230680027170365 ) ) ;
#44441=CARTESIAN_POINT ( 'NONE',  ( 755.0636971347428243, -196.2709662947835909, -341.7834795799807353 ) ) ;
#44443=CARTESIAN_POINT ( 'NONE',  ( 795.9930595647434757, -363.0783235625955854, -320.7433823573372820 ) ) ;
#44445=CARTESIAN_POINT ( 'NONE',  ( 771.3260364891663130, -235.6454272087890729, -306.0683387631859773 ) ) ;
#44448=CARTESIAN_POINT ( 'NONE',  ( 763.8424801807145741, -90.00906357242590161, -320.5453621957614700 ) ) ;
#44453=CARTESIAN_POINT ( 'NONE',  ( 784.0799538623451781, -419.8055962898681059, -364.6971507214555572 ) ) ;
#44454=CARTESIAN_POINT ( 'NONE',  ( 796.9462024416508257, -276.4527844766014368, -308.9653473494370246 ) ) ;
#44457=CARTESIAN_POINT ( 'NONE',  ( 778.1981804954714335, -34.27096629478407408, -314.8072714833589885 ) ) ;
#44459=CARTESIAN_POINT ( 'NONE',  ( 744.8212110874229666, -162.8965053807780521, -336.2046728542121627 ) ) ;
#44461=CARTESIAN_POINT ( 'NONE',  ( 744.7301800767019131, -412.8164208402372992, -337.4774526936615757 ) ) ;
#44467=CARTESIAN_POINT ( 'NONE',  ( 794.9819416627830151, -396.9982390220556567, -319.9864689768909898 ) ) ;
#44471=ORIENTED_EDGE ( 'NONE', *, *, #43665, .F. ) ;
#44472=CARTESIAN_POINT ( 'NONE',  ( 796.7845633553578182, -225.6237781080506011, -358.5707757039688204 ) ) ;
#44473=CARTESIAN_POINT ( 'NONE',  ( 765.0180583372156207, -120.9982390220565378, -360.0135310231089534 ) ) ;
#44475=CARTESIAN_POINT ( 'NONE',  ( 773.7943932421234194, -263.8055962898686175, -305.5313806188329409 ) ) ;
#44481=CARTESIAN_POINT ( 'NONE',  ( 800.2193346964447755, -186.9982390220563104, -355.1360043628815788 ) ) ;
#44483=CARTESIAN_POINT ( 'NONE',  ( 782.5225473063381969, -94.27096629478386092, -375.2698199232970637 ) ) ;
#44485=CARTESIAN_POINT ( 'NONE',  ( 794.9819416627830151, -84.99823902205663728, -319.9864689768909898 ) ) ;
#44487=CARTESIAN_POINT ( 'NONE',  ( 802.9823548866075953, -25.09997266333519050, -330.0799878456151077 ) ) ;
#44489=CARTESIAN_POINT ( 'NONE',  ( 804.6971507214547046, -363.2817908451523294, -344.0799538623459739 ) ) ;
#44494=CARTESIAN_POINT ( 'NONE',  ( 789.5584187865343893, -452.9681489794450613, -363.1011989789364520 ) ) ;
#44496=CARTESIAN_POINT ( 'NONE',  ( 796.1575198192839480, -318.0090635724251911, -359.4546378042384163 ) ) ;
#44497=CARTESIAN_POINT ( 'NONE',  ( 791.0478386215596629, -117.8272453906076151, -306.7653713866226326 ) ) ;
#44502=LINE ( 'NONE', #37347, #7894 ) ;
#44504=CARTESIAN_POINT ( 'NONE',  ( 803.8651313633788504, -269.2601417444139997, -332.4468031744301015 ) ) ;
#44505=CARTESIAN_POINT ( 'NONE',  ( 747.6481478633932056, -109.0999726633349241, -353.4146539503763620 ) ) ;
#44507=LINE ( 'NONE', #26949, #31163 ) ;
#44513=CARTESIAN_POINT ( 'NONE',  ( 804.7487373415286811, -163.5436935675109567, -364.7487373415288516 ) ) ;
#44516=CARTESIAN_POINT ( 'NONE',  ( 744.7301800767019131, -292.8164208402376971, -337.4774526936615757 ) ) ;
#44517=DIRECTION ( 'NONE',  ( -0.000000000000000000, 1.000000000000000000, -0.000000000000000000 ) ) ;
#44520=VECTOR ( 'NONE', #19569, 1000.000000000000000 ) ;
#44523=CARTESIAN_POINT ( 'NONE',  ( 766.5853460496234675, -325.9874144716865771, -372.3518521366060554 ) ) ;
#44525=CARTESIAN_POINT ( 'NONE',  ( 751.6929314249748586, -102.9982390220565520, -318.8095938919659034 ) ) ;
#44527=CARTESIAN_POINT ( 'NONE',  ( 759.0252816721024374, -384.9982390220556567, -368.0189434323527280 ) ) ;
#44532=CARTESIAN_POINT ( 'NONE',  ( 783.7566961878529810, -168.8965053807780237, -305.1792804349288417 ) ) ;
#44538=CARTESIAN_POINT ( 'NONE',  ( 754.8983024940795303, 5.103494619221427442, -336.9254006560228163 ) ) ;
#44540=CARTESIAN_POINT ( 'NONE',  ( 778.7502325331095108, -432.3510508353226669, -304.6391490659818828 ) ) ;
#44544=CARTESIAN_POINT ( 'NONE',  ( 814.4686193811664907, -387.2817908451522726, -346.2056067578752732 ) ) ;
#44545=CARTESIAN_POINT ( 'NONE',  ( 759.9864689768902508, -242.0891481129652618, -354.9819416627836404 ) ) ;
#44548=CARTESIAN_POINT ( 'NONE',  ( 755.3028492785439312, -231.2817908451527558, -335.9200461376539693 ) ) ;
#44549=CARTESIAN_POINT ( 'NONE',  ( 800.2193346964447755, -234.9982390220561683, -355.1360043628815788 ) ) ;
#44551=CARTESIAN_POINT ( 'NONE',  ( 785.3687786644885591, -419.3618753856918602, -315.3201227861280813 ) ) ;
#44555=CARTESIAN_POINT ( 'NONE',  ( 755.0636971347428243, -100.2709662947838609, -341.7834795799807353 ) ) ;
#44564=CARTESIAN_POINT ( 'NONE',  ( 797.8822607201568644, -438.5545181178793541, -370.1134526219340160 ) ) ;
#44565=CARTESIAN_POINT ( 'NONE',  ( 796.7737145352015204, -68.63460265842033436, -370.7187646348536987 ) ) ;
#44567=CARTESIAN_POINT ( 'NONE',  ( 797.8594530101008786, -421.5436935675101040, -322.1405469898980982 ) ) ;
#44568=CARTESIAN_POINT ( 'NONE',  ( 785.3141322388236176, -45.72551174932949181, -364.4286716492789537 ) ) ;
#44572=CARTESIAN_POINT ( 'NONE',  ( 800.9840315886518738, -292.9181544815162397, -354.1144889064786412 ) ) ;
#44573=CARTESIAN_POINT ( 'NONE',  ( 772.5602148656447525, -201.7255117493290015, -305.7998596910095443 ) ) ;
#44579=CARTESIAN_POINT ( 'NONE',  ( 746.7653713866222915, -233.2601417444141987, -351.0478386215610271 ) ) ;
#44581=CARTESIAN_POINT ( 'NONE',  ( 746.8695393053150156, -293.9073299311468759, -327.6429770376306010 ) ) ;
#44585=CARTESIAN_POINT ( 'NONE',  ( 805.1927285166397041, -352.8164208402374129, -341.8018195045277707 ) ) ;
#44586=AXIS2_PLACEMENT_3D ( 'NONE', #1334, #16731, #29516 ) ;
#44589=CARTESIAN_POINT ( 'NONE',  ( 776.2046728542105711, -92.19088175424406018, -304.8212110874238761 ) ) ;
#44590=CARTESIAN_POINT ( 'NONE',  ( 786.6156483768007774, -169.4419599262325562, -315.5913626894246136 ) ) ;
#44594=CARTESIAN_POINT ( 'NONE',  ( 759.7806653035534055, -54.99823902205672255, -324.8639956371180801 ) ) ;
#44595=CARTESIAN_POINT ( 'NONE',  ( 801.3366627262608972, -152.5328690171416781, -353.0897708529566899 ) ) ;
#44597=CARTESIAN_POINT ( 'NONE',  ( 754.0944755984390895, 8.376221891948691933, -364.1009440267246760 ) ) ;
#44602=CARTESIAN_POINT ( 'NONE',  ( 757.7880784355613741, -282.0090635724253048, -312.4576283171834916 ) ) ;
#44610=CARTESIAN_POINT ( 'NONE',  ( 772.4468031744293057, -105.8272453906076578, -363.8651313633793620 ) ) ;
#44611=CARTESIAN_POINT ( 'NONE',  ( 754.8072714833581358, -100.8164208402383792, -338.1981804954720587 ) ) ;
#44612=CARTESIAN_POINT ( 'NONE',  ( 803.6646147819162707, -329.9073299311467622, -348.8264449731211130 ) ) ;
#44614=CARTESIAN_POINT ( 'NONE',  ( 771.1735550268778070, -441.1800572038735027, -316.3353852180827630 ) ) ;
#44620=EDGE_LOOP ( 'NONE', ( #20798, #20023, #13489, #33341 ) ) ;
#44621=CARTESIAN_POINT ( 'NONE',  ( 744.6391490659812007, -350.7363362996978253, -338.7502325331110455 ) ) ;
#44623=CIRCLE ( 'NONE', #35025, 30.00000000000008171 ) ;
#44624=CARTESIAN_POINT ( 'NONE',  ( 781.8018195045266339, -334.2709662947829656, -365.1927285166406705 ) ) ;
#44625=CARTESIAN_POINT ( 'NONE',  ( 805.2837595273609850, -170.7363362996983938, -340.5290396650784714 ) ) ;
#44628=CARTESIAN_POINT ( 'NONE',  ( 804.7487373415286811, -379.5436935675102745, -364.7487373415288516 ) ) ;
#44630=AXIS2_PLACEMENT_3D ( 'NONE', #41703, #11194, #31965 ) ;
#44634=CARTESIAN_POINT ( 'NONE',  ( 772.5602148656447525, -9.725511749329603717, -305.7998596910095443 ) ) ;
#44635=CARTESIAN_POINT ( 'NONE',  ( 788.7366044899766848, -251.9073299311470748, -316.5762568750059813 ) ) ;
#44642=CARTESIAN_POINT ( 'NONE',  ( 755.8398074228967971, -67.44195992623289726, -333.4516893846970333 ) ) ;
#44648=CARTESIAN_POINT ( 'NONE',  ( 767.8955696845333705, -72.45278447660213317, -362.1676090361162323 ) ) ;
#44649=CARTESIAN_POINT ( 'NONE',  ( 775.9200461376533440, -359.8055962898683333, -315.3028492785443291 ) ) ;
#44653=CARTESIAN_POINT ( 'NONE',  ( 752.4576283171824116, -357.0783235625956422, -317.7880784355627952 ) ) ;
#44659=CARTESIAN_POINT ( 'NONE',  ( 805.0032342141412300, -205.5436935675108430, -314.9967657858571783 ) ) ;
#44661=ORIENTED_EDGE ( 'NONE', *, *, #21559, .T. ) ;
#44662=CARTESIAN_POINT ( 'NONE',  ( 785.3687786644885591, -203.3618753856926276, -315.3201227861280813 ) ) ;
#44664=CARTESIAN_POINT ( 'NONE',  ( 755.3201227861273992, -339.7255117493285184, -345.3687786644892981 ) ) ;
#44665=CARTESIAN_POINT ( 'NONE',  ( 802.5472867521000353, -460.3726999360611103, -350.8726784830461156 ) ) ;
#44675=ORIENTED_EDGE ( 'NONE', *, *, #13697, .F. ) ;
#44676=CARTESIAN_POINT ( 'NONE',  ( 773.4516893846965786, -451.6454272087884192, -315.8398074228977066 ) ) ;
#44678=LINE ( 'NONE', #37514, #41072 ) ;
#44680=CARTESIAN_POINT ( 'NONE',  ( 783.7953271457878373, -224.1908817542436623, -375.1787889125761239 ) ) ;
#44683=CARTESIAN_POINT ( 'NONE',  ( 794.9819416627830151, -180.9982390220563389, -319.9864689768909898 ) ) ;
#44684=CARTESIAN_POINT ( 'NONE',  ( 776.9566956441375396, -372.8965053807773415, -364.8461984189686405 ) ) ;
#44685=CARTESIAN_POINT ( 'NONE',  ( 814.8207195650702488, -242.1908817542435770, -336.2433038121456548 ) ) ;
#44686=CARTESIAN_POINT ( 'NONE',  ( 787.4999999999992042, -512.9681489794448908, -339.9999999999999432 ) ) ;
#44688=CARTESIAN_POINT ( 'NONE',  ( 759.0159684113467620, -88.91815448151682233, -325.8855110935213020 ) ) ;
#44692=CARTESIAN_POINT ( 'NONE',  ( 795.9930595647434757, -435.0783235625953580, -320.7433823573372820 ) ) ;
#44693=CARTESIAN_POINT ( 'NONE',  ( 759.0252816721024374, -264.9982390220561115, -368.0189434323527280 ) ) ;
#44696=CARTESIAN_POINT ( 'NONE',  ( 802.1676090361156639, -38.63460265842041252, -327.8955696845344505 ) ) ;
#44698=CARTESIAN_POINT ( 'NONE',  ( 744.9990715423526808, -162.3510508353235196, -341.2370466360926002 ) ) ;
#44700=CARTESIAN_POINT ( 'NONE',  ( 758.8095938919642549, -392.0891481129648355, -311.6929314249763365 ) ) ;
#44705=CARTESIAN_POINT ( 'NONE',  ( 804.9363028652555840, -424.2709662947829088, -338.2165204200192079 ) ) ;
#44713=CARTESIAN_POINT ( 'NONE',  ( 757.2208543904082489, -256.7146871989595525, -350.9844846989624330 ) ) ;
#44715=CARTESIAN_POINT ( 'NONE',  ( 788.7631598425961101, -265.4419599262323004, -305.7194118038759143 ) ) ;
#44721=CARTESIAN_POINT ( 'NONE',  ( 774.6858677611749044, -177.7255117493290868, -315.5713283507209894 ) ) ;
#44724=CARTESIAN_POINT ( 'NONE',  ( 804.7487373415286811, -115.5436935675110988, -364.7487373415288516 ) ) ;
#44725=CARTESIAN_POINT ( 'NONE',  ( 788.7366044899766848, -107.9073299311474727, -316.5762568750059813 ) ) ;
#44727=CARTESIAN_POINT ( 'NONE',  ( 754.7162404726377645, -38.73633629969877035, -339.4709603349214717 ) ) ;
#44729=CARTESIAN_POINT ( 'NONE',  ( 798.5707757039680246, -365.4636090269705164, -356.7845633553585003 ) ) ;
#44740=CARTESIAN_POINT ( 'NONE',  ( 799.2566176426618085, -360.0090635724250774, -324.0069404352559559 ) ) ;
#44741=CARTESIAN_POINT ( 'NONE',  ( 778.2165204200184689, -334.8164208402376403, -364.9363028652563230 ) ) ;
#44742=CARTESIAN_POINT ( 'NONE',  ( 791.0478386215596629, -141.8272453906075157, -306.7653713866226326 ) ) ;
#44746=CARTESIAN_POINT ( 'NONE',  ( 780.5290396650775619, -252.3510508353232353, -365.2837595273619513 ) ) ;
#44747=CARTESIAN_POINT ( 'NONE',  ( 814.2805881961230625, -121.6454272087894282, -331.2368401574024119 ) ) ;
#44754=CARTESIAN_POINT ( 'NONE',  ( 811.0346526505617248, -158.6346026584200217, -323.0537975583478101 ) ) ;
#44759=CARTESIAN_POINT ( 'NONE',  ( 746.8695393053150156, -293.9073299311468759, -327.6429770376306010 ) ) ;
#44760=CARTESIAN_POINT ( 'NONE',  ( 799.9999999999993179, 205.0000000000000568, -350.0000000000000000 ) ) ;
#44765=CARTESIAN_POINT ( 'NONE',  ( 798.0661480581538854, -386.5328690171409676, -309.5768839229118043 ) ) ;
#44766=CARTESIAN_POINT ( 'NONE',  ( 777.5031285880264704, -118.8164208402383508, -374.9108240113588408 ) ) ;
#44768=CARTESIAN_POINT ( 'NONE',  ( 814.5518280994195948, -375.7255117493283478, -332.4837098697145734 ) ) ;
#44769=DIRECTION ( 'NONE',  ( 0.000000000000000000, -1.000000000000000000, 0.000000000000000000 ) ) ;
#44774=CARTESIAN_POINT ( 'NONE',  ( 808.7758568127978833, -172.1692326535052757, -320.0363995740631822 ) ) ;
#44781=CARTESIAN_POINT ( 'NONE',  ( 756.1348686366196716, -17.26014174441486659, -347.5531968255698416 ) ) ;
#44785=CARTESIAN_POINT ( 'NONE',  ( 751.6929314249748586, -6.998239022056885972, -318.8095938919659034 ) ) ;
#44787=ORIENTED_EDGE ( 'NONE', *, *, #1300, .T. ) ;
#44789=CARTESIAN_POINT ( 'NONE',  ( 781.2370466360911223, -428.7363362996975980, -304.9990715423533629 ) ) ;
#44792=CARTESIAN_POINT ( 'NONE',  ( 801.5560724626406000, -216.5545181178800931, -326.7756240680316182 ) ) ;
#44793=CARTESIAN_POINT ( 'NONE',  ( 771.1735550268778070, -201.1800572038744690, -316.3353852180827630 ) ) ;
#44794=CARTESIAN_POINT ( 'NONE',  ( 792.1044303154646968, -420.4527844766009821, -317.8323909638837677 ) ) ;
#44799=CARTESIAN_POINT ( 'NONE',  ( 748.6759233522253680, -16.37269993606248519, -324.3348316497537098 ) ) ;
#44805=CARTESIAN_POINT ( 'NONE',  ( 783.7953271457878373, -440.1908817542430370, -375.1787889125761239 ) ) ;
#44806=CARTESIAN_POINT ( 'NONE',  ( 749.2812353651451076, -54.45278447660219001, -323.2262854647983090 ) ) ;
#44808=CARTESIAN_POINT ( 'NONE',  ( 755.3201227861273992, -435.7255117493282341, -345.3687786644892981 ) ) ;
#44809=CARTESIAN_POINT ( 'NONE',  ( 781.8018195045267476, -46.27096629478403855, -365.1927285166407273 ) ) ;
#44812=CARTESIAN_POINT ( 'NONE',  ( 772.4468031744293057, -297.8272453906070041, -363.8651313633793620 ) ) ;
#44813=CARTESIAN_POINT ( 'NONE',  ( 796.7737145352015204, -212.6346026584198796, -370.7187646348536987 ) ) ;
#44818=CARTESIAN_POINT ( 'NONE',  ( 813.9316612368132837, -247.4419599262323004, -348.6739635108323228 ) ) ;
#44820=CARTESIAN_POINT ( 'NONE',  ( 758.8095938919642549, -272.0891481129651197, -311.6929314249763365 ) ) ;
#44824=CARTESIAN_POINT ( 'NONE',  ( 759.9864689768902508, -362.0891481129648923, -354.9819416627836404 ) ) ;
#44826=CARTESIAN_POINT ( 'NONE',  ( 754.0944755984390895, -63.62377810805107714, -364.1009440267246760 ) ) ;
#44827=CARTESIAN_POINT ( 'NONE',  ( 757.2208543904082489, -160.7146871989598651, -350.9844846989624330 ) ) ;
#44831=CARTESIAN_POINT ( 'NONE',  ( 771.1735550268778070, -57.18005720387489532, -316.3353852180827630 ) ) ;
#44832=CARTESIAN_POINT ( 'NONE',  ( 799.4546378042377910, -177.0783235625961538, -356.1575198192848006 ) ) ;
#44834=CARTESIAN_POINT ( 'NONE',  ( 815.1787889125755555, 17.10349461922139369, -343.7953271457877804 ) ) ;
#44839=CARTESIAN_POINT ( 'NONE',  ( 762.1177392798416577, -282.5545181178798657, -309.8865473780659272 ) ) ;
#44846=CARTESIAN_POINT ( 'NONE',  ( 796.1575198192839480, -102.0090635724258448, -359.4546378042384163 ) ) ;
#44847=CARTESIAN_POINT ( 'NONE',  ( 756.3353852180819104, -101.9073299311474727, -331.1735550268788302 ) ) ;
#44848=CARTESIAN_POINT ( 'NONE',  ( 797.6776695296629214, -331.5436935675104451, -357.6776695296636603 ) ) ;
#44850=CARTESIAN_POINT ( 'NONE',  ( 774.6858677611749044, -441.7255117493282910, -315.5713283507209894 ) ) ;
#44857=CARTESIAN_POINT ( 'NONE',  ( 746.4236121716829757, -351.8272453906068336, -328.8385539511384650 ) ) ;
#44859=CARTESIAN_POINT ( 'NONE',  ( 781.7834795799800531, -322.8164208402377540, -315.0636971347436202 ) ) ;
#44861=CARTESIAN_POINT ( 'NONE',  ( 804.6971507214547046, -195.2817908451528410, -344.0799538623459739 ) ) ;
#44864=CARTESIAN_POINT ( 'NONE',  ( 777.4774526936600978, -370.2709662947830793, -304.7301800767028226 ) ) ;
#44870=CARTESIAN_POINT ( 'NONE',  ( 792.2312462859673587, -11.90732993114778182, -307.2067596250082602 ) ) ;
#44871=CARTESIAN_POINT ( 'NONE',  ( 754.8072714833581358, -244.8164208402378961, -338.1981804954720587 ) ) ;
#44875=CARTESIAN_POINT ( 'NONE',  ( 765.8855110935204493, -46.16923265350568784, -319.0159684113471599 ) ) ;
#44883=CARTESIAN_POINT ( 'NONE',  ( 762.1405469898971887, -73.54369356751118403, -357.8594530101015607 ) ) ;
#44884=CARTESIAN_POINT ( 'NONE',  ( 773.3843516231979720, -373.4419599262319593, -364.4086373105754433 ) ) ;
#44888=CARTESIAN_POINT ( 'NONE',  ( 814.8230680027162407, -365.8055962898682765, -333.7305795820267917 ) ) ;
#44894=CARTESIAN_POINT ( 'NONE',  ( 767.6429770376289525, -225.1800572038743269, -306.8695393053162093 ) ) ;
#44897=CARTESIAN_POINT ( 'NONE',  ( 804.9363028652555840, -208.2709662947835341, -338.2165204200192079 ) ) ;
#44900=CARTESIAN_POINT ( 'NONE',  ( 755.0636971347428243, -316.2709662947832499, -341.7834795799807353 ) ) ;
#44901=CARTESIAN_POINT ( 'NONE',  ( 768.0187753319979720, 15.36539734157940629, -318.0580252608186242 ) ) ;
#44905=CARTESIAN_POINT ( 'NONE',  ( 799.9999999999993179, -512.9681489794448908, -350.0000000000000000 ) ) ;
#44907=CARTESIAN_POINT ( 'NONE',  ( 763.8424801807145741, -450.0090635724248500, -320.5453621957614700 ) ) ;
#44911=CARTESIAN_POINT ( 'NONE',  ( 749.5768839229115201, -252.5545181178799226, -358.0661480581553064 ) ) ;
#44914=CARTESIAN_POINT ( 'NONE',  ( 756.5762568750052424, -219.1800572038744122, -348.7366044899774238 ) ) ;
#44915=CARTESIAN_POINT ( 'NONE',  ( 761.2382568024794409, -351.6237781080502032, -356.9571628226838129 ) ) ;
#44916=CARTESIAN_POINT ( 'NONE',  ( 778.7629533639073998, -248.7363362996981380, -375.0009284576466371 ) ) ;
#44919=CARTESIAN_POINT ( 'NONE',  ( 769.9779781133707957, -91.09997266333496668, -316.7813123517150871 ) ) ;
#44922=CARTESIAN_POINT ( 'NONE',  ( 761.2382568024794409, -423.6237781080499190, -356.9571628226838129 ) ) ;
#44923=CARTESIAN_POINT ( 'NONE',  ( 796.7737145352015204, -260.6346026584197375, -370.7187646348536987 ) ) ;
#44926=CARTESIAN_POINT ( 'NONE',  ( 800.0135310231082713, -38.08914811296587999, -325.0180583372163028 ) ) ;
#44928=CARTESIAN_POINT ( 'NONE',  ( 795.6651683502461765, -178.7146871989598083, -371.3240766477733814 ) ) ;
#44930=CARTESIAN_POINT ( 'NONE',  ( 772.4837098697144029, -407.3618753856920307, -374.5518280994205611 ) ) ;
#44935=CARTESIAN_POINT ( 'NONE',  ( 803.6646147819161570, -425.9073299311463074, -348.8264449731210561 ) ) ;
#44942=ADVANCED_FACE ( 'NONE', ( #39198 ), #7548, .F. ) ;
#44943=CARTESIAN_POINT ( 'NONE',  ( 780.5290396650775619, -276.3510508353231785, -365.2837595273619513 ) ) ;
#44944=CARTESIAN_POINT ( 'NONE',  ( 762.3223304703356007, -127.5436935675110561, -322.3223304703362828 ) ) ;
#44946=CARTESIAN_POINT ( 'NONE',  ( 815.0009284576459549, -270.3510508353231216, -338.7629533639073429 ) ) ;
#44952=CARTESIAN_POINT ( 'NONE',  ( 755.3201227861273992, -171.7255117493291152, -345.3687786644892981 ) ) ;
#44954=CARTESIAN_POINT ( 'NONE',  ( 763.0537975583475827, -120.4527844766019484, -371.0346526505627480 ) ) ;
#44955=CARTESIAN_POINT ( 'NONE',  ( 788.8264449731201466, -117.1800572038747106, -363.6646147819170665 ) ) ;
#44957=CARTESIAN_POINT ( 'NONE',  ( 758.4439275373578084, -36.55451811788061178, -353.2243759319684386 ) ) ;
#44958=CARTESIAN_POINT ( 'NONE',  ( 758.4439275373578084, -348.5545181178796383, -353.2243759319684386 ) ) ;
#44966=CARTESIAN_POINT ( 'NONE',  ( 754.7162404726377645, -374.7363362996978253, -339.4709603349214717 ) ) ;
#44967=CARTESIAN_POINT ( 'NONE',  ( 781.7834795799800531, -370.8164208402375834, -315.0636971347436202 ) ) ;
#44968=CARTESIAN_POINT ( 'NONE',  ( 811.3240766477731540, -124.3726999360621619, -355.6651683502462902 ) ) ;
#44973=CARTESIAN_POINT ( 'NONE',  ( 773.3843516231979720, -253.4419599262323572, -364.4086373105754433 ) ) ;
#44974=CARTESIAN_POINT ( 'NONE',  ( 749.5768839229115201, -156.5545181178802636, -358.0661480581553064 ) ) ;
#44980=CARTESIAN_POINT ( 'NONE',  ( 767.7687537140311633, -167.9073299311473022, -372.7932403749916830 ) ) ;
#44983=CARTESIAN_POINT ( 'NONE',  ( 787.5162901302840055, -299.3618753856922581, -305.4481719005792684 ) ) ;
#44990=CARTESIAN_POINT ( 'NONE',  ( 747.3154664389472828, -379.9874144716865203, -326.4474001241230781 ) ) ;
#44991=CARTESIAN_POINT ( 'NONE',  ( 767.6429770376289525, -129.1800572038746111, -306.8695393053162093 ) ) ;
#44993=CARTESIAN_POINT ( 'NONE',  ( 787.4397851343537695, -381.7255117493284615, -374.2001403089903988 ) ) ;
#44997=EDGE_CURVE ( 'NONE', #38426, #23858, #22521, .T. ) ;
#44998=CARTESIAN_POINT ( 'NONE',  ( 764.3348316497523456, -142.7146871989599219, -308.6759233522265617 ) ) ;
#45003=CARTESIAN_POINT ( 'NONE',  ( 755.8398074228967971, 4.558040073766884248, -333.4516893846970333 ) ) ;
#45005=CARTESIAN_POINT ( 'NONE',  ( 751.9810565676468741, -2.089148112965993231, -360.9747183278973921 ) ) ;
#45010=CARTESIAN_POINT ( 'NONE',  ( 788.7366044899766848, -179.9073299311472454, -316.5762568750059813 ) ) ;
#45011=CARTESIAN_POINT ( 'NONE',  ( 768.9521613784389729, -417.8272453906067199, -373.2346286133773106 ) ) ;
#45014=CARTESIAN_POINT ( 'NONE',  ( 762.1405469898971887, -265.5436935675106156, -357.8594530101015607 ) ) ;
#45018=CARTESIAN_POINT ( 'NONE',  ( 757.4527132478984868, -256.3726999360617924, -329.1273215169538844 ) ) ;
#45019=CARTESIAN_POINT ( 'NONE',  ( 788.7366044899766848, -227.9073299311471033, -316.5762568750059813 ) ) ;
#45020=CARTESIAN_POINT ( 'NONE',  ( 759.9864689768902508, -434.0891481129646081, -354.9819416627836404 ) ) ;
#45025=CARTESIAN_POINT ( 'NONE',  ( 757.7880784355613741, -66.00906357242595845, -312.4576283171834916 ) ) ;
#45030=CARTESIAN_POINT ( 'NONE',  ( 799.2566176426618085, -24.00906357242609346, -324.0069404352559559 ) ) ;
#45031=CARTESIAN_POINT ( 'NONE',  ( 787.5162901302840055, -83.36187538569299704, -305.4481719005793252 ) ) ;
#45033=CARTESIAN_POINT ( 'NONE',  ( 774.6858677611749044, -417.7255117493283478, -315.5713283507209894 ) ) ;
#45034=CARTESIAN_POINT ( 'NONE',  ( 804.9363028652555840, -40.27096629478405987, -338.2165204200192079 ) ) ;
#45037=CARTESIAN_POINT ( 'NONE',  ( 797.8594530101008786, 10.45630643248850866, -322.1405469898980982 ) ) ;
#45038=CARTESIAN_POINT ( 'NONE',  ( 813.1304606946830518, -185.9073299311472454, -352.3570229623690580 ) ) ;
#45043=DIRECTION ( 'NONE',  ( 1.000000000000000000, 0.000000000000000000, 0.000000000000000000 ) ) ;
#45044=CARTESIAN_POINT ( 'NONE',  ( 748.3538107759620743, -256.7146871989595525, -355.8262568251490165 ) ) ;
#45046=CARTESIAN_POINT ( 'NONE',  ( 813.1304606946830518, -281.9073299311468759, -352.3570229623690580 ) ) ;
#45050=CARTESIAN_POINT ( 'NONE',  ( 764.8639956371174549, -344.0891481129647786, -319.7806653035542013 ) ) ;
#45053=CARTESIAN_POINT ( 'NONE',  ( 759.8311093483677041, -46.16923265350568784, -310.9282345327691814 ) ) ;
#45054=CARTESIAN_POINT ( 'NONE',  ( 758.6633372737375112, -140.5328690171417634, -326.9102291470432533 ) ) ;
#45058=CARTESIAN_POINT ( 'NONE',  ( 758.0580252608178853, -78.45278447660211896, -328.0187753319985404 ) ) ;
#45059=CARTESIAN_POINT ( 'NONE',  ( 798.7617431975189675, -171.6237781080507432, -323.0428371773161871 ) ) ;
#45063=CARTESIAN_POINT ( 'NONE',  ( 776.2433038121456548, 11.10349461922141145, -374.8207195650711014 ) ) ;
#45069=CARTESIAN_POINT ( 'NONE',  ( 810.4231160770870019, -312.5545181178797520, -321.9338519418446936 ) ) ;
#45074=CARTESIAN_POINT ( 'NONE',  ( 787.5531968255692163, -165.8272453906074873, -316.1348686366205811 ) ) ;
#45075=CARTESIAN_POINT ( 'NONE',  ( 768.0187753319979720, -128.6346026584201354, -318.0580252608186242 ) ) ;
#45076=CARTESIAN_POINT ( 'NONE',  ( 804.6798772138710092, -327.7255117493285752, -334.6312213355106451 ) ) ;
#45084=CARTESIAN_POINT ( 'NONE',  ( 755.8990559732751535, -347.4636090269705733, -365.9055244015606831 ) ) ;
#45086=CARTESIAN_POINT ( 'NONE',  ( 795.1360043628807261, -332.0891481129649492, -360.2193346964456282 ) ) ;
#45088=FACE_OUTER_BOUND ( 'NONE', #8182, .T. ) ;
#45089=CARTESIAN_POINT ( 'NONE',  ( 769.0155153010367712, -178.3726999360619629, -362.7791456095907279 ) ) ;
#45092=CARTESIAN_POINT ( 'NONE',  ( 745.7998596910086917, -389.3618753856919739, -332.5602148656461168 ) ) ;
#45097=CARTESIAN_POINT ( 'NONE',  ( 746.8695393053150156, -5.907329931147798696, -327.6429770376306010 ) ) ;
#45099=CARTESIAN_POINT ( 'NONE',  ( 803.4237431249931660, -255.1800572038742700, -331.2633955100225194 ) ) ;
#45103=CARTESIAN_POINT ( 'NONE',  ( 760.0363995740630116, -34.91815448151697154, -368.7758568127991907 ) ) ;
#45104=CARTESIAN_POINT ( 'NONE',  ( 755.0488828828309806, -41.80559628986934229, -344.1219089521771934 ) ) ;
#45111=CARTESIAN_POINT ( 'NONE',  ( 762.3223304703356007, -79.54369356751119824, -322.3223304703362828 ) ) ;
#45112=CARTESIAN_POINT ( 'NONE',  ( 766.7756240680305382, -350.5328690171411381, -361.5560724626415663 ) ) ;
#45116=CARTESIAN_POINT ( 'NONE',  ( 783.7566961878529810, -360.8965053807773984, -305.1792804349288417 ) ) ;
#45121=CARTESIAN_POINT ( 'NONE',  ( 805.0032342141412300, -229.5436935675106440, -314.9967657858571783 ) ) ;
#45124=CARTESIAN_POINT ( 'NONE',  ( 804.6798772138710092, -207.7255117493289731, -334.6312213355106451 ) ) ;
#45126=CARTESIAN_POINT ( 'NONE',  ( 781.8018195045266339, -310.2709662947832499, -365.1927285166406705 ) ) ;
#45127=CARTESIAN_POINT ( 'NONE',  ( 801.9419747391806368, -18.45278447660230725, -351.9812246680014027 ) ) ;
#45132=CARTESIAN_POINT ( 'NONE',  ( 771.1735550268778070, 14.81994279612486309, -316.3353852180827630 ) ) ;
#45135=CARTESIAN_POINT ( 'NONE',  ( 807.2620300519052989, -240.0090635724253900, -318.0141637701419768 ) ) ;
#45138=CARTESIAN_POINT ( 'NONE',  ( 803.4237431249931660, -231.1800572038743553, -331.2633955100225194 ) ) ;
#45139=CARTESIAN_POINT ( 'NONE',  ( 805.0264073115434940, -414.3510508353227237, -339.4763451958999099 ) ) ;
#45142=CARTESIAN_POINT ( 'NONE',  ( 794.9819416627830151, 11.00176097794305541, -319.9864689768909898 ) ) ;
#45143=CARTESIAN_POINT ( 'NONE',  ( 763.0428371773158460, -83.46360902697136908, -358.7617431975195359 ) ) ;
#45146=CARTESIAN_POINT ( 'NONE',  ( 812.6845335610512393, 16.01258552831230375, -353.5525998758768651 ) ) ;
#45147=CARTESIAN_POINT ( 'NONE',  ( 745.0891759886404770, -292.2709662947831930, -342.4968714119734159 ) ) ;
#45150=CARTESIAN_POINT ( 'NONE',  ( 755.0636971347428243, -76.27096629478394618, -341.7834795799807353 ) ) ;
#45152=CARTESIAN_POINT ( 'NONE',  ( 813.2346286133761168, -173.2601417444143692, -328.9521613784389160 ) ) ;
#45154=CARTESIAN_POINT ( 'NONE',  ( 810.7187646348534145, -426.4527844766010389, -356.7737145352016341 ) ) ;
#45155=DIRECTION ( 'NONE',  ( 0.000000000000000000, -1.000000000000000000, 1.056348263647623421E-15 ) ) ;
#45158=CARTESIAN_POINT ( 'NONE',  ( 774.6858677611749044, -441.7255117493282910, -315.5713283507209894 ) ) ;
#45159=CARTESIAN_POINT ( 'NONE',  ( 799.9999999999993179, -512.9681489794448908, -339.9999999999999432 ) ) ;
#45160=FACE_OUTER_BOUND ( 'NONE', #32980, .T. ) ;
#45164=CARTESIAN_POINT ( 'NONE',  ( 759.2295555964440155, -256.1692326535049915, -353.9708237608231229 ) ) ;
#45168=CARTESIAN_POINT ( 'NONE',  ( 814.8230680027162407, -245.8055962898686460, -333.7305795820267917 ) ) ;
#45173=CARTESIAN_POINT ( 'NONE',  ( 800.0135310231082713, -158.0891481129655176, -325.0180583372163028 ) ) ;
#45175=CARTESIAN_POINT ( 'NONE',  ( 792.3570229623688874, -117.1800572038746964, -373.1304606946836202 ) ) ;
#45176=CARTESIAN_POINT ( 'NONE',  ( 771.2633955100217236, -95.90732993114751537, -363.4237431249939618 ) ) ;
#45178=CARTESIAN_POINT ( 'NONE',  ( 757.0176451133909268, -61.09997266333506616, -349.9200121543848354 ) ) ;
#45179=CARTESIAN_POINT ( 'NONE',  ( 769.0155153010367712, -346.3726999360614514, -362.7791456095907279 ) ) ;
#45186=CARTESIAN_POINT ( 'NONE',  ( 760.7433823573367135, -372.0090635724250205, -355.9930595647440441 ) ) ;
#45187=CARTESIAN_POINT ( 'NONE',  ( 785.3141322388236176, -357.7255117493285184, -364.4286716492789537 ) ) ;
#45188=CIRCLE ( 'NONE', #25261, 30.00000000000008171 ) ;
#45189=CARTESIAN_POINT ( 'NONE',  ( 814.4686193811664907, -123.2817908451530542, -346.2056067578752732 ) ) ;
#45193=CARTESIAN_POINT ( 'NONE',  ( 755.0488828828309806, -281.8055962898686175, -344.1219089521771934 ) ) ;
#45194=CARTESIAN_POINT ( 'NONE',  ( 809.0717654672305343, -148.9181544815166092, -360.1688906516309885 ) ) ;
#45199=CARTESIAN_POINT ( 'NONE',  ( 763.2262854647970016, -176.6346026584199933, -309.2812353651462445 ) ) ;
#45202=CARTESIAN_POINT ( 'NONE',  ( 763.2262854647970016, -320.6346026584195670, -309.2812353651462445 ) ) ;
#45208=CARTESIAN_POINT ( 'NONE',  ( 783.7566961878529810, -360.8965053807773984, -305.1792804349288417 ) ) ;
#45209=CARTESIAN_POINT ( 'NONE',  ( 812.7932403749906598, -135.1800572038746679, -327.7687537140311633 ) ) ;
#45211=CARTESIAN_POINT ( 'NONE',  ( 811.0346526505616112, -398.6346026584193396, -323.0537975583477532 ) ) ;
#45216=CARTESIAN_POINT ( 'NONE',  ( 747.3154664389472828, -139.9874144716872024, -326.4474001241230781 ) ) ;
#45220=PRODUCT_DEFINITION_FORMATION_WITH_SPECIFIED_SOURCE ( 'ANY', '', #26963, .NOT_KNOWN. ) ;
#45223=CARTESIAN_POINT ( 'NONE',  ( 814.9108240113580450, 7.729033705215793582, -337.5031285880265273 ) ) ;
#45227=CARTESIAN_POINT ( 'NONE',  ( 801.9419747391806368, -186.4527844766017779, -351.9812246680014027 ) ) ;
#45228=CARTESIAN_POINT ( 'NONE',  ( 749.5768839229115201, -420.5545181178793541, -358.0661480581553064 ) ) ;
#45230=CARTESIAN_POINT ( 'NONE',  ( 754.8072714833581358, -244.8164208402378961, -338.1981804954720587 ) ) ;
#45234=CARTESIAN_POINT ( 'NONE',  ( 761.4292242960306112, -257.4636090269708575, -323.2154366446414429 ) ) ;
#45235=CARTESIAN_POINT ( 'NONE',  ( 759.9864689768902508, -266.0891481129651197, -354.9819416627836404 ) ) ;
#45236=CARTESIAN_POINT ( 'NONE',  ( 767.8955696845334842, -408.4527844766009821, -362.1676090361161755 ) ) ;
#45237=CARTESIAN_POINT ( 'NONE',  ( 757.8323909638827445, -74.63460265842032015, -352.1044303154654358 ) ) ;
#45242=CARTESIAN_POINT ( 'NONE',  ( 813.5763878283155464, -51.82724539060782121, -351.1614460488615350 ) ) ;
#45249=CARTESIAN_POINT ( 'NONE',  ( 757.0176451133909268, -13.09997266333522248, -349.9200121543848354 ) ) ;
#45251=CARTESIAN_POINT ( 'NONE',  ( 811.0346526505617248, -86.63460265842024910, -323.0537975583478101 ) ) ;
#45253=CARTESIAN_POINT ( 'NONE',  ( 781.7834795799800531, -418.8164208402374129, -315.0636971347436202 ) ) ;
#45254=CARTESIAN_POINT ( 'NONE',  ( 795.1360043628808398, -44.08914811296585157, -360.2193346964456282 ) ) ;
#45256=CARTESIAN_POINT ( 'NONE',  ( 754.9967657858570647, -193.5436935675108714, -365.0032342141425374 ) ) ;
#45261=CARTESIAN_POINT ( 'NONE',  ( 788.7631598425961101, -265.4419599262323004, -305.7194118038759143 ) ) ;
#45265=CARTESIAN_POINT ( 'NONE',  ( 787.4397851343537695, -285.7255117493286889, -374.2001403089903988 ) ) ;
#45269=CARTESIAN_POINT ( 'NONE',  ( 803.4237431249931660, -399.1800572038738437, -331.2633955100225194 ) ) ;
#45272=CARTESIAN_POINT ( 'NONE',  ( 776.2433038121456548, -60.89650538077837894, -374.8207195650711014 ) ) ;
#45273=CARTESIAN_POINT ( 'NONE',  ( 801.3366627262608972, -152.5328690171416781, -353.0897708529566899 ) ) ;
#45278=CARTESIAN_POINT ( 'NONE',  ( 792.1044303154645831, -60.45278447660215448, -317.8323909638837677 ) ) ;
#45279=CARTESIAN_POINT ( 'NONE',  ( 770.0799878456142551, -181.9874144716870887, -362.9823548866085616 ) ) ;
#45281=CARTESIAN_POINT ( 'NONE',  ( 766.5853460496234675, 10.01258552831232329, -372.3518521366060554 ) ) ;
#45288=CARTESIAN_POINT ( 'NONE',  ( 811.3240766477731540, -292.3726999360616219, -355.6651683502462902 ) ) ;
#45291=EDGE_CURVE ( 'NONE', #27172, #45689, #35678, .T. ) ;
#45294=CARTESIAN_POINT ( 'NONE',  ( 755.3028492785439312, -159.2817908451529547, -335.9200461376539693 ) ) ;
#45295=CARTESIAN_POINT ( 'NONE',  ( 785.3141322388236176, -165.7255117493291152, -364.4286716492789537 ) ) ;
#45296=CARTESIAN_POINT ( 'NONE',  ( 781.7834795799800531, -298.8164208402377540, -315.0636971347436202 ) ) ;
#45304=CARTESIAN_POINT ( 'NONE',  ( 788.6739635108323228, -367.6454272087886466, -373.9316612368139090 ) ) ;
#45308=CARTESIAN_POINT ( 'NONE',  ( 764.8639956371174549, -344.0891481129647786, -319.7806653035542013 ) ) ;
#45310=CARTESIAN_POINT ( 'NONE',  ( 796.1575198192839480, -222.0090635724254184, -359.4546378042384163 ) ) ;
#45313=CARTESIAN_POINT ( 'NONE',  ( 782.4968714119720516, -418.8164208402374129, -305.0891759886411023 ) ) ;
#45315=CARTESIAN_POINT ( 'NONE',  ( 799.9999999999993179, -512.9681489794448908, -309.9999999999998863 ) ) ;
#45321=CARTESIAN_POINT ( 'NONE',  ( 772.5602148656447525, -57.72551174932945628, -305.7998596910095443 ) ) ;
#45322=CARTESIAN_POINT ( 'NONE',  ( 785.3687786644884454, -275.3618753856923149, -315.3201227861279676 ) ) ;
#45326=CARTESIAN_POINT ( 'NONE',  ( 750.9282345327678740, -16.91815448151702839, -319.8311093483690115 ) ) ;
#45327=CARTESIAN_POINT ( 'NONE',  ( 759.2295555964440155, -64.16923265350563099, -353.9708237608231229 ) ) ;
#45334=CARTESIAN_POINT ( 'NONE',  ( 794.9819416627830151, -60.99823902205671544, -319.9864689768909898 ) ) ;
#45336=CARTESIAN_POINT ( 'NONE',  ( 770.0799878456142551, -349.9874144716865771, -362.9823548866085616 ) ) ;
#45340=CARTESIAN_POINT ( 'NONE',  ( 746.7653713866222915, -401.2601417444137155, -351.0478386215610271 ) ) ;
#45349=CARTESIAN_POINT ( 'NONE',  ( 808.0189434323515343, -230.0891481129652618, -319.0252816721025511 ) ) ;
#45354=CARTESIAN_POINT ( 'NONE',  ( 762.1405469898973024, -217.5436935675107293, -357.8594530101016176 ) ) ;
#45357=CARTESIAN_POINT ( 'NONE',  ( 804.6798772138708955, -375.7255117493283478, -334.6312213355107019 ) ) ;
#45358=CARTESIAN_POINT ( 'NONE',  ( 788.8264449731200330, 2.819942796124898177, -363.6646147819171233 ) ) ;
#45360=ADVANCED_FACE ( 'NONE', ( #3580 ), #7034, .F. ) ;
#45364=CARTESIAN_POINT ( 'NONE',  ( 785.3141322388236176, 2.274488250670355871, -364.4286716492789537 ) ) ;
#45367=CARTESIAN_POINT ( 'NONE',  ( 814.8207195650702488, -290.1908817542434349, -336.2433038121456548 ) ) ;
#45371=CARTESIAN_POINT ( 'NONE',  ( 774.6312213355099630, -215.3618753856925423, -364.6798772138717482 ) ) ;
#45372=CARTESIAN_POINT ( 'NONE',  ( 805.0264073115434940, -390.3510508353227237, -339.4763451958999099 ) ) ;
#45375=CARTESIAN_POINT ( 'NONE',  ( 804.4086373105744769, -73.64542720878957027, -333.3843516231986541 ) ) ;
#45379=CARTESIAN_POINT ( 'NONE',  ( 768.8385539511368734, 24.73985825558500551, -306.4236121716840557 ) ) ;
#45380=CARTESIAN_POINT ( 'NONE',  ( 814.5518280994195948, -303.7255117493286889, -332.4837098697145166 ) ) ;
#45383=CARTESIAN_POINT ( 'NONE',  ( 800.2193346964447755, -90.99823902205663728, -355.1360043628815788 ) ) ;
#45385=CARTESIAN_POINT ( 'NONE',  ( 751.2241431872005251, -160.1692326535053326, -359.9636004259367610 ) ) ;
#45387=CARTESIAN_POINT ( 'NONE',  ( 795.8262568251477660, 1.627300063937458408, -308.3538107759623585 ) ) ;
#45392=CARTESIAN_POINT ( 'NONE',  ( 788.7366044899766848, -419.9073299311465348, -316.5762568750059813 ) ) ;
#45399=CARTESIAN_POINT ( 'NONE',  ( 754.9735926884551418, -258.3510508353231785, -340.5236548041000333 ) ) ;
#45402=CARTESIAN_POINT ( 'NONE',  ( 800.1688906516307043, -274.1692326535049915, -369.0717654672308186 ) ) ;
#45408=CARTESIAN_POINT ( 'NONE',  ( 794.1144889064781864, -34.16923265350572336, -360.9840315886528401 ) ) ;
#45409=CARTESIAN_POINT ( 'NONE',  ( 756.3353852180819104, -173.9073299311472169, -331.1735550268788302 ) ) ;
#45410=CARTESIAN_POINT ( 'NONE',  ( 757.8323909638827445, -218.6346026584197944, -352.1044303154654358 ) ) ;
#45413=CARTESIAN_POINT ( 'NONE',  ( 812.7932403749906598, -111.1800572038747532, -327.7687537140311633 ) ) ;
#45414=CARTESIAN_POINT ( 'NONE',  ( 797.6776695296629214, -91.54369356751116982, -357.6776695296636603 ) ) ;
#45416=CARTESIAN_POINT ( 'NONE',  ( 769.9779781133707957, -43.09997266333511590, -316.7813123517150871 ) ) ;
#45417=CARTESIAN_POINT ( 'NONE',  ( 769.9779781133707957, -403.0999726633339719, -316.7813123517150871 ) ) ;
#45422=DIRECTION ( 'NONE',  ( 1.000000000000000000, 0.000000000000000000, -0.000000000000000000 ) ) ;
#45425=CARTESIAN_POINT ( 'NONE',  ( 766.0291762391763086, -346.9181544815160123, -360.7704444035551319 ) ) ;
#45426=CARTESIAN_POINT ( 'NONE',  ( 788.7366044899766848, -347.9073299311467053, -316.5762568750059813 ) ) ;
#45427=CARTESIAN_POINT ( 'NONE',  ( 810.4231160770870019, -144.5545181178802636, -321.9338519418446936 ) ) ;
#45432=CARTESIAN_POINT ( 'NONE',  ( 795.9930595647434757, -291.0783235625957559, -320.7433823573372820 ) ) ;
#45433=LINE ( 'NONE', #38970, #6280 ) ;
#45434=CARTESIAN_POINT ( 'NONE',  ( 754.3581564841646241, -137.4636090269711985, -316.1443688327762516 ) ) ;
#45440=CARTESIAN_POINT ( 'NONE',  ( 792.3570229623691148, -189.1800572038744690, -373.1304606946836770 ) ) ;
#45444=CARTESIAN_POINT ( 'NONE',  ( 777.4774526936600978, -298.2709662947830793, -304.7301800767027657 ) ) ;
#45449=ORIENTED_EDGE ( 'NONE', *, *, #25580, .T. ) ;
#45451=CARTESIAN_POINT ( 'NONE',  ( 793.4146539503750546, -361.9874144716864635, -307.6481478633938877 ) ) ;
#45452=CARTESIAN_POINT ( 'NONE',  ( 782.4968714119720516, -130.8164208402383224, -305.0891759886411023 ) ) ;
#45453=CARTESIAN_POINT ( 'NONE',  ( 805.0032342141412300, -397.5436935675100472, -314.9967657858571783 ) ) ;
#45457=CARTESIAN_POINT ( 'NONE',  ( 786.2056067578752163, -155.8055962898689586, -374.4686193811670023 ) ) ;
#45465=CARTESIAN_POINT ( 'NONE',  ( 777.5031285880264704, -22.81642084023865280, -374.9108240113588408 ) ) ;
#45469=CARTESIAN_POINT ( 'NONE',  ( 795.1360043628807261, -188.0891481129653187, -360.2193346964456282 ) ) ;
#45470=CARTESIAN_POINT ( 'NONE',  ( 762.1177392798416577, -426.5545181178794678, -309.8865473780659272 ) ) ;
#45474=CARTESIAN_POINT ( 'NONE',  ( 785.3141322388236176, -261.7255117493288026, -364.4286716492789537 ) ) ;
#45478=CARTESIAN_POINT ( 'NONE',  ( 786.5483106153019435, -247.6454272087890160, -364.1601925771022366 ) ) ;
#45479=CARTESIAN_POINT ( 'NONE',  ( 797.6776695296629214, -259.5436935675106156, -357.6776695296636603 ) ) ;
#45480=CARTESIAN_POINT ( 'NONE',  ( 805.1927285166399315, -448.8164208402372424, -341.8018195045277707 ) ) ;
#45481=CARTESIAN_POINT ( 'NONE',  ( 771.2633955100217236, -95.90732993114751537, -363.4237431249939618 ) ) ;
#45485=CARTESIAN_POINT ( 'NONE',  ( 752.7379699480933368, -36.00906357242605793, -361.9858362298580232 ) ) ;
#45492=CARTESIAN_POINT ( 'NONE',  ( 805.2837595273609850, -2.736336299698892027, -340.5290396650784714 ) ) ;
#45493=CARTESIAN_POINT ( 'NONE',  ( 810.7187646348534145, -66.45278447660216159, -356.7737145352016341 ) ) ;
#45495=CARTESIAN_POINT ( 'NONE',  ( 771.1735550268778070, -417.1800572038736163, -316.3353852180827630 ) ) ;
#45497=CARTESIAN_POINT ( 'NONE',  ( 801.1904061080336987, -212.0891481129652902, -368.3070685750235498 ) ) ;
#45504=CARTESIAN_POINT ( 'NONE',  ( 756.1443688327750579, -285.6237781080502600, -314.3581564841659315 ) ) ;
#45507=CARTESIAN_POINT ( 'NONE',  ( 777.5031285880264704, -286.8164208402378677, -374.9108240113588408 ) ) ;
#45508=CARTESIAN_POINT ( 'NONE',  ( 779.9999999999992042, -452.9681489794448339, -339.9999999999999432 ) ) ;
#45511=CARTESIAN_POINT ( 'NONE',  ( 765.0180583372156207, -384.9982390220556567, -360.0135310231089534 ) ) ;
#45514=CARTESIAN_POINT ( 'NONE',  ( 771.1735550268778070, -201.1800572038744690, -316.3353852180827630 ) ) ;
#45515=CARTESIAN_POINT ( 'NONE',  ( 746.7653713866222915, -41.26014174441479554, -351.0478386215610271 ) ) ;
#45516=CARTESIAN_POINT ( 'NONE',  ( 798.7617431975189675, -195.6237781080506863, -323.0428371773161871 ) ) ;
#45519=CARTESIAN_POINT ( 'NONE',  ( 763.2154366446407039, -189.6237781080507148, -321.4292242960311228 ) ) ;
#45523=CARTESIAN_POINT ( 'NONE',  ( 791.1614460488616487, -35.26014174441480264, -373.5763878283158874 ) ) ;
#45528=CARTESIAN_POINT ( 'NONE',  ( 750.9282345327678740, -304.9181544815161828, -319.8311093483690115 ) ) ;
#45533=CARTESIAN_POINT ( 'NONE',  ( 798.5707757039680246, -149.4636090269711417, -356.7845633553585003 ) ) ;
#45534=CARTESIAN_POINT ( 'NONE',  ( 774.6858677611749044, -153.7255117493291721, -315.5713283507209894 ) ) ;
#45535=CARTESIAN_POINT ( 'NONE',  ( 781.8018195045267476, -334.2709662947830793, -365.1927285166407273 ) ) ;
#45537=CARTESIAN_POINT ( 'NONE',  ( 803.4237431249931660, -447.1800572038736732, -331.2633955100225194 ) ) ;
#45545=CARTESIAN_POINT ( 'NONE',  ( 812.3518521366052028, -361.0999726633341425, -326.5853460496235243 ) ) ;
#45550=CARTESIAN_POINT ( 'NONE',  ( 800.2193346964447755, -330.9982390220558273, -355.1360043628815788 ) ) ;
#45552=CARTESIAN_POINT ( 'NONE',  ( 761.4292242960306112, -209.4636090269709996, -323.2154366446414429 ) ) ;
#45555=CARTESIAN_POINT ( 'NONE',  ( 792.2312462859673587, -419.9073299311465348, -307.2067596250082602 ) ) ;
#45558=CARTESIAN_POINT ( 'NONE',  ( 791.4804426738954817, -453.0432664090020580, -367.7164109511201673 ) ) ;
#45560=CARTESIAN_POINT ( 'NONE',  ( 815.2698199232961542, -40.81642084023859951, -342.5225473063383106 ) ) ;
#45561=CARTESIAN_POINT ( 'NONE',  ( 756.3353852180819104, -293.9073299311468759, -331.1735550268788302 ) ) ;
#45567=CARTESIAN_POINT ( 'NONE',  ( 783.7953271457878373, -32.19088175424425913, -375.1787889125761239 ) ) ;
#45568=CARTESIAN_POINT ( 'NONE',  ( 793.2243759319678702, -98.53286901714187707, -318.4439275373583200 ) ) ;
#45574=CARTESIAN_POINT ( 'NONE',  ( 800.7704444035546203, -100.1692326535055315, -326.0291762391768771 ) ) ;
#45576=CARTESIAN_POINT ( 'NONE',  ( 754.8072714833581358, -52.81642084023856398, -338.1981804954720587 ) ) ;
#45578=ADVANCED_FACE ( 'NONE', ( #4288 ), #18379, .T. ) ;
#45579=CARTESIAN_POINT ( 'NONE',  ( 772.3691319403857278, -359.2601417444137724, -315.8894580844506663 ) ) ;
#45582=CARTESIAN_POINT ( 'NONE',  ( 810.1134526219336749, -392.5328690171409107, -357.8822607201570349 ) ) ;
#45584=ORIENTED_EDGE ( 'NONE', *, *, #34065, .T. ) ;
#45587=CARTESIAN_POINT ( 'NONE',  ( 787.4397851343537695, -237.7255117493289163, -374.2001403089903988 ) ) ;
#45591=CARTESIAN_POINT ( 'NONE',  ( 785.3141322388236176, -213.7255117493289731, -364.4286716492789537 ) ) ;
#45593=EDGE_CURVE ( 'NONE', #27172, #18205, #43517, .T. ) ;
#45594=CARTESIAN_POINT ( 'NONE',  ( 803.4237431249931660, -351.1800572038740142, -331.2633955100225194 ) ) ;
#45595=CARTESIAN_POINT ( 'NONE',  ( 771.2633955100217236, 0.09267006885218045942, -363.4237431249939618 ) ) ;
#45599=DIRECTION ( 'NONE',  ( 1.000000000000000000, 0.000000000000000000, -0.000000000000000000 ) ) ;
#45601=CARTESIAN_POINT ( 'NONE',  ( 794.9819416627830151, 11.00176097794305541, -319.9864689768909898 ) ) ;
#45602=DIRECTION ( 'NONE',  ( -0.3826814224632280603, -1.110223024625159854E-14, 0.9238803650373355048 ) ) ;
#45605=CARTESIAN_POINT ( 'NONE',  ( 809.0717654672305343, -268.9181544815162397, -360.1688906516309885 ) ) ;
#45609=CARTESIAN_POINT ( 'NONE',  ( 765.0180583372156207, -216.9982390220562252, -360.0135310231089534 ) ) ;
#45610=CARTESIAN_POINT ( 'NONE',  ( 769.1273215169530886, -406.7146871989590409, -317.4527132478988847 ) ) ;
#45613=CARTESIAN_POINT ( 'NONE',  ( 755.8894580844503253, -111.8272453906076151, -332.3691319403863531 ) ) ;
#45616=CARTESIAN_POINT ( 'NONE',  ( 793.4146539503750546, 22.01258552831228599, -307.6481478633938877 ) ) ;
#45617=CARTESIAN_POINT ( 'NONE',  ( 800.9747183278959710, -300.9982390220559409, -311.9810565676471583 ) ) ;
#45618=DIRECTION ( 'NONE',  ( 0.000000000000000000, 0.000000000000000000, -1.000000000000000000 ) ) ;
#45620=CARTESIAN_POINT ( 'NONE',  ( 805.1927285166397041, -88.81642084023842187, -341.8018195045277707 ) ) ;
#45623=CARTESIAN_POINT ( 'NONE',  ( 793.4146539503750546, -217.9874144716870035, -307.6481478633938877 ) ) ;
#45625=CARTESIAN_POINT ( 'NONE',  ( 746.8695393053150156, -437.9073299311463074, -327.6429770376306010 ) ) ;
#45630=CARTESIAN_POINT ( 'NONE',  ( 762.3223304703356007, -439.5436935675101040, -322.3223304703362828 ) ) ;
#45637=CARTESIAN_POINT ( 'NONE',  ( 798.7617431975189675, -267.6237781080504305, -323.0428371773161871 ) ) ;
#45639=CARTESIAN_POINT ( 'NONE',  ( 751.2241431872005251, -304.1692326535048210, -359.9636004259367610 ) ) ;
#45645=CARTESIAN_POINT ( 'NONE',  ( 803.2186876482843445, -55.98741447168748664, -350.0220218866286928 ) ) ;
#45646=CARTESIAN_POINT ( 'NONE',  ( 804.4286716492782716, -161.3618753856927697, -345.3141322388244703 ) ) ;
#45647=CARTESIAN_POINT ( 'NONE',  ( 803.6646147819161570, -209.9073299311470748, -348.8264449731210561 ) ) ;
#45649=CARTESIAN_POINT ( 'NONE',  ( 814.9108240113580450, -112.2709662947838325, -337.5031285880265273 ) ) ;
#45650=CARTESIAN_POINT ( 'NONE',  ( 755.3201227861273992, -123.7255117493292289, -345.3687786644892981 ) ) ;
#45652=CARTESIAN_POINT ( 'NONE',  ( 796.9571628226829034, -383.4636090269704596, -321.2382568024804641 ) ) ;
#45659=CARTESIAN_POINT ( 'NONE',  ( 769.0155153010367712, -346.3726999360614514, -362.7791456095907279 ) ) ;
#45660=CARTESIAN_POINT ( 'NONE',  ( 788.8264449731200330, -357.1800572038739006, -363.6646147819171233 ) ) ;
#45661=CARTESIAN_POINT ( 'NONE',  ( 788.6739635108323228, -151.6454272087892718, -373.9316612368139090 ) ) ;
#45664=CARTESIAN_POINT ( 'NONE',  ( 799.9999999999993179, 205.0000000000000568, -319.9999999999999432 ) ) ;
#45665=CARTESIAN_POINT ( 'NONE',  ( 787.6308680596127942, -299.2601417444139997, -364.1105419155492768 ) ) ;
#45667=CARTESIAN_POINT ( 'NONE',  ( 750.9282345327678740, -160.9181544815165807, -319.8311093483690115 ) ) ;
#45668=FACE_BOUND ( 'NONE', #38510, .T. ) ;
#45672=CARTESIAN_POINT ( 'NONE',  ( 787.5162901302840055, -203.3618753856926276, -305.4481719005793252 ) ) ;
#45677=CARTESIAN_POINT ( 'NONE',  ( 773.7943932421234194, -95.80559628986917176, -305.5313806188329409 ) ) ;
#45678=CARTESIAN_POINT ( 'NONE',  ( 814.9108240113580450, -352.2709662947830225, -337.5031285880265273 ) ) ;
#45684=CARTESIAN_POINT ( 'NONE',  ( 803.8556311672234642, -393.6237781080500326, -365.6418435158340117 ) ) ;
#45685=CARTESIAN_POINT ( 'NONE',  ( 759.0252816721024374, -144.9982390220564525, -368.0189434323527280 ) ) ;
#45686=CARTESIAN_POINT ( 'NONE',  ( 767.7687537140311633, -431.9073299311464211, -372.7932403749916830 ) ) ;
#45687=DIRECTION ( 'NONE',  ( 0.000000000000000000, -1.000000000000000000, 0.000000000000000000 ) ) ;
#45689=VERTEX_POINT ( 'NONE', #30800 ) ;
#45691=CARTESIAN_POINT ( 'NONE',  ( 751.2241431872005251, -184.1692326535052757, -359.9636004259367610 ) ) ;
#45697=CARTESIAN_POINT ( 'NONE',  ( 744.7301800767019131, -4.816420840238714085, -337.4774526936615757 ) ) ;
#45700=CARTESIAN_POINT ( 'NONE',  ( 766.4474001241216001, -403.0999726633339719, -307.3154664389482491 ) ) ;
#45705=CARTESIAN_POINT ( 'NONE',  ( 764.8639956371174549, -248.0891481129651481, -319.7806653035542013 ) ) ;
#45709=CARTESIAN_POINT ( 'NONE',  ( 758.0580252608178853, -246.4527844766016074, -328.0187753319985404 ) ) ;
#45710=CARTESIAN_POINT ( 'NONE',  ( 794.9819416627830151, -444.9982390220554862, -319.9864689768909898 ) ) ;
#45711=CARTESIAN_POINT ( 'NONE',  ( 768.0187753319979720, -104.6346026584202207, -318.0580252608186242 ) ) ;
#45715=CARTESIAN_POINT ( 'NONE',  ( 805.6418435158337843, -53.46360902697146855, -363.8556311672236916 ) ) ;
#45716=CARTESIAN_POINT ( 'NONE',  ( 779.9999999999992042, 126.4563064324884465, -350.0000000000000000 ) ) ;
#45721=CARTESIAN_POINT ( 'NONE',  ( 763.0428371773158460, -11.46360902697159290, -358.7617431975195359 ) ) ;
#45722=CARTESIAN_POINT ( 'NONE',  ( 796.7737145352015204, -92.63460265842026331, -370.7187646348536987 ) ) ;
#45759=COLOUR_RGB('Grey',0.48,0.52,0.57);
#45760=FILL_AREA_STYLE_COLOUR('',#45759);
#45761=FILL_AREA_STYLE('',(#45760));
#45762=SURFACE_STYLE_FILL_AREA(#45761);
#45763=SURFACE_SIDE_STYLE('',(#45762));
#45764=SURFACE_STYLE_USAGE(.BOTH.,#45763);
#45765=PRESENTATION_STYLE_ASSIGNMENT((#45764));
ENDSEC;
END-ISO-10303-21;
